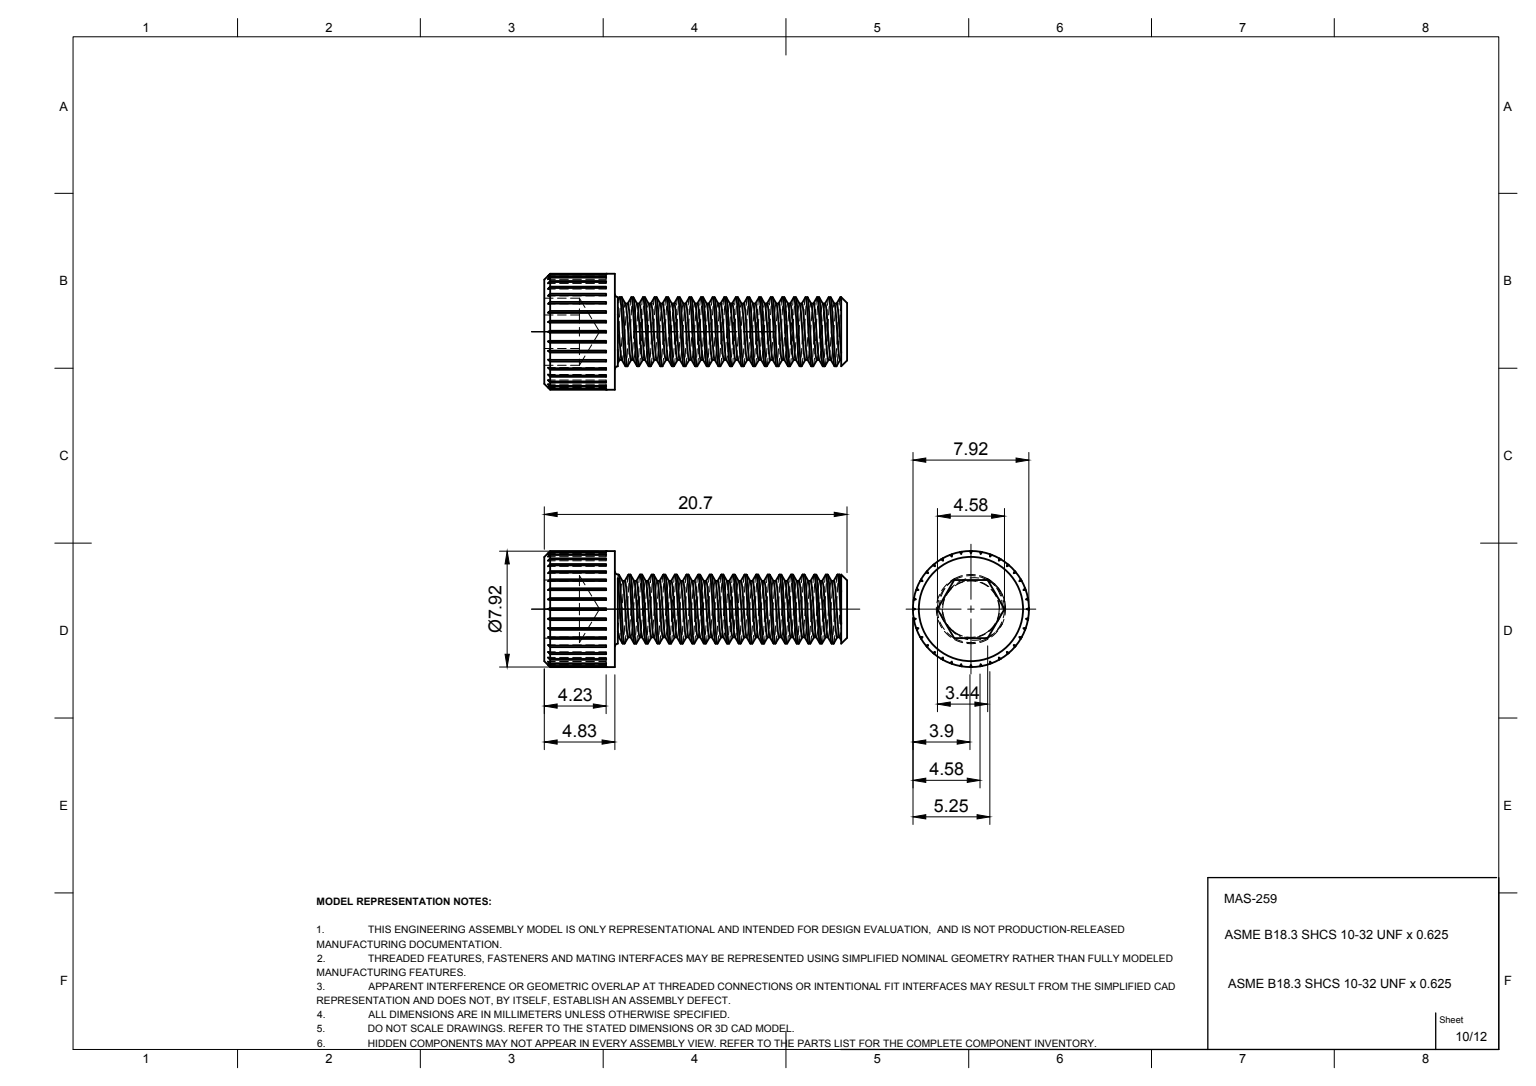
ISO-10303-21;
HEADER;
/* Generated by software containing ST-Developer
 * from STEP Tools, Inc. (www.steptools.com) 
 */

FILE_DESCRIPTION(
/* description */ (''),
/* implementation_level */ '2;1');

FILE_NAME(
/* name */ 'ASME B18.3 SHCS 10-32 UNF x 0.625.step',
/* time_stamp */ '2026-10-15T13:30:17-07:00',
/* author */ (''),
/* organization */ (''),
/* preprocessor_version */ 'ST-DEVELOPER v20.2',
/* originating_system */ 'Autodesk Translation Framework v15.15.0.0',
/* authorisation */ '');

FILE_SCHEMA (('AUTOMOTIVE_DESIGN { 1 0 10303 214 3 1 1 }'));
ENDSEC;

DATA;
#10=MECHANICAL_DESIGN_GEOMETRIC_PRESENTATION_REPRESENTATION('',(#1040),#71795);
#787=(
BOUNDED_CURVE()
B_SPLINE_CURVE(2,(#36530,#36531,#36532),.UNSPECIFIED.,.F.,.F.)
B_SPLINE_CURVE_WITH_KNOTS((3,3),(0.,0.021388782715503),.UNSPECIFIED.)
CURVE()
GEOMETRIC_REPRESENTATION_ITEM()
RATIONAL_B_SPLINE_CURVE((1.,1.00061453665269,1.00078646015663))
REPRESENTATION_ITEM('')
);
#788=(
BOUNDED_CURVE()
B_SPLINE_CURVE(2,(#36537,#36538,#36539),.UNSPECIFIED.,.F.,.F.)
B_SPLINE_CURVE_WITH_KNOTS((3,3),(0.0380048027322982,0.0593935854477557),
 .UNSPECIFIED.)
CURVE()
GEOMETRIC_REPRESENTATION_ITEM()
RATIONAL_B_SPLINE_CURVE((1.00078646015529,1.00061453665164,1.))
REPRESENTATION_ITEM('')
);
#789=(
BOUNDED_CURVE()
B_SPLINE_CURVE(2,(#36546,#36547,#36548),.UNSPECIFIED.,.F.,.F.)
B_SPLINE_CURVE_WITH_KNOTS((3,3),(0.0380048027323146,0.0593935854477557),
 .UNSPECIFIED.)
CURVE()
GEOMETRIC_REPRESENTATION_ITEM()
RATIONAL_B_SPLINE_CURVE((1.00078646015801,1.00061453665376,1.))
REPRESENTATION_ITEM('')
);
#790=(
BOUNDED_CURVE()
B_SPLINE_CURVE(2,(#36552,#36553,#36554),.UNSPECIFIED.,.F.,.F.)
B_SPLINE_CURVE_WITH_KNOTS((3,3),(0.,0.0213887827155079),.UNSPECIFIED.)
CURVE()
GEOMETRIC_REPRESENTATION_ITEM()
RATIONAL_B_SPLINE_CURVE((1.,1.00061453665303,1.00078646015707))
REPRESENTATION_ITEM('')
);
#791=(
BOUNDED_CURVE()
B_SPLINE_CURVE(2,(#36556,#36557,#36558),.UNSPECIFIED.,.F.,.F.)
B_SPLINE_CURVE_WITH_KNOTS((3,3),(0.03800480273222,0.0593935854477558),
 .UNSPECIFIED.)
CURVE()
GEOMETRIC_REPRESENTATION_ITEM()
RATIONAL_B_SPLINE_CURVE((1.00078646015217,1.0006145366492,1.))
REPRESENTATION_ITEM('')
);
#792=(
BOUNDED_CURVE()
B_SPLINE_CURVE(2,(#36562,#36563,#36564),.UNSPECIFIED.,.F.,.F.)
B_SPLINE_CURVE_WITH_KNOTS((3,3),(0.,0.0213887827155065),.UNSPECIFIED.)
CURVE()
GEOMETRIC_REPRESENTATION_ITEM()
RATIONAL_B_SPLINE_CURVE((1.,1.00061453664751,1.00078646015))
REPRESENTATION_ITEM('')
);
#793=(
BOUNDED_CURVE()
B_SPLINE_CURVE(2,(#36566,#36567,#36568),.UNSPECIFIED.,.F.,.F.)
B_SPLINE_CURVE_WITH_KNOTS((3,3),(0.0380048027322497,0.0593935854477559),
 .UNSPECIFIED.)
CURVE()
GEOMETRIC_REPRESENTATION_ITEM()
RATIONAL_B_SPLINE_CURVE((1.00078646015691,1.00061453665291,1.))
REPRESENTATION_ITEM('')
);
#794=(
BOUNDED_CURVE()
B_SPLINE_CURVE(2,(#36572,#36573,#36574),.UNSPECIFIED.,.F.,.F.)
B_SPLINE_CURVE_WITH_KNOTS((3,3),(0.,0.0213887827155146),.UNSPECIFIED.)
CURVE()
GEOMETRIC_REPRESENTATION_ITEM()
RATIONAL_B_SPLINE_CURVE((1.,1.00061453665095,1.00078646015441))
REPRESENTATION_ITEM('')
);
#795=(
BOUNDED_CURVE()
B_SPLINE_CURVE(2,(#36576,#36577,#36578),.UNSPECIFIED.,.F.,.F.)
B_SPLINE_CURVE_WITH_KNOTS((3,3),(0.0380048027321657,0.0593935854477561),
 .UNSPECIFIED.)
CURVE()
GEOMETRIC_REPRESENTATION_ITEM()
RATIONAL_B_SPLINE_CURVE((1.00078646014826,1.00061453664614,1.))
REPRESENTATION_ITEM('')
);
#796=(
BOUNDED_CURVE()
B_SPLINE_CURVE(2,(#36582,#36583,#36584),.UNSPECIFIED.,.F.,.F.)
B_SPLINE_CURVE_WITH_KNOTS((3,3),(0.,0.0213887827154277),.UNSPECIFIED.)
CURVE()
GEOMETRIC_REPRESENTATION_ITEM()
RATIONAL_B_SPLINE_CURVE((1.,1.00061453665233,1.00078646015617))
REPRESENTATION_ITEM('')
);
#797=(
BOUNDED_CURVE()
B_SPLINE_CURVE(2,(#36586,#36587,#36588),.UNSPECIFIED.,.F.,.F.)
B_SPLINE_CURVE_WITH_KNOTS((3,3),(0.0380048027322445,0.0593935854477552),
 .UNSPECIFIED.)
CURVE()
GEOMETRIC_REPRESENTATION_ITEM()
RATIONAL_B_SPLINE_CURVE((1.00078646015087,1.00061453664819,1.))
REPRESENTATION_ITEM('')
);
#798=(
BOUNDED_CURVE()
B_SPLINE_CURVE(2,(#36592,#36593,#36594),.UNSPECIFIED.,.F.,.F.)
B_SPLINE_CURVE_WITH_KNOTS((3,3),(0.,0.0213887827154996),.UNSPECIFIED.)
CURVE()
GEOMETRIC_REPRESENTATION_ITEM()
RATIONAL_B_SPLINE_CURVE((1.,1.00061453665179,1.00078646015549))
REPRESENTATION_ITEM('')
);
#799=(
BOUNDED_CURVE()
B_SPLINE_CURVE(2,(#36596,#36597,#36598),.UNSPECIFIED.,.F.,.F.)
B_SPLINE_CURVE_WITH_KNOTS((3,3),(0.0380048027322845,0.0593935854477556),
 .UNSPECIFIED.)
CURVE()
GEOMETRIC_REPRESENTATION_ITEM()
RATIONAL_B_SPLINE_CURVE((1.00078646015637,1.00061453665248,1.))
REPRESENTATION_ITEM('')
);
#800=(
BOUNDED_CURVE()
B_SPLINE_CURVE(2,(#36602,#36603,#36604),.UNSPECIFIED.,.F.,.F.)
B_SPLINE_CURVE_WITH_KNOTS((3,3),(0.,0.0213887827155547),.UNSPECIFIED.)
CURVE()
GEOMETRIC_REPRESENTATION_ITEM()
RATIONAL_B_SPLINE_CURVE((1.,1.00061453664528,1.00078646014716))
REPRESENTATION_ITEM('')
);
#801=(
BOUNDED_CURVE()
B_SPLINE_CURVE(2,(#36606,#36607,#36608),.UNSPECIFIED.,.F.,.F.)
B_SPLINE_CURVE_WITH_KNOTS((3,3),(0.0380048027322622,0.0593935854477563),
 .UNSPECIFIED.)
CURVE()
GEOMETRIC_REPRESENTATION_ITEM()
RATIONAL_B_SPLINE_CURVE((1.0007864601608,1.00061453665594,1.))
REPRESENTATION_ITEM('')
);
#802=(
BOUNDED_CURVE()
B_SPLINE_CURVE(2,(#36612,#36613,#36614),.UNSPECIFIED.,.F.,.F.)
B_SPLINE_CURVE_WITH_KNOTS((3,3),(0.,0.021388782715527),.UNSPECIFIED.)
CURVE()
GEOMETRIC_REPRESENTATION_ITEM()
RATIONAL_B_SPLINE_CURVE((1.,1.00061453664858,1.00078646015138))
REPRESENTATION_ITEM('')
);
#803=(
BOUNDED_CURVE()
B_SPLINE_CURVE(2,(#36616,#36617,#36618),.UNSPECIFIED.,.F.,.F.)
B_SPLINE_CURVE_WITH_KNOTS((3,3),(0.0380048027322087,0.0593935854477563),
 .UNSPECIFIED.)
CURVE()
GEOMETRIC_REPRESENTATION_ITEM()
RATIONAL_B_SPLINE_CURVE((1.00078646015349,1.00061453665023,1.))
REPRESENTATION_ITEM('')
);
#804=(
BOUNDED_CURVE()
B_SPLINE_CURVE(2,(#36622,#36623,#36624),.UNSPECIFIED.,.F.,.F.)
B_SPLINE_CURVE_WITH_KNOTS((3,3),(0.,0.0213887827155107),.UNSPECIFIED.)
CURVE()
GEOMETRIC_REPRESENTATION_ITEM()
RATIONAL_B_SPLINE_CURVE((1.,1.00061453665077,1.00078646015419))
REPRESENTATION_ITEM('')
);
#805=(
BOUNDED_CURVE()
B_SPLINE_CURVE(2,(#36626,#36627,#36628),.UNSPECIFIED.,.F.,.F.)
B_SPLINE_CURVE_WITH_KNOTS((3,3),(0.0380048027321878,0.0593935854477555),
 .UNSPECIFIED.)
CURVE()
GEOMETRIC_REPRESENTATION_ITEM()
RATIONAL_B_SPLINE_CURVE((1.00078646014641,1.0006145366447,1.))
REPRESENTATION_ITEM('')
);
#806=(
BOUNDED_CURVE()
B_SPLINE_CURVE(2,(#36632,#36633,#36634),.UNSPECIFIED.,.F.,.F.)
B_SPLINE_CURVE_WITH_KNOTS((3,3),(0.,0.0213887827154949),.UNSPECIFIED.)
CURVE()
GEOMETRIC_REPRESENTATION_ITEM()
RATIONAL_B_SPLINE_CURVE((1.,1.00061453665079,1.00078646015421))
REPRESENTATION_ITEM('')
);
#807=(
BOUNDED_CURVE()
B_SPLINE_CURVE(2,(#36636,#36637,#36638),.UNSPECIFIED.,.F.,.F.)
B_SPLINE_CURVE_WITH_KNOTS((3,3),(0.038004802732195,0.0593935854477556),
 .UNSPECIFIED.)
CURVE()
GEOMETRIC_REPRESENTATION_ITEM()
RATIONAL_B_SPLINE_CURVE((1.0007864601493,1.00061453664696,1.))
REPRESENTATION_ITEM('')
);
#808=(
BOUNDED_CURVE()
B_SPLINE_CURVE(2,(#36642,#36643,#36644),.UNSPECIFIED.,.F.,.F.)
B_SPLINE_CURVE_WITH_KNOTS((3,3),(0.,0.0213887827155322),.UNSPECIFIED.)
CURVE()
GEOMETRIC_REPRESENTATION_ITEM()
RATIONAL_B_SPLINE_CURVE((1.,1.00061453664703,1.00078646014939))
REPRESENTATION_ITEM('')
);
#809=(
BOUNDED_CURVE()
B_SPLINE_CURVE(2,(#36646,#36647,#36648),.UNSPECIFIED.,.F.,.F.)
B_SPLINE_CURVE_WITH_KNOTS((3,3),(0.0380048027322535,0.0593935854477551),
 .UNSPECIFIED.)
CURVE()
GEOMETRIC_REPRESENTATION_ITEM()
RATIONAL_B_SPLINE_CURVE((1.00078646015018,1.00061453664765,1.))
REPRESENTATION_ITEM('')
);
#810=(
BOUNDED_CURVE()
B_SPLINE_CURVE(2,(#36652,#36653,#36654),.UNSPECIFIED.,.F.,.F.)
B_SPLINE_CURVE_WITH_KNOTS((3,3),(0.,0.0213887827155291),.UNSPECIFIED.)
CURVE()
GEOMETRIC_REPRESENTATION_ITEM()
RATIONAL_B_SPLINE_CURVE((1.,1.00061453664596,1.00078646014803))
REPRESENTATION_ITEM('')
);
#811=(
BOUNDED_CURVE()
B_SPLINE_CURVE(2,(#36656,#36657,#36658),.UNSPECIFIED.,.F.,.F.)
B_SPLINE_CURVE_WITH_KNOTS((3,3),(0.0380048027322346,0.0593935854477561),
 .UNSPECIFIED.)
CURVE()
GEOMETRIC_REPRESENTATION_ITEM()
RATIONAL_B_SPLINE_CURVE((1.00078646015205,1.00061453664911,1.))
REPRESENTATION_ITEM('')
);
#812=(
BOUNDED_CURVE()
B_SPLINE_CURVE(2,(#36662,#36663,#36664),.UNSPECIFIED.,.F.,.F.)
B_SPLINE_CURVE_WITH_KNOTS((3,3),(0.,0.0213887827155096),.UNSPECIFIED.)
CURVE()
GEOMETRIC_REPRESENTATION_ITEM()
RATIONAL_B_SPLINE_CURVE((1.,1.00061453664827,1.00078646015098))
REPRESENTATION_ITEM('')
);
#813=(
BOUNDED_CURVE()
B_SPLINE_CURVE(2,(#36666,#36667,#36668),.UNSPECIFIED.,.F.,.F.)
B_SPLINE_CURVE_WITH_KNOTS((3,3),(0.0380048027322829,0.0593935854477556),
 .UNSPECIFIED.)
CURVE()
GEOMETRIC_REPRESENTATION_ITEM()
RATIONAL_B_SPLINE_CURVE((1.00078646015816,1.00061453665388,1.))
REPRESENTATION_ITEM('')
);
#814=(
BOUNDED_CURVE()
B_SPLINE_CURVE(2,(#36672,#36673,#36674),.UNSPECIFIED.,.F.,.F.)
B_SPLINE_CURVE_WITH_KNOTS((3,3),(0.,0.0213887827155543),.UNSPECIFIED.)
CURVE()
GEOMETRIC_REPRESENTATION_ITEM()
RATIONAL_B_SPLINE_CURVE((1.,1.00061453664662,1.00078646014886))
REPRESENTATION_ITEM('')
);
#815=(
BOUNDED_CURVE()
B_SPLINE_CURVE(2,(#36676,#36677,#36678),.UNSPECIFIED.,.F.,.F.)
B_SPLINE_CURVE_WITH_KNOTS((3,3),(0.038004802732242,0.0593935854477554),
 .UNSPECIFIED.)
CURVE()
GEOMETRIC_REPRESENTATION_ITEM()
RATIONAL_B_SPLINE_CURVE((1.00078646015479,1.00061453665125,1.))
REPRESENTATION_ITEM('')
);
#816=(
BOUNDED_CURVE()
B_SPLINE_CURVE(2,(#36682,#36683,#36684),.UNSPECIFIED.,.F.,.F.)
B_SPLINE_CURVE_WITH_KNOTS((3,3),(0.,0.0213887827155011),.UNSPECIFIED.)
CURVE()
GEOMETRIC_REPRESENTATION_ITEM()
RATIONAL_B_SPLINE_CURVE((1.,1.00061453665297,1.000786460157))
REPRESENTATION_ITEM('')
);
#817=(
BOUNDED_CURVE()
B_SPLINE_CURVE(2,(#36686,#36687,#36688),.UNSPECIFIED.,.F.,.F.)
B_SPLINE_CURVE_WITH_KNOTS((3,3),(0.0380048027323167,0.0593935854477549),
 .UNSPECIFIED.)
CURVE()
GEOMETRIC_REPRESENTATION_ITEM()
RATIONAL_B_SPLINE_CURVE((1.00078646015665,1.0006145366527,1.))
REPRESENTATION_ITEM('')
);
#818=(
BOUNDED_CURVE()
B_SPLINE_CURVE(2,(#36692,#36693,#36694),.UNSPECIFIED.,.F.,.F.)
B_SPLINE_CURVE_WITH_KNOTS((3,3),(0.,0.0213887827155084),.UNSPECIFIED.)
CURVE()
GEOMETRIC_REPRESENTATION_ITEM()
RATIONAL_B_SPLINE_CURVE((1.,1.00061453665162,1.00078646015527))
REPRESENTATION_ITEM('')
);
#819=(
BOUNDED_CURVE()
B_SPLINE_CURVE(2,(#36696,#36697,#36698),.UNSPECIFIED.,.F.,.F.)
B_SPLINE_CURVE_WITH_KNOTS((3,3),(0.0380048027322826,0.0593935854477556),
 .UNSPECIFIED.)
CURVE()
GEOMETRIC_REPRESENTATION_ITEM()
RATIONAL_B_SPLINE_CURVE((1.00078646015745,1.00061453665332,1.))
REPRESENTATION_ITEM('')
);
#820=(
BOUNDED_CURVE()
B_SPLINE_CURVE(2,(#36702,#36703,#36704),.UNSPECIFIED.,.F.,.F.)
B_SPLINE_CURVE_WITH_KNOTS((3,3),(0.,0.0213887827154213),.UNSPECIFIED.)
CURVE()
GEOMETRIC_REPRESENTATION_ITEM()
RATIONAL_B_SPLINE_CURVE((1.,1.00061453665618,1.00078646016111))
REPRESENTATION_ITEM('')
);
#821=(
BOUNDED_CURVE()
B_SPLINE_CURVE(2,(#36706,#36707,#36708),.UNSPECIFIED.,.F.,.F.)
B_SPLINE_CURVE_WITH_KNOTS((3,3),(0.0380048027322973,0.0593935854477563),
 .UNSPECIFIED.)
CURVE()
GEOMETRIC_REPRESENTATION_ITEM()
RATIONAL_B_SPLINE_CURVE((1.00078646016316,1.00061453665778,1.))
REPRESENTATION_ITEM('')
);
#822=(
BOUNDED_CURVE()
B_SPLINE_CURVE(2,(#36712,#36713,#36714),.UNSPECIFIED.,.F.,.F.)
B_SPLINE_CURVE_WITH_KNOTS((3,3),(0.,0.0213887827154844),.UNSPECIFIED.)
CURVE()
GEOMETRIC_REPRESENTATION_ITEM()
RATIONAL_B_SPLINE_CURVE((1.,1.00061453665096,1.00078646015442))
REPRESENTATION_ITEM('')
);
#823=(
BOUNDED_CURVE()
B_SPLINE_CURVE(2,(#36716,#36717,#36718),.UNSPECIFIED.,.F.,.F.)
B_SPLINE_CURVE_WITH_KNOTS((3,3),(0.0380048027322098,0.0593935854477563),
 .UNSPECIFIED.)
CURVE()
GEOMETRIC_REPRESENTATION_ITEM()
RATIONAL_B_SPLINE_CURVE((1.0007864601532,1.00061453665,1.))
REPRESENTATION_ITEM('')
);
#824=(
BOUNDED_CURVE()
B_SPLINE_CURVE(2,(#36722,#36723,#36724),.UNSPECIFIED.,.F.,.F.)
B_SPLINE_CURVE_WITH_KNOTS((3,3),(0.,0.0213887827154289),.UNSPECIFIED.)
CURVE()
GEOMETRIC_REPRESENTATION_ITEM()
RATIONAL_B_SPLINE_CURVE((1.,1.00061453665625,1.0007864601612))
REPRESENTATION_ITEM('')
);
#825=(
BOUNDED_CURVE()
B_SPLINE_CURVE(2,(#36726,#36727,#36728),.UNSPECIFIED.,.F.,.F.)
B_SPLINE_CURVE_WITH_KNOTS((3,3),(0.0380048027322686,0.0593935854477554),
 .UNSPECIFIED.)
CURVE()
GEOMETRIC_REPRESENTATION_ITEM()
RATIONAL_B_SPLINE_CURVE((1.00078646015899,1.00061453665453,1.))
REPRESENTATION_ITEM('')
);
#826=(
BOUNDED_CURVE()
B_SPLINE_CURVE(2,(#36733,#36734,#36735),.UNSPECIFIED.,.F.,.F.)
B_SPLINE_CURVE_WITH_KNOTS((3,3),(0.,0.0213887827155324),.UNSPECIFIED.)
CURVE()
GEOMETRIC_REPRESENTATION_ITEM()
RATIONAL_B_SPLINE_CURVE((1.,1.00061453664729,1.00078646014973))
REPRESENTATION_ITEM('')
);
#827=(
BOUNDED_CURVE()
B_SPLINE_CURVE(2,(#36737,#36738,#36739),.UNSPECIFIED.,.F.,.F.)
B_SPLINE_CURVE_WITH_KNOTS((3,3),(0.0380048027322402,0.0593935854477561),
 .UNSPECIFIED.)
CURVE()
GEOMETRIC_REPRESENTATION_ITEM()
RATIONAL_B_SPLINE_CURVE((1.00078646015472,1.00061453665119,1.))
REPRESENTATION_ITEM('')
);
#828=(
BOUNDED_CURVE()
B_SPLINE_CURVE(2,(#36743,#36744,#36745),.UNSPECIFIED.,.F.,.F.)
B_SPLINE_CURVE_WITH_KNOTS((3,3),(0.,0.0213887827154487),.UNSPECIFIED.)
CURVE()
GEOMETRIC_REPRESENTATION_ITEM()
RATIONAL_B_SPLINE_CURVE((1.,1.00061453665353,1.00078646015771))
REPRESENTATION_ITEM('')
);
#829=(
BOUNDED_CURVE()
B_SPLINE_CURVE(2,(#36747,#36748,#36749),.UNSPECIFIED.,.F.,.F.)
B_SPLINE_CURVE_WITH_KNOTS((3,3),(0.0380048027323105,0.0593935854477551),
 .UNSPECIFIED.)
CURVE()
GEOMETRIC_REPRESENTATION_ITEM()
RATIONAL_B_SPLINE_CURVE((1.00078646015948,1.00061453665491,1.))
REPRESENTATION_ITEM('')
);
#830=(
BOUNDED_CURVE()
B_SPLINE_CURVE(2,(#36753,#36754,#36755),.UNSPECIFIED.,.F.,.F.)
B_SPLINE_CURVE_WITH_KNOTS((3,3),(0.,0.0213887827154801),.UNSPECIFIED.)
CURVE()
GEOMETRIC_REPRESENTATION_ITEM()
RATIONAL_B_SPLINE_CURVE((1.,1.00061453665439,1.00078646015881))
REPRESENTATION_ITEM('')
);
#831=(
BOUNDED_CURVE()
B_SPLINE_CURVE(2,(#36757,#36758,#36759),.UNSPECIFIED.,.F.,.F.)
B_SPLINE_CURVE_WITH_KNOTS((3,3),(0.0380048027322703,0.0593935854477551),
 .UNSPECIFIED.)
CURVE()
GEOMETRIC_REPRESENTATION_ITEM()
RATIONAL_B_SPLINE_CURVE((1.00078646015419,1.00061453665078,1.))
REPRESENTATION_ITEM('')
);
#832=(
BOUNDED_CURVE()
B_SPLINE_CURVE(2,(#36763,#36764,#36765),.UNSPECIFIED.,.F.,.F.)
B_SPLINE_CURVE_WITH_KNOTS((3,3),(0.,0.0213887827154732),.UNSPECIFIED.)
CURVE()
GEOMETRIC_REPRESENTATION_ITEM()
RATIONAL_B_SPLINE_CURVE((1.,1.00061453665189,1.00078646015561))
REPRESENTATION_ITEM('')
);
#833=(
BOUNDED_CURVE()
B_SPLINE_CURVE(2,(#36767,#36768,#36769),.UNSPECIFIED.,.F.,.F.)
B_SPLINE_CURVE_WITH_KNOTS((3,3),(0.0380048027323814,0.0593935854477557),
 .UNSPECIFIED.)
CURVE()
GEOMETRIC_REPRESENTATION_ITEM()
RATIONAL_B_SPLINE_CURVE((1.00078646016718,1.00061453666093,1.))
REPRESENTATION_ITEM('')
);
#834=(
BOUNDED_CURVE()
B_SPLINE_CURVE(2,(#36773,#36774,#36775),.UNSPECIFIED.,.F.,.F.)
B_SPLINE_CURVE_WITH_KNOTS((3,3),(0.,0.0213887827155284),.UNSPECIFIED.)
CURVE()
GEOMETRIC_REPRESENTATION_ITEM()
RATIONAL_B_SPLINE_CURVE((1.,1.00061453664637,1.00078646014855))
REPRESENTATION_ITEM('')
);
#835=(
BOUNDED_CURVE()
B_SPLINE_CURVE(2,(#36777,#36778,#36779),.UNSPECIFIED.,.F.,.F.)
B_SPLINE_CURVE_WITH_KNOTS((3,3),(0.0380048027322513,0.0593935854477563),
 .UNSPECIFIED.)
CURVE()
GEOMETRIC_REPRESENTATION_ITEM()
RATIONAL_B_SPLINE_CURVE((1.00078646015572,1.00061453665197,1.))
REPRESENTATION_ITEM('')
);
#836=(
BOUNDED_CURVE()
B_SPLINE_CURVE(2,(#36783,#36784,#36785),.UNSPECIFIED.,.F.,.F.)
B_SPLINE_CURVE_WITH_KNOTS((3,3),(0.,0.0213887827154905),.UNSPECIFIED.)
CURVE()
GEOMETRIC_REPRESENTATION_ITEM()
RATIONAL_B_SPLINE_CURVE((1.,1.00061453665389,1.00078646015818))
REPRESENTATION_ITEM('')
);
#837=(
BOUNDED_CURVE()
B_SPLINE_CURVE(2,(#36787,#36788,#36789),.UNSPECIFIED.,.F.,.F.)
B_SPLINE_CURVE_WITH_KNOTS((3,3),(0.0380048027322515,0.0593935854477557),
 .UNSPECIFIED.)
CURVE()
GEOMETRIC_REPRESENTATION_ITEM()
RATIONAL_B_SPLINE_CURVE((1.00078646015577,1.00061453665201,1.))
REPRESENTATION_ITEM('')
);
#838=(
BOUNDED_CURVE()
B_SPLINE_CURVE(2,(#36793,#36794,#36795),.UNSPECIFIED.,.F.,.F.)
B_SPLINE_CURVE_WITH_KNOTS((3,3),(0.,0.0213887827155349),.UNSPECIFIED.)
CURVE()
GEOMETRIC_REPRESENTATION_ITEM()
RATIONAL_B_SPLINE_CURVE((1.,1.00061453664595,1.000786460148))
REPRESENTATION_ITEM('')
);
#839=(
BOUNDED_CURVE()
B_SPLINE_CURVE(2,(#36797,#36798,#36799),.UNSPECIFIED.,.F.,.F.)
B_SPLINE_CURVE_WITH_KNOTS((3,3),(0.0380048027322051,0.0593935854477563),
 .UNSPECIFIED.)
CURVE()
GEOMETRIC_REPRESENTATION_ITEM()
RATIONAL_B_SPLINE_CURVE((1.00078646015312,1.00061453664994,1.))
REPRESENTATION_ITEM('')
);
#840=(
BOUNDED_CURVE()
B_SPLINE_CURVE(2,(#36803,#36804,#36805),.UNSPECIFIED.,.F.,.F.)
B_SPLINE_CURVE_WITH_KNOTS((3,3),(0.,0.0213887827155927),.UNSPECIFIED.)
CURVE()
GEOMETRIC_REPRESENTATION_ITEM()
RATIONAL_B_SPLINE_CURVE((1.,1.00061453664415,1.0007864601457))
REPRESENTATION_ITEM('')
);
#841=(
BOUNDED_CURVE()
B_SPLINE_CURVE(2,(#36807,#36808,#36809),.UNSPECIFIED.,.F.,.F.)
B_SPLINE_CURVE_WITH_KNOTS((3,3),(0.038004802732226,0.0593935854477556),
 .UNSPECIFIED.)
CURVE()
GEOMETRIC_REPRESENTATION_ITEM()
RATIONAL_B_SPLINE_CURVE((1.0007864601527,1.00061453664962,1.))
REPRESENTATION_ITEM('')
);
#842=(
BOUNDED_CURVE()
B_SPLINE_CURVE(2,(#36813,#36814,#36815),.UNSPECIFIED.,.F.,.F.)
B_SPLINE_CURVE_WITH_KNOTS((3,3),(0.,0.0213887827155911),.UNSPECIFIED.)
CURVE()
GEOMETRIC_REPRESENTATION_ITEM()
RATIONAL_B_SPLINE_CURVE((1.,1.00061453664496,1.00078646014675))
REPRESENTATION_ITEM('')
);
#843=(
BOUNDED_CURVE()
B_SPLINE_CURVE(2,(#36817,#36818,#36819),.UNSPECIFIED.,.F.,.F.)
B_SPLINE_CURVE_WITH_KNOTS((3,3),(0.0380048027321543,0.059393585447757),
 .UNSPECIFIED.)
CURVE()
GEOMETRIC_REPRESENTATION_ITEM()
RATIONAL_B_SPLINE_CURVE((1.0007864601479,1.00061453664586,1.))
REPRESENTATION_ITEM('')
);
#844=(
BOUNDED_CURVE()
B_SPLINE_CURVE(2,(#36823,#36824,#36825),.UNSPECIFIED.,.F.,.F.)
B_SPLINE_CURVE_WITH_KNOTS((3,3),(0.,0.0213887827155128),.UNSPECIFIED.)
CURVE()
GEOMETRIC_REPRESENTATION_ITEM()
RATIONAL_B_SPLINE_CURVE((1.,1.00061453664886,1.00078646015173))
REPRESENTATION_ITEM('')
);
#845=(
BOUNDED_CURVE()
B_SPLINE_CURVE(2,(#36827,#36828,#36829),.UNSPECIFIED.,.F.,.F.)
B_SPLINE_CURVE_WITH_KNOTS((3,3),(0.0380048027322768,0.0593935854477557),
 .UNSPECIFIED.)
CURVE()
GEOMETRIC_REPRESENTATION_ITEM()
RATIONAL_B_SPLINE_CURVE((1.00078646015618,1.00061453665233,1.))
REPRESENTATION_ITEM('')
);
#846=(
BOUNDED_CURVE()
B_SPLINE_CURVE(2,(#36833,#36834,#36835),.UNSPECIFIED.,.F.,.F.)
B_SPLINE_CURVE_WITH_KNOTS((3,3),(0.,0.0213887827155095),.UNSPECIFIED.)
CURVE()
GEOMETRIC_REPRESENTATION_ITEM()
RATIONAL_B_SPLINE_CURVE((1.,1.00061453664827,1.00078646015098))
REPRESENTATION_ITEM('')
);
#847=(
BOUNDED_CURVE()
B_SPLINE_CURVE(2,(#36837,#36838,#36839),.UNSPECIFIED.,.F.,.F.)
B_SPLINE_CURVE_WITH_KNOTS((3,3),(0.0380048027321875,0.0593935854477551),
 .UNSPECIFIED.)
CURVE()
GEOMETRIC_REPRESENTATION_ITEM()
RATIONAL_B_SPLINE_CURVE((1.00078646014592,1.00061453664432,1.))
REPRESENTATION_ITEM('')
);
#848=(
BOUNDED_CURVE()
B_SPLINE_CURVE(2,(#36843,#36844,#36845),.UNSPECIFIED.,.F.,.F.)
B_SPLINE_CURVE_WITH_KNOTS((3,3),(0.,0.0213887827154677),.UNSPECIFIED.)
CURVE()
GEOMETRIC_REPRESENTATION_ITEM()
RATIONAL_B_SPLINE_CURVE((1.,1.00061453665162,1.00078646015527))
REPRESENTATION_ITEM('')
);
#849=(
BOUNDED_CURVE()
B_SPLINE_CURVE(2,(#36847,#36848,#36849),.UNSPECIFIED.,.F.,.F.)
B_SPLINE_CURVE_WITH_KNOTS((3,3),(0.0380048027322803,0.059393585447756),
 .UNSPECIFIED.)
CURVE()
GEOMETRIC_REPRESENTATION_ITEM()
RATIONAL_B_SPLINE_CURVE((1.00078646015832,1.000614536654,1.))
REPRESENTATION_ITEM('')
);
#850=(
BOUNDED_CURVE()
B_SPLINE_CURVE(2,(#36853,#36854,#36855),.UNSPECIFIED.,.F.,.F.)
B_SPLINE_CURVE_WITH_KNOTS((3,3),(0.,0.0213887827154919),.UNSPECIFIED.)
CURVE()
GEOMETRIC_REPRESENTATION_ITEM()
RATIONAL_B_SPLINE_CURVE((1.,1.00061453665363,1.00078646015784))
REPRESENTATION_ITEM('')
);
#851=(
BOUNDED_CURVE()
B_SPLINE_CURVE(2,(#36857,#36858,#36859),.UNSPECIFIED.,.F.,.F.)
B_SPLINE_CURVE_WITH_KNOTS((3,3),(0.0380048027322449,0.0593935854477551),
 .UNSPECIFIED.)
CURVE()
GEOMETRIC_REPRESENTATION_ITEM()
RATIONAL_B_SPLINE_CURVE((1.00078646015292,1.00061453664979,1.))
REPRESENTATION_ITEM('')
);
#852=(
BOUNDED_CURVE()
B_SPLINE_CURVE(2,(#36863,#36864,#36865),.UNSPECIFIED.,.F.,.F.)
B_SPLINE_CURVE_WITH_KNOTS((3,3),(0.,0.021388782715506),.UNSPECIFIED.)
CURVE()
GEOMETRIC_REPRESENTATION_ITEM()
RATIONAL_B_SPLINE_CURVE((1.,1.00061453665225,1.00078646015607))
REPRESENTATION_ITEM('')
);
#853=(
BOUNDED_CURVE()
B_SPLINE_CURVE(2,(#36867,#36868,#36869),.UNSPECIFIED.,.F.,.F.)
B_SPLINE_CURVE_WITH_KNOTS((3,3),(0.0380048027322685,0.0593935854477556),
 .UNSPECIFIED.)
CURVE()
GEOMETRIC_REPRESENTATION_ITEM()
RATIONAL_B_SPLINE_CURVE((1.00078646015217,1.0006145366492,1.))
REPRESENTATION_ITEM('')
);
#854=(
BOUNDED_CURVE()
B_SPLINE_CURVE(2,(#36873,#36874,#36875),.UNSPECIFIED.,.F.,.F.)
B_SPLINE_CURVE_WITH_KNOTS((3,3),(0.,0.0213887827154673),.UNSPECIFIED.)
CURVE()
GEOMETRIC_REPRESENTATION_ITEM()
RATIONAL_B_SPLINE_CURVE((1.,1.00061453665233,1.00078646015618))
REPRESENTATION_ITEM('')
);
#855=(
BOUNDED_CURVE()
B_SPLINE_CURVE(2,(#36877,#36878,#36879),.UNSPECIFIED.,.F.,.F.)
B_SPLINE_CURVE_WITH_KNOTS((3,3),(0.0380048027322247,0.059393585447756),
 .UNSPECIFIED.)
CURVE()
GEOMETRIC_REPRESENTATION_ITEM()
RATIONAL_B_SPLINE_CURVE((1.00078646015399,1.00061453665062,1.))
REPRESENTATION_ITEM('')
);
#856=(
BOUNDED_CURVE()
B_SPLINE_CURVE(2,(#36883,#36884,#36885),.UNSPECIFIED.,.F.,.F.)
B_SPLINE_CURVE_WITH_KNOTS((3,3),(0.,0.0213887827154374),.UNSPECIFIED.)
CURVE()
GEOMETRIC_REPRESENTATION_ITEM()
RATIONAL_B_SPLINE_CURVE((1.,1.00061453665411,1.00078646015846))
REPRESENTATION_ITEM('')
);
#857=(
BOUNDED_CURVE()
B_SPLINE_CURVE(2,(#36887,#36888,#36889),.UNSPECIFIED.,.F.,.F.)
B_SPLINE_CURVE_WITH_KNOTS((3,3),(0.0380048027322071,0.0593935854477556),
 .UNSPECIFIED.)
CURVE()
GEOMETRIC_REPRESENTATION_ITEM()
RATIONAL_B_SPLINE_CURVE((1.00078646015371,1.0006145366504,1.))
REPRESENTATION_ITEM('')
);
#858=(
BOUNDED_CURVE()
B_SPLINE_CURVE(2,(#36892,#36893,#36894),.UNSPECIFIED.,.F.,.F.)
B_SPLINE_CURVE_WITH_KNOTS((3,3),(0.,0.0213887827155641),.UNSPECIFIED.)
CURVE()
GEOMETRIC_REPRESENTATION_ITEM()
RATIONAL_B_SPLINE_CURVE((1.,1.00061453664786,1.00078646015045))
REPRESENTATION_ITEM('')
);
#1003=TOROIDAL_SURFACE('',#14146,2.56347,0.2);
#1006=B_SPLINE_SURFACE_WITH_KNOTS('',3,3,((#35331,#35332,#35333,#35334,
#35335,#35336,#35337,#35338,#35339,#35340,#35341,#35342,#35343,#35344,#35345,
#35346,#35347,#35348,#35349,#35350,#35351,#35352,#35353,#35354,#35355,#35356,
#35357,#35358,#35359,#35360,#35361,#35362,#35363,#35364,#35365,#35366,#35367,
#35368,#35369,#35370,#35371,#35372,#35373,#35374,#35375,#35376,#35377,#35378,
#35379,#35380,#35381,#35382,#35383,#35384,#35385,#35386,#35387,#35388,#35389,
#35390,#35391,#35392,#35393,#35394,#35395,#35396,#35397,#35398,#35399,#35400,
#35401,#35402,#35403,#35404,#35405,#35406,#35407,#35408,#35409,#35410,#35411,
#35412,#35413,#35414,#35415,#35416,#35417,#35418,#35419,#35420,#35421,#35422,
#35423,#35424,#35425,#35426,#35427,#35428,#35429,#35430,#35431,#35432,#35433,
#35434,#35435,#35436,#35437,#35438,#35439,#35440,#35441,#35442,#35443,#35444,
#35445,#35446,#35447,#35448,#35449,#35450,#35451,#35452,#35453,#35454,#35455,
#35456),(#35457,#35458,#35459,#35460,#35461,#35462,#35463,#35464,#35465,
#35466,#35467,#35468,#35469,#35470,#35471,#35472,#35473,#35474,#35475,#35476,
#35477,#35478,#35479,#35480,#35481,#35482,#35483,#35484,#35485,#35486,#35487,
#35488,#35489,#35490,#35491,#35492,#35493,#35494,#35495,#35496,#35497,#35498,
#35499,#35500,#35501,#35502,#35503,#35504,#35505,#35506,#35507,#35508,#35509,
#35510,#35511,#35512,#35513,#35514,#35515,#35516,#35517,#35518,#35519,#35520,
#35521,#35522,#35523,#35524,#35525,#35526,#35527,#35528,#35529,#35530,#35531,
#35532,#35533,#35534,#35535,#35536,#35537,#35538,#35539,#35540,#35541,#35542,
#35543,#35544,#35545,#35546,#35547,#35548,#35549,#35550,#35551,#35552,#35553,
#35554,#35555,#35556,#35557,#35558,#35559,#35560,#35561,#35562,#35563,#35564,
#35565,#35566,#35567,#35568,#35569,#35570,#35571,#35572,#35573,#35574,#35575,
#35576,#35577,#35578,#35579,#35580,#35581,#35582),(#35583,#35584,#35585,
#35586,#35587,#35588,#35589,#35590,#35591,#35592,#35593,#35594,#35595,#35596,
#35597,#35598,#35599,#35600,#35601,#35602,#35603,#35604,#35605,#35606,#35607,
#35608,#35609,#35610,#35611,#35612,#35613,#35614,#35615,#35616,#35617,#35618,
#35619,#35620,#35621,#35622,#35623,#35624,#35625,#35626,#35627,#35628,#35629,
#35630,#35631,#35632,#35633,#35634,#35635,#35636,#35637,#35638,#35639,#35640,
#35641,#35642,#35643,#35644,#35645,#35646,#35647,#35648,#35649,#35650,#35651,
#35652,#35653,#35654,#35655,#35656,#35657,#35658,#35659,#35660,#35661,#35662,
#35663,#35664,#35665,#35666,#35667,#35668,#35669,#35670,#35671,#35672,#35673,
#35674,#35675,#35676,#35677,#35678,#35679,#35680,#35681,#35682,#35683,#35684,
#35685,#35686,#35687,#35688,#35689,#35690,#35691,#35692,#35693,#35694,#35695,
#35696,#35697,#35698,#35699,#35700,#35701,#35702,#35703,#35704,#35705,#35706,
#35707,#35708),(#35709,#35710,#35711,#35712,#35713,#35714,#35715,#35716,
#35717,#35718,#35719,#35720,#35721,#35722,#35723,#35724,#35725,#35726,#35727,
#35728,#35729,#35730,#35731,#35732,#35733,#35734,#35735,#35736,#35737,#35738,
#35739,#35740,#35741,#35742,#35743,#35744,#35745,#35746,#35747,#35748,#35749,
#35750,#35751,#35752,#35753,#35754,#35755,#35756,#35757,#35758,#35759,#35760,
#35761,#35762,#35763,#35764,#35765,#35766,#35767,#35768,#35769,#35770,#35771,
#35772,#35773,#35774,#35775,#35776,#35777,#35778,#35779,#35780,#35781,#35782,
#35783,#35784,#35785,#35786,#35787,#35788,#35789,#35790,#35791,#35792,#35793,
#35794,#35795,#35796,#35797,#35798,#35799,#35800,#35801,#35802,#35803,#35804,
#35805,#35806,#35807,#35808,#35809,#35810,#35811,#35812,#35813,#35814,#35815,
#35816,#35817,#35818,#35819,#35820,#35821,#35822,#35823,#35824,#35825,#35826,
#35827,#35828,#35829,#35830,#35831,#35832,#35833,#35834)),.UNSPECIFIED.,
 .F.,.F.,.F.,(4,4),(4,1,1,1,1,1,1,1,1,1,1,1,1,1,1,1,1,1,1,1,1,1,1,1,1,1,
1,1,1,1,1,1,1,1,1,1,1,1,1,1,1,1,1,1,1,1,1,1,1,1,1,1,1,1,1,1,1,1,1,1,1,1,
1,1,1,1,1,1,1,1,1,1,1,1,1,1,1,1,1,1,1,1,1,1,1,1,1,1,1,1,1,1,1,1,1,1,1,1,
1,1,1,1,1,1,1,1,1,1,1,1,1,1,1,1,1,1,1,1,1,1,1,1,1,4),(-0.000406578931768313,
0.050511877590733),(8.33359626324588,9.33277702554168,10.3319577878375,
11.3311385501333,12.3303193124291,13.3295000747249,14.3286808370206,15.3278615993164,
16.3270423616122,17.326223123908,18.3254038862038,19.3245846484996,20.3237654107954,
21.3229461730912,22.322126935387,23.3213076976828,24.3204884599786,25.3196692222744,
26.3188499845702,27.318030746866,28.3172115091618,29.3163922714576,30.3155730337533,
31.3147537960491,32.3139345583449,33.3131153206407,34.3122960829365,35.3114768452323,
36.3106576075281,37.3098383698239,38.3090191321197,39.3081998944155,40.3073806567113,
41.3065614190071,42.3057421813029,43.3049229435987,44.3041037058945,45.3032844681902,
46.302465230486,47.3016459927818,48.3008267550776,49.3000075173734,50.2991882796692,
51.298369041965,52.2975498042608,53.2967305665566,54.2959113288524,55.2950920911482,
56.294272853444,57.2934536157398,58.2926343780356,59.2918151403314,60.2909959026272,
61.290176664923,62.2893574272187,63.2885381895145,64.2877189518103,65.2868997141061,
66.2860804764019,67.2852612386977,68.2844420009935,69.2836227632893,70.2828035255851,
71.2819842878809,72.2811650501767,73.2803458124725,74.2795265747683,75.2787073370641,
76.2778880993599,77.2770688616556,78.2762496239514,79.2754303862472,80.274611148543,
81.2737919108388,82.2729726731346,83.2721534354304,84.2713341977262,85.270514960022,
86.2696957223178,87.2688764846136,88.2680572469094,89.2672380092052,90.266418771501,
91.2655995337968,92.2647802960926,93.2639610583883,94.2631418206841,95.2623225829799,
96.2615033452757,97.2606841075715,98.2598648698673,99.2590456321631,100.258226394459,
101.257407156755,102.25658791905,103.255768681346,104.254949443642,105.254130205938,
106.253310968234,107.252491730529,108.251672492825,109.250853255121,110.250034017417,
111.249214779713,112.248395542008,113.247576304304,114.2467570666,115.245937828896,
116.245118591192,117.244299353487,118.243480115783,119.242660878079,120.241841640375,
121.241022402671,122.240203164966,123.239383927262,124.238564689558,125.237745451854,
126.23692621415,127.236106976445,128.235287738741,129.234468501037,130.233649263333,
131.233236604561),.UNSPECIFIED.);
#1007=B_SPLINE_SURFACE_WITH_KNOTS('',3,3,((#36002,#36003,#36004,#36005,
#36006,#36007,#36008,#36009,#36010,#36011,#36012,#36013,#36014,#36015,#36016,
#36017,#36018,#36019,#36020,#36021,#36022,#36023,#36024,#36025,#36026,#36027,
#36028,#36029,#36030,#36031,#36032,#36033,#36034,#36035,#36036,#36037,#36038,
#36039,#36040,#36041,#36042,#36043,#36044,#36045,#36046,#36047,#36048,#36049,
#36050,#36051,#36052,#36053,#36054,#36055,#36056,#36057,#36058,#36059,#36060,
#36061,#36062,#36063,#36064,#36065,#36066,#36067,#36068,#36069,#36070,#36071,
#36072,#36073,#36074,#36075,#36076,#36077,#36078,#36079,#36080,#36081,#36082,
#36083,#36084,#36085,#36086,#36087,#36088,#36089,#36090,#36091,#36092,#36093,
#36094,#36095,#36096,#36097,#36098,#36099,#36100,#36101,#36102,#36103,#36104,
#36105,#36106,#36107,#36108,#36109,#36110,#36111,#36112,#36113,#36114,#36115,
#36116,#36117,#36118,#36119,#36120,#36121,#36122,#36123,#36124,#36125,#36126,
#36127),(#36128,#36129,#36130,#36131,#36132,#36133,#36134,#36135,#36136,
#36137,#36138,#36139,#36140,#36141,#36142,#36143,#36144,#36145,#36146,#36147,
#36148,#36149,#36150,#36151,#36152,#36153,#36154,#36155,#36156,#36157,#36158,
#36159,#36160,#36161,#36162,#36163,#36164,#36165,#36166,#36167,#36168,#36169,
#36170,#36171,#36172,#36173,#36174,#36175,#36176,#36177,#36178,#36179,#36180,
#36181,#36182,#36183,#36184,#36185,#36186,#36187,#36188,#36189,#36190,#36191,
#36192,#36193,#36194,#36195,#36196,#36197,#36198,#36199,#36200,#36201,#36202,
#36203,#36204,#36205,#36206,#36207,#36208,#36209,#36210,#36211,#36212,#36213,
#36214,#36215,#36216,#36217,#36218,#36219,#36220,#36221,#36222,#36223,#36224,
#36225,#36226,#36227,#36228,#36229,#36230,#36231,#36232,#36233,#36234,#36235,
#36236,#36237,#36238,#36239,#36240,#36241,#36242,#36243,#36244,#36245,#36246,
#36247,#36248,#36249,#36250,#36251,#36252,#36253),(#36254,#36255,#36256,
#36257,#36258,#36259,#36260,#36261,#36262,#36263,#36264,#36265,#36266,#36267,
#36268,#36269,#36270,#36271,#36272,#36273,#36274,#36275,#36276,#36277,#36278,
#36279,#36280,#36281,#36282,#36283,#36284,#36285,#36286,#36287,#36288,#36289,
#36290,#36291,#36292,#36293,#36294,#36295,#36296,#36297,#36298,#36299,#36300,
#36301,#36302,#36303,#36304,#36305,#36306,#36307,#36308,#36309,#36310,#36311,
#36312,#36313,#36314,#36315,#36316,#36317,#36318,#36319,#36320,#36321,#36322,
#36323,#36324,#36325,#36326,#36327,#36328,#36329,#36330,#36331,#36332,#36333,
#36334,#36335,#36336,#36337,#36338,#36339,#36340,#36341,#36342,#36343,#36344,
#36345,#36346,#36347,#36348,#36349,#36350,#36351,#36352,#36353,#36354,#36355,
#36356,#36357,#36358,#36359,#36360,#36361,#36362,#36363,#36364,#36365,#36366,
#36367,#36368,#36369,#36370,#36371,#36372,#36373,#36374,#36375,#36376,#36377,
#36378,#36379),(#36380,#36381,#36382,#36383,#36384,#36385,#36386,#36387,
#36388,#36389,#36390,#36391,#36392,#36393,#36394,#36395,#36396,#36397,#36398,
#36399,#36400,#36401,#36402,#36403,#36404,#36405,#36406,#36407,#36408,#36409,
#36410,#36411,#36412,#36413,#36414,#36415,#36416,#36417,#36418,#36419,#36420,
#36421,#36422,#36423,#36424,#36425,#36426,#36427,#36428,#36429,#36430,#36431,
#36432,#36433,#36434,#36435,#36436,#36437,#36438,#36439,#36440,#36441,#36442,
#36443,#36444,#36445,#36446,#36447,#36448,#36449,#36450,#36451,#36452,#36453,
#36454,#36455,#36456,#36457,#36458,#36459,#36460,#36461,#36462,#36463,#36464,
#36465,#36466,#36467,#36468,#36469,#36470,#36471,#36472,#36473,#36474,#36475,
#36476,#36477,#36478,#36479,#36480,#36481,#36482,#36483,#36484,#36485,#36486,
#36487,#36488,#36489,#36490,#36491,#36492,#36493,#36494,#36495,#36496,#36497,
#36498,#36499,#36500,#36501,#36502,#36503,#36504,#36505)),.UNSPECIFIED.,
 .F.,.F.,.F.,(4,4),(4,1,1,1,1,1,1,1,1,1,1,1,1,1,1,1,1,1,1,1,1,1,1,1,1,1,
1,1,1,1,1,1,1,1,1,1,1,1,1,1,1,1,1,1,1,1,1,1,1,1,1,1,1,1,1,1,1,1,1,1,1,1,
1,1,1,1,1,1,1,1,1,1,1,1,1,1,1,1,1,1,1,1,1,1,1,1,1,1,1,1,1,1,1,1,1,1,1,1,
1,1,1,1,1,1,1,1,1,1,1,1,1,1,1,1,1,1,1,1,1,1,1,1,1,4),(-0.000343459060642306,
0.0505598735282669),(11.6721236773201,12.6717110499602,13.670891812256,
14.6700725745517,15.6692533368475,16.6684340991433,17.6676148614391,18.6667956237349,
19.6659763860307,20.6651571483265,21.6643379106223,22.6635186729181,23.6626994352139,
24.6618801975097,25.6610609598055,26.6602417221013,27.6594224843971,28.6586032466929,
29.6577840089887,30.6569647712845,31.6561455335802,32.655326295876,33.6545070581718,
34.6536878204676,35.6528685827634,36.6520493450592,37.651230107355,38.6504108696508,
39.6495916319466,40.6487723942424,41.6479531565382,42.647133918834,43.6463146811298,
44.6454954434256,45.6446762057214,46.6438569680172,47.643037730313,48.6422184926087,
49.6413992549045,50.6405800172003,51.6397607794961,52.6389415417919,53.6381223040877,
54.6373030663835,55.6364838286793,56.6356645909751,57.6348453532709,58.6340261155667,
59.6332068778625,60.6323876401583,61.6315684024541,62.6307491647499,63.6299299270457,
64.6291106893415,65.6282914516373,66.627472213933,67.6266529762288,68.6258337385246,
69.6250145008204,70.6241952631162,71.623376025412,72.6225567877078,73.6217375500036,
74.6209183122994,75.6200990745952,76.619279836891,77.6184605991868,78.6176413614826,
79.6168221237784,80.6160028860742,81.6151836483699,82.6143644106657,83.6135451729615,
84.6127259352573,85.6119066975531,86.6110874598489,87.6102682221447,88.6094489844405,
89.6086297467363,90.6078105090321,91.6069912713279,92.6061720336237,93.6053527959195,
94.6045335582153,95.6037143205111,96.6028950828069,97.6020758451027,98.6012566073985,
99.6004373696942,100.59961813199,101.598798894286,102.597979656582,103.597160418877,
104.596341181173,105.595521943469,106.594702705765,107.593883468061,108.593064230356,
109.592244992652,110.591425754948,111.590606517244,112.58978727954,113.588968041835,
114.588148804131,115.587329566427,116.586510328723,117.585691091019,118.584871853314,
119.58405261561,120.583233377906,121.582414140202,122.581594902498,123.580775664793,
124.579956427089,125.579137189385,126.578317951681,127.577498713976,128.576679476272,
129.575860238568,130.575041000864,131.57422176316,132.573402525455,133.572583287751,
134.571764050047),.UNSPECIFIED.);
#1020=SHAPE_REPRESENTATION_RELATIONSHIP('SRR','None',#72024,#1030);
#1030=ADVANCED_BREP_SHAPE_REPRESENTATION('',(#1050),#71792);
#1040=STYLED_ITEM('',(#72083),#1050);
#1050=MANIFOLD_SOLID_BREP('Body1',#13642);
#1094=CONICAL_SURFACE('',#14151,2.16347,0.785398163397448);
#1095=CONICAL_SURFACE('',#14158,3.7624,0.785398163397448);
#1096=CONICAL_SURFACE('',#14351,2.29135888084632,1.02974425867665);
#1141=B_SPLINE_CURVE_WITH_KNOTS('',3,(#19897,#19898,#19899,#19900,#19901,
#19902,#19903,#19904,#19905,#19906,#19907,#19908,#19909,#19910,#19911,#19912,
#19913,#19914,#19915,#19916,#19917,#19918,#19919,#19920,#19921,#19922,#19923,
#19924,#19925,#19926,#19927,#19928,#19929,#19930,#19931,#19932,#19933,#19934,
#19935,#19936,#19937,#19938,#19939,#19940,#19941,#19942,#19943,#19944,#19945,
#19946,#19947,#19948,#19949,#19950,#19951,#19952,#19953,#19954,#19955,#19956,
#19957,#19958,#19959,#19960,#19961,#19962,#19963,#19964,#19965,#19966,#19967,
#19968,#19969,#19970,#19971,#19972,#19973,#19974,#19975,#19976,#19977,#19978,
#19979,#19980,#19981,#19982,#19983,#19984,#19985,#19986,#19987,#19988,#19989,
#19990,#19991,#19992,#19993,#19994,#19995,#19996,#19997,#19998,#19999,#20000,
#20001,#20002,#20003,#20004,#20005,#20006,#20007,#20008,#20009,#20010,#20011,
#20012,#20013,#20014,#20015,#20016,#20017,#20018,#20019,#20020,#20021,#20022,
#20023,#20024,#20025,#20026),.UNSPECIFIED.,.F.,.F.,(4,3,3,3,3,3,3,3,3,3,
3,3,3,3,3,3,3,3,3,3,3,3,3,3,3,3,3,3,3,3,3,3,3,3,3,3,3,3,3,3,3,3,3,4),(10.3186182874638,
10.3319577878375,10.4378652798471,10.5436115957539,10.6492313119882,10.754783484694,
10.8603044745869,10.9658305963425,11.0714672342109,11.1771663451116,11.2830457101334,
11.3311385501333,11.4371331467285,11.5429710322994,11.648688489881,11.7543421829616,
11.8599683212614,11.9656030723555,12.071352874328,12.1771679068059,12.2831662388787,
12.3303193124291,12.4360258213461,12.5415702665319,12.6469878201331,12.7523377706301,
12.8576567942629,12.9629815213307,13.0684190300506,13.1739200138675,13.2796048951218,
13.3295000747249,13.4353384967336,13.5410165329372,13.6465695041155,13.7520559304393,
13.8575122821743,13.9629749846754,14.0685505048566,14.1741897271739,14.2800117420941,
14.3286808370206,14.4345182698765,14.4571413871433),.UNSPECIFIED.);
#1142=B_SPLINE_CURVE_WITH_KNOTS('',3,(#20029,#20030,#20031,#20032,#20033,
#20034,#20035,#20036,#20037,#20038,#20039,#20040,#20041,#20042,#20043,#20044,
#20045,#20046,#20047,#20048,#20049,#20050,#20051,#20052,#20053,#20054,#20055,
#20056,#20057,#20058,#20059,#20060,#20061,#20062,#20063,#20064,#20065,#20066,
#20067,#20068,#20069,#20070,#20071,#20072,#20073,#20074,#20075,#20076,#20077,
#20078,#20079,#20080,#20081,#20082,#20083,#20084,#20085,#20086,#20087,#20088,
#20089,#20090,#20091,#20092,#20093,#20094,#20095,#20096,#20097,#20098,#20099,
#20100,#20101,#20102,#20103,#20104,#20105,#20106,#20107,#20108,#20109,#20110,
#20111,#20112,#20113),.UNSPECIFIED.,.F.,.F.,(4,3,3,3,3,3,3,3,3,3,3,3,3,
3,3,3,3,3,3,3,3,3,3,3,3,3,3,3,4),(11.6725302876644,11.7807318723834,11.8921042695805,
12.0002215149502,12.1083396087937,12.2164883956815,12.3302940592512,12.4386767884211,
12.5471600419772,12.6558426310807,12.6717110499602,12.7765953511984,12.8813042105095,
12.9858701824119,13.0903589546267,13.1948083587627,13.2992561685555,13.4038114660646,
13.5084257386862,13.6132263099785,13.670891812256,13.776767494232,13.8824961979185,
13.988114518063,14.0936589161058,14.1991952494382,14.3047263271779,14.4103355213707,
14.4560074704634),.UNSPECIFIED.);
#1143=B_SPLINE_CURVE_WITH_KNOTS('',3,(#20119,#20120,#20121,#20122,#20123,
#20124,#20125,#20126,#20127,#20128,#20129,#20130,#20131,#20132,#20133,#20134,
#20135,#20136,#20137,#20138,#20139,#20140,#20141,#20142,#20143,#20144,#20145,
#20146,#20147,#20148,#20149,#20150,#20151,#20152,#20153,#20154,#20155,#20156,
#20157,#20158,#20159,#20160,#20161,#20162,#20163,#20164,#20165,#20166,#20167,
#20168,#20169,#20170,#20171,#20172,#20173,#20174,#20175,#20176,#20177,#20178,
#20179,#20180,#20181,#20182,#20183,#20184,#20185,#20186,#20187,#20188,#20189,
#20190,#20191,#20192,#20193,#20194,#20195,#20196,#20197,#20198,#20199,#20200,
#20201,#20202,#20203,#20204,#20205,#20206,#20207,#20208,#20209,#20210,#20211,
#20212,#20213,#20214,#20215,#20216,#20217,#20218,#20219,#20220,#20221,#20222,
#20223,#20224,#20225,#20226,#20227,#20228,#20229,#20230,#20231,#20232,#20233,
#20234,#20235,#20236,#20237,#20238,#20239,#20240,#20241,#20242,#20243,#20244,
#20245,#20246,#20247,#20248,#20249,#20250,#20251,#20252,#20253,#20254,#20255,
#20256,#20257,#20258,#20259,#20260,#20261,#20262,#20263,#20264,#20265,#20266,
#20267,#20268,#20269,#20270,#20271,#20272,#20273,#20274,#20275,#20276,#20277,
#20278,#20279,#20280,#20281,#20282,#20283,#20284,#20285,#20286,#20287,#20288,
#20289,#20290,#20291,#20292),.UNSPECIFIED.,.F.,.F.,(4,2,2,2,2,2,2,2,2,2,
2,2,2,2,2,2,2,2,2,2,2,2,2,2,2,2,2,2,2,2,2,2,2,2,2,2,2,2,2,2,2,2,2,2,2,2,
2,2,2,2,2,2,2,2,2,2,2,2,2,2,2,2,2,2,2,2,2,2,2,2,2,2,2,2,2,2,2,2,2,2,2,2,
2,2,2,2,4),(-0.973925068013576,-0.950916583618217,-0.905493200642175,-0.897753475521733,
-0.895184606050773,-0.893569427576055,-0.892024446877122,-0.889786345933224,
-0.883889448500355,-0.874927077808174,-0.842219678413613,-0.80692732268821,
-0.801784811841754,-0.798469610807626,-0.795803022878436,-0.792756597718315,
-0.787481654381162,-0.762329534815237,-0.729121193154261,-0.706165152782175,
-0.703027155427136,-0.701098928412001,-0.699600423889519,-0.697838800859491,
-0.694600828591246,-0.675779806694615,-0.637626900347504,-0.613177506659964,
-0.607819097580816,-0.60472347344611,-0.602061397413686,-0.598812124107507,
-0.592573771645881,-0.584649060931421,-0.566096074873262,-0.551753034556585,
-0.5150749684563,-0.510296877551879,-0.508385065260786,-0.506986508852542,
-0.505420267177212,-0.503076841056701,-0.496430331527037,-0.485859790756768,
-0.457667412673531,-0.420400942771593,-0.415279877300816,-0.411971173955281,
-0.409305076770745,-0.406254041491245,-0.400957798416744,-0.375375298975841,
-0.340102743761475,-0.31963218995123,-0.316521775388175,-0.314601626586024,
-0.31310330189229,-0.311334476348705,-0.30806554049338,-0.28842640564689,
-0.249316487113877,-0.226588624374065,-0.221307279244302,-0.218228385153227,
-0.21561712082627,-0.212448536261234,-0.209019416422941,-0.203577302512313,
-0.192881957982826,-0.14201590139986,-0.126040406731366,-0.122827049071309,
-0.121050717977937,-0.119554140856589,-0.11764657635809,-0.1136902832442,
-0.108401372273103,-0.0949827972572126,-0.0528096305379754,-0.0343385982899319,
-0.0289664209109278,-0.0255832861349313,-0.0229122525890893,-0.0204127395629368,
-0.0174678607068047,-0.010814646247928,-0.000575867290469521),
 .UNSPECIFIED.);
#1144=B_SPLINE_CURVE_WITH_KNOTS('',3,(#20293,#20294,#20295,#20296,#20297,
#20298,#20299,#20300,#20301,#20302,#20303,#20304,#20305,#20306,#20307,#20308,
#20309,#20310,#20311,#20312,#20313,#20314,#20315,#20316,#20317,#20318,#20319,
#20320,#20321,#20322,#20323,#20324,#20325,#20326,#20327,#20328,#20329,#20330,
#20331,#20332),.UNSPECIFIED.,.F.,.F.,(4,3,3,3,3,3,3,3,3,3,3,3,3,4),(14.4571413871433,
14.5659814136649,14.6715168831504,14.7769950977482,14.8824525106465,14.9879255397584,
15.0935173624096,15.1991811965176,15.3050207279912,15.3278615993164,15.4471321116664,
15.5659385083076,15.6839855814566,15.7079632675659),.UNSPECIFIED.);
#1145=B_SPLINE_CURVE_WITH_KNOTS('',3,(#20334,#20335,#20336,#20337,#20338,
#20339,#20340,#20341,#20342,#20343,#20344,#20345,#20346,#20347,#20348,#20349,
#20350,#20351,#20352,#20353,#20354,#20355,#20356,#20357,#20358,#20359,#20360,
#20361,#20362,#20363,#20364,#20365,#20366,#20367,#20368,#20369,#20370,#20371,
#20372,#20373),.UNSPECIFIED.,.F.,.F.,(4,3,3,3,3,3,3,3,3,3,3,3,3,4),(14.4560074704634,
14.5630400225075,14.6700725745517,14.776067128075,14.8819049692828,14.9876223807981,
15.0932760267801,15.1989021170178,15.3045368191538,15.410286571138,15.516101552966,
15.6220998338911,15.6692533368475,15.7079632679489),.UNSPECIFIED.);
#1146=B_SPLINE_CURVE_WITH_KNOTS('',3,(#20374,#20375,#20376,#20377,#20378,
#20379,#20380,#20381,#20382,#20383,#20384,#20385,#20386,#20387,#20388,#20389,
#20390,#20391,#20392,#20393,#20394,#20395,#20396,#20397,#20398,#20399,#20400,
#20401,#20402,#20403,#20404,#20405,#20406,#20407,#20408,#20409,#20410,#20411,
#20412,#20413,#20414,#20415,#20416,#20417,#20418,#20419,#20420,#20421,#20422,
#20423,#20424,#20425,#20426,#20427,#20428,#20429,#20430,#20431,#20432,#20433,
#20434,#20435,#20436,#20437,#20438,#20439,#20440,#20441,#20442,#20443,#20444,
#20445,#20446,#20447,#20448,#20449,#20450,#20451,#20452,#20453,#20454,#20455,
#20456,#20457,#20458,#20459,#20460,#20461,#20462,#20463,#20464,#20465,#20466,
#20467,#20468,#20469,#20470,#20471,#20472,#20473,#20474,#20475,#20476,#20477,
#20478,#20479,#20480,#20481,#20482,#20483,#20484,#20485,#20486,#20487,#20488,
#20489,#20490,#20491,#20492,#20493,#20494,#20495,#20496,#20497,#20498,#20499,
#20500,#20501,#20502,#20503,#20504,#20505,#20506,#20507,#20508,#20509,#20510,
#20511,#20512,#20513,#20514,#20515,#20516,#20517,#20518,#20519,#20520,#20521,
#20522,#20523,#20524,#20525,#20526,#20527,#20528,#20529,#20530,#20531,#20532,
#20533,#20534,#20535,#20536,#20537,#20538,#20539),.UNSPECIFIED.,.F.,.F.,
(4,2,2,2,2,2,2,2,2,2,2,2,2,2,2,2,2,2,2,2,2,2,2,2,2,2,2,2,2,2,2,2,2,2,2,
2,2,2,2,2,2,2,2,2,2,2,2,2,2,2,2,2,2,2,2,2,2,2,2,2,2,2,2,2,2,2,2,2,2,2,2,
2,2,2,2,2,2,2,2,2,2,2,4),(-2.43116705121226,-2.41825989892644,-2.36647369053139,
-2.35025992321336,-2.34562825164978,-2.34273454470215,-2.34005815576854,
-2.33658646075185,-2.32921645052342,-2.28534566527498,-2.26134546291887,
-2.25375569118682,-2.25017789072549,-2.24805388258681,-2.24618226274905,
-2.24472486204046,-2.24301186541103,-2.24007475283859,-2.22836745627527,
-2.19337697260899,-2.15973673741926,-2.15336811601201,-2.15008944227208,
-2.1474220276589,-2.14434108462187,-2.13905971325778,-2.11612030814376,
-2.07729067609646,-2.05778653059882,-2.05451766121803,-2.05274638104333,
-2.05124590055494,-2.04932184647869,-2.04620004885552,-2.02420982710104,
-1.99028567529971,-1.96496510718384,-1.95968227813066,-1.95663415458968,
-1.95396775101269,-1.950654953851,-1.94552035833235,-1.91184399138432,-1.86899400398118,
-1.86267256093303,-1.86037399166691,-1.85881744581162,-1.85741247817496,
-1.85547181027022,-1.85051634624008,-1.81953336583791,-1.78728838944621,
-1.77055887209857,-1.76586406254956,-1.76294628005505,-1.76025770014692,
-1.7567840625937,-1.74918084795132,-1.70851212927825,-1.68626113499655,
-1.67598639338314,-1.66947598569715,-1.66715266223597,-1.6655918973548,
-1.66419090788137,-1.66226812624139,-1.65742240240225,-1.6225527739334,
-1.58006393991122,-1.57380637167895,-1.5705532897928,-1.56789115924466,
-1.56479892619132,-1.55945504565141,-1.53530213154841,-1.49693977941724,
-1.47801749424984,-1.47477535942088,-1.47301270248496,-1.47151445989363,
-1.46958783402063,-1.46645427813501,-1.45799448822835),.UNSPECIFIED.);
#1147=B_SPLINE_CURVE_WITH_KNOTS('',3,(#20544,#20545,#20546,#20547,#20548,
#20549,#20550,#20551,#20552,#20553,#20554,#20555,#20556,#20557,#20558,#20559,
#20560,#20561,#20562,#20563,#20564,#20565,#20566,#20567,#20568,#20569,#20570,
#20571,#20572,#20573,#20574,#20575,#20576,#20577,#20578,#20579,#20580,#20581,
#20582,#20583,#20584,#20585,#20586,#20587,#20588,#20589,#20590,#20591,#20592,
#20593,#20594,#20595,#20596,#20597,#20598,#20599,#20600,#20601,#20602,#20603,
#20604,#20605,#20606,#20607,#20608,#20609,#20610,#20611,#20612,#20613,#20614,
#20615,#20616,#20617,#20618,#20619,#20620,#20621,#20622,#20623,#20624,#20625,
#20626,#20627,#20628,#20629,#20630,#20631,#20632,#20633,#20634,#20635,#20636,
#20637,#20638,#20639,#20640,#20641,#20642,#20643,#20644,#20645,#20646,#20647,
#20648,#20649,#20650,#20651,#20652,#20653,#20654,#20655,#20656,#20657,#20658,
#20659,#20660,#20661,#20662,#20663,#20664,#20665,#20666,#20667,#20668,#20669,
#20670,#20671,#20672,#20673,#20674,#20675,#20676,#20677,#20678,#20679,#20680,
#20681,#20682,#20683,#20684,#20685,#20686,#20687,#20688,#20689,#20690,#20691,
#20692,#20693,#20694,#20695,#20696,#20697,#20698,#20699,#20700,#20701,#20702,
#20703,#20704,#20705,#20706,#20707,#20708,#20709,#20710,#20711,#20712,#20713,
#20714,#20715,#20716,#20717,#20718,#20719,#20720,#20721,#20722,#20723,#20724,
#20725,#20726,#20727,#20728,#20729,#20730,#20731,#20732,#20733,#20734,#20735,
#20736,#20737,#20738,#20739,#20740,#20741,#20742,#20743,#20744,#20745,#20746,
#20747,#20748,#20749,#20750,#20751,#20752,#20753,#20754,#20755),
 .UNSPECIFIED.,.F.,.F.,(4,2,2,2,2,2,2,2,2,2,2,2,2,2,2,2,2,2,2,2,2,2,2,2,
2,2,2,2,2,2,2,2,2,2,2,2,2,2,2,2,2,2,2,2,2,2,2,2,2,2,2,2,2,2,2,2,2,2,2,2,
2,2,2,2,2,2,2,2,2,2,2,2,2,2,2,2,2,2,2,2,2,2,2,2,2,2,2,2,2,2,2,2,2,2,2,2,
2,2,2,2,2,2,2,2,2,4),(-2.18888770495768,-2.17440356240776,-2.15760483198674,
-2.1529013703585,-2.14998009510879,-2.14728951265677,-2.14381493702274,
-2.13621610742933,-2.09547509211733,-2.08172747531193,-2.06051870295789,
-2.05587459133256,-2.05383918232385,-2.05232911905959,-2.05063398069282,
-2.04770158677108,-2.0364564406292,-2.02570297855795,-1.99101537655758,
-1.96553909356269,-1.96024970328795,-1.95720084609208,-1.95453560810125,
-1.95122661499686,-1.94610243463115,-1.91309432495797,-1.86966794363949,
-1.86331604464308,-1.86101313797446,-1.85945555499966,-1.85805021627004,
-1.85611079474346,-1.85116696751013,-1.81977810110936,-1.78894211509328,
-1.77135846820353,-1.76658613284954,-1.76364971124354,-1.76096342398723,
-1.7575197220415,-1.7500913400709,-1.70589220198532,-1.69656608180767,-1.67987754901806,
-1.67079125353471,-1.66816622499803,-1.6665388969697,-1.66501942250558,
-1.6631765141586,-1.65847420477853,-1.61886094922967,-1.58088410189835,
-1.5745581483308,-1.57129132783081,-1.56862868744837,-1.56554790676729,
-1.56025389159061,-1.53702866601674,-1.49803501717298,-1.47872439493125,
-1.47546846403827,-1.4737031323747,-1.47220530171545,-1.47028282855015,
-1.46716349806044,-1.4452196385958,-1.41123484784928,-1.38589295777027,
-1.38060969252384,-1.37756191815101,-1.3748961844373,-1.37158469865851,
-1.36645303480537,-1.33285651672871,-1.28998301756724,-1.28366083261001,
-1.28136189386708,-1.27980499096779,-1.27839870469658,-1.27645596614525,
-1.27149344249406,-1.24188020293477,-1.21605565644257,-1.19280633788884,
-1.18751077798279,-1.18442944257999,-1.18176652851354,-1.17849963399397,
-1.17217440644923,-1.13470962514543,-1.09445035578459,-1.08980226055688,
-1.0879677578334,-1.0864501846656,-1.08481853441266,-1.08217467602329,-1.07289968352053,
-1.05567579519044,-1.01718049724718,-0.998927396005311,-0.993911819765243,
-0.990921987579742,-0.988247505054198,-0.984844934284836,-0.977833746534452,
-0.973925068013576),.UNSPECIFIED.);
#1148=B_SPLINE_CURVE_WITH_KNOTS('',3,(#20756,#20757,#20758,#20759,#20760,
#20761,#20762,#20763,#20764,#20765,#20766,#20767,#20768,#20769,#20770,#20771,
#20772,#20773,#20774,#20775,#20776,#20777,#20778,#20779,#20780,#20781,#20782,
#20783,#20784,#20785,#20786,#20787,#20788,#20789,#20790,#20791,#20792,#20793,
#20794,#20795,#20796,#20797,#20798,#20799,#20800,#20801,#20802,#20803,#20804,
#20805,#20806,#20807,#20808,#20809,#20810,#20811,#20812,#20813,#20814,#20815,
#20816,#20817,#20818,#20819,#20820,#20821,#20822,#20823,#20824,#20825,#20826,
#20827,#20828,#20829,#20830,#20831,#20832,#20833,#20834,#20835,#20836,#20837,
#20838,#20839,#20840,#20841,#20842,#20843,#20844,#20845,#20846,#20847,#20848,
#20849,#20850,#20851,#20852,#20853,#20854,#20855,#20856,#20857,#20858,#20859,
#20860,#20861,#20862,#20863,#20864,#20865,#20866,#20867,#20868,#20869,#20870,
#20871,#20872,#20873,#20874,#20875,#20876,#20877,#20878,#20879,#20880,#20881,
#20882,#20883,#20884,#20885,#20886,#20887,#20888,#20889,#20890,#20891,#20892,
#20893,#20894,#20895,#20896,#20897,#20898,#20899,#20900,#20901,#20902,#20903,
#20904,#20905,#20906,#20907,#20908,#20909,#20910,#20911,#20912,#20913,#20914,
#20915,#20916,#20917,#20918,#20919,#20920,#20921,#20922,#20923,#20924,#20925,
#20926,#20927,#20928,#20929,#20930,#20931,#20932,#20933,#20934,#20935,#20936,
#20937,#20938,#20939,#20940,#20941,#20942,#20943,#20944,#20945,#20946,#20947,
#20948,#20949,#20950,#20951,#20952,#20953,#20954,#20955,#20956,#20957,#20958,
#20959,#20960,#20961),.UNSPECIFIED.,.F.,.F.,(4,2,2,2,2,2,2,2,2,2,2,2,2,
2,2,2,2,2,2,2,2,2,2,2,2,2,2,2,2,2,2,2,2,2,2,2,2,2,2,2,2,2,2,2,2,2,2,2,2,
2,2,2,2,2,2,2,2,2,2,2,2,2,2,2,2,2,2,2,2,2,2,2,2,2,2,2,2,2,2,2,2,2,2,2,2,
2,2,2,2,2,2,2,2,2,2,2,2,2,2,2,2,2,4),(-1.45799448822835,-1.44369859826014,
-1.4103702764355,-1.38519006403529,-1.37991539342407,-1.37686979111578,
-1.37420432427642,-1.3708910545462,-1.36575257505012,-1.33176520332503,
-1.28925062247887,-1.28294848488126,-1.28065265946425,-1.27909664593552,
-1.27769028630853,-1.27574629181798,-1.27077456819685,-1.24130627610694,
-1.21615198256352,-1.19216297183634,-1.18682834779486,-1.18373868908013,
-1.18107715015986,-1.17782276776665,-1.17155637777987,-1.16358575126856,
-1.14486736881379,-1.10345826147743,-1.09115577642696,-1.08816812951347,
-1.08644352677372,-1.08509088844199,-1.08319300473201,-1.07928921225045,
-1.07409112914766,-1.06102008615378,-1.02199955019933,-0.998833693039655,
-0.993542999963677,-0.990462962085075,-0.987800262057036,-0.984532488581164,
-0.978201929049717,-0.939568411565091,-0.900633052680451,-0.895984261951173,
-0.894094773852571,-0.892563380156228,-0.890956019443983,-0.888421611277405,
-0.880200064816503,-0.865852473554847,-0.820750747330644,-0.804551168049324,
-0.799732117706123,-0.796785522238933,-0.794102054317322,-0.790620900147062,
-0.783191943218217,-0.752879198212985,-0.720642340681662,-0.704999505049405,
-0.701804168829464,-0.700032332432719,-0.698535243023055,-0.696621783418443,
-0.692637997230728,-0.68730214706372,-0.673704755880074,-0.633403907149467,
-0.612091287965335,-0.606915906687448,-0.603862129269355,-0.601197261180934,
-0.597894796916618,-0.591391778369867,-0.549596001194279,-0.514371565420689,
-0.509535194772166,-0.507613675795986,-0.506212827380192,-0.50464994023431,
-0.502321648549891,-0.495785540703312,-0.485458474152035,-0.462989283529869,
-0.422705340890909,-0.415090161046028,-0.411612385036776,-0.408921076312092,
-0.406000773055517,-0.401302808986865,-0.384570986613379,-0.352330476805928,
-0.321288902334277,-0.316331596124056,-0.314389778305016,-0.312983762683364,
-0.311426717947963,-0.309126829181139,-0.302797269005275,-0.259790057080148,
-0.242722284356607),.UNSPECIFIED.);
#1149=B_SPLINE_CURVE_WITH_KNOTS('',3,(#20967,#20968,#20969,#20970,#20971,
#20972,#20973,#20974,#20975,#20976,#20977,#20978,#20979,#20980,#20981,#20982,
#20983,#20984,#20985,#20986,#20987,#20988,#20989,#20990,#20991,#20992,#20993,
#20994,#20995,#20996,#20997,#20998,#20999,#21000,#21001,#21002,#21003,#21004,
#21005,#21006,#21007,#21008,#21009,#21010,#21011,#21012,#21013,#21014,#21015,
#21016,#21017,#21018,#21019,#21020,#21021,#21022,#21023,#21024,#21025,#21026,
#21027,#21028,#21029,#21030,#21031,#21032,#21033,#21034,#21035,#21036,#21037,
#21038,#21039,#21040,#21041,#21042,#21043,#21044,#21045,#21046,#21047,#21048,
#21049,#21050,#21051,#21052,#21053,#21054,#21055,#21056,#21057,#21058,#21059,
#21060,#21061,#21062,#21063,#21064,#21065,#21066,#21067,#21068,#21069,#21070,
#21071,#21072,#21073,#21074,#21075,#21076,#21077,#21078,#21079,#21080,#21081,
#21082,#21083,#21084,#21085,#21086,#21087,#21088,#21089,#21090,#21091,#21092,
#21093,#21094,#21095,#21096,#21097,#21098,#21099,#21100,#21101,#21102,#21103,
#21104,#21105,#21106,#21107,#21108,#21109,#21110,#21111,#21112,#21113,#21114,
#21115,#21116,#21117,#21118,#21119,#21120,#21121,#21122,#21123,#21124,#21125,
#21126,#21127,#21128,#21129,#21130,#21131,#21132,#21133,#21134,#21135,#21136,
#21137,#21138,#21139,#21140),.UNSPECIFIED.,.F.,.F.,(4,2,2,2,2,2,2,2,2,2,
2,2,2,2,2,2,2,2,2,2,2,2,2,2,2,2,2,2,2,2,2,2,2,2,2,2,2,2,2,2,2,2,2,2,2,2,
2,2,2,2,2,2,2,2,2,2,2,2,2,2,2,2,2,2,2,2,2,2,2,2,2,2,2,2,2,2,2,2,2,2,2,2,
2,2,2,2,4),(-0.97373548788866,-0.973604728194627,-0.971304204815467,-0.964972036506884,
-0.921921862329116,-0.888535807356521,-0.883406613516542,-0.880095551096803,
-0.877429421992487,-0.874380391823306,-0.869092894546673,-0.843684647440481,
-0.809416338882272,-0.787776625017307,-0.784651797334878,-0.782727512220894,
-0.78122928828612,-0.779464671914078,-0.776213097806986,-0.757031339542577,
-0.718189338689354,-0.707008573991512,-0.69317330880848,-0.688618202861663,
-0.68572859672968,-0.683025537646131,-0.679412424831105,-0.671254008276013,
-0.660051178133697,-0.627218225834422,-0.59696077961473,-0.592014492293333,
-0.590074366644002,-0.588668617756306,-0.587110685802799,-0.58480745382514,
-0.578455726437245,-0.535045578816015,-0.502037618027926,-0.49691265809777,
-0.493602900567647,-0.490936898281507,-0.48788700403431,-0.482595408226687,
-0.457102972014939,-0.422382293104705,-0.411609293767327,-0.400364188362582,
-0.39743114527212,-0.395735550918995,-0.394225006123276,-0.392188881164949,
-0.387542776652187,-0.366323765661868,-0.352429809005365,-0.311874991196785,
-0.304269038113326,-0.300792541335656,-0.298101005782164,-0.295179231159805,
-0.290476160073781,-0.273693586696225,-0.241274892374953,-0.210465338169429,
-0.205519084545317,-0.203578958087331,-0.202173203462676,-0.200646575954329,
-0.198418594633079,-0.195828334265892,-0.191064542594281,-0.142545504539599,
-0.115283373729028,-0.109800370965303,-0.106676548222583,-0.104281696601305,
-0.101175562291424,-0.0956222642232126,-0.0632739055048681,-0.0223188693324635,
-0.0134075072082791,-0.0107024827845414,-0.00905719579829945,-0.0076267449158626,
-0.00611663410577336,-0.00356811798796674,-0.000573380549723848),
 .UNSPECIFIED.);
#1150=B_SPLINE_CURVE_WITH_KNOTS('',3,(#21141,#21142,#21143,#21144,#21145,
#21146,#21147,#21148,#21149,#21150,#21151,#21152,#21153,#21154,#21155,#21156,
#21157,#21158,#21159,#21160,#21161,#21162,#21163,#21164,#21165,#21166,#21167,
#21168,#21169,#21170,#21171,#21172,#21173,#21174,#21175,#21176,#21177,#21178,
#21179,#21180,#21181,#21182),.UNSPECIFIED.,.F.,.F.,(4,2,2,2,2,2,2,2,2,2,
2,2,2,2,2,2,2,2,2,2,4),(-2.4308877319842,-2.40572329914951,-2.38654123381901,
-2.3572219218908,-2.34858689679086,-2.34489311136623,-2.34217776507696,
-2.33931915586052,-2.33490404708301,-2.32218461137482,-2.26758946851478,
-2.25664267001732,-2.25202917463806,-2.24949613063449,-2.24735265802882,
-2.24583264341316,-2.24442746066131,-2.24248841672118,-2.23754619127848,
-2.20688713278786,-2.18888770495768),.UNSPECIFIED.);
#1151=B_SPLINE_CURVE_WITH_KNOTS('',3,(#21184,#21185,#21186,#21187,#21188,
#21189,#21190,#21191,#21192,#21193,#21194,#21195,#21196,#21197,#21198,#21199,
#21200,#21201,#21202,#21203,#21204,#21205,#21206,#21207,#21208,#21209,#21210,
#21211,#21212,#21213,#21214,#21215,#21216,#21217,#21218,#21219,#21220,#21221,
#21222,#21223,#21224,#21225,#21226,#21227,#21228,#21229,#21230,#21231,#21232,
#21233,#21234,#21235,#21236,#21237,#21238,#21239,#21240,#21241,#21242,#21243,
#21244,#21245),.UNSPECIFIED.,.F.,.F.,(4,2,2,2,2,2,2,2,2,2,2,2,2,2,2,2,2,
2,2,2,2,2,2,2,2,2,2,2,2,2,4),(-0.242722284356607,-0.226318259385084,-0.22120460494511,
-0.217898602287688,-0.215233340481677,-0.215182011302106,-0.215143779362832,
-0.215083835499035,-0.215027516824497,-0.211975580060041,-0.208709367535101,
-0.203661761444521,-0.194061184282351,-0.168978162152365,-0.128935362626007,
-0.123295441388878,-0.121032386526694,-0.119498167859693,-0.117894973057576,
-0.115379671990079,-0.107330219378015,-0.0934241922212276,-0.0512612172895995,
-0.0327255814975402,-0.0272962239111053,-0.0241847876084111,-0.0217759015420467,
-0.0192546829051084,-0.0161911752762037,-0.00990648707394315,-0.00057360079793139),
 .UNSPECIFIED.);
#1152=B_SPLINE_CURVE_WITH_KNOTS('',3,(#21246,#21247,#21248,#21249,#21250,
#21251,#21252,#21253,#21254,#21255,#21256,#21257,#21258,#21259,#21260,#21261,
#21262,#21263,#21264,#21265,#21266,#21267,#21268,#21269,#21270,#21271,#21272,
#21273,#21274,#21275,#21276,#21277,#21278,#21279,#21280,#21281,#21282,#21283,
#21284,#21285,#21286,#21287,#21288,#21289,#21290,#21291,#21292,#21293,#21294,
#21295,#21296,#21297,#21298,#21299,#21300,#21301,#21302,#21303,#21304,#21305,
#21306,#21307,#21308,#21309,#21310,#21311,#21312,#21313,#21314,#21315,#21316,
#21317,#21318,#21319,#21320,#21321,#21322,#21323,#21324,#21325,#21326,#21327,
#21328,#21329,#21330,#21331,#21332,#21333,#21334,#21335,#21336,#21337,#21338,
#21339,#21340,#21341,#21342,#21343,#21344,#21345,#21346,#21347,#21348,#21349,
#21350,#21351,#21352,#21353,#21354,#21355,#21356,#21357,#21358,#21359,#21360,
#21361,#21362,#21363,#21364,#21365,#21366,#21367,#21368,#21369,#21370,#21371,
#21372,#21373,#21374,#21375,#21376,#21377,#21378,#21379,#21380,#21381,#21382,
#21383,#21384,#21385,#21386,#21387,#21388,#21389,#21390,#21391,#21392,#21393,
#21394,#21395,#21396,#21397,#21398,#21399,#21400,#21401,#21402,#21403,#21404,
#21405,#21406,#21407,#21408,#21409,#21410,#21411,#21412,#21413,#21414,#21415,
#21416,#21417,#21418,#21419,#21420,#21421,#21422,#21423),.UNSPECIFIED.,
 .F.,.F.,(4,2,2,2,2,2,2,2,2,2,2,2,2,2,2,2,2,2,2,2,2,2,2,2,2,2,2,2,2,2,2,
2,2,2,2,2,2,2,2,2,2,2,2,2,2,2,2,2,2,2,2,2,2,2,2,2,2,2,2,2,2,2,2,2,2,2,2,
2,2,2,2,2,2,2,2,2,2,2,2,2,2,2,2,2,2,2,2,2,4),(-2.43072114342198,-2.38276134734879,
-2.36879770025489,-2.36072718495424,-2.35821004161092,-2.35660680600177,
-2.35507351307365,-2.35317550959972,-2.34847524724012,-2.31077926545563,
-2.28801107601814,-2.27515887765741,-2.2689788211344,-2.26524959406597,
-2.26187752410252,-2.26181526849542,-2.26178716691591,-2.2617563388158,
-2.26172245002302,-2.26168511195143,-2.26164386986024,-2.25908620410354,
-2.25610229025896,-2.25111016739191,-2.23315677617736,-2.18976770432065,
-2.17566124075281,-2.16753467588931,-2.16501116048251,-2.16340645597938,
-2.16187399488937,-2.15997937094444,-2.15529911200416,-2.11708003630143,
-2.08982473700654,-2.07973586822317,-2.07220657030665,-2.06870726012314,
-2.06602180216787,-2.06308493925768,-2.05830887488936,-2.04249631680944,
-2.00169566616791,-1.97596383251657,-1.97253734310369,-1.97073623965491,
-1.96924137849381,-1.9673646643111,-1.96439723563123,-1.94775450060935,
-1.90890171522837,-1.88288479493016,-1.87756958646194,-1.87451533452724,
-1.87185095261923,-1.86855025571772,-1.86345285229067,-1.83277661150112,
-1.78478913746452,-1.78000728641993,-1.77794786395009,-1.7764343884367,
-1.77475134709595,-1.77187389523294,-1.76125209015473,-1.72539049655759,
-1.6913224699871,-1.68501461540306,-1.68175167537826,-1.67908952215944,
-1.6760063166571,-1.67070072643705,-1.64726180099989,-1.60837527431319,
-1.58916777450283,-1.58591577596048,-1.58415139795992,-1.58265366920229,
-1.5807304568846,-1.57760826524219,-1.555500156363,-1.52163916867148,-1.49632195760372,
-1.49104018898702,-1.4879929511025,-1.48532750636872,-1.48201615788284,
-1.4768843119462,-1.45771362438087),.UNSPECIFIED.);
#1153=B_SPLINE_CURVE_WITH_KNOTS('',3,(#21428,#21429,#21430,#21431,#21432,
#21433,#21434,#21435,#21436,#21437,#21438,#21439,#21440,#21441,#21442,#21443,
#21444,#21445,#21446,#21447,#21448,#21449,#21450,#21451,#21452,#21453,#21454,
#21455,#21456,#21457,#21458,#21459,#21460,#21461,#21462,#21463,#21464,#21465,
#21466,#21467,#21468,#21469,#21470,#21471,#21472,#21473,#21474,#21475,#21476,
#21477,#21478,#21479,#21480,#21481,#21482,#21483,#21484,#21485,#21486,#21487,
#21488,#21489,#21490,#21491,#21492,#21493,#21494,#21495,#21496,#21497,#21498,
#21499,#21500,#21501,#21502,#21503,#21504,#21505,#21506,#21507,#21508,#21509,
#21510,#21511,#21512,#21513,#21514,#21515,#21516,#21517,#21518,#21519,#21520,
#21521,#21522,#21523,#21524,#21525,#21526,#21527,#21528,#21529,#21530,#21531,
#21532,#21533,#21534,#21535,#21536,#21537,#21538,#21539,#21540,#21541,#21542,
#21543,#21544,#21545,#21546,#21547,#21548,#21549,#21550,#21551,#21552,#21553,
#21554,#21555,#21556,#21557,#21558,#21559,#21560,#21561,#21562,#21563,#21564,
#21565,#21566,#21567,#21568,#21569,#21570,#21571,#21572,#21573,#21574,#21575,
#21576,#21577,#21578,#21579,#21580,#21581,#21582,#21583,#21584,#21585,#21586,
#21587,#21588,#21589,#21590,#21591,#21592,#21593,#21594,#21595,#21596,#21597,
#21598,#21599,#21600,#21601,#21602,#21603,#21604,#21605,#21606,#21607,#21608,
#21609,#21610,#21611,#21612,#21613,#21614,#21615,#21616,#21617,#21618,#21619,
#21620,#21621,#21622,#21623,#21624,#21625,#21626,#21627,#21628,#21629,#21630,
#21631,#21632,#21633,#21634,#21635,#21636,#21637,#21638,#21639),
 .UNSPECIFIED.,.F.,.F.,(4,2,2,2,2,2,2,2,2,2,2,2,2,2,2,2,2,2,2,2,2,2,2,2,
2,2,2,2,2,2,2,2,2,2,2,2,2,2,2,2,2,2,2,2,2,2,2,2,2,2,2,2,2,2,2,2,2,2,2,2,
2,2,2,2,2,2,2,2,2,2,2,2,2,2,2,2,2,2,2,2,2,2,2,2,2,2,2,2,2,2,2,2,2,2,2,2,
2,2,2,2,2,2,2,2,2,4),(-2.18887902963404,-2.18779188971815,-2.14458953969837,
-2.13824969393521,-2.13594842248798,-2.13439114163079,-2.13298544183683,
-2.13104471703317,-2.12609350142366,-2.09669228265521,-2.06440082352862,
-2.0463670771056,-2.04155693725538,-2.03861220791026,-2.03592809262195,
-2.03250060481311,-2.02516071506774,-1.9798097606552,-1.97156333430698,
-1.94711875847882,-1.94371736288988,-1.94192125821609,-1.94042577121953,
-1.93854220906575,-1.93555284436288,-1.9183831448492,-1.90436129199647,
-1.88057157478502,-1.85570341255035,-1.84946564663623,-1.84621659021721,
-1.84355463634892,-1.84045908688399,-1.83510062419631,-1.81067803282439,
-1.7724906343299,-1.75365097440494,-1.7504122192542,-1.74865045401465,-1.74715209650678,
-1.74522436266864,-1.74208761634755,-1.7191674717933,-1.67918445458263,
-1.66010267785497,-1.65520884403076,-1.65224565862551,-1.64956578452849,
-1.64611563298955,-1.63885393747365,-1.59262975537905,-1.57043742882706,
-1.56317742478124,-1.55813637820146,-1.55603272210668,-1.55451209701436,
-1.55284854193223,-1.55006047043855,-1.54041060039024,-1.49782899287477,
-1.47053882238745,-1.46347976150915,-1.46006810383705,-1.45739272614607,
-1.45440836201934,-1.44941748281705,-1.43164248648742,-1.38269062400031,
-1.37209248498086,-1.36543427394653,-1.36308930374289,-1.3615227641838,
-1.36012441989612,-1.35821359358642,-1.35344143863045,-1.31685842951866,
-1.28852631141926,-1.27298714008495,-1.26840126191458,-1.26550502906752,
-1.26280466704692,-1.25927044523936,-1.25164384538175,-1.21558541551855,
-1.17621304810398,-1.17148743978843,-1.16964060539473,-1.16811992585334,
-1.16649383191799,-1.16387548828637,-1.15485953794626,-1.13837303329464,
-1.12568279567418,-1.08484665284819,-1.07725059933467,-1.07377588084827,
-1.07108459708419,-1.06816197155948,-1.06345503779931,-1.04662967522134,
-1.01405979828696,-0.98346852379255,-0.978510534681342,-0.976568391694447,
-0.975162117925436,-0.97373548788866),.UNSPECIFIED.);
#1154=B_SPLINE_CURVE_WITH_KNOTS('',3,(#21640,#21641,#21642,#21643,#21644,
#21645,#21646,#21647,#21648,#21649,#21650,#21651,#21652,#21653,#21654,#21655,
#21656,#21657,#21658,#21659,#21660,#21661,#21662,#21663,#21664,#21665,#21666,
#21667,#21668,#21669,#21670,#21671,#21672,#21673,#21674,#21675,#21676,#21677,
#21678,#21679,#21680,#21681,#21682,#21683,#21684,#21685,#21686,#21687,#21688,
#21689,#21690,#21691,#21692,#21693,#21694,#21695,#21696,#21697,#21698,#21699,
#21700,#21701,#21702,#21703,#21704,#21705,#21706,#21707,#21708,#21709,#21710,
#21711,#21712,#21713,#21714,#21715,#21716,#21717,#21718,#21719,#21720,#21721,
#21722,#21723,#21724,#21725,#21726,#21727,#21728,#21729,#21730,#21731,#21732,
#21733,#21734,#21735,#21736,#21737,#21738,#21739,#21740,#21741,#21742,#21743,
#21744,#21745,#21746,#21747,#21748,#21749,#21750,#21751,#21752,#21753,#21754,
#21755,#21756,#21757,#21758,#21759,#21760,#21761,#21762,#21763,#21764,#21765,
#21766,#21767,#21768,#21769,#21770,#21771,#21772,#21773,#21774,#21775,#21776,
#21777,#21778,#21779,#21780,#21781,#21782,#21783,#21784,#21785,#21786,#21787,
#21788,#21789,#21790,#21791,#21792,#21793,#21794,#21795,#21796,#21797,#21798,
#21799,#21800,#21801,#21802,#21803,#21804,#21805,#21806,#21807,#21808,#21809,
#21810,#21811,#21812,#21813,#21814,#21815,#21816,#21817,#21818,#21819,#21820,
#21821,#21822,#21823,#21824,#21825,#21826,#21827,#21828,#21829,#21830,#21831,
#21832,#21833,#21834,#21835,#21836,#21837,#21838,#21839,#21840,#21841,#21842,
#21843),.UNSPECIFIED.,.F.,.F.,(4,2,2,2,2,2,2,2,2,2,2,2,2,2,2,2,2,2,2,2,
2,2,2,2,2,2,2,2,2,2,2,2,2,2,2,2,2,2,2,2,2,2,2,2,2,2,2,2,2,2,2,2,2,2,2,2,
2,2,2,2,2,2,2,2,2,2,2,2,2,2,2,2,2,2,2,2,2,2,2,2,2,2,2,2,2,2,2,2,2,2,2,2,
2,2,2,2,2,2,2,2,2,4),(-1.45771362438087,-1.44042256863282,-1.41399613211339,
-1.39586250675788,-1.39265172242565,-1.39089612954797,-1.38939737789245,
-1.38746187054114,-1.38429831392562,-1.35951211632451,-1.35277051501603,
-1.32818523683517,-1.30307746458597,-1.29780601040883,-1.2947609234272,
-1.29209511672579,-1.28878039382736,-1.2836376629233,-1.24835200954516,
-1.21559674475117,-1.20240893850855,-1.19935924627799,-1.19762033398754,
-1.19626970511579,-1.19439158724814,-1.19058812509207,-1.16040482887616,
-1.11287268119788,-1.10574900670334,-1.10232533647546,-1.09964898027898,
-1.09667222563652,-1.0917148101817,-1.07177465942165,-1.02472905344581,
-1.00933686210975,-1.00615464267641,-1.00438570022016,-1.00288824948975,
-1.00097072482877,-0.996966241393652,-0.991594654335988,-0.97785942373292,
-0.936875085724848,-0.916349886461119,-0.911226143515123,-0.908184034343339,
-0.905543163612789,-0.902236222277869,-0.895711341102798,-0.887319638126186,
-0.867067484876713,-0.842139587236554,-0.816595305298695,-0.813424871707151,
-0.81148728411627,-0.809988284158567,-0.808233972044277,-0.805029465425721,
-0.787049734118612,-0.760781535610508,-0.723975493133445,-0.718874583209737,
-0.715572499401652,-0.71290759203684,-0.709853388922403,-0.704539966444257,
-0.678580991744954,-0.640357146823222,-0.623018272463115,-0.620021929988422,
-0.618136314402451,-0.616640801704105,-0.614846618791814,-0.61145419257761,
-0.587408093184771,-0.57413411884912,-0.533845271999984,-0.526230477237613,
-0.522752830216865,-0.520061602518235,-0.517141368687712,-0.512443476116218,
-0.495711471755008,-0.463469771819595,-0.43243120601779,-0.427473836368519,
-0.425532040276686,-0.424126057893796,-0.422569062606413,-0.420269284231241,
-0.413940270099266,-0.370941323991666,-0.337493047809635,-0.332363644730183,
-0.329052902822178,-0.326387339871642,-0.323339304539173,-0.31805446218761,
-0.292685391250116,-0.258662021533076,-0.242408550118657),.UNSPECIFIED.);
#1155=B_SPLINE_CURVE_WITH_KNOTS('',3,(#21849,#21850,#21851,#21852,#21853,
#21854,#21855,#21856,#21857,#21858,#21859,#21860,#21861,#21862,#21863,#21864,
#21865,#21866,#21867,#21868,#21869,#21870,#21871,#21872,#21873,#21874,#21875,
#21876,#21877,#21878,#21879,#21880,#21881,#21882,#21883,#21884,#21885,#21886,
#21887,#21888,#21889,#21890,#21891,#21892,#21893,#21894,#21895,#21896,#21897,
#21898,#21899,#21900,#21901,#21902,#21903,#21904,#21905,#21906,#21907,#21908,
#21909,#21910,#21911,#21912,#21913,#21914,#21915,#21916,#21917,#21918,#21919,
#21920,#21921,#21922,#21923,#21924,#21925,#21926,#21927,#21928,#21929,#21930,
#21931,#21932,#21933,#21934,#21935,#21936,#21937,#21938,#21939,#21940,#21941,
#21942,#21943,#21944,#21945,#21946,#21947,#21948,#21949,#21950,#21951,#21952,
#21953,#21954,#21955,#21956,#21957,#21958,#21959,#21960,#21961,#21962,#21963,
#21964,#21965,#21966,#21967,#21968,#21969,#21970,#21971,#21972,#21973,#21974,
#21975,#21976,#21977,#21978,#21979,#21980,#21981,#21982,#21983,#21984,#21985,
#21986,#21987,#21988,#21989,#21990,#21991,#21992,#21993,#21994,#21995,#21996,
#21997,#21998,#21999,#22000,#22001,#22002,#22003,#22004,#22005,#22006,#22007,
#22008,#22009,#22010,#22011,#22012,#22013,#22014,#22015,#22016,#22017,#22018,
#22019,#22020,#22021,#22022,#22023,#22024,#22025,#22026,#22027,#22028,#22029,
#22030,#22031,#22032,#22033,#22034,#22035,#22036,#22037,#22038),
 .UNSPECIFIED.,.F.,.F.,(4,2,2,2,2,2,2,2,2,2,2,2,2,2,2,2,2,2,2,2,2,2,2,2,
2,2,2,2,2,2,2,2,2,2,2,2,2,2,2,2,2,2,2,2,2,2,2,2,2,2,2,2,2,2,2,2,2,2,2,2,
2,2,2,2,2,2,2,2,2,2,2,2,2,2,2,2,2,2,2,2,2,2,2,2,2,2,2,2,2,2,2,2,2,2,4),
(-0.973910253760765,-0.970007335956458,-0.964667944357671,-0.961576352313021,
-0.958913621710933,-0.955658361597496,-0.949392046898408,-0.91112105632681,
-0.871659387208275,-0.866939882565676,-0.865093908203904,-0.863573345849303,
-0.861946636119496,-0.859325930210996,-0.850287972304353,-0.833740452778761,
-0.82193107628202,-0.780241949326078,-0.772678529725419,-0.769209537951511,
-0.766518907252409,-0.763593202294974,-0.758872884172139,-0.741900740212514,
-0.708807985344714,-0.67889608448649,-0.673943935020186,-0.672002696917308,
-0.670596576677982,-0.669038754928178,-0.666736571655642,-0.660393359338801,
-0.617147114423141,-0.583959659125359,-0.578832377611862,-0.575521746446493,
-0.572855445137152,-0.569805650796398,-0.564515367204381,-0.539057550574652,
-0.504539140678535,-0.493805736823831,-0.482311645400885,-0.479357328303278,
-0.477656965076492,-0.476147471472981,-0.474119931413592,-0.469523055971169,
-0.448768158291233,-0.412539521157562,-0.390043428086862,-0.38478985217901,
-0.38171762119792,-0.379053360498759,-0.375773064954076,-0.369383835400975,
-0.326330713663641,-0.29224060814059,-0.287357532236295,-0.285427782319721,
-0.28402453072648,-0.282463307492475,-0.280144862564058,-0.273684522411905,
-0.263524488281457,-0.234864010360416,-0.197416756382406,-0.191838908032126,
-0.188669621715466,-0.186071841971015,-0.185953164450266,-0.185842802818211,
-0.185739176926683,-0.18564104505233,-0.185547409424046,-0.18545745196806,
-0.185370489254994,-0.185285940113418,-0.185203301766309,-0.185122131959548,
-0.185042035091654,-0.181629860913606,-0.17770542800625,-0.148797542523752,
-0.113508106682466,-0.0963909586767748,-0.0934027590896143,-0.0915192262306326,
-0.0900232638601776,-0.0882259807922269,-0.0848207291040813,-0.0602277111366393,
-0.00936464206830907,-0.00384968017010287,-0.00057394889050387),
 .UNSPECIFIED.);
#1156=B_SPLINE_CURVE_WITH_KNOTS('',3,(#22039,#22040,#22041,#22042,#22043,
#22044,#22045,#22046,#22047,#22048,#22049,#22050,#22051,#22052,#22053,#22054,
#22055,#22056,#22057,#22058,#22059,#22060,#22061,#22062,#22063,#22064,#22065,
#22066,#22067,#22068,#22069,#22070,#22071,#22072,#22073,#22074,#22075,#22076,
#22077,#22078,#22079,#22080,#22081,#22082,#22083,#22084,#22085,#22086),
 .UNSPECIFIED.,.F.,.F.,(4,2,2,2,2,2,2,2,2,2,2,2,2,2,2,2,2,2,2,2,2,2,2,4),
(-2.43085648084854,-2.42887934336279,-2.42647850822906,-2.42393550147241,
-2.42107988776888,-2.41684207527017,-2.40480128623111,-2.35859764609427,
-2.33571224737799,-2.33089544752737,-2.32882995986386,-2.32731553120602,
-2.32563524922959,-2.32277050655347,-2.31228859045544,-2.27633802420747,
-2.25267587834801,-2.2387796649061,-2.23548276615809,-2.23240114174611,
-2.22979458349587,-2.22662945598436,-2.22106611756832,-2.18887902963404),
 .UNSPECIFIED.);
#1157=B_SPLINE_CURVE_WITH_KNOTS('',3,(#22088,#22089,#22090,#22091,#22092,
#22093,#22094,#22095,#22096,#22097,#22098,#22099,#22100,#22101,#22102,#22103,
#22104,#22105,#22106,#22107,#22108,#22109,#22110,#22111,#22112,#22113,#22114,
#22115,#22116,#22117,#22118,#22119,#22120,#22121,#22122,#22123,#22124,#22125,
#22126,#22127,#22128,#22129,#22130,#22131,#22132,#22133,#22134,#22135,#22136,
#22137,#22138,#22139),.UNSPECIFIED.,.F.,.F.,(4,2,2,2,2,2,2,2,2,2,2,2,2,
2,2,2,2,2,2,2,2,2,2,2,2,4),(-0.242408550118657,-0.236717564735722,-0.233597745241758,
-0.231675167927113,-0.230177381040449,-0.228412269050664,-0.225272045602489,
-0.221258788898725,-0.212327099012181,-0.179844890610788,-0.144261837331527,
-0.139122017576931,-0.135808131122734,-0.133142346452952,-0.130096575382254,
-0.124822129015066,-0.101721457752813,-0.0693196227094799,-0.0435634375784882,
-0.0403919137704319,-0.0384540101339557,-0.0369549914634115,-0.0352009208108212,
-0.0333298928224582,-0.0303889327839463,-0.000573497123783065),
 .UNSPECIFIED.);
#1158=B_SPLINE_CURVE_WITH_KNOTS('',3,(#22140,#22141,#22142,#22143,#22144,
#22145,#22146,#22147,#22148,#22149,#22150,#22151,#22152,#22153,#22154,#22155,
#22156,#22157,#22158,#22159,#22160,#22161,#22162,#22163,#22164,#22165,#22166,
#22167,#22168,#22169,#22170,#22171,#22172,#22173,#22174,#22175,#22176,#22177,
#22178,#22179,#22180,#22181,#22182,#22183,#22184,#22185,#22186,#22187,#22188,
#22189,#22190,#22191,#22192,#22193,#22194,#22195,#22196,#22197,#22198,#22199,
#22200,#22201,#22202,#22203,#22204,#22205,#22206,#22207,#22208,#22209,#22210,
#22211,#22212,#22213,#22214,#22215,#22216,#22217,#22218,#22219,#22220,#22221,
#22222,#22223,#22224,#22225,#22226,#22227,#22228,#22229,#22230,#22231,#22232,
#22233,#22234,#22235,#22236,#22237,#22238,#22239,#22240,#22241,#22242,#22243,
#22244,#22245,#22246,#22247,#22248,#22249,#22250,#22251,#22252,#22253,#22254,
#22255,#22256,#22257,#22258,#22259,#22260,#22261,#22262,#22263,#22264,#22265,
#22266,#22267,#22268,#22269,#22270,#22271,#22272,#22273,#22274,#22275,#22276,
#22277,#22278,#22279,#22280,#22281,#22282,#22283,#22284,#22285,#22286,#22287,
#22288,#22289,#22290,#22291,#22292,#22293,#22294,#22295,#22296,#22297,#22298,
#22299,#22300,#22301,#22302,#22303,#22304,#22305,#22306,#22307),
 .UNSPECIFIED.,.F.,.F.,(4,2,2,2,2,2,2,2,2,2,2,2,2,2,2,2,2,2,2,2,2,2,2,2,
2,2,2,2,2,2,2,2,2,2,2,2,2,2,2,2,2,2,2,2,2,2,2,2,2,2,2,2,2,2,2,2,2,2,2,2,
2,2,2,2,2,2,2,2,2,2,2,2,2,2,2,2,2,2,2,2,2,2,2,4),(-2.43118060654611,-2.39196463195278,
-2.3809253323704,-2.37561453331713,-2.37256143721174,-2.36989725642257,
-2.36659576347962,-2.36149512428364,-2.32465356621113,-2.29362904853487,
-2.28451810846221,-2.27862253645854,-2.27642174469659,-2.2748560104628,
-2.2734582909036,-2.27154822780952,-2.26677753380414,-2.2302723028536,-2.20189143935604,
-2.19156205004826,-2.18389507731415,-2.18037068504966,-2.17768191026985,
-2.17475706331223,-2.17003557193757,-2.15471966165479,-2.14713155745807,
-2.1064341139553,-2.08729506461695,-2.08404597051078,-2.08228237933332,
-2.08078483115809,-2.07886122321812,-2.07573717832556,-2.05416041397805,
-2.01987877406766,-1.99447550416318,-1.98919010730847,-1.98614238427989,
-1.98347746232974,-1.98016799574784,-1.9750414445666,-1.9417843913852,-1.89858104190176,
-1.89224129540744,-1.88994027453577,-1.88838323447976,-1.88697782964416,
-1.88503763803769,-1.88008844053518,-1.8501980744753,-1.81712877061964,
-1.8001653238274,-1.79544731112538,-1.79252301168753,-1.78983366583339,
-1.78636633137133,-1.77880668002459,-1.73703102362976,-1.72529624345423,
-1.70873127944794,-1.69968890412828,-1.69706851448798,-1.6954423769428,
-1.69392266450157,-1.69207810075664,-1.6873641910727,-1.64788570824375,
-1.60977856535439,-1.60345220448604,-1.60018561015662,-1.59752338242236,
-1.59444334597592,-1.58915130795254,-1.56595436450651,-1.52693288556181,
-1.50760561576952,-1.50434940332452,-1.50258418239375,-1.50108662753164,
-1.49916478288441,-1.49604701680975,-1.47434180177083,-1.45794268266291),
 .UNSPECIFIED.);
#1159=B_SPLINE_CURVE_WITH_KNOTS('',3,(#22312,#22313,#22314,#22315,#22316,
#22317,#22318,#22319,#22320,#22321,#22322,#22323,#22324,#22325,#22326,#22327,
#22328,#22329,#22330,#22331,#22332,#22333,#22334,#22335,#22336,#22337,#22338,
#22339,#22340,#22341,#22342,#22343,#22344,#22345,#22346,#22347,#22348,#22349,
#22350,#22351,#22352,#22353,#22354,#22355,#22356,#22357,#22358,#22359,#22360,
#22361,#22362,#22363,#22364,#22365,#22366,#22367,#22368,#22369,#22370,#22371,
#22372,#22373,#22374,#22375,#22376,#22377,#22378,#22379,#22380,#22381,#22382,
#22383,#22384,#22385,#22386,#22387,#22388,#22389,#22390,#22391,#22392,#22393,
#22394,#22395,#22396,#22397,#22398,#22399,#22400,#22401,#22402,#22403,#22404,
#22405,#22406,#22407,#22408,#22409,#22410,#22411,#22412,#22413,#22414,#22415,
#22416,#22417,#22418,#22419,#22420,#22421,#22422,#22423,#22424,#22425,#22426,
#22427,#22428,#22429,#22430,#22431,#22432,#22433,#22434,#22435,#22436,#22437,
#22438,#22439,#22440,#22441,#22442,#22443,#22444,#22445,#22446,#22447,#22448,
#22449,#22450,#22451,#22452,#22453,#22454,#22455,#22456,#22457,#22458,#22459,
#22460,#22461,#22462,#22463,#22464,#22465,#22466,#22467,#22468,#22469,#22470,
#22471,#22472,#22473,#22474,#22475,#22476,#22477,#22478,#22479,#22480,#22481,
#22482,#22483,#22484,#22485,#22486,#22487,#22488,#22489,#22490,#22491,#22492,
#22493,#22494,#22495,#22496,#22497,#22498,#22499,#22500,#22501,#22502,#22503,
#22504,#22505,#22506,#22507,#22508,#22509,#22510,#22511,#22512,#22513,#22514,
#22515,#22516,#22517),.UNSPECIFIED.,.F.,.F.,(4,2,2,2,2,2,2,2,2,2,2,2,2,
2,2,2,2,2,2,2,2,2,2,2,2,2,2,2,2,2,2,2,2,2,2,2,2,2,2,2,2,2,2,2,2,2,2,2,2,
2,2,2,2,2,2,2,2,2,2,2,2,2,2,2,2,2,2,2,2,2,2,2,2,2,2,2,2,2,2,2,2,2,2,2,2,
2,2,2,2,2,2,2,2,2,2,2,2,2,2,2,2,2,4),(-2.18915184178403,-2.15490999477389,
-2.12934284439123,-2.12404765414707,-2.12099690624184,-2.11833086968842,
-2.11502199532586,-2.10990013838036,-2.07245149451288,-2.04381121124193,
-2.03361443564529,-2.0271380977853,-2.02481763265576,-2.02325613646213,
-2.02185347927595,-2.0199256280696,-2.01505300186312,-1.98075382772371,
-1.95086985910927,-1.9402303164555,-1.93238640388379,-1.92882890385024,
-1.92613420710193,-1.92322163857381,-1.91856116240269,-1.90382209648975,
-1.86207770094449,-1.83823982733854,-1.8333281168825,-1.83124601000624,
-1.82972864175353,-1.82805520105691,-1.82522306717366,-1.81510238335029,
-1.77887203181308,-1.74477528697373,-1.73834683113047,-1.73505875360406,
-1.73239414653274,-1.72932813196587,-1.72410141056089,-1.70204385928499,
-1.66235668161618,-1.64888273188695,-1.64357872247701,-1.63961342816253,
-1.63770320160982,-1.6363487401082,-1.6346312495718,-1.63167656027281,-1.61981590200441,
-1.61021933546096,-1.57859516134911,-1.5594777374016,-1.55139465839931,
-1.54505788097344,-1.54178826282123,-1.53912471138593,-1.53604440800509,
-1.53075501662727,-1.50763454073341,-1.46857267785558,-1.44919311550179,
-1.44593392733638,-1.44416757799018,-1.44266935110309,-1.44074696870063,
-1.43762893070031,-1.41582932483268,-1.38170779025377,-1.35633135472746,
-1.35104517410425,-1.34799620257989,-1.34532970765976,-1.34201764868971,
-1.33688581603828,-1.30026302319391,-1.27371520508049,-1.25583597384861,
-1.25263466486787,-1.2508806650077,-1.24938100123402,-1.24744132589427,
-1.24426505959426,-1.21611646879554,-1.16847562782958,-1.15992461066259,
-1.15651728394349,-1.15400981362371,-1.15128505896313,-1.14754291434882,
-1.13862344030486,-1.11156221845835,-1.08570731636402,-1.06302336013755,
-1.05988994033273,-1.057963036089,-1.05646451961364,-1.05470160784962,-1.05145835426928,
-1.03250609183763,-0.994058097561331,-0.973910253760765),.UNSPECIFIED.);
#1160=B_SPLINE_CURVE_WITH_KNOTS('',3,(#22518,#22519,#22520,#22521,#22522,
#22523,#22524,#22525,#22526,#22527,#22528,#22529,#22530,#22531,#22532,#22533,
#22534,#22535,#22536,#22537,#22538,#22539,#22540,#22541,#22542,#22543,#22544,
#22545,#22546,#22547,#22548,#22549,#22550,#22551,#22552,#22553,#22554,#22555,
#22556,#22557,#22558,#22559,#22560,#22561,#22562,#22563,#22564,#22565,#22566,
#22567,#22568,#22569,#22570,#22571,#22572,#22573,#22574,#22575,#22576,#22577,
#22578,#22579,#22580,#22581,#22582,#22583,#22584,#22585,#22586,#22587,#22588,
#22589,#22590,#22591,#22592,#22593,#22594,#22595,#22596,#22597,#22598,#22599,
#22600,#22601,#22602,#22603,#22604,#22605,#22606,#22607,#22608,#22609,#22610,
#22611,#22612,#22613,#22614,#22615,#22616,#22617,#22618,#22619,#22620,#22621,
#22622,#22623,#22624,#22625,#22626,#22627,#22628,#22629,#22630,#22631,#22632,
#22633,#22634,#22635,#22636,#22637,#22638,#22639,#22640,#22641,#22642,#22643,
#22644,#22645,#22646,#22647,#22648,#22649,#22650,#22651,#22652,#22653,#22654,
#22655,#22656,#22657,#22658,#22659,#22660,#22661,#22662,#22663,#22664,#22665,
#22666,#22667,#22668,#22669,#22670,#22671,#22672,#22673,#22674,#22675,#22676,
#22677,#22678,#22679,#22680,#22681,#22682,#22683,#22684,#22685,#22686,#22687,
#22688,#22689,#22690,#22691,#22692,#22693,#22694,#22695,#22696,#22697,#22698,
#22699,#22700,#22701,#22702,#22703,#22704,#22705,#22706,#22707,#22708,#22709,
#22710,#22711,#22712,#22713,#22714,#22715,#22716,#22717,#22718,#22719,#22720,
#22721,#22722,#22723,#22724,#22725,#22726,#22727,#22728,#22729),
 .UNSPECIFIED.,.F.,.F.,(4,2,2,2,2,2,2,2,2,2,2,2,2,2,2,2,2,2,2,2,2,2,2,2,
2,2,2,2,2,2,2,2,2,2,2,2,2,2,2,2,2,2,2,2,2,2,2,2,2,2,2,2,2,2,2,2,2,2,2,2,
2,2,2,2,2,2,2,2,2,2,2,2,2,2,2,2,2,2,2,2,2,2,2,2,2,2,2,2,2,2,2,2,2,2,2,2,
2,2,2,2,2,2,2,2,2,4),(-1.45794268266291,-1.44741604209633,-1.41523403763836,
-1.4096870430057,-1.40658285703536,-1.40418878487334,-1.4010649788763,-1.39557942906996,
-1.368235977078,-1.31973183901951,-1.31498320576016,-1.31134506237608,-1.30950018017305,
-1.30815247162596,-1.30638760804386,-1.3032233109807,-1.28815722245847,
-1.24084097654734,-1.22086306844774,-1.21590312159041,-1.21292585344607,
-1.21024966652087,-1.20682708690974,-1.19970896741868,-1.17194602596127,
-1.14588706875495,-1.1215090502018,-1.11835002744888,-1.11641589782808,
-1.11491729963146,-1.11316080137868,-1.10994568863615,-1.0916990789769,
-1.06538139823776,-1.02898729524518,-1.02385073471877,-1.02053797097581,
-1.01787245770853,-1.01482630823605,-1.00954943799119,-0.984333624491158,
-0.95089539424183,-0.928229785922014,-0.925097503499517,-0.923171307247067,
-0.921673356854007,-0.919911167851877,-0.916669426887916,-0.897734553467061,
-0.859316396819779,-0.849172847576924,-0.833933291937676,-0.829219660349825,
-0.826296177641502,-0.823606316291107,-0.820077087298475,-0.812385741515092,
-0.802012983536029,-0.773429723432609,-0.769801592665367,-0.73737707533017,
-0.732451521680624,-0.73051521712097,-0.729110727930674,-0.727552401013611,
-0.72524557892704,-0.718864847481034,-0.674901249235493,-0.642473041565614,
-0.63735448937604,-0.63404722312669,-0.631382174919448,-0.628332232641843,
-0.623037649948009,-0.597461823843092,-0.562234841188767,-0.541711838760622,
-0.538600249233992,-0.536680221536827,-0.535182762950412,-0.533416087002461,
-0.530153227023742,-0.510637425658817,-0.471499603816394,-0.448624523026994,
-0.443350625960008,-0.440274604786087,-0.437611926626121,-0.434339794927307,
-0.427986655175696,-0.419875367136937,-0.400651783053862,-0.365369896465283,
-0.34825509704715,-0.345268039864167,-0.343385344048045,-0.341890137594176,
-0.340093911674002,-0.336691105833041,-0.312151847820454,-0.274447010008433,
-0.254991237744784,-0.249878314528817,-0.246867795098266,-0.244464745431678,
-0.242785158976033),.UNSPECIFIED.);
#1161=B_SPLINE_CURVE_WITH_KNOTS('',3,(#22735,#22736,#22737,#22738,#22739,
#22740,#22741,#22742,#22743,#22744,#22745,#22746,#22747,#22748,#22749,#22750,
#22751,#22752,#22753,#22754,#22755,#22756,#22757,#22758,#22759,#22760,#22761,
#22762,#22763,#22764,#22765,#22766,#22767,#22768,#22769,#22770,#22771,#22772,
#22773,#22774,#22775,#22776,#22777,#22778,#22779,#22780,#22781,#22782,#22783,
#22784,#22785,#22786,#22787,#22788,#22789,#22790,#22791,#22792,#22793,#22794,
#22795,#22796,#22797,#22798,#22799,#22800,#22801,#22802,#22803,#22804,#22805,
#22806,#22807,#22808,#22809,#22810,#22811,#22812,#22813,#22814,#22815,#22816,
#22817,#22818,#22819,#22820,#22821,#22822,#22823,#22824,#22825,#22826,#22827,
#22828,#22829,#22830,#22831,#22832,#22833,#22834,#22835,#22836,#22837,#22838,
#22839,#22840,#22841,#22842,#22843,#22844,#22845,#22846,#22847,#22848,#22849,
#22850,#22851,#22852,#22853,#22854,#22855,#22856,#22857,#22858,#22859,#22860,
#22861,#22862,#22863,#22864,#22865,#22866,#22867,#22868,#22869,#22870,#22871,
#22872,#22873,#22874,#22875,#22876,#22877,#22878,#22879,#22880,#22881,#22882,
#22883,#22884,#22885,#22886,#22887,#22888,#22889,#22890,#22891,#22892,#22893,
#22894,#22895,#22896,#22897,#22898,#22899,#22900,#22901,#22902),
 .UNSPECIFIED.,.F.,.F.,(4,2,2,2,2,2,2,2,2,2,2,2,2,2,2,2,2,2,2,2,2,2,2,2,
2,2,2,2,2,2,2,2,2,2,2,2,2,2,2,2,2,2,2,2,2,2,2,2,2,2,2,2,2,2,2,2,2,2,2,2,
2,2,2,2,2,2,2,2,2,2,2,2,2,2,2,2,2,2,2,2,2,2,2,4),(-0.973989629254837,-0.95370340523295,
-0.949006287027863,-0.947108390963949,-0.945574726407962,-0.943970481800047,
-0.941450662212924,-0.933361580641841,-0.919354220863292,-0.876879867039386,
-0.858036318789459,-0.852975820902075,-0.849976343347942,-0.847571115569945,
-0.84431636718101,-0.838050651751994,-0.830081547811707,-0.811369770786281,
-0.770038718874264,-0.757673886359593,-0.754681189889249,-0.752955156507968,
-0.751602403878788,-0.74970556619611,-0.745807973286562,-0.74062067838746,
-0.727590901734445,-0.688640449053001,-0.665367696956002,-0.660070769465804,
-0.656989085533034,-0.654326136787533,-0.651059537064942,-0.644735961771175,
-0.607644871700186,-0.566942885259483,-0.562339545667482,-0.560332770647229,
-0.558821431547906,-0.557129108857349,-0.554210772635803,-0.541587226277578,
-0.512481966633443,-0.475900708408141,-0.468210944966627,-0.464719486296983,
-0.462025838666575,-0.459111181434841,-0.454440292483736,-0.43800874162127,
-0.384560180050917,-0.371264718516689,-0.368207345636911,-0.366466373572813,
-0.364979287713289,-0.363028789375391,-0.358853087871692,-0.330670806325827,
-0.281389189774354,-0.274471941641788,-0.271087335097601,-0.268414552712803,
-0.26541362182941,-0.260347862576554,-0.23884078735134,-0.211095868981101,
-0.181048084277188,-0.176095616844316,-0.174154413701037,-0.172748376948766,
-0.17122194460444,-0.169094856309564,-0.166569417164278,-0.1619767698802,
-0.151105029433998,-0.0978381037468989,-0.0839777173712444,-0.0794197387270606,
-0.0765296024105952,-0.073826943794206,-0.0702157250734403,-0.062067537268756,
-0.050882973528803,-0.000574376623881859),.UNSPECIFIED.);
#1162=B_SPLINE_CURVE_WITH_KNOTS('',3,(#22903,#22904,#22905,#22906,#22907,
#22908,#22909,#22910,#22911,#22912,#22913,#22914,#22915,#22916,#22917,#22918,
#22919,#22920,#22921,#22922,#22923,#22924,#22925,#22926,#22927,#22928,#22929,
#22930,#22931,#22932,#22933,#22934,#22935,#22936,#22937,#22938,#22939,#22940,
#22941,#22942,#22943,#22944,#22945,#22946,#22947,#22948,#22949,#22950,#22951,
#22952,#22953,#22954,#22955,#22956,#22957,#22958,#22959,#22960,#22961,#22962,
#22963,#22964,#22965,#22966,#22967,#22968,#22969,#22970,#22971,#22972,#22973,
#22974,#22975,#22976,#22977,#22978,#22979,#22980,#22981,#22982,#22983,#22984,
#22985,#22986,#22987,#22988,#22989,#22990,#22991,#22992,#22993,#22994,#22995,
#22996,#22997,#22998,#22999,#23000,#23001,#23002,#23003,#23004,#23005,#23006,
#23007,#23008,#23009,#23010,#23011,#23012,#23013,#23014,#23015,#23016,#23017,
#23018,#23019,#23020,#23021,#23022,#23023,#23024,#23025,#23026,#23027,#23028,
#23029,#23030,#23031,#23032),.UNSPECIFIED.,.F.,.F.,(4,2,2,2,2,2,2,2,2,2,
2,2,2,2,2,2,2,2,2,2,2,2,2,2,2,2,2,2,2,2,2,2,2,2,2,2,2,2,2,2,2,2,2,2,2,2,
2,2,2,2,2,2,2,2,2,2,2,2,2,2,2,2,2,2,4),(-2.43101907711719,-2.4201435497811,
-2.41446115353093,-2.41244095905634,-2.4109370374652,-2.409500923963,-2.40784459936654,
-2.40508954469771,-2.39574741320926,-2.38292146361354,-2.34823399544202,
-2.32258381158638,-2.31728473374966,-2.31423321738437,-2.31156737387828,
-2.30825986190856,-2.30314227594429,-2.26685454718313,-2.240844590539,-2.22820931205344,
-2.22312722866662,-2.21932249573791,-2.21745208274786,-2.21744545958929,
-2.21743877481767,-2.21743202798643,-2.21742521798897,-2.21741834407562,
-2.21741140573566,-2.2174044021135,-2.21739733223398,-2.21739019518902,
-2.21738299025269,-2.21737571665299,-2.21736837358268,-2.2173609600107,
-2.21735347508426,-2.21734591824579,-2.21733828827653,-2.21733058430711,
-2.21732280549441,-2.21731495081584,-2.21730701928989,-2.21729900993269,
-2.21729092185761,-2.21728275405164,-2.21727450538882,-2.21726617507049,
-2.21725776191911,-2.21724926482013,-2.21724068268989,-2.21723201446122,
-2.21722325925826,-2.21721441571959,-2.21720548263654,-2.21719645901663,
-2.21718734360108,-2.21717813541115,-2.21716883304915,-2.21715943530605,
-2.21566153841624,-2.21374197653291,-2.21063311736965,-2.1896358019075,
-2.18915184178403),.UNSPECIFIED.);
#1163=B_SPLINE_CURVE_WITH_KNOTS('',3,(#23034,#23035,#23036,#23037,#23038,
#23039,#23040,#23041,#23042,#23043,#23044,#23045,#23046,#23047,#23048,#23049,
#23050,#23051,#23052,#23053,#23054,#23055,#23056,#23057,#23058,#23059,#23060,
#23061,#23062,#23063,#23064,#23065,#23066,#23067,#23068,#23069,#23070,#23071,
#23072,#23073,#23074,#23075,#23076,#23077),.UNSPECIFIED.,.F.,.F.,(4,2,2,
2,2,2,2,2,2,2,2,2,2,2,2,2,2,2,2,2,2,4),(-0.242785158976033,-0.241227316072973,
-0.235044448781371,-0.227208788780809,-0.208968798338147,-0.164855613220994,
-0.154238467454242,-0.151361302165026,-0.149678282332967,-0.148164701370528,
-0.146105001164423,-0.141515626576424,-0.117068669363286,-0.092648514982216,
-0.0627097051517281,-0.0576267011093042,-0.0543300841093095,-0.0516656013047632,
-0.0486075016806466,-0.0454116381819875,-0.0405346762332557,-0.000573798641427919),
 .UNSPECIFIED.);
#1164=B_SPLINE_CURVE_WITH_KNOTS('',3,(#23078,#23079,#23080,#23081,#23082,
#23083,#23084,#23085,#23086,#23087,#23088,#23089,#23090,#23091,#23092,#23093,
#23094,#23095,#23096,#23097,#23098,#23099,#23100,#23101,#23102,#23103,#23104,
#23105,#23106,#23107,#23108,#23109,#23110,#23111,#23112,#23113,#23114,#23115,
#23116,#23117,#23118,#23119,#23120,#23121,#23122,#23123,#23124,#23125,#23126,
#23127,#23128,#23129,#23130,#23131,#23132,#23133,#23134,#23135,#23136,#23137,
#23138,#23139,#23140,#23141,#23142,#23143,#23144,#23145,#23146,#23147,#23148,
#23149,#23150,#23151,#23152,#23153,#23154,#23155,#23156,#23157,#23158,#23159,
#23160,#23161,#23162,#23163,#23164,#23165,#23166,#23167,#23168,#23169,#23170,
#23171,#23172,#23173,#23174,#23175,#23176,#23177,#23178,#23179,#23180,#23181,
#23182,#23183,#23184,#23185,#23186,#23187,#23188,#23189,#23190,#23191,#23192,
#23193,#23194,#23195,#23196,#23197,#23198,#23199,#23200,#23201,#23202,#23203,
#23204,#23205,#23206,#23207,#23208,#23209,#23210,#23211,#23212,#23213,#23214,
#23215,#23216,#23217,#23218,#23219,#23220,#23221,#23222,#23223,#23224,#23225,
#23226,#23227,#23228),.UNSPECIFIED.,.F.,.F.,(4,3,3,3,3,3,3,3,3,3,3,3,3,
3,3,3,3,3,3,3,3,3,3,3,3,3,3,3,3,3,3,3,3,3,3,3,3,3,3,3,3,3,3,3,3,3,3,3,3,
3,4),(53.4070751110264,53.5488498236995,53.6381223040877,53.7439426673302,
53.8496026361662,53.9551376190527,54.0606061171701,54.1660446288859,54.2714896077376,
54.3770477039605,54.4826696481002,54.5884747927751,54.6373030663835,54.743123429626,
54.8487833984619,54.9543183813483,55.0597868794657,55.1652253911815,55.2706703700334,
55.3762284662562,55.481850410396,55.5876555550709,55.6364838286793,55.7423041919218,
55.8479641607577,55.9534991436442,56.0589676417616,56.1644061534774,56.2698511323292,
56.3754092285521,56.4810311726919,56.5868363173668,56.6356645909751,56.7414849542176,
56.8471449230535,56.95267990594,57.0581484040574,57.1635869157733,57.2690318946251,
57.374589990848,57.4802119349878,57.5860170796627,57.6348453532709,57.7406331779413,
57.8462753337061,57.9518085486852,58.0572694189163,58.1627286964347,58.2681840438519,
58.3737305088498,58.438333049783),.UNSPECIFIED.);
#1165=B_SPLINE_CURVE_WITH_KNOTS('',3,(#23233,#23234,#23235,#23236,#23237,
#23238,#23239,#23240,#23241,#23242,#23243,#23244,#23245,#23246,#23247,#23248,
#23249,#23250,#23251,#23252,#23253,#23254,#23255,#23256,#23257,#23258,#23259,
#23260,#23261,#23262,#23263,#23264,#23265,#23266,#23267,#23268,#23269,#23270,
#23271,#23272,#23273,#23274,#23275,#23276,#23277,#23278,#23279,#23280,#23281,
#23282,#23283,#23284,#23285,#23286,#23287,#23288,#23289,#23290,#23291,#23292,
#23293,#23294,#23295,#23296,#23297,#23298,#23299,#23300,#23301,#23302,#23303,
#23304,#23305,#23306,#23307,#23308,#23309,#23310,#23311,#23312,#23313,#23314,
#23315,#23316,#23317,#23318,#23319,#23320,#23321,#23322,#23323,#23324,#23325,
#23326,#23327,#23328,#23329,#23330,#23331,#23332,#23333,#23334,#23335,#23336,
#23337,#23338,#23339,#23340,#23341,#23342,#23343,#23344,#23345,#23346,#23347,
#23348,#23349,#23350,#23351,#23352,#23353,#23354,#23355,#23356,#23357,#23358,
#23359,#23360,#23361,#23362,#23363,#23364,#23365,#23366,#23367,#23368,#23369,
#23370,#23371,#23372,#23373,#23374,#23375,#23376,#23377,#23378,#23379,#23380,
#23381,#23382,#23383,#23384,#23385,#23386,#23387,#23388,#23389,#23390,#23391,
#23392,#23393,#23394,#23395,#23396,#23397,#23398,#23399,#23400,#23401,#23402,
#23403,#23404,#23405,#23406,#23407,#23408,#23409,#23410,#23411,#23412,#23413,
#23414,#23415,#23416,#23417,#23418,#23419,#23420,#23421,#23422,#23423,#23424,
#23425,#23426,#23427,#23428,#23429,#23430,#23431,#23432,#23433,#23434,#23435,
#23436,#23437,#23438),.UNSPECIFIED.,.F.,.F.,(4,2,2,2,2,2,2,2,2,2,2,2,2,
2,2,2,2,2,2,2,2,2,2,2,2,2,2,2,2,2,2,2,2,2,2,2,2,2,2,2,2,2,2,2,2,2,2,2,2,
2,2,2,2,2,2,2,2,2,2,2,2,2,2,2,2,2,2,2,2,2,2,2,2,2,2,2,2,2,2,2,2,2,2,2,2,
2,2,2,2,2,2,2,2,2,2,2,2,2,2,2,2,2,4),(-2.189001750981,-2.14225794250904,
-2.11149306444298,-2.10767380722915,-2.10579262300464,-2.10444175848357,
-2.10270521951084,-2.09966569351592,-2.08662571360936,-2.08131111737203,
-2.07758280351107,-2.04317976059327,-2.01775494815292,-2.01246798904254,
-2.00941961035485,-2.00675424740815,-2.00344439262422,-1.99831751517754,
-1.96506045065472,-1.92186946920969,-1.91553026636808,-1.91322909264721,
-1.9116718380376,-1.9102661305893,-1.90832535526835,-1.90337380772395,-1.8725717084742,
-1.84020013229762,-1.82343242970201,-1.81873147053482,-1.81581056814682,
-1.8131195384669,-1.80964327519445,-1.80203615956091,-1.76150922799894,
-1.73919681621692,-1.72890645338217,-1.72238784261669,-1.72006195559318,
-1.71849959533238,-1.71709832776201,-1.71517512064348,-1.71032859246593,
-1.67550056100348,-1.63295953315827,-1.62672164201925,-1.62347278327525,
-1.62081112223071,-1.61771606136226,-1.6123588178702,-1.58798198472502,
-1.54976824761276,-1.53091804545937,-1.52767917739744,-1.5259175089066,
-1.52441933182097,-1.52249195669889,-1.51935603948711,-1.49646617107584,
-1.46899890230181,-1.4411879861954,-1.43406339052084,-1.43063938873421,
-1.4279628061315,-1.42498582254446,-1.42002804972072,-1.40262899828603,
-1.36290024948229,-1.34584224522774,-1.33662599841886,-1.33398803534395,
-1.33235780167674,-1.33083974129108,-1.32900280833424,-1.32433863369126,
-1.28428918802367,-1.27846229687321,-1.25063430291216,-1.24170277689903,
-1.23795922699513,-1.23523472839415,-1.2323911005675,-1.22804851800325,
-1.21589747069481,-1.19601363549382,-1.15347748098336,-1.14371425460895,
-1.1409151249908,-1.13924915491815,-1.13772948436155,-1.13563157467613,
-1.13062475074033,-1.1234308251802,-1.10157858815624,-1.05486202190455,
-1.04765304364835,-1.0442129006471,-1.04153428988957,-1.03856586990926,
-1.03364785696611,-1.01424781010532,-0.991532890587958,-0.973989629254837),
 .UNSPECIFIED.);
#1166=B_SPLINE_CURVE_WITH_KNOTS('',3,(#23440,#23441,#23442,#23443,#23444,
#23445,#23446,#23447,#23448,#23449,#23450,#23451,#23452,#23453,#23454,#23455,
#23456,#23457,#23458,#23459,#23460,#23461,#23462,#23463,#23464,#23465,#23466,
#23467,#23468,#23469,#23470,#23471,#23472,#23473,#23474,#23475,#23476,#23477,
#23478,#23479),.UNSPECIFIED.,.F.,.F.,(4,3,3,3,3,3,3,3,3,3,3,3,3,4),(58.438333049783,
58.5441224300846,58.6340261155667,58.7398464788092,58.8455064476451,58.9510414305316,
59.0565099286489,59.1619484403647,59.2673934192164,59.3729515154392,59.478573459579,
59.5843786042538,59.6332068778625,59.6902604182061),.UNSPECIFIED.);
#1167=B_SPLINE_CURVE_WITH_KNOTS('',3,(#23480,#23481,#23482,#23483,#23484,
#23485,#23486,#23487,#23488),.UNSPECIFIED.,.F.,.F.,(4,1,1,1,1,1,4),(59.6902673029908,
60.6323876401583,61.6315684024541,62.6307491647499,63.6299299270457,64.6291106893415,
64.7226639182745),.UNSPECIFIED.);
#1168=B_SPLINE_CURVE_WITH_KNOTS('',3,(#23494,#23495,#23496,#23497,#23498,
#23499,#23500,#23501,#23502),.UNSPECIFIED.,.F.,.F.,(4,1,1,1,1,1,4),(65.9734520027693,
66.2860804764019,67.2852612386977,68.2844420009935,69.2836227632893,70.2828035255851,
71.0044067958708),.UNSPECIFIED.);
#1169=B_SPLINE_CURVE_WITH_KNOTS('',3,(#23503,#23504,#23505,#23506,#23507,
#23508,#23509,#23510,#23511,#23512,#23513,#23514,#23515,#23516,#23517,#23518,
#23519,#23520,#23521,#23522,#23523,#23524,#23525,#23526,#23527,#23528,#23529,
#23530,#23531,#23532,#23533,#23534,#23535,#23536,#23537,#23538,#23539,#23540,
#23541,#23542,#23543,#23544,#23545,#23546,#23547,#23548,#23549,#23550,#23551,
#23552,#23553,#23554,#23555,#23556,#23557,#23558,#23559,#23560,#23561,#23562,
#23563,#23564,#23565,#23566,#23567,#23568,#23569,#23570,#23571,#23572,#23573,
#23574,#23575,#23576,#23577,#23578,#23579,#23580,#23581,#23582,#23583,#23584,
#23585,#23586,#23587,#23588,#23589,#23590,#23591,#23592,#23593,#23594,#23595,
#23596,#23597,#23598,#23599,#23600,#23601,#23602,#23603,#23604,#23605,#23606,
#23607,#23608,#23609,#23610),.UNSPECIFIED.,.F.,.F.,(4,2,2,2,2,2,2,2,2,2,
2,2,2,2,2,2,2,2,2,2,2,2,2,2,2,2,2,2,2,2,2,2,2,2,2,2,2,2,2,2,2,2,2,2,2,2,
2,2,2,2,2,2,2,4),(-2.43103019217924,-2.41217091518336,-2.40266616406287,
-2.39929537754217,-2.39668852902964,-2.39400774005481,-2.39105235808666,
-2.3861918764179,-2.3695930752094,-2.35000957128429,-2.30999805620414,-2.3048060717791,
-2.30090625589495,-2.29900927956527,-2.2976568206229,-2.29593167669591,
-2.29294169404183,-2.28060525376839,-2.27405386106923,-2.2428478186499,
-2.22185086546765,-2.21326197753705,-2.20666897445879,-2.2034488225326,
-2.20343115831572,-2.20341246364597,-2.20339267491428,-2.20337172420637,
-2.20334953900008,-2.20332604187673,-2.20330114998533,-2.20327477463628,
-2.20324682097543,-2.20321718749107,-2.20318576532779,-2.20315243785984,
-2.20311707992428,-2.20307955727866,-2.20303972585846,-2.20299743086428,
-2.2029525060551,-2.20290477272776,-2.20285403884808,-2.20280009795184,
-2.20274272813671,-2.20268169089799,-2.20263697406887,-2.20257699048357,
-2.20249652378171,-2.202388585695,-2.19971090533018,-2.19627453084266,-2.18908317483088,
-2.189001750981),.UNSPECIFIED.);
#1170=B_SPLINE_CURVE_WITH_KNOTS('',3,(#23612,#23613,#23614,#23615,#23616),
 .UNSPECIFIED.,.F.,.F.,(4,1,4),(64.7226639182745,65.6282914516373,65.9734383180058),
 .UNSPECIFIED.);
#1171=B_SPLINE_CURVE_WITH_KNOTS('',3,(#23617,#23618,#23619,#23620,#23621,
#23622,#23623,#23624,#23625,#23626,#23627,#23628,#23629,#23630,#23631,#23632,
#23633,#23634,#23635,#23636,#23637,#23638,#23639,#23640,#23641,#23642,#23643,
#23644,#23645,#23646,#23647,#23648,#23649,#23650,#23651,#23652,#23653,#23654,
#23655,#23656,#23657,#23658,#23659,#23660,#23661,#23662,#23663,#23664,#23665,
#23666,#23667,#23668,#23669,#23670,#23671,#23672,#23673,#23674,#23675,#23676,
#23677,#23678,#23679,#23680,#23681,#23682,#23683,#23684,#23685,#23686,#23687,
#23688,#23689,#23690,#23691,#23692,#23693,#23694,#23695,#23696,#23697,#23698,
#23699,#23700,#23701,#23702,#23703,#23704,#23705,#23706,#23707,#23708,#23709,
#23710,#23711,#23712,#23713,#23714,#23715,#23716,#23717,#23718,#23719,#23720,
#23721,#23722,#23723,#23724,#23725,#23726,#23727,#23728,#23729,#23730,#23731,
#23732,#23733,#23734,#23735,#23736,#23737,#23738,#23739,#23740,#23741,#23742,
#23743,#23744,#23745,#23746,#23747,#23748,#23749,#23750,#23751,#23752,#23753,
#23754,#23755,#23756,#23757,#23758,#23759,#23760,#23761,#23762,#23763,#23764,
#23765,#23766,#23767,#23768,#23769,#23770,#23771,#23772,#23773,#23774,#23775,
#23776,#23777,#23778,#23779,#23780,#23781,#23782,#23783,#23784,#23785,#23786,
#23787,#23788,#23789,#23790,#23791,#23792),.UNSPECIFIED.,.F.,.F.,(4,2,2,
2,2,2,2,2,2,2,2,2,2,2,2,2,2,2,2,2,2,2,2,2,2,2,2,2,2,2,2,2,2,2,2,2,2,2,2,
2,2,2,2,2,2,2,2,2,2,2,2,2,2,2,2,2,2,2,2,2,2,2,2,2,2,2,2,2,2,2,2,2,2,2,2,
2,2,2,2,2,2,2,2,2,2,2,2,4),(-2.43122156991905,-2.41740188853736,-2.4093327733779,
-2.40590964227835,-2.4032856118482,-2.40072669449692,-2.39783687629169,
-2.39327630227369,-2.37938394661034,-2.35744382917557,-2.31469050536173,
-2.30837579829069,-2.30607838843393,-2.30452217671395,-2.30311624872971,
-2.30117371357907,-2.29621020343292,-2.26662662311645,-2.24085266165562,
-2.2252094959536,-2.21813981860739,-2.21405477499885,-2.21042245807682,
-2.20774918356246,-2.20524828129091,-2.20121608808074,-2.19118114876341,
-2.14506180475598,-2.1409661220333,-2.11722528897416,-2.11384007303311,
-2.11204760675826,-2.11055229022504,-2.10866537196592,-2.10566413752689,
-2.08818712863389,-2.07437502791,-2.04036593179245,-2.02314655945143,-2.01840598438993,
-2.01547675198109,-2.01278887666726,-2.00933181003124,-2.00182875647805,
-1.95885090316993,-1.94832763199638,-1.92402418771038,-1.92062621899117,
-1.91883102801624,-1.9173357913925,-1.91545194236067,-1.91246104236256,
-1.89524555958718,-1.88160975532147,-1.84724874496579,-1.82993540816725,
-1.82518651326017,-1.82225538142978,-1.81956790872277,-1.81611434207564,
-1.80863100464044,-1.76528520350111,-1.73176870790186,-1.72775452305202,
-1.72583522224988,-1.72433776182905,-1.7225704142123,-1.71939490784715,
-1.70412150133219,-1.65262819098408,-1.64188440756512,-1.63398231757764,
-1.63041523817908,-1.62771998166277,-1.62481325919949,-1.6201762290837,
-1.60563418704462,-1.55868324364107,-1.5441942441099,-1.53863120870868,
-1.53451720653437,-1.53257881871942,-1.53109340826038,-1.5293454572945,
-1.52625567310631,-1.51247154949388,-1.47891218751976,-1.45794880066605),
 .UNSPECIFIED.);
#1172=B_SPLINE_CURVE_WITH_KNOTS('',3,(#23798,#23799,#23800,#23801,#23802,
#23803,#23804,#23805,#23806,#23807,#23808,#23809,#23810,#23811,#23812,#23813,
#23814,#23815,#23816,#23817,#23818,#23819,#23820,#23821,#23822,#23823,#23824,
#23825,#23826,#23827,#23828,#23829,#23830,#23831,#23832,#23833,#23834,#23835,
#23836,#23837,#23838,#23839,#23840,#23841,#23842,#23843,#23844,#23845,#23846,
#23847,#23848,#23849,#23850,#23851,#23852,#23853,#23854,#23855,#23856,#23857,
#23858,#23859,#23860,#23861,#23862,#23863,#23864,#23865,#23866,#23867,#23868,
#23869,#23870,#23871,#23872,#23873,#23874,#23875,#23876,#23877,#23878,#23879,
#23880,#23881,#23882,#23883,#23884,#23885,#23886,#23887,#23888,#23889,#23890,
#23891,#23892,#23893,#23894,#23895,#23896,#23897,#23898,#23899,#23900,#23901,
#23902,#23903,#23904,#23905,#23906,#23907,#23908,#23909,#23910,#23911,#23912,
#23913,#23914,#23915,#23916,#23917,#23918,#23919,#23920,#23921,#23922,#23923,
#23924,#23925,#23926,#23927,#23928,#23929,#23930,#23931,#23932,#23933,#23934,
#23935,#23936,#23937,#23938,#23939,#23940,#23941,#23942,#23943,#23944,#23945,
#23946,#23947,#23948,#23949,#23950,#23951,#23952,#23953,#23954),
 .UNSPECIFIED.,.F.,.F.,(4,3,3,3,3,3,3,3,3,3,3,3,3,3,3,3,3,3,3,3,3,3,3,3,
3,3,3,3,3,3,3,3,3,3,3,3,3,3,3,3,3,3,3,3,3,3,3,3,3,3,3,3,4),(72.2566310325652,
72.2811650501767,72.3869854134193,72.4926453822552,72.5981803651418,72.7036488632592,
72.809087374975,72.9145323538269,73.0200904500499,73.1257123941897,73.2315175388647,
73.2803458124725,73.386166175715,73.4918261445509,73.5973611274374,73.7028296255547,
73.8082681372705,73.9137131161223,74.0192712123451,74.1248931564849,74.2306983011597,
74.2795265747683,74.3853469380109,74.4910069068467,74.5965418897333,74.7020103878507,
74.8074488995665,74.9128938784183,75.0184519746412,75.124073918781,75.2298790634559,
75.2787073370641,75.3845277003066,75.4901876691425,75.595722652029,75.7011911501463,
75.8066296618621,75.9120746407139,76.0176327369367,76.1232546810765,76.2290598257514,
76.2778880993599,76.3837084626024,76.4893684314383,76.5949034143247,76.7003719124421,
76.8058104241579,76.9112554030097,77.0168134992326,77.1224354433723,77.2282405880472,
77.2770688616556,77.2885547891013),.UNSPECIFIED.);
#1173=B_SPLINE_CURVE_WITH_KNOTS('',3,(#23955,#23956,#23957,#23958,#23959),
 .UNSPECIFIED.,.F.,.F.,(4,1,4),(71.0044067958708,71.2819842878809,72.256627539715),
 .UNSPECIFIED.);
#1174=B_SPLINE_CURVE_WITH_KNOTS('',3,(#23960,#23961,#23962,#23963,#23964,
#23965,#23966,#23967,#23968,#23969,#23970,#23971,#23972,#23973,#23974,#23975,
#23976,#23977,#23978,#23979,#23980,#23981,#23982,#23983,#23984,#23985,#23986,
#23987,#23988,#23989,#23990,#23991,#23992,#23993,#23994,#23995,#23996,#23997,
#23998,#23999,#24000,#24001,#24002,#24003,#24004,#24005,#24006,#24007,#24008,
#24009,#24010,#24011,#24012,#24013,#24014,#24015,#24016,#24017,#24018,#24019,
#24020,#24021,#24022,#24023,#24024,#24025,#24026,#24027,#24028,#24029,#24030,
#24031,#24032,#24033,#24034,#24035,#24036,#24037,#24038,#24039,#24040,#24041,
#24042,#24043,#24044,#24045,#24046,#24047,#24048,#24049,#24050,#24051,#24052,
#24053,#24054,#24055,#24056,#24057,#24058,#24059,#24060,#24061,#24062,#24063,
#24064,#24065,#24066,#24067,#24068,#24069,#24070,#24071,#24072,#24073,#24074,
#24075,#24076,#24077,#24078,#24079,#24080,#24081,#24082,#24083,#24084,#24085,
#24086,#24087,#24088,#24089,#24090,#24091,#24092,#24093,#24094,#24095,#24096,
#24097,#24098,#24099,#24100,#24101,#24102,#24103,#24104,#24105,#24106,#24107,
#24108,#24109,#24110,#24111,#24112,#24113,#24114,#24115,#24116,#24117,#24118,
#24119,#24120,#24121,#24122,#24123,#24124,#24125,#24126,#24127,#24128,#24129,
#24130,#24131,#24132,#24133,#24134,#24135,#24136,#24137,#24138,#24139,#24140,
#24141,#24142,#24143,#24144,#24145,#24146,#24147,#24148,#24149,#24150,#24151,
#24152,#24153,#24154,#24155,#24156,#24157,#24158,#24159,#24160,#24161,#24162,
#24163,#24164,#24165,#24166,#24167,#24168,#24169,#24170,#24171,#24172,#24173,
#24174,#24175,#24176,#24177,#24178,#24179,#24180,#24181),.UNSPECIFIED.,
 .F.,.F.,(4,2,2,2,2,2,2,2,2,2,2,2,2,2,2,2,2,2,2,2,2,2,2,2,2,2,2,2,2,2,2,
2,2,2,2,2,2,2,2,2,2,2,2,2,2,2,2,2,2,2,2,2,2,2,2,2,2,2,2,2,2,2,2,2,2,2,2,
2,2,2,2,2,2,2,2,2,2,2,2,2,2,2,2,2,2,2,2,2,2,2,2,2,2,2,2,2,2,2,2,2,2,2,2,
2,2,2,2,2,2,2,4),(-1.45794880066605,-1.44624583571765,-1.43988442584939,
-1.43661057713039,-1.43394773679398,-1.43087290480914,-1.42560445174949,
-1.40283074358948,-1.36365295036055,-1.35037177699628,-1.3451186259298,
-1.34118311006444,-1.33927907839669,-1.33792574755609,-1.33620524424236,
-1.33323582115914,-1.32117645524588,-1.31414670900283,-1.28263613648096,
-1.25432591061907,-1.24713909071555,-1.24370345531477,-1.24102573820999,
-1.23805564787756,-1.23312863735979,-1.21583347700753,-1.18497150596766,
-1.15355369204604,-1.14860798580015,-1.14666826839542,-1.1452628842504,
-1.14370546287263,-1.14140320700633,-1.13505565425296,-1.09171147953475,
-1.05863054385238,-1.05350572852608,-1.05019650976018,-1.04753124311002,
-1.04448253104394,-1.03919389959753,-1.01374196838361,-0.979244378436831,
-0.968515689473857,-0.956998261618626,-0.954042680044054,-0.952342440646011,
-0.950833670468636,-0.948807974718877,-0.944218910033777,-0.923529693423371,
-0.887367842065201,-0.864747161548468,-0.859487633063125,-0.856414765503111,
-0.853751675864774,-0.850475033727133,-0.844100159448475,-0.835953623514413,
-0.816602813065972,-0.781181109754996,-0.77816482347728,-0.76410347150806,
-0.760998252123578,-0.759246768097607,-0.757747476756573,-0.755806015301985,
-0.751676037795849,-0.746085610191573,-0.731488182406631,-0.682244381522221,
-0.669687503721353,-0.665292923386707,-0.662438501485609,-0.659720558330306,
-0.656012876785706,-0.647296464341834,-0.618761573177164,-0.586297399801915,
-0.570972098293276,-0.567793724762032,-0.566025764400172,-0.564528403530472,
-0.562610041717839,-0.55860056303628,-0.553220146140338,-0.539449872453238,
-0.498283151384905,-0.477975133994351,-0.47280529456626,-0.469782366597916,
-0.46738088870423,-0.464160365097725,-0.458059881052783,-0.418238394251748,
-0.38016866975499,-0.375480296488304,-0.37358407013704,-0.372051004934755,
-0.370446495475348,-0.367924749888287,-0.359816415676196,-0.345759603294467,
-0.302983491661031,-0.284454747495694,-0.279418354307256,-0.276424414403936,
-0.274018760713709,-0.270757045763547,-0.264455664153103,-0.242747535804741),
 .UNSPECIFIED.);
#1175=B_SPLINE_CURVE_WITH_KNOTS('',3,(#24187,#24188,#24189,#24190,#24191,
#24192,#24193,#24194,#24195,#24196,#24197,#24198,#24199,#24200,#24201,#24202,
#24203,#24204,#24205,#24206,#24207,#24208,#24209,#24210,#24211,#24212,#24213,
#24214,#24215,#24216,#24217,#24218,#24219,#24220,#24221,#24222,#24223,#24224,
#24225,#24226,#24227,#24228,#24229,#24230,#24231,#24232,#24233,#24234,#24235,
#24236,#24237,#24238,#24239,#24240,#24241,#24242,#24243,#24244,#24245,#24246,
#24247,#24248,#24249,#24250,#24251,#24252,#24253,#24254,#24255,#24256,#24257,
#24258,#24259,#24260,#24261,#24262,#24263,#24264,#24265,#24266,#24267,#24268,
#24269,#24270,#24271,#24272,#24273,#24274,#24275,#24276,#24277,#24278,#24279,
#24280,#24281,#24282,#24283,#24284,#24285,#24286,#24287,#24288,#24289,#24290,
#24291,#24292,#24293,#24294,#24295,#24296,#24297,#24298,#24299,#24300,#24301,
#24302,#24303,#24304,#24305,#24306,#24307,#24308,#24309,#24310,#24311,#24312,
#24313,#24314,#24315,#24316,#24317,#24318,#24319,#24320,#24321,#24322,#24323,
#24324,#24325,#24326,#24327,#24328,#24329,#24330,#24331,#24332,#24333,#24334,
#24335,#24336,#24337,#24338,#24339,#24340,#24341,#24342,#24343,#24344,#24345,
#24346,#24347,#24348,#24349,#24350,#24351,#24352,#24353,#24354,#24355,#24356,
#24357,#24358,#24359,#24360),.UNSPECIFIED.,.F.,.F.,(4,2,2,2,2,2,2,2,2,2,
2,2,2,2,2,2,2,2,2,2,2,2,2,2,2,2,2,2,2,2,2,2,2,2,2,2,2,2,2,2,2,2,2,2,2,2,
2,2,2,2,2,2,2,2,2,2,2,2,2,2,2,2,2,2,2,2,2,2,2,2,2,2,2,2,2,2,2,2,2,2,2,2,
2,2,2,2,4),(-0.973882930196809,-0.944219937250399,-0.921904536119179,-0.918777710195008,
-0.91685282360926,-0.915354543274545,-0.913590344154815,-0.91034076376922,
-0.891213882423294,-0.852451212595539,-0.844176821288675,-0.827850967344199,
-0.823016528795024,-0.820066095282667,-0.81738273765496,-0.813906840357539,
-0.806508943917871,-0.776464141743833,-0.76839603253496,-0.730722904709127,
-0.726018052964024,-0.724118672175214,-0.722584467970821,-0.72098046981968,
-0.718462445648489,-0.71039140922058,-0.696431000629615,-0.654238625258667,
-0.635090389733211,-0.629998336572393,-0.626991719434676,-0.624587153286583,
-0.621341639154425,-0.615122516984872,-0.60722902830931,-0.588787258900323,
-0.562682126076683,-0.535520250092716,-0.532346444750821,-0.530407652113421,
-0.5289082615078,-0.527154085472223,-0.52395125884013,-0.50602312727782,
-0.479496203386512,-0.442948143474137,-0.437823682432759,-0.434514084214073,
-0.431848104869673,-0.42879812173562,-0.423506074937283,-0.398004075686,
-0.363228067327037,-0.352443867188458,-0.341265491734738,-0.338338188761974,
-0.33664385964487,-0.33513298368972,-0.333094430513295,-0.32843449508106,
-0.307084319225128,-0.276704102858013,-0.249475516282498,-0.243993774060742,
-0.240870156261451,-0.238234585146884,-0.235028725449389,-0.229158204643075,
-0.221721078250796,-0.204858344090895,-0.164049181648068,-0.148561766286696,
-0.145373992918243,-0.143603540342072,-0.142105807475087,-0.14018915712708,
-0.136376403077181,-0.105253522109437,-0.0818081601489447,-0.056113797427619,
-0.050699364712091,-0.0475907848367115,-0.0449544151876206,-0.0417309778911177,
-0.038301942588913,-0.0328593950830175,-0.000573591561804652),
 .UNSPECIFIED.);
#1176=B_SPLINE_CURVE_WITH_KNOTS('',3,(#24361,#24362,#24363,#24364,#24365,
#24366,#24367,#24368,#24369,#24370,#24371,#24372,#24373,#24374,#24375,#24376,
#24377,#24378,#24379,#24380,#24381,#24382,#24383,#24384,#24385,#24386,#24387,
#24388,#24389,#24390,#24391,#24392,#24393,#24394,#24395,#24396,#24397),
 .UNSPECIFIED.,.F.,.F.,(4,3,3,3,3,3,3,3,3,3,3,3,4),(77.2885547891013,77.3943557879778,
77.5045925174745,77.6101150423719,77.7155766333603,77.8210137795483,77.9264629309739,
78.0320286129095,78.1376631195039,78.2434760803445,78.2762496239514,78.4105186845177,
78.5398163394612),.UNSPECIFIED.);
#1177=B_SPLINE_CURVE_WITH_KNOTS('',3,(#24399,#24400,#24401,#24402,#24403,
#24404,#24405,#24406,#24407,#24408,#24409,#24410,#24411,#24412,#24413,#24414,
#24415,#24416,#24417,#24418,#24419,#24420,#24421,#24422,#24423,#24424,#24425,
#24426,#24427,#24428,#24429,#24430,#24431,#24432,#24433,#24434,#24435,#24436),
 .UNSPECIFIED.,.F.,.F.,(4,2,2,2,2,2,2,2,2,2,2,2,2,2,2,2,2,2,4),(-0.242747535804741,
-0.223836868626812,-0.186992156459622,-0.18223779622474,-0.180330219392406,
-0.178932872265027,-0.177397228214326,-0.175215061136868,-0.172619024178979,
-0.167839411107292,-0.119303502477546,-0.0920807826407651,-0.0866003096148791,
-0.0834775358710877,-0.0808427586427267,-0.0776379762208395,-0.0716139334229604,
-0.0340705181892316,-0.000574328313784234),.UNSPECIFIED.);
#1178=B_SPLINE_CURVE_WITH_KNOTS('',3,(#24437,#24438,#24439,#24440,#24441,
#24442,#24443,#24444,#24445,#24446,#24447,#24448,#24449,#24450,#24451,#24452,
#24453,#24454,#24455,#24456,#24457,#24458,#24459,#24460,#24461,#24462,#24463,
#24464,#24465,#24466,#24467,#24468,#24469,#24470,#24471,#24472,#24473,#24474,
#24475,#24476,#24477,#24478,#24479,#24480,#24481,#24482,#24483,#24484,#24485,
#24486,#24487,#24488,#24489,#24490,#24491,#24492,#24493,#24494,#24495,#24496,
#24497,#24498,#24499,#24500,#24501,#24502,#24503,#24504,#24505,#24506,#24507,
#24508,#24509,#24510,#24511,#24512,#24513,#24514,#24515,#24516,#24517,#24518,
#24519,#24520,#24521,#24522,#24523,#24524,#24525,#24526,#24527,#24528,#24529,
#24530,#24531,#24532,#24533,#24534,#24535,#24536,#24537,#24538,#24539,#24540,
#24541,#24542,#24543,#24544,#24545,#24546,#24547,#24548,#24549,#24550,#24551,
#24552,#24553,#24554,#24555,#24556,#24557,#24558,#24559,#24560,#24561,#24562,
#24563,#24564,#24565,#24566,#24567,#24568,#24569,#24570,#24571,#24572,#24573,
#24574,#24575,#24576,#24577,#24578,#24579,#24580,#24581,#24582,#24583,#24584,
#24585,#24586,#24587,#24588,#24589,#24590,#24591,#24592,#24593,#24594,#24595,
#24596,#24597,#24598,#24599,#24600,#24601,#24602,#24603,#24604,#24605,#24606),
 .UNSPECIFIED.,.F.,.F.,(4,2,2,2,2,2,2,2,2,2,2,2,2,2,2,2,2,2,2,2,2,2,2,2,
2,2,2,2,2,2,2,2,2,2,2,2,2,2,2,2,2,2,2,2,2,2,2,2,2,2,2,2,2,2,2,2,2,2,2,2,
2,2,2,2,2,2,2,2,2,2,2,2,2,2,2,2,2,2,2,2,2,2,2,2,4),(-2.43107777278142,-2.4216364324254,
-2.41932244202859,-2.41770638159793,-2.41630998116545,-2.41479108515786,
-2.41294963960475,-2.40825520827373,-2.39630263645416,-2.36157565826851,
-2.32934693264584,-2.32379892703653,-2.32069466021498,-2.31830074764382,
-2.31517746502707,-2.30969365184746,-2.28238376064854,-2.23386733437854,
-2.22910969561732,-2.22652207082348,-2.22429890510821,-2.22277261991302,
-2.22136752681913,-2.21942880521082,-2.21448858493093,-2.18328521629785,
-2.15118763940105,-2.13449740174692,-2.12980367821092,-2.12688453840775,
-2.12419331191462,-2.12071424852467,-2.11309053295057,-2.07304840388646,
-2.05038849796661,-2.0400160823175,-2.03346018588833,-2.03112937133336,
-2.02956609366946,-2.02816588101134,-2.02624651462117,-2.02142215583497,
-1.9859760447991,-1.94399983033855,-1.93776351499308,-1.93451516597527,
-1.93185378161207,-1.92875889438622,-1.92340161419112,-1.89913200765131,
-1.8608297152583,-1.84194398007218,-1.83870393329097,-1.83694211661892,
-1.83544413256886,-1.83351745958127,-1.83038358874895,-1.80760884713865,
-1.77428789038115,-1.74910774785104,-1.74383285866949,-1.74078712610847,
-1.73812154444079,-1.73480813158663,-1.72966942538366,-1.6956762828095,
-1.65316954903024,-1.64686762612116,-1.64457168082692,-1.64301551906721,
-1.64160889423659,-1.63966444876635,-1.63469108009369,-1.60523632508808,
-1.57299071051188,-1.56105717805104,-1.55249767501423,-1.54881615395698,
-1.54610247230968,-1.5435818490515,-1.54012025179612,-1.53123501631135,
-1.48392839280664,-1.46447905982084,-1.45793772452377),.UNSPECIFIED.);
#1179=B_SPLINE_CURVE_WITH_KNOTS('',3,(#24611,#24612,#24613,#24614,#24615,
#24616,#24617,#24618,#24619,#24620,#24621,#24622,#24623,#24624,#24625,#24626,
#24627,#24628,#24629,#24630,#24631,#24632,#24633,#24634,#24635,#24636,#24637,
#24638,#24639,#24640,#24641,#24642,#24643,#24644,#24645,#24646,#24647,#24648,
#24649,#24650,#24651,#24652,#24653,#24654,#24655,#24656,#24657,#24658,#24659,
#24660,#24661,#24662,#24663,#24664,#24665,#24666,#24667,#24668,#24669,#24670,
#24671,#24672,#24673,#24674,#24675,#24676,#24677,#24678,#24679,#24680,#24681,
#24682,#24683,#24684,#24685,#24686,#24687,#24688,#24689,#24690,#24691,#24692,
#24693,#24694,#24695,#24696,#24697,#24698,#24699,#24700,#24701,#24702,#24703,
#24704,#24705,#24706,#24707,#24708,#24709,#24710,#24711,#24712,#24713,#24714,
#24715,#24716,#24717,#24718,#24719,#24720,#24721,#24722,#24723,#24724,#24725,
#24726,#24727,#24728,#24729,#24730,#24731,#24732,#24733,#24734,#24735,#24736,
#24737,#24738,#24739,#24740,#24741,#24742,#24743,#24744,#24745,#24746,#24747,
#24748,#24749,#24750,#24751,#24752,#24753,#24754,#24755,#24756,#24757,#24758,
#24759,#24760,#24761,#24762,#24763,#24764,#24765,#24766,#24767,#24768,#24769,
#24770,#24771,#24772,#24773,#24774,#24775,#24776,#24777,#24778,#24779,#24780,
#24781,#24782,#24783,#24784,#24785,#24786,#24787,#24788,#24789,#24790,#24791,
#24792,#24793,#24794,#24795,#24796,#24797,#24798,#24799,#24800,#24801,#24802,
#24803,#24804,#24805,#24806,#24807,#24808,#24809,#24810,#24811,#24812,#24813,
#24814,#24815,#24816,#24817,#24818,#24819,#24820,#24821,#24822,#24823,#24824),
 .UNSPECIFIED.,.F.,.F.,(4,2,2,2,2,2,2,2,2,2,2,2,2,2,2,2,2,2,2,2,2,2,2,2,
2,2,2,2,2,2,2,2,2,2,2,2,2,2,2,2,2,2,2,2,2,2,2,2,2,2,2,2,2,2,2,2,2,2,2,2,
2,2,2,2,2,2,2,2,2,2,2,2,2,2,2,2,2,2,2,2,2,2,2,2,2,2,2,2,2,2,2,2,2,2,2,2,
2,2,2,2,2,2,2,2,2,2,4),(-2.18919381409884,-2.18542769624879,-2.1777550237912,
-2.17422858908373,-2.17153847469439,-2.16861237384775,-2.16388928441978,
-2.14857128267781,-2.10261070908038,-2.08809248688705,-2.08252165729276,
-2.07840294323425,-2.07646327995554,-2.07497731303468,-2.0732291679483,
-2.07014005085251,-2.05637759821995,-2.00342625063843,-1.98705445192856,
-1.98238917352435,-1.97947574326804,-1.976781691186,-1.97328752886651,-1.96586912773494,
-1.92308683471171,-1.89858077769942,-1.89089199082272,-1.88562898840809,
-1.88348891756278,-1.88196214043551,-1.88051843314864,-1.87800479452204,
-1.8706858724857,-1.82469417385007,-1.79784198361439,-1.79083888670194,
-1.78743792333612,-1.78476366425887,-1.78177299964344,-1.77675342853374,
-1.75845083450918,-1.71544045981571,-1.70134356018655,-1.69321996452482,
-1.690696145298,-1.68909095117362,-1.6875577429757,-1.68566187193951,-1.68097691931811,
-1.64285247617887,-1.6203412173297,-1.60103565878672,-1.59612451272635,
-1.5931573941776,-1.59047814195304,-1.58703463879686,-1.57980908547012,
-1.53320777337025,-1.51124999396228,-1.50403509618806,-1.49901756117681,
-1.49691771975033,-1.49539761352437,-1.49373219991273,-1.49093611821525,
-1.48120699232189,-1.43867198146836,-1.41141562442926,-1.40436056946333,
-1.40094950720844,-1.39827400401815,-1.39528888692692,-1.39029528082016,
-1.37249159492932,-1.32356413018792,-1.31296712999778,-1.30630927328946,
-1.30396422927291,-1.30239758477807,-1.30099910392051,-1.2990880372357,
-1.29431500741867,-1.25773782524663,-1.21592120741526,-1.21077910597509,
-1.20746409577167,-1.2047976176147,-1.2017512723742,-1.19647635650801,-1.1713220702832,
-1.13810540300183,-1.1151603057416,-1.11202252287472,-1.11009437201323,
-1.10859582331981,-1.10683397245524,-1.10359544058248,-1.08476539751549,
-1.04659329765605,-1.02217500090176,-1.01681715453497,-1.01372148048733,
-1.01105913531796,-1.00780924510266,-1.00156877734155,-0.977939243506538,
-0.973882930196809),.UNSPECIFIED.);
#1180=B_SPLINE_CURVE_WITH_KNOTS('',3,(#24825,#24826,#24827,#24828,#24829,
#24830,#24831,#24832,#24833,#24834,#24835,#24836,#24837,#24838,#24839,#24840,
#24841,#24842,#24843,#24844,#24845,#24846,#24847,#24848,#24849,#24850,#24851,
#24852,#24853,#24854,#24855,#24856,#24857,#24858,#24859,#24860,#24861,#24862,
#24863,#24864,#24865,#24866,#24867,#24868,#24869,#24870,#24871,#24872,#24873,
#24874,#24875,#24876,#24877,#24878,#24879,#24880,#24881,#24882,#24883,#24884,
#24885,#24886,#24887,#24888,#24889,#24890,#24891,#24892,#24893,#24894,#24895,
#24896,#24897,#24898,#24899,#24900,#24901,#24902,#24903,#24904,#24905,#24906,
#24907,#24908,#24909,#24910,#24911,#24912,#24913,#24914,#24915,#24916,#24917,
#24918,#24919,#24920,#24921,#24922,#24923,#24924,#24925,#24926,#24927,#24928,
#24929,#24930,#24931,#24932,#24933,#24934,#24935,#24936,#24937,#24938,#24939,
#24940,#24941,#24942,#24943,#24944,#24945,#24946,#24947,#24948,#24949,#24950,
#24951,#24952,#24953,#24954,#24955,#24956,#24957,#24958,#24959,#24960,#24961,
#24962,#24963,#24964,#24965,#24966,#24967,#24968,#24969,#24970,#24971,#24972,
#24973,#24974,#24975,#24976,#24977,#24978,#24979,#24980,#24981,#24982,#24983,
#24984,#24985,#24986,#24987,#24988,#24989,#24990,#24991,#24992,#24993,#24994,
#24995,#24996,#24997,#24998,#24999,#25000,#25001,#25002,#25003,#25004,#25005,
#25006,#25007,#25008,#25009,#25010,#25011,#25012,#25013,#25014,#25015,#25016,
#25017,#25018,#25019,#25020,#25021,#25022,#25023,#25024,#25025,#25026,#25027,
#25028,#25029,#25030,#25031,#25032,#25033,#25034,#25035,#25036,#25037,#25038,
#25039,#25040,#25041,#25042),.UNSPECIFIED.,.F.,.F.,(4,2,2,2,2,2,2,2,2,2,
2,2,2,2,2,2,2,2,2,2,2,2,2,2,2,2,2,2,2,2,2,2,2,2,2,2,2,2,2,2,2,2,2,2,2,2,
2,2,2,2,2,2,2,2,2,2,2,2,2,2,2,2,2,2,2,2,2,2,2,2,2,2,2,2,2,2,2,2,2,2,2,2,
2,2,2,2,2,2,2,2,2,2,2,2,2,2,2,2,2,2,2,2,2,2,2,2,2,2,4),(-1.45793772452377,
-1.45777260193418,-1.45302510647799,-1.45097148119764,-1.44945870609026,
-1.44777250859995,-1.44488130714998,-1.43410949080527,-1.42326776027908,
-1.38816492231145,-1.36261109191867,-1.35731728178986,-1.35426725838252,
-1.35160182549809,-1.34829367472127,-1.34317292084646,-1.31064906147403,
-1.26672852869036,-1.2603490701703,-1.25804216883641,-1.25648364598898,
-1.25507886058817,-1.25314201465082,-1.24821429570316,-1.21607450283724,
-1.17290643617366,-1.16541401843643,-1.16195846157678,-1.15927034153411,
-1.15633941416287,-1.15159290171079,-1.13431420204943,-1.10008974803179,
-1.08603721795572,-1.0689892503762,-1.06600454508107,-1.06412240731802,
-1.06262700769033,-1.0608297859991,-1.05742302373645,-1.03271633723126,
-1.03018026579809,-0.985573901999544,-0.974000860973215,-0.969739201323046,
-0.967195311141253,-0.964495470080255,-0.960900192787971,-0.952840943924294,
-0.941815908503195,-0.909944670525386,-0.878387172933484,-0.87344512441187,
-0.871505950686854,-0.8701006318668,-0.868542888226062,-0.866239485521736,
-0.85988450826816,-0.816409187166543,-0.783459588513825,-0.778335694898967,
-0.775026615041645,-0.77236116509105,-0.769311920914844,-0.764021535459174,
-0.738540521405353,-0.70389236572519,-0.693133871966376,-0.681793968046884,
-0.678853204095014,-0.677156130011352,-0.675646392456661,-0.673614280273694,
-0.668989536000823,-0.647968709999461,-0.637911410746544,-0.592909663164301,
-0.585541557029416,-0.582108903140882,-0.579424125852703,-0.576482132769866,
-0.571684385101919,-0.553801624567775,-0.52201272084882,-0.491855394997577,
-0.48690870579373,-0.484968752166898,-0.483563251706732,-0.482005767265275,
-0.47970352997016,-0.473356738445829,-0.430031118061,-0.396925879821879,
-0.391800519269523,-0.388491027004843,-0.385825590895464,-0.382776740491327,
-0.37748801206359,-0.352039160988258,-0.317564269844856,-0.306839703351112,
-0.295291557202058,-0.29233325901375,-0.290632359355875,-0.289123635477083,
-0.287098856002939,-0.282515369392134,-0.261879296234975,-0.242598015109206),
 .UNSPECIFIED.);
#1181=B_SPLINE_CURVE_WITH_KNOTS('',3,(#25048,#25049,#25050,#25051,#25052,
#25053,#25054,#25055,#25056,#25057,#25058,#25059,#25060,#25061,#25062,#25063,
#25064,#25065,#25066,#25067,#25068,#25069,#25070,#25071,#25072,#25073,#25074,
#25075,#25076,#25077,#25078,#25079,#25080,#25081,#25082,#25083,#25084,#25085,
#25086,#25087,#25088,#25089,#25090,#25091,#25092,#25093,#25094,#25095,#25096,
#25097,#25098,#25099,#25100,#25101,#25102,#25103,#25104,#25105,#25106,#25107,
#25108,#25109,#25110,#25111,#25112,#25113,#25114,#25115,#25116,#25117,#25118,
#25119,#25120,#25121,#25122,#25123,#25124,#25125,#25126,#25127,#25128,#25129,
#25130,#25131,#25132,#25133,#25134,#25135,#25136,#25137,#25138,#25139,#25140,
#25141,#25142,#25143,#25144,#25145,#25146,#25147,#25148,#25149,#25150,#25151,
#25152,#25153,#25154,#25155,#25156,#25157,#25158,#25159,#25160,#25161,#25162,
#25163,#25164,#25165,#25166,#25167,#25168,#25169,#25170,#25171,#25172,#25173,
#25174,#25175,#25176,#25177,#25178,#25179,#25180,#25181,#25182,#25183,#25184,
#25185,#25186,#25187,#25188,#25189,#25190,#25191,#25192,#25193,#25194,#25195,
#25196,#25197,#25198,#25199,#25200,#25201,#25202,#25203,#25204,#25205,#25206,
#25207,#25208,#25209,#25210,#25211,#25212,#25213,#25214,#25215,#25216,#25217,
#25218,#25219,#25220,#25221,#25222,#25223),.UNSPECIFIED.,.F.,.F.,(4,2,2,
2,2,2,2,2,2,2,2,2,2,2,2,2,2,2,2,2,2,2,2,2,2,2,2,2,2,2,2,2,2,2,2,2,2,2,2,
2,2,2,2,2,2,2,2,2,2,2,2,2,2,2,2,2,2,2,2,2,2,2,2,2,2,2,2,2,2,2,2,2,2,2,2,
2,2,2,2,2,2,2,2,2,2,2,2,4),(-0.973675603579949,-0.971516545702564,-0.930207628100764,
-0.910055662766931,-0.904894525557746,-0.901872638858196,-0.899469778060034,
-0.896244545073618,-0.890125455208344,-0.882393248108257,-0.864518822685786,
-0.822516491085122,-0.809555093950112,-0.806519786723747,-0.80478373302264,
-0.803432056024337,-0.801548231090491,-0.797718261896276,-0.766595679976655,
-0.720227631034037,-0.712980580123312,-0.709532686935743,-0.70685253418381,
-0.703886974766604,-0.698984401662838,-0.679800807313866,-0.639366388857412,
-0.616934035005804,-0.613804741691513,-0.611878969585161,-0.610380414445586,
-0.608616378284783,-0.605368329087662,-0.58629352483316,-0.547613866466647,
-0.523885721762268,-0.518563001989904,-0.515475006691077,-0.512811776446246,
-0.509551367970992,-0.50326068605035,-0.495251781037841,-0.476400612464549,
-0.453745058672016,-0.443404562924578,-0.423606817613433,-0.420522643710844,
-0.418610360662707,-0.417112853054904,-0.415338884977469,-0.412043920266098,
-0.391611772752849,-0.350030570565927,-0.330191463439554,-0.325051095962264,
-0.322033793843072,-0.31963044514499,-0.316399220770562,-0.310250665249883,
-0.302471048839356,-0.284430818090247,-0.261065134729581,-0.232835747709177,
-0.227898432150552,-0.225959748821636,-0.224554301354016,-0.222995809771584,
-0.22077740087351,-0.214805222085212,-0.205623932127911,-0.171239789863074,
-0.137946773011612,-0.13281829323107,-0.129507294688439,-0.126840960263971,
-0.123791414958773,-0.118502302402707,-0.093068436308353,-0.075759600010088,
-0.0561909817124832,-0.0370787145087763,-0.0340184316652335,-0.032113354409625,
-0.0306164029671963,-0.0291941361075527,-0.0274304870625983,-0.0247525085311,
-0.00057331623553469),.UNSPECIFIED.);
#1182=B_SPLINE_CURVE_WITH_KNOTS('',3,(#25224,#25225,#25226,#25227,#25228,
#25229,#25230,#25231,#25232,#25233,#25234,#25235,#25236,#25237,#25238,#25239,
#25240,#25241,#25242,#25243,#25244,#25245,#25246,#25247,#25248,#25249,#25250,
#25251,#25252,#25253,#25254,#25255,#25256,#25257,#25258,#25259,#25260,#25261,
#25262,#25263),.UNSPECIFIED.,.F.,.F.,(4,2,2,2,2,2,2,2,2,2,2,2,2,2,2,2,2,
2,2,4),(-2.43135763693152,-2.39010762561609,-2.3736094853284,-2.3689324498023,
-2.36601639977979,-2.36332310713148,-2.35983442650161,-2.35216055904289,
-2.31704743805613,-2.28764413026702,-2.27844799834302,-2.27249722781729,
-2.2702960836424,-2.26872965301005,-2.26733120275681,-2.26541997702744,
-2.26064552361995,-2.2241812751241,-2.19576577617892,-2.18919381409884),
 .UNSPECIFIED.);
#1183=B_SPLINE_CURVE_WITH_KNOTS('',3,(#25265,#25266,#25267,#25268,#25269,
#25270,#25271,#25272,#25273,#25274,#25275,#25276,#25277,#25278,#25279,#25280,
#25281,#25282,#25283,#25284,#25285,#25286,#25287,#25288,#25289,#25290,#25291,
#25292,#25293,#25294,#25295,#25296,#25297,#25298,#25299,#25300,#25301,#25302,
#25303,#25304,#25305,#25306,#25307,#25308),.UNSPECIFIED.,.F.,.F.,(4,2,2,
2,2,2,2,2,2,2,2,2,2,2,2,2,2,2,2,2,2,4),(-0.242598015109206,-0.227163281818878,
-0.203228039698266,-0.197905029555936,-0.194857094765726,-0.192436765906469,
-0.189919151777873,-0.18506649448357,-0.166510004901814,-0.12697888806249,
-0.102972664901064,-0.0998183661447284,-0.0978855205166566,-0.0963868748126413,
-0.0946291020277296,-0.0914086123451188,-0.0730339436113313,-0.0468214669586457,
-0.0105994822371148,-0.0049216022030536,-0.00224184904898379,-0.000573763776605669),
 .UNSPECIFIED.);
#1184=B_SPLINE_CURVE_WITH_KNOTS('',3,(#25309,#25310,#25311,#25312,#25313,
#25314,#25315,#25316,#25317,#25318,#25319,#25320,#25321,#25322,#25323,#25324,
#25325,#25326,#25327,#25328,#25329,#25330,#25331,#25332,#25333,#25334,#25335,
#25336,#25337,#25338,#25339,#25340,#25341,#25342,#25343,#25344,#25345,#25346,
#25347,#25348,#25349,#25350,#25351,#25352,#25353,#25354,#25355,#25356,#25357,
#25358,#25359,#25360,#25361,#25362,#25363,#25364,#25365,#25366,#25367,#25368,
#25369,#25370,#25371,#25372,#25373,#25374,#25375,#25376,#25377,#25378,#25379,
#25380,#25381,#25382,#25383,#25384,#25385,#25386,#25387,#25388,#25389,#25390,
#25391,#25392,#25393,#25394,#25395,#25396,#25397,#25398,#25399,#25400,#25401,
#25402,#25403,#25404,#25405,#25406,#25407,#25408,#25409,#25410,#25411,#25412,
#25413,#25414,#25415,#25416,#25417,#25418,#25419,#25420,#25421,#25422,#25423,
#25424,#25425,#25426,#25427,#25428,#25429,#25430,#25431,#25432,#25433,#25434,
#25435,#25436,#25437,#25438,#25439,#25440,#25441,#25442,#25443,#25444,#25445,
#25446,#25447,#25448,#25449,#25450,#25451,#25452,#25453,#25454,#25455,#25456,
#25457,#25458,#25459,#25460,#25461,#25462,#25463,#25464,#25465,#25466,#25467,
#25468,#25469,#25470,#25471,#25472,#25473,#25474,#25475,#25476,#25477,#25478,
#25479,#25480),.UNSPECIFIED.,.F.,.F.,(4,2,2,2,2,2,2,2,2,2,2,2,2,2,2,2,2,
2,2,2,2,2,2,2,2,2,2,2,2,2,2,2,2,2,2,2,2,2,2,2,2,2,2,2,2,2,2,2,2,2,2,2,2,
2,2,2,2,2,2,2,2,2,2,2,2,2,2,2,2,2,2,2,2,2,2,2,2,2,2,2,2,2,2,2,2,4),(-2.43064787994583,
-2.4289190210585,-2.42590811732101,-2.42030236014,-2.38685906955935,-2.34389011788488,
-2.33756419720643,-2.33526545999383,-2.33370916013169,-2.33230379034719,
-2.33036283993118,-2.32540758614958,-2.29569892686985,-2.26251447774013,
-2.24552119086148,-2.24080133843114,-2.23829282289489,-2.23584217532018,
-2.23273719918661,-2.22715894983949,-2.19068040242632,-2.16422719106788,
-2.14615275733102,-2.14294522181671,-2.14119069149659,-2.13969239880238,
-2.13775690350697,-2.13459222877797,-2.10959332943499,-2.10307293607284,
-2.07848455943645,-2.05340159386969,-2.04813276729518,-2.04508890314991,
-2.04242399270497,-2.03911015689396,-2.03396836240495,-1.9988459325157,
-1.96627775410301,-1.95711350629871,-1.95112099402074,-1.94886973898967,
-1.94732291346048,-1.94590794469718,-1.9439301998852,-1.93984041333757,
-1.89855366435952,-1.86609895593524,-1.85705972856345,-1.85329963442785,
-1.85057314229474,-1.84807189670572,-1.8446850018454,-1.83624862938741,
-1.78259217885247,-1.76191112988104,-1.75732366100261,-1.75529851846876,
-1.75379011226426,-1.7520902015077,-1.74913505322763,-1.73761679237468,
-1.72690675488464,-1.69243946737807,-1.66700178032922,-1.66171495221982,
-1.65866704501352,-1.65600233945449,-1.65269363251008,-1.64756920491083,
-1.61448414016948,-1.57112173838723,-1.56477359990295,-1.56247150322932,
-1.56091431370218,-1.55950922833424,-1.55757005656073,-1.55262638160502,
-1.52231856401055,-1.4906834685268,-1.47887261063741,-1.47038015652668,
-1.46671046107402,-1.46399919321191,-1.46113238353101,-1.45771014066774),
 .UNSPECIFIED.);
#1185=B_SPLINE_CURVE_WITH_KNOTS('',3,(#25485,#25486,#25487,#25488,#25489,
#25490,#25491,#25492,#25493,#25494,#25495,#25496,#25497,#25498,#25499,#25500,
#25501,#25502,#25503,#25504,#25505,#25506,#25507,#25508,#25509,#25510,#25511,
#25512,#25513,#25514,#25515,#25516,#25517,#25518,#25519,#25520,#25521,#25522,
#25523,#25524,#25525,#25526,#25527,#25528,#25529,#25530,#25531,#25532,#25533,
#25534,#25535,#25536,#25537,#25538,#25539,#25540,#25541,#25542,#25543,#25544,
#25545,#25546,#25547,#25548,#25549,#25550,#25551,#25552,#25553,#25554,#25555,
#25556,#25557,#25558,#25559,#25560,#25561,#25562,#25563,#25564,#25565,#25566,
#25567,#25568,#25569,#25570,#25571,#25572,#25573,#25574,#25575,#25576,#25577,
#25578,#25579,#25580,#25581,#25582,#25583,#25584,#25585,#25586,#25587,#25588,
#25589,#25590,#25591,#25592,#25593,#25594,#25595,#25596,#25597,#25598,#25599,
#25600,#25601,#25602,#25603,#25604,#25605,#25606,#25607,#25608,#25609,#25610,
#25611,#25612,#25613,#25614,#25615,#25616,#25617,#25618,#25619,#25620,#25621,
#25622,#25623,#25624,#25625,#25626,#25627,#25628,#25629,#25630,#25631,#25632,
#25633,#25634,#25635,#25636,#25637,#25638,#25639,#25640,#25641,#25642,#25643,
#25644,#25645,#25646,#25647,#25648,#25649,#25650,#25651,#25652,#25653,#25654,
#25655,#25656,#25657,#25658,#25659,#25660,#25661,#25662,#25663,#25664,#25665,
#25666,#25667,#25668,#25669,#25670,#25671,#25672,#25673,#25674,#25675,#25676,
#25677,#25678,#25679,#25680,#25681,#25682,#25683,#25684,#25685,#25686,#25687,
#25688,#25689,#25690,#25691,#25692,#25693,#25694,#25695,#25696,#25697,#25698,
#25699,#25700,#25701,#25702,#25703,#25704,#25705,#25706),.UNSPECIFIED.,
 .F.,.F.,(4,2,2,2,2,2,2,2,2,2,2,2,2,2,2,2,2,2,2,2,2,2,2,2,2,2,2,2,2,2,2,
2,2,2,2,2,2,2,2,2,2,2,2,2,2,2,2,2,2,2,2,2,2,2,2,2,2,2,2,2,2,2,2,2,2,2,2,
2,2,2,2,2,2,2,2,2,2,2,2,2,2,2,2,2,2,2,2,2,2,2,2,2,2,2,2,2,2,2,2,2,2,2,2,
2,2,2,2,2,2,2,4),(-2.18893440373178,-2.18602305786878,-2.16487091400591,
-2.16023231457417,-2.15819763181326,-2.1566874213041,-2.15499135353963,
-2.15205568663814,-2.14077685919479,-2.13002647373089,-2.09535795113231,
-2.06988112048211,-2.064590891489,-2.06154147031496,-2.05887569195832,-2.05556596644588,
-2.05044053335471,-2.01740304575757,-1.97398955760533,-1.96763755204927,
-1.9653343451133,-1.9637764821387,-1.96237082841933,-1.96043089521855,-1.95548537618928,
-1.92535396810428,-1.89358592516691,-1.88174720020594,-1.87323888998993,
-1.86956560541463,-1.86685287536765,-1.86432949074828,-1.86085835727804,
-1.85191396969911,-1.79887899223932,-1.77827687901786,-1.7736967184568,
-1.77167218648568,-1.7701631495298,-1.76846127573765,-1.76549991484857,
-1.75392099002902,-1.74321722797438,-1.70879026024711,-1.68335451852561,
-1.67806565603243,-1.67501622121556,-1.67234995917235,-1.66903901954368,
-1.66391052276692,-1.6306526074751,-1.5874370888434,-1.58109519990408,-1.57879317217166,
-1.57723537522772,-1.57582920619691,-1.57388782924634,-1.5689349279576,
-1.53808269105599,-1.5057295628002,-1.48896453399656,-1.48426273646838,
-1.4813410096129,-1.47864901713721,-1.47517122472504,-1.46755958068519,
-1.42707670052492,-1.40471700609384,-1.39441375747966,-1.38788865915149,
-1.38556140289252,-1.38399839314225,-1.38259675313312,-1.38067329990869,
-1.37582753832456,-1.3409293869156,-1.31144764697642,-1.30088876153053,
-1.29309029771994,-1.28954076003256,-1.28684701406824,-1.28393055504674,
-1.27925305117643,-1.26435976829608,-1.25438270843973,-1.21556411502999,
-1.20696664149327,-1.19582403134391,-1.1928994913769,-1.19120559517347,
-1.18969427530323,-1.18765399453005,-1.18298537480698,-1.16155642862552,
-1.14618853845349,-1.10741217210891,-1.0997575243565,-1.09627189659431,
-1.09357863695319,-1.09066031336706,-1.08597455117074,-1.06938876259283,
-1.03766007233324,-1.02329890733008,-1.00343974320704,-1.00035324565996,
-0.998440232838664,-0.99694262591694,-0.995169098041974,-0.991876390883277,
-0.973675603579949),.UNSPECIFIED.);
#1186=B_SPLINE_CURVE_WITH_KNOTS('',3,(#25707,#25708,#25709,#25710,#25711,
#25712,#25713,#25714,#25715,#25716,#25717,#25718,#25719,#25720,#25721,#25722,
#25723,#25724,#25725,#25726,#25727,#25728,#25729,#25730,#25731,#25732,#25733,
#25734,#25735,#25736,#25737,#25738,#25739,#25740,#25741,#25742,#25743,#25744,
#25745,#25746,#25747,#25748,#25749,#25750,#25751,#25752,#25753,#25754,#25755,
#25756,#25757,#25758,#25759,#25760,#25761,#25762,#25763,#25764,#25765,#25766,
#25767,#25768,#25769,#25770,#25771,#25772,#25773,#25774,#25775,#25776,#25777,
#25778,#25779,#25780,#25781,#25782,#25783,#25784,#25785,#25786,#25787,#25788,
#25789,#25790,#25791,#25792,#25793,#25794,#25795,#25796,#25797,#25798,#25799,
#25800,#25801,#25802,#25803,#25804,#25805,#25806,#25807,#25808,#25809,#25810,
#25811,#25812,#25813,#25814,#25815,#25816,#25817,#25818,#25819,#25820,#25821,
#25822,#25823,#25824,#25825,#25826,#25827,#25828,#25829,#25830,#25831,#25832,
#25833,#25834,#25835,#25836,#25837,#25838,#25839,#25840,#25841,#25842,#25843,
#25844,#25845,#25846,#25847,#25848,#25849,#25850,#25851,#25852,#25853,#25854,
#25855,#25856,#25857,#25858,#25859,#25860,#25861,#25862,#25863,#25864,#25865,
#25866,#25867,#25868,#25869,#25870,#25871,#25872,#25873,#25874,#25875,#25876,
#25877,#25878,#25879,#25880,#25881,#25882,#25883,#25884,#25885,#25886,#25887,
#25888,#25889,#25890,#25891,#25892,#25893,#25894,#25895,#25896,#25897,#25898,
#25899,#25900,#25901,#25902,#25903,#25904,#25905,#25906,#25907,#25908),
 .UNSPECIFIED.,.F.,.F.,(4,2,2,2,2,2,2,2,2,2,2,2,2,2,2,2,2,2,2,2,2,2,2,2,
2,2,2,2,2,2,2,2,2,2,2,2,2,2,2,2,2,2,2,2,2,2,2,2,2,2,2,2,2,2,2,2,2,2,2,2,
2,2,2,2,2,2,2,2,2,2,2,2,2,2,2,2,2,2,2,2,2,2,2,2,2,2,2,2,2,2,2,2,2,2,2,2,
2,2,2,2,4),(-1.45771014066774,-1.45667896209667,-1.4436589147369,-1.3949449356228,
-1.38036652437068,-1.37478123034979,-1.37065459855406,-1.36871390249068,
-1.36721483707466,-1.36546317299772,-1.36235665252896,-1.34826800834459,
-1.29563748950007,-1.27930531203896,-1.2746449174408,-1.27173332242007,
-1.26904015774483,-1.26554601325508,-1.25812343967897,-1.21546100192093,
-1.18283601992191,-1.17791177013262,-1.17597580612725,-1.1745715048641,
-1.17301331536511,-1.17070657569251,-1.16432529795637,-1.12034299655681,
-1.08794315292719,-1.08282539651323,-1.07951856671759,-1.07685381988491,
-1.07380416748319,-1.06850994601822,-1.04293230290773,-1.00767946574459,
-0.987191059266374,-0.984081164631363,-0.982161751905746,-0.980664489394589,
-0.978897711057709,-0.975633811286164,-0.956080509205561,-0.916934485389681,
-0.894111378017313,-0.888840883348332,-0.885765842745586,-0.883103411165743,
-0.879830815892662,-0.873474297335921,-0.830878874654645,-0.796266644605056,
-0.791407783296881,-0.789482695654562,-0.788081124010819,-0.786519723641954,
-0.784197549563012,-0.777704262364909,-0.767470357860424,-0.74538974999726,
-0.70455457474415,-0.696960129142908,-0.693486529616642,-0.690796286215908,
-0.687874974636894,-0.683170592283469,-0.666360274833386,-0.633837989435531,
-0.603209809923447,-0.598237640064125,-0.596293539579796,-0.594887128982579,
-0.593331145199573,-0.591035377371374,-0.584733268469614,-0.542208660200637,
-0.508282019138443,-0.503145329396524,-0.499832687773274,-0.497167405390114,
-0.49412166431872,-0.488845872908267,-0.463644235162826,-0.430252348335858,
-0.407534388992947,-0.404401451037019,-0.402475151664517,-0.400977316991683,
-0.399215493912936,-0.395975005937027,-0.377067344638283,-0.338707948943681,
-0.314576396216332,-0.309214885121022,-0.306119167061324,-0.303458019368198,
-0.300211151864504,-0.293981470332704,-0.286070135113773,-0.267562130815639,
-0.242523000470694),.UNSPECIFIED.);
#1187=B_SPLINE_CURVE_WITH_KNOTS('',3,(#25914,#25915,#25916,#25917,#25918,
#25919,#25920,#25921,#25922,#25923,#25924,#25925,#25926,#25927,#25928,#25929,
#25930,#25931,#25932,#25933,#25934,#25935,#25936,#25937,#25938,#25939,#25940,
#25941,#25942,#25943,#25944,#25945,#25946,#25947,#25948,#25949,#25950,#25951,
#25952,#25953,#25954,#25955,#25956,#25957,#25958,#25959,#25960,#25961,#25962,
#25963,#25964,#25965,#25966,#25967,#25968,#25969,#25970,#25971,#25972,#25973,
#25974,#25975,#25976,#25977,#25978,#25979,#25980,#25981,#25982,#25983,#25984,
#25985,#25986,#25987,#25988,#25989,#25990,#25991,#25992,#25993,#25994,#25995,
#25996,#25997,#25998,#25999,#26000,#26001,#26002,#26003,#26004,#26005,#26006,
#26007,#26008,#26009,#26010,#26011,#26012,#26013,#26014,#26015,#26016,#26017,
#26018,#26019,#26020,#26021,#26022,#26023,#26024,#26025,#26026,#26027,#26028,
#26029,#26030,#26031,#26032,#26033,#26034,#26035,#26036,#26037,#26038,#26039,
#26040,#26041,#26042,#26043,#26044,#26045,#26046,#26047,#26048,#26049,#26050,
#26051,#26052,#26053,#26054,#26055,#26056,#26057,#26058,#26059,#26060,#26061,
#26062,#26063,#26064,#26065,#26066,#26067,#26068,#26069,#26070,#26071,#26072,
#26073,#26074,#26075,#26076,#26077,#26078,#26079,#26080,#26081,#26082,#26083,
#26084,#26085,#26086,#26087),.UNSPECIFIED.,.F.,.F.,(4,2,2,2,2,2,2,2,2,2,
2,2,2,2,2,2,2,2,2,2,2,2,2,2,2,2,2,2,2,2,2,2,2,2,2,2,2,2,2,2,2,2,2,2,2,2,
2,2,2,2,2,2,2,2,2,2,2,2,2,2,2,2,2,2,2,2,2,2,2,2,2,2,2,2,2,2,2,2,2,2,2,2,
2,2,2,2,4),(-0.973953791624347,-0.967465283548968,-0.93257382470948,-0.894350184248222,
-0.889667267830394,-0.887771673941779,-0.886238480733053,-0.884633020449155,
-0.882108315310275,-0.873977447167938,-0.859864109875752,-0.816722088528658,
-0.798592648572637,-0.793583341054268,-0.790594766678859,-0.787919862796101,
-0.784514637423928,-0.777490251075113,-0.750471891894025,-0.706204541135851,
-0.697629614907016,-0.69495920454513,-0.693321547969722,-0.691789277177381,
-0.689618848966036,-0.684165984301634,-0.676104448185037,-0.649427519433313,
-0.609666667085141,-0.602035471931189,-0.598554287537814,-0.595861918601123,
-0.592942027209865,-0.58824815409868,-0.571569594685118,-0.539517057923146,
-0.508214878954685,-0.503267252809573,-0.501326820288319,-0.49992092930726,
-0.498362936215472,-0.496059777511753,-0.489709292117109,-0.446327241972436,
-0.413284282842176,-0.408158636613833,-0.40484854774077,-0.402182350935323,
-0.399132313220868,-0.393840672264474,-0.368353088603507,-0.333667606726196,
-0.32290141055539,-0.311610242154255,-0.308673126592816,-0.306976564446801,
-0.305466139022737,-0.303431506604102,-0.298794354924746,-0.277661467989196,
-0.267257679463108,-0.222792088207318,-0.215387494571896,-0.211947562297166,
-0.209338104763373,-0.209118628772211,-0.206205006617162,-0.203140246674459,
-0.19858310458366,-0.19029767399017,-0.170441064598559,-0.127939719980367,
-0.118095997031503,-0.11528904690412,-0.113621126960683,-0.112101720114293,
-0.110007019702433,-0.105020942601532,-0.0804123930246865,-0.0394781845988557,
-0.0248226972464058,-0.020173041506687,-0.0172627057060512,-0.0146929297418167,
-0.0120771358670828,-0.00710051591487547,-0.000573354566209522),
 .UNSPECIFIED.);
#1188=B_SPLINE_CURVE_WITH_KNOTS('',3,(#26088,#26089,#26090,#26091,#26092,
#26093,#26094,#26095,#26096,#26097,#26098,#26099,#26100,#26101,#26102,#26103,
#26104,#26105,#26106,#26107,#26108,#26109,#26110,#26111,#26112,#26113,#26114,
#26115,#26116,#26117,#26118,#26119,#26120,#26121,#26122,#26123,#26124,#26125,
#26126,#26127,#26128,#26129),.UNSPECIFIED.,.F.,.F.,(4,2,2,2,2,2,2,2,2,2,
2,2,2,2,2,2,2,2,2,2,4),(-2.43089244675199,-2.40677745000843,-2.35827798625117,
-2.35352462500566,-2.35146986841046,-2.34995680866057,-2.34827086484605,
-2.34538127194777,-2.33462896991367,-2.32694146459418,-2.28202576276737,
-2.26906222322403,-2.26284470438802,-2.25909990257145,-2.25575924492405,
-2.25317421810439,-2.25062377863152,-2.24632839655743,-2.23451447360949,
-2.19012167723457,-2.18893440373178),.UNSPECIFIED.);
#1189=B_SPLINE_CURVE_WITH_KNOTS('',3,(#26131,#26132,#26133,#26134,#26135,
#26136,#26137,#26138,#26139,#26140,#26141,#26142,#26143,#26144,#26145,#26146,
#26147,#26148,#26149,#26150,#26151,#26152,#26153,#26154,#26155,#26156,#26157,
#26158,#26159,#26160,#26161,#26162,#26163,#26164,#26165,#26166,#26167,#26168,
#26169,#26170,#26171,#26172,#26173,#26174,#26175,#26176,#26177,#26178,#26179,
#26180,#26181,#26182,#26183,#26184),.UNSPECIFIED.,.F.,.F.,(4,2,2,2,2,2,
2,2,2,2,2,2,2,2,2,2,2,2,2,2,2,2,2,2,2,2,4),(-0.242523000470694,-0.225437215451584,
-0.213483329943007,-0.21052208750719,-0.208803534643909,-0.207328355820071,
-0.205402718327066,-0.203242716653735,-0.199587124904956,-0.191779697504846,
-0.166594550645333,-0.124805976705311,-0.117249000866896,-0.113782134205105,
-0.111092826629847,-0.108168244987422,-0.103449063901853,-0.0864739067951593,
-0.0342141991625467,-0.0222927842798497,-0.0184345143076221,-0.0165127155936031,
-0.0151118482286253,-0.0137081037350018,-0.0121594087514008,-0.0100183340058566,
-0.000573215276035292),.UNSPECIFIED.);
#1190=B_SPLINE_CURVE_WITH_KNOTS('',3,(#26185,#26186,#26187,#26188,#26189,
#26190,#26191,#26192,#26193,#26194,#26195,#26196,#26197,#26198,#26199,#26200,
#26201,#26202,#26203,#26204,#26205,#26206,#26207,#26208,#26209,#26210,#26211,
#26212,#26213,#26214,#26215,#26216,#26217,#26218,#26219,#26220,#26221,#26222,
#26223,#26224,#26225,#26226,#26227,#26228,#26229,#26230,#26231,#26232,#26233,
#26234,#26235,#26236,#26237,#26238,#26239,#26240,#26241,#26242,#26243,#26244,
#26245,#26246,#26247,#26248,#26249,#26250,#26251,#26252,#26253,#26254,#26255,
#26256,#26257,#26258,#26259,#26260,#26261,#26262,#26263,#26264,#26265,#26266,
#26267,#26268,#26269,#26270,#26271,#26272,#26273,#26274,#26275,#26276,#26277,
#26278,#26279,#26280,#26281,#26282,#26283,#26284,#26285,#26286,#26287,#26288,
#26289,#26290,#26291,#26292,#26293,#26294,#26295,#26296,#26297,#26298,#26299,
#26300,#26301,#26302,#26303,#26304,#26305,#26306,#26307,#26308,#26309,#26310,
#26311,#26312,#26313,#26314,#26315,#26316,#26317,#26318,#26319,#26320,#26321,
#26322,#26323,#26324,#26325,#26326,#26327,#26328,#26329,#26330,#26331,#26332,
#26333,#26334,#26335,#26336,#26337,#26338,#26339,#26340,#26341,#26342,#26343,
#26344,#26345,#26346,#26347,#26348,#26349,#26350),.UNSPECIFIED.,.F.,.F.,
(4,2,2,2,2,2,2,2,2,2,2,2,2,2,2,2,2,2,2,2,2,2,2,2,2,2,2,2,2,2,2,2,2,2,2,
2,2,2,2,2,2,2,2,2,2,2,2,2,2,2,2,2,2,2,2,2,2,2,2,2,2,2,2,2,2,2,2,2,2,2,2,
2,2,2,2,2,2,2,2,2,2,2,4),(-2.43140146279566,-2.38370979736051,-2.35858650028034,
-2.35331485990005,-2.35027001609835,-2.34760462941594,-2.3442906989176,
-2.33914971997813,-2.30371362431687,-2.27108906035359,-2.26213777882005,
-2.25811879143242,-2.25581520230946,-2.2538368257165,-2.2523519783445,-2.25070353057344,
-2.24798224076958,-2.2389479479071,-2.20195248740586,-2.17119534139135,
-2.1621984943043,-2.15844482225991,-2.1557190505994,-2.15321574617055,-2.14982190611309,
-2.14134635258128,-2.08772673698565,-2.06704764588328,-2.06245990744073,
-2.06043447086318,-2.05892577366725,-2.05722545440735,-2.05426941865898,
-2.04274542382737,-2.03203374958153,-1.99756225872869,-1.97211992349234,
-1.96683204606896,-1.96378352461148,-1.96111827654726,-1.95780888885823,
-1.95268339319331,-1.91958902034189,-1.87622025808154,-1.86987096202069,
-1.86756841575638,-1.86601091336605,-1.86460553882285,-1.86266595920262,
-1.85772120050715,-1.82743146116468,-1.79464970466104,-1.77776521256565,
-1.77305379162657,-1.77013066613508,-1.76744045664711,-1.76396928754582,
-1.75639006957688,-1.71506016713977,-1.68950523112516,-1.68163302011892,
-1.67627664297594,-1.67412185138993,-1.67259272297262,-1.6709500866416,
-1.66825578780362,-1.65946702755077,-1.62221375103456,-1.58735157548973,
-1.58103957103891,-1.57777563667933,-1.57511323924908,-1.57203038677833,
-1.56672698860878,-1.54333370761027,-1.5044156167401,-1.48518439795463,
-1.48193133968392,-1.48016665390761,-1.47866882862526,-1.47674570447627,
-1.47362406522875,-1.45805210159456),.UNSPECIFIED.);
#1191=B_SPLINE_CURVE_WITH_KNOTS('',3,(#26355,#26356,#26357,#26358,#26359,
#26360,#26361,#26362,#26363,#26364,#26365,#26366,#26367,#26368,#26369,#26370,
#26371,#26372,#26373,#26374,#26375,#26376,#26377,#26378,#26379,#26380,#26381,
#26382,#26383,#26384,#26385,#26386,#26387,#26388,#26389,#26390,#26391,#26392,
#26393,#26394,#26395,#26396,#26397,#26398,#26399,#26400,#26401,#26402,#26403,
#26404,#26405,#26406,#26407,#26408,#26409,#26410,#26411,#26412,#26413,#26414,
#26415,#26416,#26417,#26418,#26419,#26420,#26421,#26422,#26423,#26424,#26425,
#26426,#26427,#26428,#26429,#26430,#26431,#26432,#26433,#26434,#26435,#26436,
#26437,#26438,#26439,#26440,#26441,#26442,#26443,#26444,#26445,#26446,#26447,
#26448,#26449,#26450,#26451,#26452,#26453,#26454,#26455,#26456,#26457,#26458,
#26459,#26460,#26461,#26462,#26463,#26464,#26465,#26466,#26467,#26468,#26469,
#26470,#26471,#26472,#26473,#26474,#26475,#26476,#26477,#26478,#26479,#26480,
#26481,#26482,#26483,#26484,#26485,#26486,#26487,#26488,#26489,#26490,#26491,
#26492,#26493,#26494,#26495,#26496,#26497,#26498,#26499,#26500,#26501,#26502,
#26503,#26504,#26505,#26506,#26507,#26508,#26509,#26510,#26511,#26512,#26513,
#26514,#26515,#26516,#26517,#26518,#26519,#26520,#26521,#26522,#26523,#26524,
#26525,#26526,#26527,#26528,#26529,#26530,#26531,#26532,#26533,#26534,#26535,
#26536,#26537,#26538,#26539,#26540,#26541,#26542,#26543,#26544,#26545,#26546,
#26547,#26548,#26549,#26550,#26551,#26552,#26553,#26554,#26555,#26556,#26557,
#26558,#26559,#26560,#26561,#26562,#26563,#26564,#26565,#26566,#26567,#26568,
#26569,#26570),.UNSPECIFIED.,.F.,.F.,(4,2,2,2,2,2,2,2,2,2,2,2,2,2,2,2,2,
2,2,2,2,2,2,2,2,2,2,2,2,2,2,2,2,2,2,2,2,2,2,2,2,2,2,2,2,2,2,2,2,2,2,2,2,
2,2,2,2,2,2,2,2,2,2,2,2,2,2,2,2,2,2,2,2,2,2,2,2,2,2,2,2,2,2,2,2,2,2,2,2,
2,2,2,2,2,2,2,2,2,2,2,2,2,2,2,2,2,2,4),(-2.18908437233165,-2.18018897530132,
-2.16147584202253,-2.1535059286629,-2.14723917490848,-2.14398413157484,
-2.14157877424435,-2.13857926260685,-2.13351900829028,-2.11468332877233,
-2.07646810778413,-2.05169001029865,-2.04828132401378,-2.04648358683509,
-2.04498802921325,-2.04310600217505,-2.04012204858244,-2.02309177048872,
-1.98461402729307,-1.95863660825575,-1.95332209409581,-1.95026735957319,
-1.94760202824388,-1.94429945837683,-1.93919779280146,-1.90236137329814,
-1.87607577873784,-1.85811309456896,-1.85490881003816,-1.85315437472235,
-1.8516550916492,-1.84971688455819,-1.8465449384384,-1.82061848294505,-1.79609686870761,
-1.76840600251381,-1.76129593804436,-1.75787438079302,-1.75519771874331,
-1.75221859884262,-1.74725240130115,-1.7297647183804,-1.68599126390407,
-1.67178639394292,-1.66362059419485,-1.66109199454717,-1.6594856939297,
-1.65795309219008,-1.6560597201182,-1.65138956113164,-1.61289579102747,
-1.57393927536086,-1.56758160551049,-1.56430792359671,-1.56164434582861,
-1.55856767741368,-1.55329360686779,-1.5304384447075,-1.49128283574657,
-1.4717223947889,-1.46845698503998,-1.46668940168618,-1.46519144171741,
-1.46327109001382,-1.46015959070346,-1.43965840171215,-1.40444384221564,
-1.3788735253873,-1.37357817129341,-1.37052738355103,-1.36786134426156,
-1.36455250817576,-1.35943079075152,-1.32201509685289,-1.29311230136627,
-1.28305869310448,-1.27664802728967,-1.27433658392991,-1.27277694721012,
-1.27137266659989,-1.26943840522657,-1.26452736074527,-1.23136005854359,
-1.21611666486218,-1.18625101294632,-1.18116878531827,-1.17787190342583,
-1.1752066923533,-1.17214717987868,-1.16681158537516,-1.1403977464359,-1.11656711192485,
-1.1025136908001,-1.08534256231142,-1.08235254472572,-1.08046861774952,
-1.07897285931959,-1.07717644124281,-1.07377450652148,-1.04931653877236,
-1.04148220225156,-0.995695977725987,-0.989120603118532,-0.985762090778382,
-0.983266831226487,-0.980532244715124,-0.976733915400356,-0.973953791624347),
 .UNSPECIFIED.);
#1192=B_SPLINE_CURVE_WITH_KNOTS('',3,(#26571,#26572,#26573,#26574,#26575,
#26576,#26577,#26578,#26579,#26580,#26581,#26582,#26583,#26584,#26585,#26586,
#26587,#26588,#26589,#26590,#26591,#26592,#26593,#26594,#26595,#26596,#26597,
#26598,#26599,#26600,#26601,#26602,#26603,#26604,#26605,#26606,#26607,#26608,
#26609,#26610,#26611,#26612,#26613,#26614,#26615,#26616,#26617,#26618,#26619,
#26620,#26621,#26622,#26623,#26624,#26625,#26626,#26627,#26628,#26629,#26630,
#26631,#26632,#26633,#26634,#26635,#26636,#26637,#26638,#26639,#26640,#26641,
#26642,#26643,#26644,#26645,#26646,#26647,#26648,#26649,#26650,#26651,#26652,
#26653,#26654,#26655,#26656,#26657,#26658,#26659,#26660,#26661,#26662,#26663,
#26664,#26665,#26666,#26667,#26668,#26669,#26670,#26671,#26672,#26673,#26674,
#26675,#26676,#26677,#26678,#26679,#26680,#26681,#26682,#26683,#26684,#26685,
#26686,#26687,#26688,#26689,#26690,#26691,#26692,#26693,#26694,#26695,#26696,
#26697,#26698,#26699,#26700,#26701,#26702,#26703,#26704,#26705,#26706,#26707,
#26708,#26709,#26710,#26711,#26712,#26713,#26714,#26715,#26716,#26717,#26718,
#26719,#26720,#26721,#26722,#26723,#26724,#26725,#26726,#26727,#26728,#26729,
#26730,#26731,#26732,#26733,#26734,#26735,#26736,#26737,#26738,#26739,#26740,
#26741,#26742,#26743,#26744,#26745,#26746,#26747,#26748,#26749,#26750,#26751,
#26752,#26753,#26754,#26755,#26756,#26757,#26758,#26759,#26760,#26761,#26762,
#26763,#26764,#26765,#26766,#26767,#26768,#26769,#26770,#26771,#26772,#26773,
#26774,#26775,#26776,#26777,#26778,#26779,#26780,#26781,#26782),
 .UNSPECIFIED.,.F.,.F.,(4,2,2,2,2,2,2,2,2,2,2,2,2,2,2,2,2,2,2,2,2,2,2,2,
2,2,2,2,2,2,2,2,2,2,2,2,2,2,2,2,2,2,2,2,2,2,2,2,2,2,2,2,2,2,2,2,2,2,2,2,
2,2,2,2,2,2,2,2,2,2,2,2,2,2,2,2,2,2,2,2,2,2,2,2,2,2,2,2,2,2,2,2,2,2,2,2,
2,2,2,2,2,2,2,2,2,4),(-1.45805210159456,-1.45155832824827,-1.41765818253014,
-1.39233078637762,-1.38704820423083,-1.38400064475323,-1.38133500580256,
-1.37802352940773,-1.37289170412753,-1.33930255891899,-1.29639934286917,
-1.2900751176326,-1.28777593157304,-1.28621901397535,-1.28481283948997,
-1.28287046280774,-1.27790994558091,-1.24824005346882,-1.21613472700597,
-1.19848888329236,-1.19350923827962,-1.19052739993062,-1.18785166355357,
-1.18443594985395,-1.17735535784278,-1.14989380355426,-1.13973334595397,
-1.10100471792365,-1.09634369476463,-1.09445204800143,-1.09292005251862,
-1.09131341960513,-1.08878266943041,-1.08059533491553,-1.06633662164289,
-1.02209861898637,-1.00505955494107,-1.00015690592514,-0.997191891165642,
-0.994512615658126,-0.991066404841612,-0.983825110958358,-0.95507452038955,
-0.923972351031826,-0.917250699546878,-0.904971523359243,-0.901985201712351,
-0.900260689400688,-0.8989077994464,-0.897009080966061,-0.893101552106182,
-0.887897196921466,-0.874803028849946,-0.835751626717067,-0.812637959816677,
-0.807349899771707,-0.804270337130832,-0.80160741738904,-0.798338576229525,
-0.792003391534514,-0.783921681803954,-0.764806748120944,-0.729639509155669,
-0.712247545169637,-0.709248964360094,-0.707362622897675,-0.705867002370958,
-0.704073250379847,-0.700683148148376,-0.676746967370331,-0.662588265387774,
-0.623102640789911,-0.615464304194692,-0.611982296638298,-0.609290300048909,
-0.606371828086698,-0.601682506472688,-0.585046985829955,-0.553142881480964,
-0.521627852765654,-0.516684149974468,-0.514744636695253,-0.513339186199238,
-0.511781433824716,-0.509478251580026,-0.503125366750244,-0.459692398241449,
-0.426694449356944,-0.421569845191526,-0.41826046255989,-0.415594869710006,
-0.412545572364426,-0.40725537892338,-0.38178235461823,-0.347183712815403,
-0.336434810682388,-0.325032544647356,-0.322086412055251,-0.320388107912964,
-0.318878592942747,-0.316848563458607,-0.312235938004416,-0.291329855913279,
-0.287488014356654,-0.244499584275477,-0.242711045913264),.UNSPECIFIED.);
#1193=B_SPLINE_CURVE_WITH_KNOTS('',3,(#26788,#26789,#26790,#26791,#26792,
#26793,#26794,#26795,#26796,#26797,#26798,#26799,#26800,#26801,#26802,#26803,
#26804,#26805,#26806,#26807,#26808,#26809,#26810,#26811,#26812,#26813,#26814,
#26815,#26816,#26817,#26818,#26819,#26820,#26821,#26822,#26823,#26824,#26825,
#26826,#26827,#26828,#26829,#26830,#26831,#26832,#26833,#26834,#26835,#26836,
#26837,#26838,#26839,#26840,#26841,#26842,#26843,#26844,#26845,#26846,#26847,
#26848,#26849,#26850,#26851,#26852,#26853,#26854,#26855,#26856,#26857,#26858,
#26859,#26860,#26861,#26862,#26863,#26864,#26865,#26866,#26867,#26868,#26869,
#26870,#26871,#26872,#26873,#26874,#26875,#26876,#26877,#26878,#26879,#26880,
#26881,#26882,#26883,#26884,#26885,#26886,#26887,#26888,#26889,#26890,#26891,
#26892,#26893,#26894,#26895,#26896,#26897,#26898,#26899,#26900,#26901,#26902,
#26903,#26904,#26905,#26906,#26907,#26908,#26909,#26910,#26911,#26912,#26913,
#26914,#26915,#26916,#26917,#26918,#26919,#26920,#26921,#26922,#26923,#26924,
#26925,#26926,#26927,#26928,#26929,#26930,#26931,#26932,#26933,#26934,#26935,
#26936,#26937,#26938,#26939,#26940,#26941,#26942,#26943,#26944,#26945,#26946,
#26947,#26948,#26949,#26950,#26951,#26952,#26953,#26954,#26955,#26956,#26957,
#26958,#26959,#26960,#26961,#26962,#26963,#26964,#26965),.UNSPECIFIED.,
 .F.,.F.,(4,2,2,2,2,2,2,2,2,2,2,2,2,2,2,2,2,2,2,2,2,2,2,2,2,2,2,2,2,2,2,
2,2,2,2,2,2,2,2,2,2,2,2,2,2,2,2,2,2,2,2,2,2,2,2,2,2,2,2,2,2,2,2,2,2,2,2,
2,2,2,2,2,2,2,2,2,2,2,2,2,2,2,2,2,2,2,2,2,4),(-0.973680670967328,-0.973307112572624,
-0.970220541363192,-0.968473310280311,-0.966987818653059,-0.965048391252937,
-0.960928624075663,-0.95535589718811,-0.940828043205159,-0.893006977768661,
-0.879263898633052,-0.874720999707776,-0.871834782675239,-0.869131868753156,
-0.865514359003847,-0.857325865642324,-0.846067488257675,-0.812917873193628,
-0.783111919959633,-0.778158141897692,-0.77621714532033,-0.774811531052763,
-0.773254517483143,-0.770954214231317,-0.76462061636457,-0.721522501514497,
-0.688210222796253,-0.683083250219667,-0.679773334948916,-0.677107942420935,
-0.674059548236232,-0.668772614842662,-0.643352814329744,-0.608991222007037,
-0.594277944636392,-0.586000149579008,-0.583365199668248,-0.5817357104235,
-0.580199965929129,-0.578008413965618,-0.572416758313034,-0.564076622368752,
-0.535656242335143,-0.498199762596961,-0.490532534490196,-0.487045628025484,
-0.484353187475155,-0.481437547404829,-0.476760049399391,-0.460248456596532,
-0.406066518825857,-0.393522706038287,-0.390517210355603,-0.388788323940043,
-0.387436142727619,-0.385543740037546,-0.381668302843481,-0.376518843685185,
-0.363631187904509,-0.324961652495334,-0.301243430819132,-0.295922541049584,
-0.292835567998951,-0.290173196477519,-0.286913810897248,-0.280625014431996,
-0.243988883928487,-0.202645276554972,-0.198234021075032,-0.196223672501802,
-0.194763546437064,-0.193364279321359,-0.191718970663122,-0.186607333298091,
-0.179212623817119,-0.156310733632371,-0.111229925958632,-0.103869968369257,
-0.100438647868069,-0.0977538578003124,-0.0948107634063591,-0.0900087154509661,
-0.0720766169546895,-0.0143120872675185,-0.0061825986812647,-0.00361975116399399,
-0.00201508611533718,-0.00101558929569232,-0.0005762572455496),
 .UNSPECIFIED.);
#1194=B_SPLINE_CURVE_WITH_KNOTS('',3,(#26966,#26967,#26968,#26969,#26970,
#26971,#26972,#26973,#26974,#26975,#26976,#26977,#26978,#26979,#26980,#26981,
#26982,#26983,#26984,#26985,#26986,#26987,#26988,#26989,#26990,#26991,#26992,
#26993,#26994,#26995,#26996,#26997,#26998,#26999,#27000,#27001,#27002,#27003,
#27004,#27005,#27006,#27007),.UNSPECIFIED.,.F.,.F.,(4,2,2,2,2,2,2,2,2,2,
2,2,2,2,2,2,2,2,2,2,4),(-2.43110192767283,-2.43046386845514,-2.4286601279836,
-2.42395621479106,-2.38392888016529,-2.34632532223177,-2.34029961040404,
-2.33709440964267,-2.3344595056279,-2.3313368283343,-2.32585712279234,-2.29865413240242,
-2.25008607935706,-2.24301003239931,-2.24061086161376,-2.23921421723126,
-2.23770922238876,-2.23560160568965,-2.23067339359046,-2.20291808918862,
-2.18908437233165),.UNSPECIFIED.);
#1195=B_SPLINE_CURVE_WITH_KNOTS('',3,(#27009,#27010,#27011,#27012,#27013,
#27014,#27015,#27016,#27017,#27018,#27019,#27020,#27021,#27022,#27023,#27024,
#27025,#27026,#27027,#27028,#27029,#27030,#27031,#27032,#27033,#27034,#27035,
#27036,#27037,#27038,#27039,#27040,#27041,#27042,#27043,#27044,#27045,#27046,
#27047,#27048,#27049,#27050,#27051,#27052,#27053,#27054,#27055,#27056,#27057,
#27058,#27059,#27060,#27061,#27062,#27063,#27064),.UNSPECIFIED.,.F.,.F.,
(4,2,2,2,2,2,2,2,2,2,2,2,2,2,2,2,2,2,2,2,2,2,2,2,2,2,2,4),(-0.242711045913264,
-0.231176709974483,-0.226684594073206,-0.22380892673107,-0.221154531929772,
-0.217633423655963,-0.213704703696832,-0.207029271880388,-0.192651858150418,
-0.164304706903861,-0.157250992792754,-0.132746176728411,-0.12958524641712,
-0.127650438261172,-0.126151631030437,-0.124395257839107,-0.121181296267978,
-0.102970487894109,-0.0656064654841873,-0.047230945741886,-0.0370128089892073,
-0.0329512545508428,-0.0304445845184497,-0.0279065401753038,-0.0252520144840107,
-0.0217418394651842,-0.0138411091822967,-0.000573273520096065),
 .UNSPECIFIED.);
#1196=B_SPLINE_CURVE_WITH_KNOTS('',3,(#27065,#27066,#27067,#27068,#27069,
#27070,#27071,#27072,#27073,#27074,#27075,#27076,#27077,#27078,#27079,#27080,
#27081,#27082,#27083,#27084,#27085,#27086,#27087,#27088,#27089,#27090,#27091,
#27092,#27093,#27094,#27095,#27096,#27097,#27098,#27099,#27100,#27101,#27102,
#27103,#27104,#27105,#27106,#27107,#27108,#27109,#27110,#27111,#27112,#27113,
#27114,#27115,#27116,#27117,#27118,#27119,#27120,#27121,#27122,#27123,#27124,
#27125,#27126,#27127,#27128,#27129,#27130,#27131,#27132,#27133,#27134,#27135,
#27136,#27137,#27138,#27139,#27140,#27141,#27142,#27143,#27144,#27145,#27146,
#27147,#27148,#27149,#27150,#27151,#27152,#27153,#27154,#27155,#27156,#27157,
#27158,#27159,#27160,#27161,#27162,#27163,#27164,#27165,#27166,#27167,#27168,
#27169,#27170,#27171,#27172,#27173,#27174,#27175,#27176,#27177,#27178,#27179,
#27180,#27181,#27182,#27183,#27184,#27185,#27186,#27187,#27188,#27189,#27190,
#27191,#27192,#27193,#27194,#27195,#27196,#27197,#27198,#27199,#27200,#27201,
#27202,#27203,#27204,#27205,#27206,#27207,#27208,#27209,#27210,#27211,#27212,
#27213,#27214,#27215,#27216,#27217,#27218,#27219,#27220,#27221,#27222,#27223,
#27224,#27225,#27226,#27227,#27228,#27229,#27230,#27231,#27232,#27233,#27234,
#27235,#27236,#27237,#27238,#27239,#27240,#27241,#27242,#27243,#27244,#27245,
#27246,#27247,#27248),.UNSPECIFIED.,.F.,.F.,(4,2,2,2,2,2,2,2,2,2,2,2,2,
2,2,2,2,2,2,2,2,2,2,2,2,2,2,2,2,2,2,2,2,2,2,2,2,2,2,2,2,2,2,2,2,2,2,2,2,
2,2,2,2,2,2,2,2,2,2,2,2,2,2,2,2,2,2,2,2,2,2,2,2,2,2,2,2,2,2,2,2,2,2,2,2,
2,2,2,2,2,2,4),(-2.43059120140729,-2.40176411519585,-2.37924065705335,-2.37191823912807,
-2.36684510743679,-2.36473671149885,-2.36321586566685,-2.3615555629141,
-2.35877998558255,-2.34924819275323,-2.31258978755237,-2.28864380702338,
-2.27931354962663,-2.2722873728991,-2.26891256605437,-2.26885041105801,
-2.26882259043734,-2.26879192438638,-2.26875805672232,-2.26872057308606,
-2.26867898886497,-2.268632733327,-2.26600523940527,-2.26298236445286,-2.25781076479936,
-2.23771651997203,-2.19527932024513,-2.1759384101753,-2.17268207697178,
-2.17091698551516,-2.16941966203352,-2.1674982700754,-2.16438153606426,
-2.1425609685007,-2.10847038795447,-2.08310668312617,-2.07782340813856,
-2.07477622294913,-2.0721113674349,-2.06880145790918,-2.06367320676321,
-2.03025474691899,-1.98720856692464,-1.98087757698263,-1.97857783629604,
-1.97702110400056,-1.97561553824432,-1.97367456521103,-1.96872052565076,
-1.9377000258246,-1.90548737825386,-1.88876505130444,-1.88406877644971,
-1.88114929104664,-1.87845857759594,-1.87498134652716,-1.86736649729363,
-1.82707107844286,-1.80459233392749,-1.7942629259308,-1.7877267676132,-1.78539878519538,
-1.7838362138004,-1.78243569868484,-1.78051474842912,-1.7756803150939,-1.74047688857932,
-1.71121863782505,-1.70070704339347,-1.69293626210463,-1.68939286501308,
-1.68670119331296,-1.68378448128163,-1.67910109205838,-1.66413884314958,
-1.65424683554806,-1.61543674897209,-1.59628315833094,-1.5930333385922,
-1.59126951169962,-1.58977187376964,-1.58784828772541,-1.58472452416869,
-1.56320591087893,-1.52887149709664,-1.50345648675929,-1.49817025296574,
-1.49512223096155,-1.49245715624619,-1.48914764185125,-1.48402129172557,
-1.45774156469356),.UNSPECIFIED.);
#1197=B_SPLINE_CURVE_WITH_KNOTS('',3,(#27253,#27254,#27255,#27256,#27257,
#27258,#27259,#27260,#27261,#27262,#27263,#27264,#27265,#27266,#27267,#27268,
#27269,#27270,#27271,#27272,#27273,#27274,#27275,#27276,#27277,#27278,#27279,
#27280,#27281,#27282,#27283,#27284,#27285,#27286,#27287,#27288,#27289,#27290,
#27291,#27292,#27293,#27294,#27295,#27296,#27297,#27298,#27299,#27300,#27301,
#27302,#27303,#27304,#27305,#27306,#27307,#27308,#27309,#27310,#27311,#27312,
#27313,#27314,#27315,#27316,#27317,#27318,#27319,#27320,#27321,#27322,#27323,
#27324,#27325,#27326,#27327,#27328,#27329,#27330,#27331,#27332,#27333,#27334,
#27335,#27336,#27337,#27338,#27339,#27340,#27341,#27342,#27343,#27344,#27345,
#27346,#27347,#27348,#27349,#27350,#27351,#27352,#27353,#27354,#27355,#27356,
#27357,#27358,#27359,#27360,#27361,#27362,#27363,#27364,#27365,#27366,#27367,
#27368,#27369,#27370,#27371,#27372,#27373,#27374,#27375,#27376,#27377,#27378,
#27379,#27380,#27381,#27382,#27383,#27384,#27385,#27386,#27387,#27388,#27389,
#27390,#27391,#27392,#27393,#27394,#27395,#27396,#27397,#27398,#27399,#27400,
#27401,#27402,#27403,#27404,#27405,#27406,#27407,#27408,#27409,#27410,#27411,
#27412,#27413,#27414,#27415,#27416,#27417,#27418,#27419,#27420,#27421,#27422,
#27423,#27424,#27425,#27426,#27427,#27428,#27429,#27430,#27431,#27432,#27433,
#27434,#27435,#27436,#27437,#27438,#27439,#27440,#27441,#27442,#27443,#27444,
#27445,#27446,#27447,#27448,#27449,#27450,#27451,#27452,#27453,#27454,#27455,
#27456),.UNSPECIFIED.,.F.,.F.,(4,2,2,2,2,2,2,2,2,2,2,2,2,2,2,2,2,2,2,2,
2,2,2,2,2,2,2,2,2,2,2,2,2,2,2,2,2,2,2,2,2,2,2,2,2,2,2,2,2,2,2,2,2,2,2,2,
2,2,2,2,2,2,2,2,2,2,2,2,2,2,2,2,2,2,2,2,2,2,2,2,2,2,2,2,2,2,2,2,2,2,2,2,
2,2,2,2,2,2,2,2,2,4),(-2.18849108915717,-2.15266013468229,-2.13281934407809,
-2.12953807643128,-2.12776459071803,-2.1262696251205,-2.12436212834478,
-2.12127664626578,-2.10117972039313,-2.06558767109897,-2.04160339281333,
-2.03538884025472,-2.03215696032724,-2.02976736911702,-2.02678602079028,
-2.0217536328847,-2.00304045513004,-1.95472191134549,-1.94416894088238,
-1.93753929223462,-1.93520875496794,-1.93365257342325,-1.93225578835142,
-1.93034928785462,-1.92559383454869,-1.8886671237466,-1.84844494068774,
-1.84195091334751,-1.83864673129327,-1.83600188812104,-1.83294821141922,
-1.82778782534966,-1.80675962260305,-1.76643055187204,-1.74633971953345,
-1.74305035011965,-1.7412745648043,-1.73977427310048,-1.73785560607621,
-1.73475232613582,-1.71448898236866,-1.67909908352295,-1.65352095508538,
-1.64822512625401,-1.64517395417711,-1.64250749105697,-1.63919799698376,
-1.63407499966821,-1.59659594405102,-1.5679143463654,-1.55774813459632,
-1.55128604804088,-1.54896793492492,-1.54740728361188,-1.54600572536922,
-1.5440787692502,-1.53920555437016,-1.50500423318681,-1.48755700157245,
-1.46953798830174,-1.46176657325522,-1.45562407869187,-1.45239637310504,
-1.44999580223646,-1.44698224204046,-1.44184898309285,-1.42206268676701,
-1.38039460898463,-1.35994186780902,-1.35664890488591,-1.35487669537028,
-1.35338027033035,-1.35146931769891,-1.34838859788563,-1.32866247366433,
-1.29274268820445,-1.26707154246869,-1.2617714319881,-1.25871962402025,
-1.25605368973657,-1.25274626062083,-1.2476291187028,-1.21544667268272,
-1.19159390250438,-1.16714204705005,-1.16398156093356,-1.16204651928411,
-1.16054735685897,-1.15879040479579,-1.1555739960999,-1.13730219780434,
-1.111015762905,-1.0746174170429,-1.06949637276067,-1.06618819079095,-1.06352283731794,
-1.06047300664893,-1.05517977129378,-1.02963633647775,-0.994598971063149,
-0.987054886639988,-0.973680670967328),.UNSPECIFIED.);
#1198=B_SPLINE_CURVE_WITH_KNOTS('',3,(#27457,#27458,#27459,#27460,#27461,
#27462,#27463,#27464,#27465,#27466,#27467,#27468,#27469,#27470,#27471,#27472,
#27473,#27474,#27475,#27476,#27477,#27478,#27479,#27480,#27481,#27482,#27483,
#27484,#27485,#27486,#27487,#27488,#27489,#27490,#27491,#27492,#27493,#27494,
#27495,#27496,#27497,#27498,#27499,#27500,#27501,#27502,#27503,#27504,#27505,
#27506,#27507,#27508,#27509,#27510,#27511,#27512,#27513,#27514,#27515,#27516,
#27517,#27518,#27519,#27520,#27521,#27522,#27523,#27524,#27525,#27526,#27527,
#27528,#27529,#27530,#27531,#27532,#27533,#27534,#27535,#27536,#27537,#27538,
#27539,#27540,#27541,#27542,#27543,#27544,#27545,#27546,#27547,#27548,#27549,
#27550,#27551,#27552,#27553,#27554,#27555,#27556,#27557,#27558,#27559,#27560,
#27561,#27562,#27563,#27564,#27565,#27566,#27567,#27568,#27569,#27570,#27571,
#27572,#27573,#27574,#27575,#27576,#27577,#27578,#27579,#27580,#27581,#27582,
#27583,#27584,#27585,#27586,#27587,#27588,#27589,#27590,#27591,#27592,#27593,
#27594,#27595,#27596,#27597,#27598,#27599,#27600,#27601,#27602,#27603,#27604,
#27605,#27606,#27607,#27608,#27609,#27610,#27611,#27612,#27613,#27614,#27615,
#27616,#27617,#27618,#27619,#27620,#27621,#27622,#27623,#27624,#27625,#27626,
#27627,#27628,#27629,#27630,#27631,#27632,#27633,#27634,#27635,#27636,#27637,
#27638,#27639,#27640,#27641,#27642,#27643,#27644,#27645,#27646,#27647,#27648,
#27649,#27650,#27651,#27652,#27653,#27654,#27655,#27656,#27657,#27658,#27659,
#27660,#27661,#27662,#27663,#27664,#27665,#27666),.UNSPECIFIED.,.F.,.F.,
(4,2,2,2,2,2,2,2,2,2,2,2,2,2,2,2,2,2,2,2,2,2,2,2,2,2,2,2,2,2,2,2,2,2,2,
2,2,2,2,2,2,2,2,2,2,2,2,2,2,2,2,2,2,2,2,2,2,2,2,2,2,2,2,2,2,2,2,2,2,2,2,
2,2,2,2,2,2,2,2,2,2,2,2,2,2,2,2,2,2,2,2,2,2,2,2,2,2,2,2,2,2,2,2,2,4),(-1.45774156469356,
-1.44739981159367,-1.42086196857323,-1.40297846348158,-1.39977814107482,
-1.39802489162989,-1.3965260130748,-1.39458758625038,-1.39141385330027,
-1.36359096878459,-1.35983368817261,-1.33512240877691,-1.31019738194206,
-1.30493554098366,-1.30189269784308,-1.29922689825234,-1.29590962827869,
-1.29075799384052,-1.25434783568208,-1.22794769439444,-1.21569342014878,
-1.2084541263403,-1.20595162122452,-1.2045103706597,-1.20298269617185,-1.20083591818395,
-1.19552938897309,-1.18775587556551,-1.16276588515745,-1.12070722810191,
-1.11391086713143,-1.11049812197198,-1.10798992813832,-1.10526752472965,
-1.10153432047915,-1.09266411867427,-1.04164484768245,-1.01700046353567,
-1.01383803011727,-1.01190282475087,-1.01040411329617,-1.00864838145331,
-1.00543660980835,-0.98727117919836,-0.960889904626584,-0.924453566308083,
-0.919322527633418,-0.916011508584598,-0.913346231091153,-0.910299081276575,
-0.905017225778567,-0.879699325078244,-0.845854186821235,-0.823684998781276,
-0.820561437869342,-0.818637867130274,-0.817140134727259,-0.815376050876469,
-0.812125556132187,-0.792956890817172,-0.754118616731859,-0.743488300243655,
-0.729182413309358,-0.724572265490336,-0.721671134195013,-0.718973363557861,
-0.715391464363775,-0.707407736370249,-0.696517620997121,-0.643187740116664,
-0.629767640441604,-0.626702273475596,-0.624959562333876,-0.62347255218525,
-0.621524341348986,-0.61736225612228,-0.611716185186961,-0.596898061999179,
-0.546733502324264,-0.535158172327656,-0.530895471465228,-0.528350851481221,
-0.525650144588506,-0.522053536958216,-0.513990430579724,-0.50295954172223,
-0.47106306676251,-0.439533622379584,-0.434589937295616,-0.432650548447213,
-0.43124514422834,-0.429688700694187,-0.427387590571668,-0.421040792031044,
-0.377695071781274,-0.344568260414681,-0.339444298874924,-0.3361364709531,
-0.333472915158102,-0.330426840172926,-0.325144641405455,-0.299778962680421,
-0.26546578814229,-0.243803969752984,-0.242412075418231),.UNSPECIFIED.);
#1199=B_SPLINE_CURVE_WITH_KNOTS('',3,(#27670,#27671,#27672,#27673,#27674,
#27675,#27676,#27677,#27678,#27679,#27680,#27681,#27682,#27683,#27684,#27685,
#27686,#27687,#27688,#27689,#27690,#27691,#27692,#27693,#27694,#27695,#27696,
#27697,#27698,#27699,#27700,#27701,#27702,#27703,#27704,#27705,#27706,#27707,
#27708,#27709,#27710,#27711,#27712,#27713,#27714,#27715,#27716,#27717,#27718,
#27719,#27720,#27721,#27722,#27723,#27724,#27725,#27726,#27727,#27728,#27729,
#27730,#27731,#27732,#27733,#27734,#27735,#27736),.UNSPECIFIED.,.F.,.F.,
(4,3,3,3,3,3,3,3,3,3,3,3,3,3,3,3,3,3,3,3,3,3,4),(-4.03543298028448,-3.99672304918318,
-3.89595759133389,-3.79533840330999,-3.69483804394509,-3.59440285562119,
-3.49400173130791,-3.39360360625489,-3.29310883660255,-3.19256758969348,
-3.09184776189799,-2.99754228688738,-2.89689019062382,-2.79638182227688,
-2.69598798286087,-2.59565665698743,-2.49535661742761,-2.39505667661869,
-2.29465488736954,-2.1942039278363,-2.09356879289011,-1.99836152459159,
-1.98502202421796),.UNSPECIFIED.);
#1200=B_SPLINE_CURVE_WITH_KNOTS('',3,(#27740,#27741,#27742,#27743,#27744),
 .UNSPECIFIED.,.F.,.F.,(4,1,4),(0.,0.99918076229579,1.09118169752329),
 .UNSPECIFIED.);
#1201=B_SPLINE_CURVE_WITH_KNOTS('',3,(#27746,#27747,#27748,#27749,#27750,
#27751,#27752,#27753,#27754,#27755,#27756,#27757,#27758,#27759,#27760,#27761,
#27762,#27763,#27764,#27765,#27766,#27767,#27768,#27769,#27770,#27771,#27772,
#27773,#27774,#27775,#27776,#27777,#27778,#27779,#27780,#27781,#27782,#27783,
#27784,#27785,#27786,#27787,#27788,#27789,#27790,#27791,#27792,#27793,#27794,
#27795,#27796,#27797,#27798,#27799,#27800,#27801,#27802,#27803,#27804,#27805,
#27806,#27807,#27808,#27809,#27810,#27811,#27812,#27813,#27814,#27815,#27816,
#27817,#27818,#27819,#27820,#27821,#27822,#27823,#27824,#27825,#27826,#27827,
#27828,#27829,#27830,#27831,#27832,#27833,#27834,#27835,#27836,#27837,#27838,
#27839,#27840,#27841,#27842,#27843,#27844,#27845,#27846,#27847,#27848,#27849,
#27850,#27851,#27852,#27853,#27854,#27855,#27856,#27857,#27858,#27859,#27860,
#27861,#27862,#27863,#27864,#27865,#27866,#27867,#27868,#27869,#27870,#27871,
#27872,#27873,#27874,#27875,#27876,#27877,#27878,#27879,#27880,#27881,#27882,
#27883,#27884,#27885,#27886,#27887,#27888,#27889,#27890,#27891,#27892,#27893,
#27894,#27895,#27896,#27897,#27898,#27899,#27900,#27901,#27902,#27903,#27904,
#27905,#27906,#27907,#27908,#27909,#27910,#27911,#27912,#27913,#27914,#27915,
#27916,#27917,#27918,#27919,#27920,#27921,#27922,#27923,#27924,#27925,#27926,
#27927,#27928,#27929,#27930,#27931,#27932,#27933,#27934,#27935,#27936,#27937,
#27938),.UNSPECIFIED.,.F.,.F.,(4,3,3,3,3,3,3,3,3,3,3,3,3,3,3,3,3,3,3,3,
3,3,3,3,3,3,3,3,3,3,3,3,3,3,3,3,3,3,3,3,3,3,3,3,3,3,3,3,3,3,3,3,3,3,3,3,
3,3,3,3,3,3,3,3,4),(1.09118169752329,1.1896959556779,1.29077915179211,1.38904433454204,
1.48725511535204,1.58544488685155,1.68867404628656,1.78698419332035,1.88536024163621,
1.98389249908034,1.99836152459159,2.09902676471727,2.19954548948454,2.29994544373208,
2.40028030446876,2.50058130287116,2.60087962797148,2.70127576315601,2.801718856171,
2.90234245763168,2.99754228688738,3.09829032006072,3.1988958757297,3.29938836910179,
3.39981920029758,3.50021947039764,3.60062024155676,3.7011231397562,3.80167552218592,
3.9024114541881,3.99672304918318,4.09719725455871,4.19752413466765,4.29773195500147,
4.39787459266619,4.49798354981372,4.59809028643905,4.6982969173245,4.798551330636,
4.89898993011201,4.99590381147897,5.09650340045884,5.19695718532926,5.29729360980329,
5.39756583082475,5.49780517353264,5.5980429218164,5.69838063612143,5.79876638986576,
5.89933520417227,5.99508457377477,6.09568510891062,6.196140215738,6.29647852714504,
6.39675297823251,6.49699489176417,6.59723554958376,6.69757669172742,6.79796616153923,
6.8985391436799,6.99426533607056,7.10763214834903,7.22058123652918,7.33282228707307,
7.37436700447423),.UNSPECIFIED.);
#1202=B_SPLINE_CURVE_WITH_KNOTS('',3,(#27940,#27941,#27942,#27943,#27944,
#27945,#27946,#27947,#27948,#27949,#27950,#27951,#27952,#27953,#27954,#27955,
#27956,#27957,#27958,#27959,#27960,#27961,#27962,#27963,#27964,#27965,#27966,
#27967,#27968,#27969,#27970,#27971,#27972,#27973,#27974,#27975,#27976,#27977,
#27978,#27979,#27980,#27981,#27982,#27983,#27984,#27985,#27986,#27987,#27988,
#27989,#27990,#27991,#27992,#27993,#27994,#27995,#27996,#27997,#27998,#27999,
#28000,#28001,#28002,#28003,#28004,#28005,#28006,#28007,#28008,#28009,#28010,
#28011,#28012,#28013,#28014,#28015,#28016,#28017,#28018,#28019,#28020,#28021,
#28022,#28023,#28024,#28025,#28026,#28027,#28028,#28029,#28030,#28031,#28032,
#28033,#28034,#28035,#28036,#28037,#28038,#28039,#28040,#28041,#28042,#28043,
#28044,#28045,#28046,#28047,#28048,#28049,#28050,#28051,#28052,#28053,#28054,
#28055,#28056,#28057,#28058,#28059,#28060,#28061,#28062,#28063,#28064,#28065,
#28066,#28067,#28068,#28069,#28070,#28071,#28072,#28073,#28074,#28075,#28076,
#28077,#28078,#28079,#28080,#28081,#28082,#28083,#28084,#28085,#28086,#28087,
#28088,#28089,#28090,#28091,#28092,#28093,#28094,#28095,#28096,#28097,#28098,
#28099,#28100,#28101,#28102,#28103,#28104,#28105,#28106,#28107,#28108,#28109,
#28110,#28111,#28112,#28113,#28114,#28115,#28116,#28117,#28118,#28119,#28120,
#28121,#28122,#28123,#28124,#28125,#28126,#28127,#28128,#28129),
 .UNSPECIFIED.,.F.,.F.,(4,3,3,3,3,3,3,3,3,3,3,3,3,3,3,3,3,3,3,3,3,3,3,3,
3,3,3,3,3,3,3,3,3,3,3,3,3,3,3,3,3,3,3,3,3,3,3,3,3,3,3,3,3,3,3,3,3,3,3,3,
3,3,3,4),(7.37436700470286,7.47544920574276,7.5765487283242,7.68077307083474,
7.78206527225033,7.88775568530835,7.99344609836636,8.09403166845495,8.19447144366285,
8.29479394118139,8.39505229193151,8.49527784072248,8.59550189117569,8.69582615791945,
8.79619857851924,8.89675441596759,8.99262686066215,9.09321116618092,9.19364970284286,
9.29397100745409,9.39422819361974,9.49445260784943,9.59467555549259,9.69499877779154,
9.7953701840505,9.89592507111648,9.99180762295794,10.0923882266938,10.1928229895668,
10.2931404293427,10.393393696979,10.4936141443668,10.5938330821875,10.6941522547303,
10.7945195828049,10.8950703914646,10.9909883852537,11.0915713241027,11.1920084546912,
11.2923283001836,11.392583995592,11.4928068894489,11.5930282890972,11.6933499304325,
11.793719735156,11.8942730043996,11.9901691475495,12.0907517522298,12.191188549124,
12.2915080632764,12.3917634289269,12.4919859950748,12.5922070695311,12.6925283919897,
12.7928978807551,12.893450842842,12.9893499098453,13.0898277925669,13.190163629574,
13.2903890484297,13.390540824841,13.4906480029083,13.590772326802,13.6575523118825),
 .UNSPECIFIED.);
#1203=B_SPLINE_CURVE_WITH_KNOTS('',3,(#28131,#28132,#28133,#28134,#28135,
#28136,#28137,#28138,#28139,#28140,#28141,#28142,#28143,#28144,#28145,#28146,
#28147,#28148,#28149,#28150,#28151,#28152,#28153,#28154,#28155,#28156,#28157,
#28158,#28159,#28160,#28161,#28162,#28163,#28164,#28165,#28166,#28167,#28168,
#28169,#28170,#28171,#28172,#28173,#28174,#28175,#28176,#28177,#28178,#28179,
#28180,#28181,#28182,#28183,#28184,#28185,#28186,#28187,#28188,#28189,#28190,
#28191,#28192,#28193,#28194,#28195,#28196,#28197,#28198,#28199,#28200,#28201,
#28202,#28203,#28204,#28205,#28206,#28207,#28208,#28209,#28210,#28211,#28212,
#28213,#28214,#28215,#28216,#28217,#28218,#28219,#28220,#28221,#28222,#28223,
#28224,#28225,#28226,#28227,#28228,#28229,#28230,#28231,#28232,#28233,#28234,
#28235,#28236,#28237,#28238,#28239,#28240,#28241,#28242,#28243,#28244,#28245,
#28246,#28247,#28248,#28249,#28250,#28251,#28252,#28253,#28254,#28255,#28256,
#28257,#28258,#28259,#28260,#28261,#28262,#28263,#28264,#28265,#28266,#28267,
#28268,#28269,#28270,#28271,#28272,#28273,#28274,#28275,#28276,#28277,#28278,
#28279,#28280,#28281,#28282,#28283,#28284,#28285,#28286,#28287,#28288,#28289,
#28290,#28291,#28292,#28293,#28294,#28295,#28296,#28297,#28298,#28299,#28300,
#28301,#28302,#28303,#28304,#28305,#28306,#28307,#28308,#28309,#28310,#28311,
#28312,#28313,#28314,#28315,#28316,#28317,#28318,#28319,#28320),
 .UNSPECIFIED.,.F.,.F.,(4,3,3,3,3,3,3,3,3,3,3,3,3,3,3,3,3,3,3,3,3,3,3,3,
3,3,3,3,3,3,3,3,3,3,3,3,3,3,3,3,3,3,3,3,3,3,3,3,3,3,3,3,3,3,3,3,3,3,3,3,
3,3,3,4),(13.6575523120968,13.774561329179,13.8928200570759,13.9885306721411,
14.089113174966,14.1895498660058,14.2898692687403,14.3901245196356,14.4903469678447,
14.590567921329,14.6908891188475,14.791258480304,14.8918113125242,14.9877114344369,
15.0882938735373,15.1887305005501,15.289049839111,15.3893050257722,15.4895274097768,
15.5897482991763,15.6900694332554,15.7904387315201,15.89099150173,15.9868921967327,
16.0874745927285,16.1879111756588,16.2882304688656,16.3884856094189,16.4887079466247,
16.5889287885971,16.6892498745856,16.7896191243191,16.8901718458187,16.9860729590285,
17.0866553946192,17.1870920177533,17.2874113518932,17.3876665338053,17.4878889127384,
17.5881097967499,17.6884309249752,17.7888002171228,17.8893529808349,17.9852537213243,
18.0858361462718,18.186272758679,18.2865920820166,18.3868472530856,18.4870696211499,
18.5872904942819,18.687611611688,18.7879808930314,18.8885336460944,18.9844344836201,
19.0843400792264,19.1841005133511,19.2837456873425,19.383328985701,19.4828826102244,
19.5824387231545,19.6820933266986,19.7818013921032,19.8816760023566,19.9407376187629),
 .UNSPECIFIED.);
#1204=B_SPLINE_CURVE_WITH_KNOTS('',3,(#28322,#28323,#28324,#28325,#28326,
#28327,#28328,#28329,#28330,#28331,#28332,#28333,#28334,#28335,#28336,#28337,
#28338,#28339,#28340,#28341,#28342,#28343,#28344,#28345,#28346,#28347,#28348,
#28349,#28350,#28351,#28352,#28353,#28354,#28355,#28356,#28357,#28358,#28359,
#28360,#28361,#28362,#28363,#28364,#28365,#28366,#28367,#28368,#28369,#28370,
#28371,#28372,#28373,#28374,#28375,#28376,#28377,#28378,#28379,#28380,#28381,
#28382,#28383,#28384,#28385,#28386,#28387,#28388,#28389,#28390,#28391,#28392,
#28393,#28394,#28395,#28396,#28397,#28398,#28399,#28400,#28401,#28402,#28403,
#28404,#28405,#28406,#28407,#28408,#28409,#28410,#28411,#28412,#28413,#28414,
#28415,#28416,#28417,#28418,#28419,#28420,#28421,#28422,#28423,#28424,#28425,
#28426,#28427,#28428,#28429,#28430,#28431,#28432,#28433,#28434,#28435,#28436,
#28437,#28438,#28439,#28440,#28441,#28442,#28443,#28444,#28445,#28446,#28447,
#28448,#28449,#28450,#28451,#28452,#28453,#28454,#28455,#28456,#28457,#28458,
#28459,#28460,#28461,#28462,#28463,#28464,#28465,#28466,#28467,#28468,#28469,
#28470,#28471,#28472,#28473,#28474,#28475,#28476,#28477,#28478,#28479,#28480,
#28481,#28482,#28483,#28484,#28485,#28486,#28487,#28488,#28489,#28490,#28491,
#28492,#28493,#28494,#28495,#28496,#28497,#28498,#28499,#28500,#28501,#28502,
#28503,#28504,#28505,#28506,#28507,#28508,#28509,#28510,#28511),
 .UNSPECIFIED.,.F.,.F.,(4,3,3,3,3,3,3,3,3,3,3,3,3,3,3,3,3,3,3,3,3,3,3,3,
3,3,3,3,3,3,3,3,3,3,3,3,3,3,3,3,3,3,3,3,3,3,3,3,3,3,3,3,3,3,3,3,3,3,3,3,
3,3,3,4),(19.9407376190621,19.9836152459159,20.0841976716306,20.1846342847766,
20.2849536088068,20.3852087805397,20.4854311492384,20.585652022974,20.6859731409308,
20.7863424227969,20.8868951763282,20.9827960082117,21.0833784322771,21.1838150437577,
21.2841343661058,21.3843895361473,21.4846119031475,21.5848327751802,21.6851538914387,
21.7855231716063,21.886075923459,21.9819767705075,22.0825591942063,22.1829958053088,
22.2833151272632,22.3835702969016,22.4837926634901,22.5840135351027,22.6843346509311,
22.7847039306623,22.8852566820731,22.9811575328033,23.0817399571192,23.1821765688491,
23.2824958914437,23.3827510617297,23.4829734289723,23.5831943012447,23.6835154177372,
23.783884698136,23.8844374502123,23.9803382950991,24.0809207191718,24.1813573306558,
24.2816766530015,24.381931823037,24.4821541900276,24.5823750620472,24.682696178287,
24.7830654584328,24.8836182102586,24.9795190573948,25.0801014814436,25.1805380929028,
25.2808574152219,25.3811125852299,25.4813349521921,25.5815558241822,25.6818769403915,
25.7822462205059,25.8827989722996,25.9786998196906,26.1100759682844,26.2239229259801),
 .UNSPECIFIED.);
#1205=B_SPLINE_CURVE_WITH_KNOTS('',3,(#28513,#28514,#28515,#28516,#28517,
#28518,#28519,#28520,#28521,#28522,#28523,#28524,#28525,#28526,#28527,#28528,
#28529,#28530,#28531,#28532,#28533,#28534,#28535,#28536,#28537,#28538,#28539,
#28540,#28541,#28542,#28543,#28544,#28545,#28546,#28547,#28548,#28549,#28550,
#28551,#28552,#28553,#28554,#28555,#28556,#28557,#28558,#28559,#28560,#28561,
#28562,#28563,#28564,#28565,#28566,#28567,#28568,#28569,#28570,#28571,#28572,
#28573,#28574,#28575,#28576,#28577,#28578,#28579,#28580,#28581,#28582,#28583,
#28584,#28585,#28586,#28587,#28588,#28589,#28590,#28591,#28592,#28593,#28594,
#28595,#28596,#28597,#28598,#28599,#28600,#28601,#28602,#28603,#28604,#28605,
#28606,#28607,#28608,#28609,#28610,#28611,#28612,#28613,#28614,#28615,#28616,
#28617,#28618,#28619,#28620,#28621,#28622,#28623,#28624,#28625,#28626,#28627,
#28628,#28629,#28630,#28631,#28632,#28633,#28634,#28635,#28636,#28637,#28638,
#28639,#28640,#28641,#28642,#28643,#28644,#28645,#28646,#28647,#28648,#28649,
#28650,#28651,#28652,#28653,#28654,#28655,#28656,#28657,#28658,#28659,#28660,
#28661,#28662,#28663,#28664,#28665,#28666,#28667,#28668,#28669,#28670,#28671,
#28672,#28673,#28674,#28675,#28676,#28677,#28678,#28679,#28680,#28681,#28682,
#28683,#28684,#28685,#28686,#28687,#28688,#28689,#28690,#28691,#28692,#28693,
#28694,#28695,#28696,#28697,#28698,#28699,#28700,#28701,#28702),
 .UNSPECIFIED.,.F.,.F.,(4,3,3,3,3,3,3,3,3,3,3,3,3,3,3,3,3,3,3,3,3,3,3,3,
3,3,3,3,3,3,3,3,3,3,3,3,3,3,3,3,3,3,3,3,3,3,3,3,3,3,3,3,3,3,3,3,3,3,3,3,
3,3,3,4),(26.2239229262416,26.3230559083015,26.4221251848231,26.5211634966858,
26.6202035420719,26.7193428737506,26.8185358680633,26.9178980737154,26.9778805819864,
27.0784630060752,27.1788996175751,27.2792189399362,27.3794741099869,27.4796964769925,
27.5799173490265,27.6802384652802,27.7806077454396,27.8811604972783,27.9770613442822,
28.077643768371,28.1780803798707,28.2783997022315,28.3786548722818,28.4788772392868,
28.5790981113202,28.6794192275731,28.7797885077316,28.8803412595694,28.976242106578,
29.0768245306755,29.1772611421844,29.2775804645544,29.3778356346138,29.4780580016284,
29.5782788736713,29.6785999899338,29.778969270102,29.8795220219494,29.9754228688738,
30.0760052929666,30.1764419044703,30.2767612268354,30.3770163968898,30.4772387638994,
30.5774596359376,30.6777807521952,30.7781500323582,30.8787027842006,30.9746036311696,
31.0751860552629,31.1756226667668,31.2759419891322,31.3761971591871,31.4764195261968,
31.5766403982353,31.676961514493,31.7773307946564,31.8778835464991,31.9737843934654,
32.0780783946679,32.1853358543562,32.2892156838711,32.3981619586461,32.5071082334212),
 .UNSPECIFIED.);
#1206=B_SPLINE_CURVE_WITH_KNOTS('',3,(#28704,#28705,#28706,#28707,#28708,
#28709,#28710,#28711,#28712,#28713,#28714,#28715,#28716,#28717,#28718,#28719,
#28720,#28721,#28722,#28723,#28724,#28725,#28726,#28727,#28728,#28729,#28730,
#28731,#28732,#28733,#28734,#28735,#28736,#28737,#28738,#28739,#28740,#28741,
#28742,#28743,#28744,#28745,#28746,#28747,#28748,#28749,#28750,#28751,#28752,
#28753,#28754,#28755,#28756,#28757,#28758,#28759,#28760,#28761,#28762,#28763,
#28764,#28765,#28766,#28767,#28768,#28769,#28770,#28771,#28772,#28773,#28774,
#28775,#28776,#28777,#28778,#28779,#28780,#28781,#28782,#28783,#28784,#28785,
#28786,#28787,#28788,#28789,#28790,#28791,#28792,#28793,#28794,#28795,#28796,
#28797,#28798,#28799,#28800,#28801,#28802,#28803,#28804,#28805,#28806,#28807,
#28808,#28809,#28810,#28811,#28812,#28813,#28814,#28815,#28816,#28817,#28818,
#28819,#28820,#28821,#28822,#28823,#28824,#28825,#28826,#28827,#28828,#28829,
#28830,#28831,#28832,#28833,#28834,#28835,#28836,#28837,#28838,#28839,#28840,
#28841,#28842,#28843,#28844,#28845,#28846,#28847,#28848,#28849,#28850,#28851,
#28852,#28853,#28854,#28855,#28856,#28857,#28858,#28859,#28860,#28861,#28862,
#28863,#28864,#28865,#28866,#28867,#28868,#28869,#28870,#28871,#28872,#28873,
#28874,#28875,#28876,#28877,#28878,#28879,#28880,#28881,#28882,#28883,#28884,
#28885,#28886,#28887,#28888,#28889,#28890,#28891,#28892,#28893,#28894,#28895,
#28896),.UNSPECIFIED.,.F.,.F.,(4,3,3,3,3,3,3,3,3,3,3,3,3,3,3,3,3,3,3,3,
3,3,3,3,3,3,3,3,3,3,3,3,3,3,3,3,3,3,3,3,3,3,3,3,3,3,3,3,3,3,3,3,3,3,3,3,
3,3,3,3,3,3,3,3,4),(32.5071082337745,32.6136854124345,32.7206393044122,
32.8277947974754,32.935264742081,32.9729651557612,33.0735475798547,33.1739841913593,
33.274303513725,33.3745586837803,33.4747810507904,33.575001922829,33.6753230390872,
33.775692319251,33.8762450710941,33.972145918057,34.0727283421507,34.1731649536554,
34.2734842760213,34.3737394460767,34.473961813087,34.5741826851257,34.6745038013841,
34.7748730815481,34.8754258333912,34.9713266803528,35.0719091044466,35.1723457159514,
35.2726650383175,35.372920208373,35.4731425753834,35.5733634474223,35.6736845636808,
35.7740538438449,35.8746065956882,35.9705074426486,36.0710898667423,36.1715264782471,
36.271845800613,36.3721009706685,36.4723233376788,36.5725442097176,36.672865325976,
36.77323460614,36.8737873579833,36.9696882049444,37.0702706290381,37.1707072405429,
37.2710265629088,37.3712817329643,37.4715040999747,37.5717249720135,37.6720460882719,
37.772415368436,37.8729681202792,37.9688689672402,38.0715470388752,38.1704609817843,
38.2692818278376,38.3680426710374,38.4667765229307,38.5655590052605,38.6643713321975,
38.7632960917447,38.7902935403205),.UNSPECIFIED.);
#1207=B_SPLINE_CURVE_WITH_KNOTS('',3,(#28898,#28899,#28900,#28901,#28902,
#28903,#28904,#28905,#28906,#28907,#28908,#28909,#28910,#28911,#28912,#28913,
#28914,#28915,#28916,#28917,#28918,#28919,#28920,#28921,#28922,#28923,#28924,
#28925,#28926,#28927,#28928,#28929,#28930,#28931,#28932,#28933,#28934,#28935,
#28936,#28937,#28938,#28939,#28940,#28941,#28942,#28943,#28944,#28945,#28946,
#28947,#28948,#28949,#28950,#28951,#28952,#28953,#28954,#28955,#28956,#28957,
#28958,#28959,#28960,#28961,#28962,#28963,#28964,#28965,#28966,#28967,#28968,
#28969,#28970,#28971,#28972,#28973,#28974,#28975,#28976,#28977,#28978,#28979,
#28980,#28981,#28982,#28983,#28984,#28985,#28986,#28987,#28988,#28989,#28990,
#28991,#28992,#28993,#28994,#28995,#28996,#28997,#28998,#28999,#29000,#29001,
#29002,#29003,#29004,#29005,#29006,#29007,#29008,#29009,#29010,#29011,#29012,
#29013,#29014,#29015,#29016,#29017,#29018,#29019,#29020,#29021,#29022,#29023,
#29024,#29025,#29026,#29027,#29028,#29029,#29030,#29031,#29032,#29033,#29034,
#29035,#29036,#29037,#29038,#29039,#29040,#29041,#29042,#29043,#29044,#29045,
#29046,#29047,#29048,#29049,#29050,#29051,#29052,#29053,#29054,#29055,#29056,
#29057,#29058,#29059,#29060,#29061,#29062,#29063,#29064,#29065,#29066,#29067,
#29068,#29069,#29070,#29071,#29072,#29073,#29074,#29075,#29076,#29077,#29078,
#29079,#29080,#29081,#29082,#29083,#29084,#29085,#29086,#29087),
 .UNSPECIFIED.,.F.,.F.,(4,3,3,3,3,3,3,3,3,3,3,3,3,3,3,3,3,3,3,3,3,3,3,3,
3,3,3,3,3,3,3,3,3,3,3,3,3,3,3,3,3,3,3,3,3,3,3,3,3,3,3,3,3,3,3,3,3,3,3,3,
3,3,3,4),(38.7902935406008,38.9439982042354,38.968049729536,39.0686321536296,
39.1690687651342,39.2693880875,39.3696432575553,39.4698656245654,39.5700864966042,
39.6704076128624,39.7707768930262,39.8713296448693,39.9672304918318,40.0678129159255,
40.1682495274303,40.2685688497962,40.3688240198517,40.469046386862,40.5692672589008,
40.6695883751592,40.7699576553232,40.8705104071664,40.9664112541276,41.0669936782214,
41.1674302897262,41.2677496120922,41.3680047821478,41.4682271491582,41.5684480211971,
41.6687691374555,41.7691384176196,41.8696911694629,41.9655920164233,42.0661744405169,
42.1666110520216,42.2669303743875,42.3671855444429,42.4674079114532,42.567628783492,
42.6679498997503,42.7683191799143,42.8688719317574,42.9647727787191,43.0653552028129,
43.1657918143178,43.2661111366838,43.3663663067393,43.4665886737497,43.5668095457887,
43.6671306620471,43.7674999422112,43.8680526940545,43.9639535410149,44.0645359651086,
44.1649725766133,44.2652918989792,44.3655470690347,44.465769436045,44.5659903080837,
44.6663114243421,44.7666807045061,44.8672334563492,44.9631343033107,45.0734788477804),
 .UNSPECIFIED.);
#1208=B_SPLINE_CURVE_WITH_KNOTS('',3,(#29089,#29090,#29091,#29092,#29093,
#29094,#29095,#29096,#29097,#29098,#29099,#29100,#29101,#29102,#29103,#29104,
#29105,#29106,#29107,#29108,#29109,#29110,#29111,#29112,#29113,#29114,#29115,
#29116,#29117,#29118,#29119,#29120,#29121,#29122,#29123,#29124,#29125,#29126,
#29127,#29128,#29129,#29130,#29131,#29132,#29133,#29134,#29135,#29136,#29137,
#29138,#29139,#29140,#29141,#29142,#29143,#29144,#29145,#29146,#29147,#29148,
#29149,#29150,#29151,#29152,#29153,#29154,#29155,#29156,#29157,#29158,#29159,
#29160,#29161,#29162,#29163,#29164,#29165,#29166,#29167,#29168,#29169,#29170,
#29171,#29172,#29173,#29174,#29175,#29176,#29177,#29178,#29179,#29180,#29181,
#29182,#29183,#29184,#29185,#29186,#29187,#29188,#29189,#29190,#29191,#29192,
#29193,#29194,#29195,#29196,#29197,#29198,#29199,#29200,#29201,#29202,#29203,
#29204,#29205,#29206,#29207,#29208,#29209,#29210,#29211,#29212,#29213,#29214,
#29215,#29216,#29217,#29218,#29219,#29220,#29221,#29222,#29223,#29224,#29225,
#29226,#29227,#29228,#29229,#29230,#29231,#29232,#29233,#29234,#29235,#29236,
#29237,#29238,#29239,#29240,#29241,#29242,#29243,#29244,#29245,#29246,#29247,
#29248,#29249,#29250,#29251,#29252,#29253,#29254,#29255,#29256,#29257,#29258,
#29259,#29260,#29261,#29262,#29263,#29264,#29265,#29266,#29267,#29268,#29269,
#29270,#29271,#29272,#29273,#29274,#29275,#29276,#29277,#29278),
 .UNSPECIFIED.,.F.,.F.,(4,3,3,3,3,3,3,3,3,3,3,3,3,3,3,3,3,3,3,3,3,3,3,3,
3,3,3,3,3,3,3,3,3,3,3,3,3,3,3,3,3,3,3,3,3,3,3,3,3,3,3,3,3,3,3,3,3,3,3,3,
3,3,3,4),(45.0734788480091,45.1726643676828,45.2717096259563,45.3706772508578,
45.4696001387515,45.5685111265611,45.6675114574198,45.7665534619267,45.8657746186064,
45.9623150656065,46.0628974897002,46.1633341012049,46.2636534235708,46.3639085936263,
46.4641309606367,46.5643518326753,46.6646729489337,46.7650422290977,46.8655949809409,
46.9614958279023,47.062078251996,47.1625148635009,47.2628341858669,47.3630893559225,
47.4633117229327,47.5635325949716,47.6638537112301,47.764222991394,47.8647757432373,
47.9606765901981,48.0612590142918,48.1616956257966,48.2620149481625,48.3622701182179,
48.4624924852283,48.562713357267,48.6630344735255,48.7634037536895,48.8639565055327,
48.9598573524939,49.0604397765875,49.1608763880926,49.2611957104586,49.3614508805141,
49.4616732475243,49.5618941195634,49.6622152358218,49.7625845159858,49.863137267829,
49.9590381147897,50.0596205388833,50.1600571503878,50.2603764727537,50.3606316428091,
50.4608540098193,50.5610748818582,50.6613959981166,50.7617652782805,50.8623180301237,
50.9582188770855,51.070080858906,51.181585042824,51.2924809446677,51.3566641547469),
 .UNSPECIFIED.);
#1209=B_SPLINE_CURVE_WITH_KNOTS('',3,(#29280,#29281,#29282,#29283,#29284,
#29285,#29286,#29287,#29288,#29289,#29290,#29291,#29292,#29293,#29294,#29295,
#29296,#29297,#29298,#29299,#29300,#29301,#29302,#29303,#29304,#29305,#29306,
#29307,#29308,#29309,#29310,#29311,#29312,#29313,#29314,#29315,#29316,#29317,
#29318,#29319,#29320,#29321,#29322,#29323,#29324,#29325,#29326,#29327,#29328,
#29329,#29330,#29331,#29332,#29333,#29334,#29335,#29336,#29337,#29338,#29339,
#29340,#29341,#29342,#29343,#29344,#29345,#29346,#29347,#29348,#29349,#29350,
#29351,#29352,#29353,#29354,#29355,#29356,#29357,#29358,#29359,#29360,#29361,
#29362,#29363,#29364,#29365,#29366,#29367,#29368,#29369,#29370,#29371,#29372,
#29373,#29374,#29375,#29376,#29377,#29378,#29379,#29380,#29381,#29382,#29383,
#29384,#29385,#29386,#29387,#29388,#29389,#29390,#29391,#29392,#29393,#29394,
#29395,#29396,#29397,#29398,#29399,#29400,#29401,#29402,#29403,#29404,#29405,
#29406,#29407,#29408,#29409,#29410,#29411,#29412,#29413,#29414,#29415,#29416,
#29417,#29418,#29419,#29420,#29421,#29422,#29423,#29424,#29425,#29426,#29427,
#29428,#29429,#29430,#29431,#29432,#29433,#29434,#29435,#29436,#29437,#29438,
#29439,#29440,#29441,#29442,#29443,#29444,#29445,#29446,#29447,#29448,#29449,
#29450,#29451,#29452,#29453,#29454,#29455,#29456,#29457,#29458,#29459,#29460,
#29461,#29462,#29463,#29464,#29465,#29466,#29467,#29468,#29469),
 .UNSPECIFIED.,.F.,.F.,(4,3,3,3,3,3,3,3,3,3,3,3,3,3,3,3,3,3,3,3,3,3,3,3,
3,3,3,3,3,3,3,3,3,3,3,3,3,3,3,3,3,3,3,3,3,3,3,3,3,3,3,3,3,3,3,3,3,3,3,3,
3,3,3,4),(51.35666415496,51.4582046051034,51.5597783328067,51.6614969549953,
51.7632886368995,51.8652929421708,51.9573996393813,52.057982063475,52.1584186749796,
52.2587379973455,52.3589931674009,52.4592155344113,52.5594364064501,52.6597575227085,
52.7601268028724,52.8606795547156,52.9565804016771,53.0571628257708,53.1575994372756,
53.2579187596415,53.358173929697,53.4583962967073,53.5586171687462,53.6589382850046,
53.7593075651686,53.8598603170118,53.9557611639729,54.0563435880666,54.1567801995714,
54.2570995219374,54.3573546919928,54.4575770590032,54.5577979310419,54.6581190473004,
54.7584883274645,54.8590410793077,54.9549419262687,55.0555243503623,55.1559609618672,
55.2562802842331,55.3565354542886,55.456757821299,55.556978693338,55.6572998095964,
55.7576690897604,55.8582218416037,55.9541226885645,56.0547051126583,56.1551417241628,
56.2554610465287,56.3557162165841,56.4559385835944,56.556159455633,56.6564805718914,
56.7568498520554,56.8574026038986,56.9533034508602,57.053466577448,57.1534907762757,
57.2534080991903,57.3532611161024,57.4530730259249,57.5529179342892,57.6398494621396),
 .UNSPECIFIED.);
#1210=B_SPLINE_CURVE_WITH_KNOTS('',3,(#29471,#29472,#29473,#29474,#29475,
#29476,#29477,#29478,#29479,#29480,#29481,#29482,#29483,#29484,#29485,#29486,
#29487,#29488,#29489,#29490,#29491,#29492,#29493,#29494,#29495,#29496,#29497,
#29498,#29499,#29500,#29501,#29502,#29503,#29504,#29505,#29506,#29507,#29508,
#29509,#29510,#29511,#29512,#29513,#29514,#29515,#29516,#29517,#29518,#29519,
#29520,#29521,#29522,#29523,#29524,#29525,#29526,#29527,#29528,#29529,#29530,
#29531,#29532,#29533,#29534,#29535,#29536,#29537,#29538,#29539,#29540,#29541,
#29542,#29543,#29544,#29545,#29546,#29547,#29548,#29549,#29550,#29551,#29552,
#29553,#29554,#29555,#29556,#29557,#29558,#29559,#29560,#29561,#29562,#29563,
#29564,#29565,#29566,#29567,#29568,#29569,#29570,#29571,#29572,#29573,#29574,
#29575,#29576,#29577,#29578,#29579,#29580,#29581,#29582,#29583,#29584,#29585,
#29586,#29587,#29588,#29589,#29590,#29591,#29592,#29593,#29594,#29595,#29596,
#29597,#29598,#29599,#29600,#29601,#29602,#29603,#29604,#29605,#29606,#29607,
#29608,#29609,#29610,#29611,#29612,#29613,#29614,#29615,#29616,#29617,#29618,
#29619,#29620,#29621,#29622,#29623,#29624,#29625,#29626,#29627,#29628,#29629,
#29630,#29631,#29632,#29633,#29634,#29635,#29636,#29637,#29638,#29639,#29640,
#29641,#29642,#29643,#29644,#29645,#29646,#29647,#29648,#29649,#29650,#29651,
#29652,#29653,#29654,#29655,#29656,#29657,#29658,#29659,#29660),
 .UNSPECIFIED.,.F.,.F.,(4,3,3,3,3,3,3,3,3,3,3,3,3,3,3,3,3,3,3,3,3,3,3,3,
3,3,3,3,3,3,3,3,3,3,3,3,3,3,3,3,3,3,3,3,3,3,3,3,3,3,3,3,3,3,3,3,3,3,3,3,
3,3,3,4),(57.6398494625214,57.7589701131946,57.8795801756191,57.9524842131561,
58.0530666372499,58.1535032487546,58.2538225711206,58.354077741176,58.4543001081864,
58.5545209802252,58.6548420964837,58.7552113766477,58.855764128491,58.9516649754518,
59.0522473995455,59.1526840110503,59.2530033334162,59.3532585034717,59.4534808704821,
59.553701742521,59.6540228587794,59.7543921389434,59.8549448907867,59.9508457377476,
60.0514281618413,60.1518647733461,60.252184095712,60.3524392657675,60.4526616327778,
60.5528825048166,60.653203621075,60.753572901239,60.8541256530822,60.9500265000434,
61.0506089241371,61.1510455356419,61.2513648580079,61.3516200280634,61.4518423950738,
61.5520632671126,61.652384383371,61.752753663535,61.8533064153783,61.9492072623392,
62.0497896864329,62.1502262979376,62.2505456203036,62.3508007903591,62.4510231573694,
62.5512440294082,62.6515651456666,62.7519344258307,62.8524871776739,62.948388024635,
63.0485570779958,63.1485806798993,63.2484883191134,63.3483332353989,63.4481473208821,
63.5479624276795,63.6478773952426,63.7478438550818,63.8479848096707,63.9230347689432),
 .UNSPECIFIED.);
#1211=B_SPLINE_CURVE_WITH_KNOTS('',3,(#29662,#29663,#29664,#29665,#29666,
#29667,#29668,#29669,#29670,#29671,#29672,#29673,#29674,#29675,#29676,#29677,
#29678,#29679,#29680,#29681,#29682,#29683,#29684,#29685,#29686,#29687,#29688,
#29689,#29690,#29691,#29692,#29693,#29694,#29695,#29696,#29697,#29698,#29699,
#29700,#29701,#29702,#29703,#29704,#29705,#29706,#29707,#29708,#29709,#29710,
#29711,#29712,#29713,#29714,#29715,#29716,#29717,#29718,#29719,#29720,#29721,
#29722,#29723,#29724,#29725,#29726,#29727,#29728,#29729,#29730,#29731,#29732,
#29733,#29734,#29735,#29736,#29737,#29738,#29739,#29740,#29741,#29742,#29743,
#29744,#29745,#29746,#29747,#29748,#29749,#29750,#29751,#29752,#29753,#29754,
#29755,#29756,#29757,#29758,#29759,#29760,#29761,#29762,#29763,#29764,#29765,
#29766,#29767,#29768,#29769,#29770,#29771,#29772,#29773,#29774,#29775,#29776,
#29777,#29778,#29779,#29780,#29781,#29782,#29783,#29784,#29785,#29786,#29787,
#29788,#29789,#29790,#29791,#29792,#29793,#29794,#29795,#29796,#29797,#29798,
#29799,#29800,#29801,#29802,#29803,#29804,#29805,#29806,#29807,#29808,#29809,
#29810,#29811,#29812,#29813,#29814,#29815,#29816,#29817,#29818,#29819,#29820,
#29821,#29822,#29823,#29824,#29825,#29826,#29827,#29828,#29829,#29830,#29831,
#29832,#29833,#29834,#29835,#29836,#29837,#29838,#29839,#29840,#29841,#29842,
#29843,#29844,#29845,#29846,#29847,#29848,#29849,#29850,#29851),
 .UNSPECIFIED.,.F.,.F.,(4,3,3,3,3,3,3,3,3,3,3,3,3,3,3,3,3,3,3,3,3,3,3,3,
3,3,3,3,3,3,3,3,3,3,3,3,3,3,3,3,3,3,3,3,3,3,3,3,3,3,3,3,3,3,3,3,3,3,3,3,
3,3,3,4),(63.9230347693192,63.9475687869308,64.0481512110245,64.1485878225294,
64.2489071448954,64.3491623149509,64.4493846819612,64.5496055540001,64.6499266702586,
64.7502959504226,64.8508487022659,64.9467495492266,65.0473319733203,65.1477685848251,
65.248087907191,65.3483430772466,65.448565444257,65.5487863162958,65.6491074325543,
65.7494767127183,65.8500294645616,65.9459303115224,66.0465127356161,66.1469493471208,
66.2472686694868,66.3475238395422,66.4477462065526,66.5479670785914,66.6482881948498,
66.7486574750138,66.849210226857,66.9451110738182,67.0456934979119,67.1461301094167,
67.2464494317826,67.3467046018381,67.4469269688484,67.5471478408872,67.6474689571456,
67.7478382373096,67.8483909891528,67.944291836114,68.0448742602077,68.1453108717125,
68.2456301940785,68.345885364134,68.4461077311443,68.5463286031831,68.6466497194415,
68.7470189996055,68.8475717514488,68.9434725984098,69.0440550225035,69.1444916340084,
69.2448109563743,69.3450661264298,69.4452884934402,69.5455093654791,69.6458304817376,
69.7461997619017,69.8467525137449,69.9426533607056,70.0744367184332,70.2062200761607),
 .UNSPECIFIED.);
#1212=B_SPLINE_CURVE_WITH_KNOTS('',3,(#29853,#29854,#29855,#29856,#29857,
#29858,#29859,#29860,#29861,#29862,#29863,#29864,#29865,#29866,#29867,#29868,
#29869,#29870,#29871,#29872,#29873,#29874,#29875,#29876,#29877,#29878,#29879,
#29880,#29881,#29882,#29883,#29884,#29885,#29886,#29887,#29888,#29889,#29890,
#29891,#29892,#29893,#29894,#29895,#29896,#29897,#29898,#29899,#29900,#29901,
#29902,#29903,#29904,#29905,#29906,#29907,#29908,#29909,#29910,#29911,#29912,
#29913,#29914,#29915,#29916,#29917,#29918,#29919,#29920,#29921,#29922,#29923,
#29924,#29925,#29926,#29927,#29928,#29929,#29930,#29931,#29932,#29933,#29934,
#29935,#29936,#29937,#29938,#29939,#29940,#29941,#29942,#29943,#29944,#29945,
#29946,#29947,#29948,#29949,#29950,#29951,#29952,#29953,#29954,#29955,#29956,
#29957,#29958,#29959,#29960,#29961,#29962,#29963,#29964,#29965,#29966,#29967,
#29968,#29969,#29970,#29971,#29972,#29973,#29974,#29975,#29976,#29977,#29978,
#29979,#29980,#29981,#29982,#29983,#29984,#29985,#29986,#29987,#29988,#29989,
#29990,#29991,#29992,#29993,#29994,#29995,#29996,#29997,#29998,#29999,#30000,
#30001,#30002,#30003,#30004,#30005,#30006,#30007,#30008,#30009,#30010,#30011,
#30012,#30013,#30014,#30015,#30016,#30017,#30018,#30019,#30020,#30021,#30022,
#30023,#30024,#30025,#30026,#30027,#30028,#30029,#30030,#30031,#30032,#30033,
#30034,#30035,#30036,#30037,#30038,#30039,#30040,#30041,#30042,#30043,#30044,
#30045),.UNSPECIFIED.,.F.,.F.,(4,3,3,3,3,3,3,3,3,3,3,3,3,3,3,3,3,3,3,3,
3,3,3,3,3,3,3,3,3,3,3,3,3,3,3,3,3,3,3,3,3,3,3,3,3,3,3,3,3,3,3,3,3,3,3,3,
3,3,3,3,3,3,3,3,4),(70.2062200764988,70.305495551724,70.4047158033365,70.503913389098,
70.6031208337801,70.7024336389929,70.8018070712722,70.9013453472432,70.9418341230014,
71.0424165470951,71.1428531586,71.243172480966,71.3434276510215,71.4436500180318,
71.5438708900706,71.644192006329,71.744561286493,71.8451140383363,71.9410148852972,
72.0415973093909,72.1420339208956,72.2423532432615,72.3426084133169,72.4428307803273,
72.5430516523662,72.6433727686245,72.7437420487885,72.8442948006317,72.9401956475929,
73.0407780716866,73.1412146831914,73.2415340055574,73.3417891756129,73.4420115426231,
73.5422324146621,73.6425535309205,73.7429228110844,73.8434755629275,73.9393764098887,
74.0399588339824,74.1403954454876,74.2407147678536,74.340969937909,74.4411923049193,
74.5414131769583,74.6417342932166,74.7421035733806,74.8426563252239,74.9385571721845,
75.0391395962781,75.139576207783,75.239895530149,75.3401507002046,75.440373067215,
75.5405939392537,75.6409150555122,75.7412843356761,75.8418370875194,75.9377379344803,
76.0413335477396,76.1447484660192,76.247965445848,76.3510651505503,76.4540511721591,
76.4894053836784),.UNSPECIFIED.);
#1213=B_SPLINE_CURVE_WITH_KNOTS('',3,(#30047,#30048,#30049,#30050,#30051,
#30052,#30053,#30054,#30055,#30056,#30057,#30058,#30059,#30060,#30061,#30062,
#30063,#30064,#30065,#30066,#30067,#30068,#30069,#30070,#30071,#30072,#30073,
#30074,#30075,#30076,#30077,#30078,#30079,#30080,#30081,#30082,#30083,#30084,
#30085,#30086,#30087,#30088,#30089,#30090,#30091,#30092,#30093,#30094,#30095,
#30096,#30097,#30098,#30099,#30100,#30101,#30102,#30103,#30104,#30105,#30106,
#30107,#30108,#30109,#30110,#30111,#30112,#30113,#30114,#30115,#30116,#30117,
#30118,#30119,#30120,#30121,#30122,#30123,#30124,#30125,#30126,#30127,#30128,
#30129,#30130,#30131,#30132,#30133,#30134,#30135,#30136,#30137,#30138,#30139,
#30140,#30141,#30142,#30143,#30144,#30145,#30146,#30147,#30148,#30149,#30150,
#30151,#30152,#30153,#30154,#30155,#30156,#30157,#30158,#30159,#30160,#30161,
#30162,#30163,#30164,#30165,#30166,#30167,#30168,#30169,#30170,#30171,#30172,
#30173,#30174,#30175,#30176,#30177,#30178,#30179,#30180,#30181,#30182,#30183,
#30184,#30185,#30186,#30187,#30188,#30189,#30190,#30191,#30192,#30193,#30194,
#30195,#30196,#30197,#30198,#30199,#30200,#30201,#30202,#30203,#30204,#30205,
#30206,#30207,#30208,#30209,#30210,#30211,#30212,#30213,#30214,#30215,#30216,
#30217,#30218,#30219,#30220,#30221,#30222,#30223,#30224,#30225,#30226,#30227,
#30228,#30229,#30230,#30231,#30232,#30233,#30234,#30235,#30236),
 .UNSPECIFIED.,.F.,.F.,(4,3,3,3,3,3,3,3,3,3,3,3,3,3,3,3,3,3,3,3,3,3,3,3,
3,3,3,3,3,3,3,3,3,3,3,3,3,3,3,3,3,3,3,3,3,3,3,3,3,3,3,3,3,3,3,3,3,3,3,3,
3,3,3,4),(76.4894053839406,76.6012837121495,76.7092937118267,76.8231062043014,
76.9369186967761,77.0375011208698,77.1379377323746,77.2382570547405,77.338512224796,
77.4387345918064,77.5389554638453,77.6392765801037,77.7396458602678,77.840198612111,
77.9360994590719,78.0366818831656,78.1371184946705,78.2374378170365,78.337692987092,
78.4379153541024,78.5381362261413,78.6384573423997,78.7388266225638,78.8393793744071,
78.9352802213677,79.0358626454614,79.1362992569661,79.2366185793321,79.3368737493875,
79.4370961163978,79.5373169884366,79.637638104695,79.7380073848589,79.8385601367021,
79.9344609836635,80.0350434077572,80.135480019262,80.235799341628,80.3360545116835,
80.4362768786938,80.5364977507326,80.636818866991,80.737188147155,80.8377408989983,
80.9336417459593,81.0342241700531,81.1346607815578,81.2349801039237,81.3352352739792,
81.4354576409896,81.5356785130284,81.6359996292869,81.7363689094508,81.8369216612941,
81.9328225082551,82.0319079799504,82.130826023152,82.229650296528,82.3284138954426,
82.427149832368,82.5259386101351,82.6247563736218,82.723698889131,82.7725906905032),
 .UNSPECIFIED.);
#1214=B_SPLINE_CURVE_WITH_KNOTS('',3,(#30238,#30239,#30240,#30241,#30242,
#30243,#30244,#30245,#30246,#30247,#30248,#30249,#30250,#30251,#30252,#30253,
#30254,#30255,#30256,#30257,#30258,#30259,#30260,#30261,#30262,#30263,#30264,
#30265,#30266,#30267,#30268,#30269,#30270,#30271,#30272,#30273,#30274,#30275,
#30276,#30277,#30278,#30279,#30280,#30281,#30282,#30283,#30284,#30285,#30286,
#30287,#30288,#30289,#30290,#30291,#30292,#30293,#30294,#30295,#30296,#30297,
#30298,#30299,#30300,#30301,#30302,#30303,#30304,#30305,#30306,#30307,#30308,
#30309,#30310,#30311,#30312,#30313,#30314,#30315,#30316,#30317,#30318,#30319,
#30320,#30321,#30322,#30323,#30324,#30325,#30326,#30327,#30328,#30329,#30330,
#30331,#30332,#30333,#30334,#30335,#30336,#30337,#30338,#30339,#30340,#30341,
#30342,#30343,#30344,#30345,#30346,#30347,#30348,#30349,#30350,#30351,#30352,
#30353,#30354,#30355,#30356,#30357,#30358,#30359,#30360,#30361,#30362,#30363,
#30364,#30365,#30366,#30367,#30368,#30369,#30370,#30371,#30372,#30373,#30374,
#30375,#30376,#30377,#30378,#30379,#30380,#30381,#30382,#30383,#30384,#30385,
#30386,#30387,#30388,#30389,#30390,#30391,#30392,#30393,#30394,#30395,#30396,
#30397,#30398,#30399,#30400,#30401,#30402,#30403,#30404,#30405,#30406,#30407,
#30408,#30409,#30410,#30411,#30412,#30413,#30414,#30415,#30416,#30417,#30418,
#30419,#30420,#30421,#30422,#30423,#30424),.UNSPECIFIED.,.F.,.F.,(4,3,3,
3,3,3,3,3,3,3,3,3,3,3,3,3,3,3,3,3,3,3,3,3,3,3,3,3,3,3,3,3,3,3,3,3,3,3,3,
3,3,3,3,3,3,3,3,3,3,3,3,3,3,3,3,3,3,3,3,3,3,3,4),(82.772590690858,82.9320032705509,
83.0325856946445,83.1330223061491,83.2333416285149,83.3335967985702,83.4338191655803,
83.5340400376191,83.6343611538773,83.7347304340412,83.8352831858843,83.9311840328467,
84.0317664569405,84.1322030684453,84.2325223908113,84.3327775608669,84.4329999278774,
84.5332207999163,84.6335419161747,84.7339111963388,84.8344639481822,84.9303647951425,
85.0309472192362,85.131383830741,85.231703153107,85.3319583231625,85.4321806901728,
85.5324015622116,85.63272267847,85.733091958634,85.8336447104773,85.9295455574383,
86.0301279815319,86.1305645930366,86.2308839154025,86.3311390854579,86.4313614524681,
86.5315823245069,86.6319034407652,86.7322727209291,86.8328254727723,86.9287263197341,
87.0293087438279,87.1297453553328,87.2300646776988,87.3303198477544,87.4305422147649,
87.5307630868038,87.6310842030623,87.7314534832264,87.8320062350697,87.9279070820299,
88.0284895061235,88.1289261176283,88.2292454399941,88.3295006100496,88.4297229770599,
88.5299438490986,88.6302649653569,88.7306342455209,88.8311869973641,88.9270878443257,
89.0557759980376),.UNSPECIFIED.);
#1215=B_SPLINE_CURVE_WITH_KNOTS('',3,(#30426,#30427,#30428,#30429,#30430,
#30431,#30432,#30433,#30434,#30435,#30436,#30437,#30438,#30439,#30440,#30441,
#30442,#30443,#30444,#30445,#30446,#30447,#30448,#30449,#30450,#30451,#30452,
#30453,#30454,#30455,#30456,#30457,#30458,#30459,#30460,#30461,#30462,#30463,
#30464,#30465,#30466,#30467,#30468,#30469,#30470,#30471,#30472,#30473,#30474,
#30475,#30476,#30477,#30478,#30479,#30480,#30481,#30482,#30483,#30484,#30485,
#30486,#30487,#30488,#30489,#30490,#30491,#30492,#30493,#30494,#30495,#30496,
#30497,#30498,#30499,#30500,#30501,#30502,#30503,#30504,#30505,#30506,#30507,
#30508,#30509,#30510,#30511,#30512,#30513,#30514,#30515,#30516,#30517,#30518,
#30519,#30520,#30521,#30522,#30523,#30524,#30525,#30526,#30527,#30528,#30529,
#30530,#30531,#30532,#30533,#30534,#30535,#30536,#30537,#30538,#30539,#30540,
#30541,#30542,#30543,#30544,#30545,#30546,#30547,#30548,#30549,#30550,#30551,
#30552,#30553,#30554,#30555,#30556,#30557,#30558,#30559,#30560,#30561,#30562,
#30563,#30564,#30565,#30566,#30567,#30568,#30569,#30570,#30571,#30572,#30573,
#30574,#30575,#30576,#30577,#30578,#30579,#30580,#30581,#30582,#30583,#30584,
#30585,#30586,#30587,#30588,#30589,#30590,#30591,#30592,#30593,#30594,#30595,
#30596,#30597,#30598,#30599,#30600,#30601,#30602,#30603,#30604,#30605,#30606,
#30607,#30608,#30609,#30610,#30611,#30612,#30613,#30614,#30615),
 .UNSPECIFIED.,.F.,.F.,(4,3,3,3,3,3,3,3,3,3,3,3,3,3,3,3,3,3,3,3,3,3,3,3,
3,3,3,3,3,3,3,3,3,3,3,3,3,3,3,3,3,3,3,3,3,3,3,3,3,3,3,3,3,3,3,3,3,3,3,3,
3,3,3,4),(89.0557759982561,89.1548478356137,89.2537870669335,89.3526536190256,
89.4514804608427,89.550300507013,89.6492130022719,89.7481719107378,89.8473039942485,
89.9262686066214,90.0268510307156,90.1272876422209,90.2276069645874,90.3278621346434,
90.4280845016543,90.5283053736936,90.6286264899526,90.7289957701171,90.8295485219609,
90.9254493689172,91.0260317930103,91.1264684045144,91.2267877268798,91.3270428969347,
91.4272652639444,91.5274861359828,91.6278072522406,91.728176532404,91.8287292842468,
91.924630131213,92.0252125553059,92.1256491668097,92.2259684891748,92.3262236592295,
92.426446026239,92.5266668982769,92.6269880145345,92.7273572946976,92.82791004654,
92.9238108935088,93.0243933176066,93.1248299291159,93.2251492514859,93.3254044215455,
93.42562678856,93.525847660603,93.6261687768654,93.7265380570335,93.8270908088807,
93.9229916558046,94.0235740798929,94.1240106913923,94.2243300137529,94.324585183803,
94.4248075508081,94.5250284228413,94.6253495390945,94.7257188192534,94.8262715710917,
94.9221724181004,95.0326493234279,95.1428149119553,95.2524554430212,95.3389613048398),
 .UNSPECIFIED.);
#1216=B_SPLINE_CURVE_WITH_KNOTS('',3,(#30617,#30618,#30619,#30620,#30621,
#30622,#30623,#30624,#30625,#30626,#30627,#30628,#30629,#30630,#30631,#30632,
#30633,#30634,#30635,#30636,#30637,#30638,#30639,#30640,#30641,#30642,#30643,
#30644,#30645,#30646,#30647,#30648,#30649,#30650,#30651,#30652,#30653,#30654,
#30655,#30656,#30657,#30658,#30659,#30660,#30661,#30662,#30663,#30664,#30665,
#30666,#30667,#30668,#30669,#30670,#30671,#30672,#30673,#30674,#30675,#30676,
#30677,#30678,#30679,#30680,#30681,#30682,#30683,#30684,#30685,#30686,#30687,
#30688,#30689,#30690,#30691,#30692,#30693,#30694,#30695,#30696,#30697,#30698,
#30699,#30700,#30701,#30702,#30703,#30704,#30705,#30706,#30707,#30708,#30709,
#30710,#30711,#30712,#30713,#30714,#30715,#30716,#30717,#30718,#30719,#30720,
#30721,#30722,#30723,#30724,#30725,#30726,#30727,#30728,#30729,#30730,#30731,
#30732,#30733,#30734,#30735,#30736,#30737,#30738,#30739,#30740,#30741,#30742,
#30743,#30744,#30745,#30746,#30747,#30748,#30749,#30750,#30751,#30752,#30753,
#30754,#30755,#30756,#30757,#30758,#30759,#30760,#30761,#30762,#30763,#30764,
#30765,#30766,#30767,#30768,#30769,#30770,#30771,#30772,#30773,#30774,#30775,
#30776,#30777,#30778,#30779,#30780,#30781,#30782,#30783,#30784,#30785,#30786,
#30787,#30788,#30789,#30790,#30791,#30792,#30793,#30794,#30795,#30796,#30797,
#30798,#30799,#30800,#30801,#30802,#30803,#30804,#30805,#30806),
 .UNSPECIFIED.,.F.,.F.,(4,3,3,3,3,3,3,3,3,3,3,3,3,3,3,3,3,3,3,3,3,3,3,3,
3,3,3,3,3,3,3,3,3,3,3,3,3,3,3,3,3,3,3,3,3,3,3,3,3,3,3,3,3,3,3,3,3,3,3,3,
3,3,3,4),(95.3389613052171,95.4409974933841,95.5430847052396,95.6453339618529,
95.7476693299862,95.8502180918647,95.9213531803962,96.0219356045212,96.1223722160572,
96.2226915384546,96.3229467085413,96.4231690755829,96.5233899476529,96.6237110639422,
96.7240803441367,96.8246330960099,96.920533942692,97.0211163667362,97.1215529781915,
97.2218723005085,97.3221274705153,97.4223498374773,97.5225707094681,97.6228918256795,
97.723261105797,97.823813857595,97.9197147049878,98.0202971290644,98.1207337405514,
98.2210530628988,98.3213082329353,98.4215305999262,98.521751471945,98.6220725881831,
98.7224418683265,98.8229946201489,98.9188954672836,99.0194778916097,99.1199145033476,
99.2202338259468,99.3204889962355,99.4207113634785,99.5209322357496,99.6212533522374,
99.7216226326296,99.8221753846965,99.9180762295794,100.018658653241,100.119095264314,
100.219414586251,100.31966975588,100.419892122466,100.520112994084,100.62043410993,
100.720803389684,100.821356141129,100.917256991875,101.017146774421,101.116900249328,
101.216549802348,101.31794900486,101.417504245207,101.519825428802,101.622146612397),
 .UNSPECIFIED.);
#1217=B_SPLINE_CURVE_WITH_KNOTS('',3,(#30808,#30809,#30810,#30811,#30812,
#30813,#30814,#30815,#30816,#30817,#30818,#30819,#30820,#30821,#30822,#30823,
#30824,#30825,#30826,#30827,#30828,#30829,#30830,#30831,#30832,#30833,#30834,
#30835,#30836,#30837,#30838,#30839,#30840,#30841,#30842,#30843,#30844,#30845,
#30846,#30847,#30848,#30849,#30850,#30851,#30852,#30853,#30854,#30855,#30856,
#30857,#30858,#30859,#30860,#30861,#30862,#30863,#30864,#30865,#30866,#30867,
#30868,#30869,#30870,#30871,#30872,#30873,#30874,#30875,#30876,#30877,#30878,
#30879,#30880,#30881,#30882,#30883,#30884,#30885,#30886,#30887,#30888,#30889,
#30890,#30891,#30892,#30893,#30894,#30895,#30896,#30897,#30898,#30899,#30900,
#30901,#30902,#30903,#30904,#30905,#30906,#30907,#30908,#30909,#30910,#30911,
#30912,#30913,#30914,#30915,#30916,#30917,#30918,#30919,#30920,#30921,#30922,
#30923,#30924,#30925,#30926,#30927,#30928,#30929,#30930,#30931,#30932,#30933,
#30934,#30935,#30936,#30937,#30938,#30939,#30940,#30941,#30942,#30943,#30944,
#30945,#30946,#30947,#30948,#30949,#30950,#30951,#30952,#30953,#30954,#30955,
#30956,#30957,#30958,#30959,#30960,#30961,#30962,#30963,#30964,#30965,#30966,
#30967,#30968,#30969,#30970,#30971,#30972,#30973,#30974,#30975,#30976,#30977,
#30978,#30979,#30980,#30981,#30982,#30983,#30984,#30985,#30986,#30987,#30988,
#30989,#30990,#30991,#30992,#30993,#30994,#30995,#30996,#30997),
 .UNSPECIFIED.,.F.,.F.,(4,3,3,3,3,3,3,3,3,3,3,3,3,3,3,3,3,3,3,3,3,3,3,3,
3,3,3,3,3,3,3,3,3,3,3,3,3,3,3,3,3,3,3,3,3,3,3,3,3,3,3,3,3,3,3,3,3,3,3,3,
3,3,3,4),(101.622146612713,101.743648563498,101.866952969244,101.916437754171,
102.017020179948,102.117456793143,102.217776117202,102.318031288951,102.418253657653,
102.51847453138,102.618795649309,102.719164931136,102.819717684611,102.915618516467,
103.016200936897,103.11663754474,103.216956863466,103.317212029896,103.417434393299,
103.517655261755,103.617976374493,103.718345651164,103.818898399605,103.914799278763,
104.015381704087,104.115818316789,104.216137640298,104.316392811462,104.416615179546,
104.516836052622,104.617157169854,104.717526450959,104.818079203675,104.913980041058,
105.01456247698,105.114999100375,105.215318434665,105.315573616661,105.415795995612,
105.516016879574,105.616338007647,105.716707299584,105.817260062992,105.913160803354,
106.013743197147,106.114179778353,106.214499070561,106.314754210557,106.414976547646,
106.515197389943,106.615518476947,106.715887728074,106.816440451595,106.91234156565,
107.012812979089,107.113138663605,107.213347435279,107.313492448411,107.413605205227,
107.51371716713,107.61392945356,107.714190827401,107.81463362687,107.905331919362),
 .UNSPECIFIED.);
#1218=B_SPLINE_CURVE_WITH_KNOTS('',3,(#30999,#31000,#31001,#31002,#31003,
#31004,#31005,#31006,#31007,#31008,#31009,#31010,#31011,#31012,#31013,#31014,
#31015,#31016,#31017,#31018,#31019,#31020,#31021,#31022,#31023,#31024,#31025,
#31026,#31027,#31028,#31029,#31030,#31031,#31032,#31033,#31034,#31035,#31036,
#31037,#31038,#31039,#31040,#31041,#31042,#31043,#31044,#31045,#31046,#31047,
#31048,#31049,#31050,#31051,#31052,#31053,#31054,#31055,#31056,#31057,#31058,
#31059,#31060,#31061,#31062,#31063,#31064,#31065,#31066,#31067,#31068,#31069,
#31070,#31071,#31072,#31073,#31074,#31075,#31076,#31077,#31078,#31079,#31080,
#31081,#31082,#31083,#31084,#31085,#31086,#31087,#31088,#31089,#31090,#31091,
#31092,#31093,#31094,#31095,#31096,#31097,#31098,#31099,#31100,#31101,#31102,
#31103,#31104,#31105,#31106,#31107,#31108,#31109,#31110,#31111,#31112,#31113,
#31114,#31115,#31116,#31117,#31118,#31119,#31120,#31121,#31122,#31123,#31124,
#31125,#31126,#31127,#31128,#31129,#31130,#31131,#31132,#31133,#31134,#31135,
#31136,#31137,#31138,#31139,#31140,#31141,#31142,#31143,#31144,#31145,#31146,
#31147,#31148,#31149,#31150,#31151,#31152,#31153,#31154,#31155,#31156,#31157,
#31158,#31159,#31160,#31161,#31162,#31163,#31164,#31165,#31166,#31167,#31168,
#31169,#31170,#31171,#31172,#31173,#31174,#31175,#31176,#31177,#31178,#31179,
#31180,#31181,#31182,#31183,#31184,#31185,#31186,#31187,#31188,#31189,#31190,
#31191),.UNSPECIFIED.,.F.,.F.,(4,3,3,3,3,3,3,3,3,3,3,3,3,3,3,3,3,3,3,3,
3,3,3,3,3,3,3,3,3,3,3,3,3,3,3,3,3,3,3,3,3,3,3,3,3,3,3,3,3,3,3,3,3,3,3,3,
3,3,3,3,3,3,3,3,4),(107.905331919576,107.911522327946,108.012104832105,
108.11254152419,108.212860927529,108.313116178762,108.413338627042,108.51355958033,
108.613880777234,108.714250137846,108.814802968842,108.910703090242,109.011285269332,
109.111721635678,109.212040713789,109.312295640242,109.412517764625,109.51273839534,
109.613059274002,109.713428318213,109.813980839695,109.909883852537,110.010466487225,
110.110903307623,110.211222835385,110.311478208629,110.411700776365,110.511921846407,
110.612243155036,110.712612624817,110.813165559368,110.909064614833,111.009647553955,
111.110084684757,111.210404530373,111.310660225851,111.410883119722,111.51110451933,
111.61142616054,111.711795965091,111.812349234085,111.908245377129,112.008825861756,
112.109260531332,112.209577917086,112.309831154579,112.410051595662,112.510270551,
112.610589778432,112.710957181861,112.811508099817,112.907426139425,113.008010700115,
113.10844943665,113.20877085699,113.309028107726,113.409252535454,113.509475445561,
113.609798550258,113.71016979507,113.810724447976,113.906606901721,114.032061637831,
114.155474775546,114.188517226495),.UNSPECIFIED.);
#1219=B_SPLINE_CURVE_WITH_KNOTS('',3,(#31193,#31194,#31195,#31196,#31197,
#31198,#31199,#31200,#31201,#31202,#31203,#31204,#31205,#31206,#31207,#31208,
#31209,#31210,#31211,#31212,#31213,#31214,#31215,#31216,#31217,#31218,#31219,
#31220,#31221,#31222,#31223,#31224,#31225,#31226,#31227,#31228,#31229,#31230,
#31231,#31232,#31233,#31234,#31235,#31236,#31237,#31238,#31239,#31240,#31241,
#31242,#31243,#31244,#31245,#31246,#31247,#31248,#31249,#31250,#31251,#31252,
#31253,#31254,#31255,#31256,#31257,#31258,#31259,#31260,#31261,#31262,#31263,
#31264,#31265,#31266,#31267,#31268,#31269,#31270,#31271,#31272,#31273,#31274,
#31275,#31276,#31277,#31278,#31279,#31280,#31281,#31282,#31283,#31284,#31285,
#31286,#31287,#31288,#31289,#31290,#31291,#31292,#31293,#31294,#31295,#31296,
#31297,#31298,#31299,#31300,#31301,#31302,#31303,#31304,#31305,#31306,#31307,
#31308,#31309,#31310,#31311,#31312,#31313,#31314,#31315,#31316,#31317,#31318,
#31319,#31320,#31321,#31322,#31323,#31324,#31325,#31326,#31327,#31328,#31329,
#31330,#31331,#31332,#31333,#31334,#31335,#31336,#31337,#31338,#31339,#31340,
#31341,#31342,#31343,#31344,#31345,#31346,#31347,#31348,#31349,#31350,#31351,
#31352,#31353,#31354,#31355,#31356,#31357,#31358,#31359,#31360,#31361,#31362,
#31363,#31364,#31365,#31366,#31367,#31368,#31369,#31370,#31371,#31372,#31373,
#31374,#31375,#31376,#31377,#31378,#31379,#31380,#31381,#31382,#31383,#31384,
#31385),.UNSPECIFIED.,.F.,.F.,(4,3,3,3,3,3,3,3,3,3,3,3,3,3,3,3,3,3,3,3,
3,3,3,3,3,3,3,3,3,3,3,3,3,3,3,3,3,3,3,3,3,3,3,3,3,3,3,3,3,3,3,3,3,3,3,3,
3,3,3,3,3,3,3,3,4),(114.188517226756,114.287978532167,114.387393774356,
114.486795269358,114.586215309855,114.685747211439,114.785347086434,114.885107888347,
114.905787664016,115.006355055542,115.106776605851,115.207080893984,115.307321052522,
115.407528450849,115.507734417188,115.60804083083,115.708395494866,115.808933951395,
115.904968426312,116.005571080338,116.10602784679,116.20636711905,116.306642106101,
116.406884131427,116.507124477183,116.607464642396,116.707852771135,116.80842380852,
116.904149188608,117.004747547077,117.105200368142,117.205536234604,117.305808144354,
117.406047422113,117.506285351591,117.606623633199,117.70701016571,117.807580109372,
117.903329950904,118.003798493702,118.104120937105,118.204326186812,118.30446738779,
118.404576040251,118.504683603356,118.604892837216,118.705150825343,118.805594615079,
118.902510713199,119.003276219575,119.103895455646,119.204395862128,119.304831096984,
119.405232267188,119.505630437432,119.606125250882,119.706666540895,119.807386410131,
119.901691475495,120.004328434329,120.106799487655,120.209100979967,120.311302855602,
120.413424519418,120.471702533936),.UNSPECIFIED.);
#1220=B_SPLINE_CURVE_WITH_KNOTS('',3,(#31387,#31388,#31389,#31390,#31391,
#31392,#31393,#31394,#31395,#31396,#31397,#31398,#31399,#31400,#31401,#31402),
 .UNSPECIFIED.,.F.,.F.,(4,3,3,3,3,4),(120.471702534265,120.581378567869,
120.691378633643,120.801880018795,120.900872237791,120.914211738165),
 .UNSPECIFIED.);
#1221=B_SPLINE_CURVE_WITH_KNOTS('',3,(#31408,#31409,#31410,#31411,#31412,
#31413,#31414,#31415,#31416),.UNSPECIFIED.,.F.,.F.,(4,1,1,1,1,1,4),(-122.899233762383,
-121.900053000087,-120.900872237791,-119.901691475495,-118.9025107132,-117.903329950904,
-117.132769022939),.UNSPECIFIED.);
#1222=B_SPLINE_CURVE_WITH_KNOTS('',3,(#31418,#31419,#31420,#31421,#31422,
#31423,#31424,#31425,#31426,#31427,#31428,#31429,#31430,#31431,#31432,#31433,
#31434,#31435,#31436,#31437,#31438,#31439,#31440,#31441,#31442,#31443,#31444,
#31445,#31446,#31447,#31448,#31449,#31450,#31451,#31452,#31453,#31454,#31455,
#31456,#31457,#31458,#31459,#31460,#31461,#31462,#31463,#31464,#31465,#31466,
#31467,#31468,#31469,#31470,#31471,#31472,#31473,#31474,#31475,#31476,#31477,
#31478,#31479,#31480,#31481,#31482,#31483,#31484,#31485,#31486,#31487,#31488,
#31489,#31490,#31491,#31492,#31493,#31494,#31495,#31496,#31497,#31498,#31499,
#31500,#31501,#31502,#31503,#31504,#31505,#31506,#31507,#31508,#31509,#31510,
#31511,#31512,#31513,#31514,#31515,#31516,#31517,#31518,#31519,#31520,#31521,
#31522,#31523,#31524,#31525,#31526,#31527,#31528,#31529,#31530,#31531,#31532,
#31533,#31534,#31535,#31536,#31537,#31538,#31539,#31540,#31541,#31542,#31543,
#31544,#31545,#31546,#31547,#31548,#31549,#31550,#31551,#31552,#31553,#31554,
#31555,#31556,#31557,#31558,#31559,#31560,#31561,#31562,#31563,#31564,#31565,
#31566,#31567,#31568,#31569,#31570,#31571,#31572,#31573,#31574,#31575,#31576,
#31577,#31578,#31579,#31580,#31581,#31582,#31583,#31584,#31585,#31586,#31587,
#31588,#31589,#31590,#31591,#31592,#31593,#31594,#31595,#31596,#31597,#31598,
#31599,#31600,#31601,#31602,#31603,#31604,#31605,#31606,#31607),
 .UNSPECIFIED.,.F.,.F.,(4,3,3,3,3,3,3,3,3,3,3,3,3,3,3,3,3,3,3,3,3,3,3,3,
3,3,3,3,3,3,3,3,3,3,3,3,3,3,3,3,3,3,3,3,3,3,3,3,3,3,3,3,3,3,3,3,3,3,3,3,
3,3,3,4),(-117.132768509517,-116.99762221968,-116.904149188608,-116.803548664545,
-116.70309356908,-116.602755269422,-116.502480830314,-116.402238928977,
-116.30199828355,-116.20165715403,-116.101267696988,-116.000694727717,-115.904968426312,
-115.804400176277,-115.703977948936,-115.603673260019,-115.50343286865,
-115.403225405187,-115.303019541313,-115.20271349326,-115.102359338845,
-115.001821631126,-114.905787664016,-114.805202101569,-114.704762334078,
-114.604439844353,-114.504181501441,-114.40395596052,-114.303731917959,
-114.203407659086,-114.103035246359,-114.002479416692,-113.906606901721,
-113.806022597919,-113.705584063024,-113.605262760248,-113.505005575957,
-113.404781163642,-113.304558217948,-113.204234997641,-113.103863593401,
-113.003308708377,-112.907426139425,-112.806845532387,-112.70641076616,
-112.606093322967,-112.505840051877,-112.405619601004,-112.305400659671,
-112.205081483597,-112.104714151975,-112.004163339784,-111.908245377129,
-111.807662439649,-111.707225310445,-111.606905466351,-111.50664977235,
-111.406426879908,-111.306205481679,-111.20588384176,-111.105514038454,
-111.004960770612,-110.909064614833,-110.849583202338),.UNSPECIFIED.);
#1223=B_SPLINE_CURVE_WITH_KNOTS('',3,(#31609,#31610,#31611,#31612,#31613,
#31614,#31615,#31616,#31617,#31618,#31619,#31620,#31621,#31622,#31623,#31624,
#31625,#31626,#31627,#31628,#31629,#31630,#31631,#31632,#31633,#31634,#31635,
#31636,#31637,#31638,#31639,#31640,#31641,#31642,#31643,#31644,#31645,#31646,
#31647,#31648,#31649,#31650,#31651,#31652,#31653,#31654,#31655,#31656,#31657,
#31658,#31659,#31660,#31661,#31662,#31663,#31664,#31665,#31666,#31667,#31668,
#31669,#31670,#31671,#31672,#31673,#31674,#31675,#31676,#31677,#31678,#31679,
#31680,#31681,#31682,#31683,#31684,#31685,#31686,#31687,#31688,#31689,#31690,
#31691,#31692,#31693,#31694,#31695,#31696,#31697,#31698,#31699,#31700,#31701,
#31702,#31703,#31704,#31705,#31706,#31707,#31708,#31709,#31710,#31711,#31712,
#31713,#31714,#31715,#31716,#31717,#31718,#31719,#31720,#31721,#31722,#31723,
#31724,#31725,#31726,#31727,#31728,#31729,#31730,#31731,#31732,#31733,#31734,
#31735,#31736,#31737,#31738,#31739,#31740,#31741,#31742,#31743,#31744,#31745,
#31746,#31747,#31748,#31749,#31750,#31751,#31752,#31753,#31754,#31755,#31756,
#31757,#31758,#31759,#31760,#31761,#31762,#31763,#31764,#31765,#31766,#31767,
#31768,#31769,#31770,#31771,#31772,#31773,#31774,#31775,#31776,#31777,#31778,
#31779,#31780,#31781,#31782,#31783,#31784,#31785,#31786,#31787,#31788,#31789,
#31790,#31791,#31792,#31793,#31794,#31795,#31796,#31797,#31798),
 .UNSPECIFIED.,.F.,.F.,(4,3,3,3,3,3,3,3,3,3,3,3,3,3,3,3,3,3,3,3,3,3,3,3,
3,3,3,3,3,3,3,3,3,3,3,3,3,3,3,3,3,3,3,3,3,3,3,3,3,3,3,3,3,3,3,3,3,3,3,3,
3,3,3,4),(-110.849583201969,-110.749906777761,-110.65036988621,-110.550939824221,
-110.451566049954,-110.352216145972,-110.252857728841,-110.153395285142,
-110.053873649823,-109.954186934386,-109.909883852537,-109.80930165653,
-109.708865276814,-109.608546190731,-109.50829125959,-109.408069133795,
-109.307848504946,-109.207527633292,-109.107158598905,-109.006606091923,
-108.910703090242,-108.810120587652,-108.709683896851,-108.609364494357,
-108.509109243704,-108.408886795739,-108.308665842499,-108.208344645225,
-108.107975284014,-108.007422452036,-107.911522327946,-107.81093988886,
-107.710503261861,-107.610183923317,-107.509928736672,-107.409706352685,
-107.309485463304,-107.209164329244,-107.108795031,-107.008242260811,-106.91234156565,
-106.811759169579,-106.711322586572,-106.611003293288,-106.510748152655,
-106.41052581537,-106.310304973317,-106.209983887248,-106.109614637433,
-106.009061915852,-105.913160803354,-105.812578367802,-105.712141744707,
-105.611822410606,-105.511567228734,-105.411344849841,-105.31112396587,
-105.210802837685,-105.110433545577,-105.009880781905,-104.913980041058,
-104.797419643664,-104.681890702285,-104.566397895385),.UNSPECIFIED.);
#1224=B_SPLINE_CURVE_WITH_KNOTS('',3,(#31800,#31801,#31802,#31803,#31804,
#31805,#31806,#31807,#31808,#31809,#31810,#31811,#31812,#31813,#31814,#31815,
#31816,#31817,#31818,#31819,#31820,#31821,#31822,#31823,#31824,#31825,#31826,
#31827,#31828,#31829,#31830,#31831,#31832,#31833,#31834,#31835,#31836,#31837,
#31838,#31839,#31840,#31841,#31842,#31843,#31844,#31845,#31846,#31847,#31848,
#31849,#31850,#31851,#31852,#31853,#31854,#31855,#31856,#31857,#31858,#31859,
#31860,#31861,#31862,#31863,#31864,#31865,#31866,#31867,#31868,#31869,#31870,
#31871,#31872,#31873,#31874,#31875,#31876,#31877,#31878,#31879,#31880,#31881,
#31882,#31883,#31884,#31885,#31886,#31887,#31888,#31889,#31890,#31891,#31892,
#31893,#31894,#31895,#31896,#31897,#31898,#31899,#31900,#31901,#31902,#31903,
#31904,#31905,#31906,#31907,#31908,#31909,#31910,#31911,#31912,#31913,#31914,
#31915,#31916,#31917,#31918,#31919,#31920,#31921,#31922,#31923,#31924,#31925,
#31926,#31927,#31928,#31929,#31930,#31931,#31932,#31933,#31934,#31935,#31936,
#31937,#31938,#31939,#31940,#31941,#31942,#31943,#31944,#31945,#31946,#31947,
#31948,#31949,#31950,#31951,#31952,#31953,#31954,#31955,#31956,#31957,#31958,
#31959,#31960,#31961,#31962,#31963,#31964,#31965,#31966,#31967,#31968,#31969,
#31970,#31971,#31972,#31973,#31974,#31975,#31976,#31977,#31978,#31979,#31980,
#31981,#31982,#31983,#31984,#31985,#31986,#31987,#31988,#31989,#31990,#31991,
#31992),.UNSPECIFIED.,.F.,.F.,(4,3,3,3,3,3,3,3,3,3,3,3,3,3,3,3,3,3,3,3,
3,3,3,3,3,3,3,3,3,3,3,3,3,3,3,3,3,3,3,3,3,3,3,3,3,3,3,3,3,3,3,3,3,3,3,3,
3,3,3,3,3,3,3,3,4),(-104.566397895158,-104.465980669188,-104.365570501461,
-104.265136550864,-104.164578820184,-104.063951390142,-103.9631441112,-103.914799278763,
-103.814216858034,-103.713780249953,-103.613460931085,-103.513205764572,
-103.412983401142,-103.312762532717,-103.212441420101,-103.112072143601,
-103.011519395415,-102.915618516467,-102.815036090758,-102.714599477618,
-102.614280153594,-102.514024981867,-102.413802613174,-102.313581739445,
-102.213260621494,-102.112891339635,-102.01233858611,-101.916437754171,
-101.815855330105,-101.715418718623,-101.615099396275,-101.514844226233,
-101.414621859232,-101.314400987198,-101.214079870939,-101.113710590771,
-101.013157838918,-100.917256991875,-100.816674568175,-100.716237957071,
-100.615918635115,-100.515663465475,-100.415441098886,-100.315220227272,
-100.214899111442,-100.114529831709,-100.013977080297,-99.9180762295794,
-99.8174938052647,-99.7170571935358,-99.6167378709423,-99.5164827006572,
-99.4162603334156,-99.316039461144,-99.2157183446526,-99.1153490642547,
-99.0147963121794,-98.9188954672836,-98.8177509139559,-98.7167554082157,
-98.6158783757221,-98.5150934552823,-98.414361403763,-98.3136395349575,
-98.2832125879784),.UNSPECIFIED.);
#1225=B_SPLINE_CURVE_WITH_KNOTS('',3,(#31994,#31995,#31996,#31997,#31998,
#31999,#32000,#32001,#32002,#32003,#32004,#32005,#32006,#32007,#32008,#32009,
#32010,#32011,#32012,#32013,#32014,#32015,#32016,#32017,#32018,#32019,#32020,
#32021,#32022,#32023,#32024,#32025,#32026,#32027,#32028,#32029,#32030,#32031,
#32032,#32033,#32034,#32035,#32036,#32037,#32038,#32039,#32040,#32041,#32042,
#32043,#32044,#32045,#32046,#32047,#32048,#32049,#32050,#32051,#32052,#32053,
#32054,#32055,#32056,#32057,#32058,#32059,#32060,#32061,#32062,#32063,#32064,
#32065,#32066,#32067,#32068,#32069,#32070,#32071,#32072,#32073,#32074,#32075,
#32076,#32077,#32078,#32079,#32080,#32081,#32082,#32083,#32084,#32085,#32086,
#32087,#32088,#32089,#32090,#32091,#32092,#32093,#32094,#32095,#32096,#32097,
#32098,#32099,#32100,#32101,#32102,#32103,#32104,#32105,#32106,#32107,#32108,
#32109,#32110,#32111,#32112,#32113,#32114,#32115,#32116,#32117,#32118,#32119,
#32120,#32121,#32122,#32123,#32124,#32125,#32126,#32127,#32128,#32129,#32130,
#32131,#32132,#32133,#32134,#32135,#32136,#32137,#32138,#32139,#32140,#32141,
#32142,#32143,#32144,#32145,#32146,#32147,#32148,#32149,#32150,#32151,#32152,
#32153,#32154,#32155,#32156,#32157,#32158,#32159,#32160,#32161,#32162,#32163,
#32164,#32165,#32166,#32167,#32168,#32169,#32170,#32171,#32172,#32173,#32174,
#32175,#32176,#32177,#32178,#32179,#32180,#32181,#32182,#32183,#32184,#32185,
#32186),.UNSPECIFIED.,.F.,.F.,(4,3,3,3,3,3,3,3,3,3,3,3,3,3,3,3,3,3,3,3,
3,3,3,3,3,3,3,3,3,3,3,3,3,3,3,3,3,3,3,3,3,3,3,3,3,3,3,3,3,3,3,3,3,3,3,3,
3,3,3,3,3,3,3,3,4),(-98.2832125877455,-98.1694097971249,-98.0550264144753,
-97.9399742888503,-97.9197147049878,-97.8191322809388,-97.7186956694796,
-97.6183763471603,-97.5181211771522,-97.4178988101899,-97.3176779381995,
-97.2173568219901,-97.1169875418754,-97.0164347900815,-96.920533942692,
-96.8199515185687,-96.719514907034,-96.6191955846376,-96.5189404145513,
-96.4187180475099,-96.3184971754399,-96.2181760591502,-96.1178067789548,
-96.0172540270803,-95.9213531803962,-95.8207707563073,-95.7203341448072,
-95.620014822446,-95.5197596523953,-95.4195372853897,-95.3193164133555,
-95.2189952971017,-95.1186260169423,-95.0180732651035,-94.9221724181004,
-94.8215899940116,-94.7211533825118,-94.620834060151,-94.5205788901007,
-94.4203565230957,-94.3201356510622,-94.2198145348092,-94.1194452546507,
-94.0188925028129,-93.9229916558047,-93.8224092317071,-93.7219726201984,
-93.6216532978285,-93.5213981277689,-93.4211757607546,-93.3209548887116,
-93.2206337724491,-93.1202644922809,-93.0197117404336,-92.9238108935089,
-92.8242800268147,-92.7212484335895,-92.6219796999193,-92.5227705795473,
-92.4235884764662,-92.3244008328193,-92.2251181263679,-92.1257782787119,
-92.0262884834329,-92.0000272810126),.UNSPECIFIED.);
#1226=B_SPLINE_CURVE_WITH_KNOTS('',3,(#32188,#32189,#32190,#32191,#32192,
#32193,#32194,#32195,#32196,#32197,#32198,#32199,#32200,#32201,#32202,#32203,
#32204,#32205,#32206,#32207,#32208,#32209,#32210,#32211,#32212,#32213,#32214,
#32215,#32216,#32217,#32218,#32219,#32220,#32221,#32222,#32223,#32224,#32225,
#32226,#32227,#32228,#32229,#32230,#32231,#32232,#32233,#32234,#32235,#32236,
#32237,#32238,#32239,#32240,#32241,#32242,#32243,#32244,#32245,#32246,#32247,
#32248,#32249,#32250,#32251,#32252,#32253,#32254,#32255,#32256,#32257,#32258,
#32259,#32260,#32261,#32262,#32263,#32264,#32265,#32266,#32267,#32268,#32269,
#32270,#32271,#32272,#32273,#32274,#32275,#32276,#32277,#32278,#32279,#32280,
#32281,#32282,#32283,#32284,#32285,#32286,#32287,#32288,#32289,#32290,#32291,
#32292,#32293,#32294,#32295,#32296,#32297,#32298,#32299,#32300,#32301,#32302,
#32303,#32304,#32305,#32306,#32307,#32308,#32309,#32310,#32311,#32312,#32313,
#32314,#32315,#32316,#32317,#32318,#32319,#32320,#32321,#32322,#32323,#32324,
#32325,#32326,#32327,#32328,#32329,#32330,#32331,#32332,#32333,#32334,#32335,
#32336,#32337,#32338,#32339,#32340,#32341,#32342,#32343,#32344,#32345,#32346,
#32347,#32348,#32349,#32350,#32351,#32352,#32353,#32354,#32355,#32356,#32357,
#32358,#32359,#32360,#32361,#32362,#32363,#32364,#32365,#32366,#32367,#32368,
#32369,#32370,#32371,#32372,#32373,#32374,#32375,#32376,#32377),
 .UNSPECIFIED.,.F.,.F.,(4,3,3,3,3,3,3,3,3,3,3,3,3,3,3,3,3,3,3,3,3,3,3,3,
3,3,3,3,3,3,3,3,3,3,3,3,3,3,3,3,3,3,3,3,3,3,3,3,3,3,3,3,3,3,3,3,3,3,3,3,
3,3,3,4),(-92.0000272807988,-91.9246301312131,-91.82404770712,-91.7236110956159,
-91.6232917732506,-91.5230366031958,-91.4228142361862,-91.3225933641481,
-91.2222722478904,-91.1219029677271,-91.0213502158846,-90.9254493689173,
-90.824866944823,-90.7244303333177,-90.6241110109511,-90.523855840895,-90.4236334738841,
-90.3234126018446,-90.2230914855856,-90.122722205421,-90.0221694535771,
-89.9262686066215,-89.825686182528,-89.7252495710234,-89.6249302486576,
-89.5246750786023,-89.4244527115922,-89.3242318395535,-89.2239107232953,
-89.1235414431315,-89.0229886912884,-88.9270878443257,-88.826505420232,
-88.7260688087273,-88.6257494863614,-88.5254943163059,-88.4252719492956,
-88.3250510772568,-88.2247299609984,-88.1243606808344,-88.0238079289912,
-87.9279070820299,-87.8273246579361,-87.7268880464313,-87.6265687240653,
-87.5263135540097,-87.4260911869993,-87.3258703149604,-87.2255491987019,
-87.1251799185378,-87.0246271666945,-86.9287263197341,-86.8281438956404,
-86.7277072841356,-86.6273879617697,-86.5271327917142,-86.426910424704,
-86.3266895526652,-86.2263684364068,-86.1259991562429,-86.0254464043996,
-85.9295455574383,-85.7895984276924,-85.7168419736192),.UNSPECIFIED.);
#1227=B_SPLINE_CURVE_WITH_KNOTS('',3,(#32379,#32380,#32381,#32382,#32383,
#32384,#32385,#32386,#32387,#32388,#32389,#32390,#32391,#32392,#32393,#32394,
#32395,#32396,#32397,#32398,#32399,#32400,#32401,#32402,#32403,#32404,#32405,
#32406,#32407,#32408,#32409,#32410,#32411,#32412,#32413,#32414,#32415,#32416,
#32417,#32418,#32419,#32420,#32421,#32422,#32423,#32424,#32425,#32426,#32427,
#32428,#32429,#32430,#32431,#32432,#32433,#32434,#32435,#32436,#32437,#32438,
#32439,#32440,#32441,#32442,#32443,#32444,#32445,#32446,#32447,#32448,#32449,
#32450,#32451,#32452,#32453,#32454,#32455,#32456,#32457,#32458,#32459,#32460,
#32461,#32462,#32463,#32464,#32465,#32466,#32467,#32468,#32469,#32470,#32471,
#32472,#32473,#32474,#32475,#32476,#32477,#32478,#32479,#32480,#32481,#32482,
#32483,#32484,#32485,#32486,#32487,#32488,#32489,#32490,#32491,#32492,#32493,
#32494,#32495,#32496,#32497,#32498,#32499,#32500,#32501,#32502,#32503,#32504,
#32505,#32506,#32507,#32508,#32509,#32510,#32511,#32512,#32513,#32514,#32515,
#32516,#32517,#32518,#32519,#32520,#32521,#32522,#32523,#32524,#32525,#32526,
#32527,#32528,#32529,#32530,#32531,#32532,#32533,#32534,#32535,#32536,#32537,
#32538,#32539,#32540,#32541,#32542,#32543,#32544,#32545,#32546,#32547,#32548,
#32549,#32550,#32551,#32552,#32553,#32554,#32555,#32556,#32557,#32558,#32559,
#32560,#32561,#32562,#32563,#32564,#32565,#32566,#32567,#32568),
 .UNSPECIFIED.,.F.,.F.,(4,3,3,3,3,3,3,3,3,3,3,3,3,3,3,3,3,3,3,3,3,3,3,3,
3,3,3,3,3,3,3,3,3,3,3,3,3,3,3,3,3,3,3,3,3,3,3,3,3,3,3,3,3,3,3,3,3,3,3,3,
3,3,3,4),(-85.7168419733983,-85.6178735192426,-85.5189824534746,-85.4201358121954,
-85.3213006913025,-85.2223761543513,-85.1234094807557,-85.0242647323262,
-84.9303647951425,-84.8297823710488,-84.7293457595441,-84.6290264371782,
-84.5287712671227,-84.4285489001124,-84.3283280280738,-84.2280069118154,
-84.1276376316514,-84.0270848798082,-83.9311840328467,-83.8306016087529,
-83.7301649972482,-83.6298456748821,-83.5295905048266,-83.4293681378162,
-83.3291472657775,-83.228826149519,-83.1284568693549,-83.0279041175116,
-82.9320032705509,-82.8314208464572,-82.7309842349524,-82.6306649125865,
-82.5304097425309,-82.4301873755207,-82.3299665034819,-82.2296453872236,
-82.1292761070595,-82.0287233552163,-81.9328225082551,-81.8322400841614,
-81.7318034726565,-81.6314841502906,-81.5312289802351,-81.4310066132246,
-81.3307857411861,-81.2304646249277,-81.1300953447638,-81.0295425929205,
-80.9336417459593,-80.8330593218657,-80.7326227103606,-80.6323033879947,
-80.5320482179393,-80.4318258509289,-80.3316049788899,-80.2312838626314,
-80.1309145824676,-80.0303618306243,-79.9344609836635,-79.8287563918983,
-79.7233516333537,-79.6181260623224,-79.5131294138356,-79.4336566664396),
 .UNSPECIFIED.);
#1228=B_SPLINE_CURVE_WITH_KNOTS('',3,(#32570,#32571,#32572,#32573,#32574,
#32575,#32576,#32577,#32578,#32579,#32580,#32581,#32582,#32583,#32584,#32585,
#32586,#32587,#32588,#32589,#32590,#32591,#32592,#32593,#32594,#32595,#32596,
#32597,#32598,#32599,#32600,#32601,#32602,#32603,#32604,#32605,#32606,#32607,
#32608,#32609,#32610,#32611,#32612,#32613,#32614,#32615,#32616,#32617,#32618,
#32619,#32620,#32621,#32622,#32623,#32624,#32625,#32626,#32627,#32628,#32629,
#32630,#32631,#32632,#32633,#32634,#32635,#32636,#32637,#32638,#32639,#32640,
#32641,#32642,#32643,#32644,#32645,#32646,#32647,#32648,#32649,#32650,#32651,
#32652,#32653,#32654,#32655,#32656,#32657,#32658,#32659,#32660,#32661,#32662,
#32663,#32664,#32665,#32666,#32667,#32668,#32669,#32670,#32671,#32672,#32673,
#32674,#32675,#32676,#32677,#32678,#32679,#32680,#32681,#32682,#32683,#32684,
#32685,#32686,#32687,#32688,#32689,#32690,#32691,#32692,#32693,#32694,#32695,
#32696,#32697,#32698,#32699,#32700,#32701,#32702,#32703,#32704,#32705,#32706,
#32707,#32708,#32709,#32710,#32711,#32712,#32713,#32714,#32715,#32716,#32717,
#32718,#32719,#32720,#32721,#32722,#32723,#32724,#32725,#32726,#32727,#32728,
#32729,#32730,#32731,#32732,#32733,#32734,#32735,#32736,#32737,#32738,#32739,
#32740,#32741,#32742,#32743,#32744,#32745,#32746,#32747,#32748,#32749,#32750,
#32751,#32752,#32753,#32754,#32755,#32756,#32757,#32758,#32759),
 .UNSPECIFIED.,.F.,.F.,(4,3,3,3,3,3,3,3,3,3,3,3,3,3,3,3,3,3,3,3,3,3,3,3,
3,3,3,3,3,3,3,3,3,3,3,3,3,3,3,3,3,3,3,3,3,3,3,3,3,3,3,3,3,3,3,3,3,3,3,3,
3,3,3,4),(-79.4336566660391,-79.32862297329,-79.223297972688,-79.1178224512306,
-79.0120566743491,-78.9352802213677,-78.834697797274,-78.7342611857693,
-78.6339418634034,-78.5336866933479,-78.4334643263377,-78.3332434542988,
-78.2329223380405,-78.1325530578765,-78.0320003060333,-77.936099459072,
-77.8355170349783,-77.7350804234736,-77.6347611011076,-77.5345059310521,
-77.4342835640418,-77.334062692003,-77.2337415757446,-77.1333722955806,
-77.0328195437373,-76.9369186967762,-76.8363362726825,-76.7358996611777,
-76.6355803388117,-76.5353251687562,-76.4351028017458,-76.334881929707,
-76.2345608134485,-76.1341915332845,-76.0336387814412,-75.9377379344804,
-75.8371555103867,-75.7367188988819,-75.636399576516,-75.5361444064605,
-75.4359220394502,-75.3357011674114,-75.235380051153,-75.1350107709891,
-75.0344580191458,-74.9385571721846,-74.8379747480909,-74.737538136586,
-74.6372188142201,-74.5369636441646,-74.4367412771542,-74.3365204051153,
-74.2361992888569,-74.1358300086929,-74.0352772568497,-73.9393764098888,
-73.8402435573838,-73.7412396430733,-73.6423315119675,-73.5434861373362,
-73.4446309224566,-73.3457775064429,-73.246816995228,-73.1504713595064),
 .UNSPECIFIED.);
#1229=B_SPLINE_CURVE_WITH_KNOTS('',3,(#32761,#32762,#32763,#32764,#32765,
#32766,#32767,#32768,#32769,#32770,#32771,#32772,#32773,#32774,#32775,#32776,
#32777,#32778,#32779,#32780,#32781,#32782,#32783,#32784,#32785,#32786,#32787,
#32788,#32789,#32790,#32791,#32792,#32793,#32794,#32795,#32796,#32797,#32798,
#32799,#32800,#32801,#32802,#32803,#32804,#32805,#32806,#32807,#32808,#32809,
#32810,#32811,#32812,#32813,#32814,#32815,#32816,#32817,#32818,#32819,#32820,
#32821,#32822,#32823,#32824,#32825,#32826,#32827,#32828,#32829,#32830,#32831,
#32832,#32833,#32834,#32835,#32836,#32837,#32838,#32839,#32840,#32841,#32842,
#32843,#32844,#32845,#32846,#32847,#32848,#32849,#32850,#32851,#32852,#32853,
#32854,#32855,#32856,#32857,#32858,#32859,#32860,#32861,#32862,#32863,#32864,
#32865,#32866,#32867,#32868,#32869,#32870,#32871,#32872,#32873,#32874,#32875,
#32876,#32877,#32878,#32879,#32880,#32881,#32882,#32883,#32884,#32885,#32886,
#32887,#32888,#32889,#32890,#32891,#32892,#32893,#32894,#32895,#32896,#32897,
#32898,#32899,#32900,#32901,#32902,#32903,#32904,#32905,#32906,#32907,#32908,
#32909,#32910,#32911,#32912,#32913,#32914,#32915,#32916,#32917,#32918,#32919,
#32920,#32921,#32922,#32923,#32924,#32925,#32926,#32927,#32928,#32929,#32930,
#32931,#32932,#32933,#32934,#32935,#32936,#32937,#32938,#32939,#32940,#32941,
#32942,#32943,#32944,#32945,#32946,#32947,#32948,#32949,#32950),
 .UNSPECIFIED.,.F.,.F.,(4,3,3,3,3,3,3,3,3,3,3,3,3,3,3,3,3,3,3,3,3,3,3,3,
3,3,3,3,3,3,3,3,3,3,3,3,3,3,3,3,3,3,3,3,3,3,3,3,3,3,3,3,3,3,3,3,3,3,3,3,
3,3,3,4),(-73.15047135926,-73.0097533718863,-72.940195647593,-72.8396132234992,
-72.7391766119943,-72.6388572896282,-72.5386021195726,-72.4383797525622,
-72.3381588805232,-72.2378377642647,-72.1374684841005,-72.0369157322571,
-71.9410148852972,-71.8404324612035,-71.7399958496988,-71.6396765273329,
-71.5394213572774,-71.4391989902671,-71.3389781182283,-71.2386570019699,
-71.138287721806,-71.0377349699627,-70.9418341230014,-70.8412516989077,
-70.7408150874029,-70.6404957650369,-70.5402405949815,-70.4400182279711,
-70.3397973559323,-70.2394762396739,-70.1391069595099,-70.0385542076666,
-69.9426533607056,-69.8420709366119,-69.7416343251071,-69.6413150027412,
-69.5410598326856,-69.4408374656753,-69.3406165936365,-69.2402954773781,
-69.1399261972141,-69.0393734453708,-68.9434725984098,-68.8428901743161,
-68.7424535628113,-68.6421342404454,-68.5418790703899,-68.4416567033796,
-68.3414358313408,-68.2411147150824,-68.1407454349183,-68.0401926830751,
-67.944291836114,-67.8437094120203,-67.7432728005156,-67.6429534781497,
-67.5426983080942,-67.4424759410838,-67.3422550690451,-67.2419339527867,
-67.1415646726227,-67.0410119207795,-66.9451110738182,-66.8672860520804),
 .UNSPECIFIED.);
#1230=B_SPLINE_CURVE_WITH_KNOTS('',3,(#32952,#32953,#32954,#32955,#32956,
#32957,#32958,#32959,#32960,#32961,#32962,#32963,#32964,#32965,#32966,#32967,
#32968,#32969,#32970,#32971,#32972,#32973,#32974,#32975,#32976,#32977,#32978,
#32979,#32980,#32981,#32982,#32983,#32984,#32985,#32986,#32987,#32988,#32989,
#32990,#32991,#32992,#32993,#32994,#32995,#32996,#32997,#32998,#32999,#33000,
#33001,#33002,#33003,#33004,#33005,#33006,#33007,#33008,#33009,#33010,#33011,
#33012,#33013,#33014,#33015,#33016,#33017,#33018,#33019,#33020,#33021,#33022,
#33023,#33024,#33025,#33026,#33027,#33028,#33029,#33030,#33031,#33032,#33033,
#33034,#33035,#33036,#33037,#33038,#33039,#33040,#33041,#33042,#33043,#33044,
#33045,#33046,#33047,#33048,#33049,#33050,#33051,#33052,#33053,#33054,#33055,
#33056,#33057,#33058,#33059,#33060,#33061,#33062,#33063,#33064,#33065,#33066,
#33067,#33068,#33069,#33070,#33071,#33072,#33073,#33074,#33075,#33076,#33077,
#33078,#33079,#33080,#33081,#33082,#33083,#33084,#33085,#33086,#33087,#33088,
#33089,#33090,#33091,#33092,#33093,#33094,#33095,#33096,#33097,#33098,#33099,
#33100,#33101,#33102,#33103,#33104,#33105,#33106,#33107,#33108,#33109,#33110,
#33111,#33112,#33113,#33114,#33115,#33116,#33117,#33118,#33119,#33120,#33121,
#33122,#33123,#33124,#33125,#33126,#33127,#33128,#33129,#33130,#33131,#33132,
#33133,#33134,#33135,#33136,#33137,#33138,#33139,#33140,#33141,#33142,#33143,
#33144),.UNSPECIFIED.,.F.,.F.,(4,3,3,3,3,3,3,3,3,3,3,3,3,3,3,3,3,3,3,3,
3,3,3,3,3,3,3,3,3,3,3,3,3,3,3,3,3,3,3,3,3,3,3,3,3,3,3,3,3,3,3,3,3,3,3,3,
3,3,3,3,3,3,3,3,4),(-66.8672860518669,-66.7678166672169,-66.6650808727551,
-66.5658511493962,-66.4666728636925,-66.3675134088591,-66.2683402071068,
-66.1690603763527,-66.0697162817546,-65.9702133876511,-65.9459303115224,
-65.8453478874287,-65.7449112759237,-65.6445919535578,-65.5443367835023,
-65.4441144164919,-65.3438935444529,-65.2435724281946,-65.1432031480306,
-65.0426503961873,-64.9467495492266,-64.8461671251329,-64.7457305136282,
-64.6454111912623,-64.5451560212068,-64.4449336541966,-64.3447127821579,
-64.2443916658995,-64.1440223857354,-64.0434696338922,-63.9475687869308,
-63.8469863628371,-63.7465497513326,-63.6462304289666,-63.5459752589111,
-63.4457528919008,-63.3455320198621,-63.2452109036037,-63.1448416234397,
-63.0442888715964,-62.948388024635,-62.8478056005413,-62.7473689890367,
-62.6470496666707,-62.5467944966153,-62.4465721296051,-62.3463512575662,
-62.2460301413079,-62.1456608611438,-62.0451081093007,-61.9492072623393,
-61.8486248382457,-61.7481882267407,-61.6478689043748,-61.5476137343193,
-61.4473913673091,-61.34717049527,-61.2468493790115,-61.1464800988477,-61.0459273470045,
-60.9500265000435,-60.8353267768354,-60.7211028297473,-60.607680245254,
-60.5841007451335),.UNSPECIFIED.);
#1231=B_SPLINE_CURVE_WITH_KNOTS('',3,(#33146,#33147,#33148,#33149,#33150,
#33151,#33152,#33153,#33154,#33155,#33156,#33157,#33158,#33159,#33160,#33161,
#33162,#33163,#33164,#33165,#33166,#33167,#33168,#33169,#33170,#33171,#33172,
#33173,#33174,#33175,#33176,#33177,#33178,#33179,#33180,#33181,#33182,#33183,
#33184,#33185,#33186,#33187,#33188,#33189,#33190,#33191,#33192,#33193,#33194,
#33195,#33196,#33197,#33198,#33199,#33200,#33201,#33202,#33203,#33204,#33205,
#33206,#33207,#33208,#33209,#33210,#33211,#33212,#33213,#33214,#33215,#33216,
#33217,#33218,#33219,#33220,#33221,#33222,#33223,#33224,#33225,#33226,#33227,
#33228,#33229,#33230,#33231,#33232,#33233,#33234,#33235,#33236,#33237,#33238,
#33239,#33240,#33241,#33242,#33243,#33244,#33245,#33246,#33247,#33248,#33249,
#33250,#33251,#33252,#33253,#33254,#33255,#33256,#33257,#33258,#33259,#33260,
#33261,#33262,#33263,#33264,#33265,#33266,#33267,#33268,#33269,#33270,#33271,
#33272,#33273,#33274,#33275,#33276,#33277,#33278,#33279,#33280,#33281,#33282,
#33283,#33284,#33285,#33286,#33287,#33288,#33289,#33290,#33291,#33292,#33293,
#33294,#33295,#33296,#33297,#33298,#33299,#33300,#33301,#33302,#33303,#33304,
#33305,#33306,#33307,#33308,#33309,#33310,#33311,#33312,#33313,#33314,#33315,
#33316,#33317,#33318,#33319,#33320,#33321,#33322,#33323,#33324,#33325,#33326,
#33327,#33328,#33329,#33330,#33331,#33332,#33333,#33334,#33335,#33336,#33337,
#33338),.UNSPECIFIED.,.F.,.F.,(4,3,3,3,3,3,3,3,3,3,3,3,3,3,3,3,3,3,3,3,
3,3,3,3,3,3,3,3,3,3,3,3,3,3,3,3,3,3,3,3,3,3,3,3,3,3,3,3,3,3,3,3,3,3,3,3,
3,3,3,3,3,3,3,3,4),(-60.5841007449008,-60.4833190396952,-60.3825311205423,
-60.2817068382764,-60.1807479736463,-60.0797095309897,-59.978493193977,
-59.9508457377477,-59.850263313654,-59.749826702149,-59.649507379783,-59.5492522097275,
-59.4490298427171,-59.3488089706783,-59.2484878544198,-59.1481185742557,
-59.0475658224124,-58.9516649754519,-58.8510825513582,-58.7506459398535,
-58.6503266174876,-58.5500714474321,-58.4498490804218,-58.3496282083831,
-58.2493070921247,-58.1489378119608,-58.0483850601176,-57.9524842131561,
-57.8519017890623,-57.7514651775573,-57.6511458551914,-57.5508906851359,
-57.4506683181256,-57.3504474460868,-57.2501263298283,-57.1497570496644,
-57.0492042978211,-56.9533034508603,-56.8527210267666,-56.7522844152619,
-56.651965092896,-56.5517099228405,-56.4514875558302,-56.3512666837915,
-56.2509455675331,-56.1505762873691,-56.0500235355259,-55.9541226885645,
-55.8535402644708,-55.7531036529662,-55.6527843306003,-55.5525291605447,
-55.4523067935341,-55.3520859214954,-55.251764805237,-55.1513955250728,
-55.0508427732296,-54.9549419262687,-54.8541907418917,-54.7535843979548,
-54.6530916721567,-54.5526803013764,-54.4523167667248,-54.3519481085295,
-54.3009154377212),.UNSPECIFIED.);
#1232=B_SPLINE_CURVE_WITH_KNOTS('',3,(#33340,#33341,#33342,#33343,#33344,
#33345,#33346,#33347,#33348,#33349,#33350,#33351,#33352,#33353,#33354,#33355,
#33356,#33357,#33358,#33359,#33360,#33361,#33362,#33363,#33364,#33365,#33366,
#33367,#33368,#33369,#33370,#33371,#33372,#33373,#33374,#33375,#33376,#33377,
#33378,#33379,#33380,#33381,#33382,#33383,#33384,#33385,#33386,#33387,#33388,
#33389,#33390,#33391,#33392,#33393,#33394,#33395,#33396,#33397,#33398,#33399,
#33400,#33401,#33402,#33403,#33404,#33405,#33406,#33407,#33408,#33409,#33410,
#33411,#33412,#33413,#33414,#33415,#33416,#33417,#33418,#33419,#33420,#33421,
#33422,#33423,#33424,#33425,#33426,#33427,#33428,#33429,#33430,#33431,#33432,
#33433,#33434,#33435,#33436,#33437,#33438,#33439,#33440,#33441,#33442,#33443,
#33444,#33445,#33446,#33447,#33448,#33449,#33450,#33451,#33452,#33453,#33454,
#33455,#33456,#33457,#33458,#33459,#33460,#33461,#33462,#33463,#33464,#33465,
#33466,#33467,#33468,#33469,#33470,#33471,#33472,#33473,#33474,#33475,#33476,
#33477,#33478,#33479,#33480,#33481,#33482,#33483,#33484,#33485,#33486,#33487,
#33488,#33489,#33490,#33491,#33492,#33493,#33494,#33495,#33496,#33497,#33498,
#33499,#33500,#33501,#33502,#33503,#33504,#33505,#33506,#33507,#33508,#33509,
#33510,#33511,#33512,#33513,#33514,#33515,#33516,#33517,#33518,#33519,#33520,
#33521,#33522,#33523,#33524,#33525,#33526,#33527,#33528,#33529),
 .UNSPECIFIED.,.F.,.F.,(4,3,3,3,3,3,3,3,3,3,3,3,3,3,3,3,3,3,3,3,3,3,3,3,
3,3,3,3,3,3,3,3,3,3,3,3,3,3,3,3,3,3,3,3,3,3,3,3,3,3,3,3,3,3,3,3,3,3,3,3,
3,3,3,4),(-54.3009154374959,-54.185380291694,-54.0687436090842,-53.9557611639729,
-53.855178739879,-53.754742128374,-53.654422806008,-53.5541676359524,-53.4539452689419,
-53.353724396903,-53.2534032806445,-53.1530340004804,-53.052481248637,-52.9565804016771,
-52.8559979775834,-52.7555613660786,-52.6552420437127,-52.5549868736572,
-52.454764506647,-52.3545436346082,-52.2542225183498,-52.1538532381859,
-52.0533004863427,-51.9573996393813,-51.8568172152876,-51.7563806037828,
-51.6560612814169,-51.5558061113614,-51.455583744351,-51.3553628723122,
-51.2550417560538,-51.1546724758898,-51.0541197240466,-50.9582188770855,
-50.8576364529918,-50.757199841487,-50.656880519121,-50.5566253490656,-50.4564029820552,
-50.3561821100164,-50.255860993758,-50.155491713594,-50.0549389617507,-49.9590381147897,
-49.858455690696,-49.7580190791912,-49.6576997568252,-49.5574445867697,
-49.4572222197594,-49.3570013477206,-49.2566802314622,-49.1563109512982,
-49.0557581994549,-48.9598573524939,-48.8601294116964,-48.7605464198726,
-48.6610783124346,-48.5616715488526,-48.4622937332782,-48.3629125092727,
-48.2634343733349,-48.1639015109284,-48.064208747103,-48.0177301309082),
 .UNSPECIFIED.);
#1233=B_SPLINE_CURVE_WITH_KNOTS('',3,(#33531,#33532,#33533,#33534,#33535,
#33536,#33537,#33538,#33539,#33540,#33541,#33542,#33543,#33544,#33545,#33546,
#33547,#33548,#33549,#33550,#33551,#33552,#33553,#33554,#33555,#33556,#33557,
#33558,#33559,#33560,#33561,#33562,#33563,#33564,#33565,#33566,#33567,#33568,
#33569,#33570,#33571,#33572,#33573,#33574,#33575,#33576,#33577,#33578,#33579,
#33580,#33581,#33582,#33583,#33584,#33585,#33586,#33587,#33588,#33589,#33590,
#33591,#33592,#33593,#33594,#33595,#33596,#33597,#33598,#33599,#33600,#33601,
#33602,#33603,#33604,#33605,#33606,#33607,#33608,#33609,#33610,#33611,#33612,
#33613,#33614,#33615,#33616,#33617,#33618,#33619,#33620,#33621,#33622,#33623,
#33624,#33625,#33626,#33627,#33628,#33629,#33630,#33631,#33632,#33633,#33634,
#33635,#33636,#33637,#33638,#33639,#33640,#33641,#33642,#33643,#33644,#33645,
#33646,#33647,#33648,#33649,#33650,#33651,#33652,#33653,#33654,#33655,#33656,
#33657,#33658,#33659,#33660,#33661,#33662,#33663,#33664,#33665,#33666,#33667,
#33668,#33669,#33670,#33671,#33672,#33673,#33674,#33675,#33676,#33677,#33678,
#33679,#33680,#33681,#33682,#33683,#33684,#33685,#33686,#33687,#33688,#33689,
#33690,#33691,#33692,#33693,#33694,#33695,#33696,#33697,#33698,#33699,#33700,
#33701,#33702,#33703,#33704,#33705,#33706,#33707,#33708,#33709,#33710,#33711,
#33712,#33713,#33714,#33715,#33716,#33717,#33718,#33719,#33720),
 .UNSPECIFIED.,.F.,.F.,(4,3,3,3,3,3,3,3,3,3,3,3,3,3,3,3,3,3,3,3,3,3,3,3,
3,3,3,3,3,3,3,3,3,3,3,3,3,3,3,3,3,3,3,3,3,3,3,3,3,3,3,3,3,3,3,3,3,3,3,3,
3,3,3,4),(-48.0177301305417,-47.9606765901981,-47.8600941661048,-47.7596575546004,
-47.6593382322349,-47.5590830621798,-47.45886069517,-47.3586398231315,-47.2583187068736,
-47.1579494267101,-47.0573966748673,-46.9614958279023,-46.8609134038085,
-46.7604767923035,-46.6601574699374,-46.5599022998818,-46.4596799328713,
-46.3594590608323,-46.2591379445738,-46.1587686644096,-46.0582159125662,
-45.9623150656065,-45.8617326415128,-45.761296030008,-45.660976707642,-45.5607215375865,
-45.4604991705762,-45.3602782985374,-45.2599571822789,-45.1595879021149,
-45.0590351502717,-44.9631343033107,-44.862551879217,-44.7621152677123,
-44.6617959453463,-44.5615407752909,-44.4613184082806,-44.3610975362418,
-44.2607764199834,-44.1604071398194,-44.0598543879762,-43.9639535410149,
-43.8633711169212,-43.7629345054164,-43.6626151830505,-43.562360012995,
-43.4621376459846,-43.3619167739458,-43.2615956576874,-43.1612263775234,
-43.0606736256801,-42.9647727787192,-42.8641903546255,-42.7637537431207,
-42.6634344207548,-42.5631792506994,-42.4629568836891,-42.3627360116502,
-42.2624148953918,-42.1620456152278,-42.0614928633846,-41.9655920164234,
-41.830834925829,-41.734544823362),.UNSPECIFIED.);
#1234=B_SPLINE_CURVE_WITH_KNOTS('',3,(#33722,#33723,#33724,#33725,#33726,
#33727,#33728,#33729,#33730,#33731,#33732,#33733,#33734,#33735,#33736,#33737,
#33738,#33739,#33740,#33741,#33742,#33743,#33744,#33745,#33746,#33747,#33748,
#33749,#33750,#33751,#33752,#33753,#33754,#33755,#33756,#33757,#33758,#33759,
#33760,#33761,#33762,#33763,#33764,#33765,#33766,#33767,#33768,#33769,#33770,
#33771,#33772,#33773,#33774,#33775,#33776,#33777,#33778,#33779,#33780,#33781,
#33782,#33783,#33784,#33785,#33786,#33787,#33788,#33789,#33790,#33791,#33792,
#33793,#33794,#33795,#33796,#33797,#33798,#33799,#33800,#33801,#33802,#33803,
#33804,#33805,#33806,#33807,#33808,#33809,#33810,#33811,#33812,#33813,#33814,
#33815,#33816,#33817,#33818,#33819,#33820,#33821,#33822,#33823,#33824,#33825,
#33826,#33827,#33828,#33829,#33830,#33831,#33832,#33833,#33834,#33835,#33836,
#33837,#33838,#33839,#33840,#33841,#33842,#33843,#33844,#33845,#33846,#33847,
#33848,#33849,#33850,#33851,#33852,#33853,#33854,#33855,#33856,#33857,#33858,
#33859,#33860,#33861,#33862,#33863,#33864,#33865,#33866,#33867,#33868,#33869,
#33870,#33871,#33872,#33873,#33874,#33875,#33876,#33877,#33878,#33879,#33880,
#33881,#33882,#33883,#33884,#33885,#33886,#33887,#33888,#33889,#33890,#33891,
#33892,#33893,#33894,#33895,#33896,#33897,#33898,#33899,#33900,#33901,#33902,
#33903,#33904,#33905,#33906,#33907,#33908,#33909,#33910,#33911),
 .UNSPECIFIED.,.F.,.F.,(4,3,3,3,3,3,3,3,3,3,3,3,3,3,3,3,3,3,3,3,3,3,3,3,
3,3,3,3,3,3,3,3,3,3,3,3,3,3,3,3,3,3,3,3,3,3,3,3,3,3,3,3,3,3,3,3,3,3,3,3,
3,3,3,4),(-41.7345448230988,-41.6354972405392,-41.536519530477,-41.4375788402514,
-41.3386423674142,-41.2396110473611,-41.1405312145927,-41.0412784805418,
-40.9664112541276,-40.8658288300339,-40.7653922185292,-40.6650728961633,
-40.5648177261078,-40.4645953590974,-40.3643744870585,-40.2640533708001,
-40.1636840906361,-40.0631313387928,-39.9672304918318,-39.8666480677381,
-39.7662114562332,-39.6658921338672,-39.5656369638116,-39.4654145968013,
-39.3651937247626,-39.2648726085041,-39.1645033283401,-39.0639505764968,
-38.968049729536,-38.8674673054423,-38.7670306939372,-38.6667113715712,
-38.5664562015157,-38.4662338345054,-38.3660129624668,-38.2656918462084,
-38.1653225660444,-38.0647698142011,-37.9688689672402,-37.8682865431464,
-37.7678499316415,-37.6675306092756,-37.56727543922,-37.4670530722098,-37.3668322001707,
-37.2665110839123,-37.1661418037483,-37.0655890519051,-36.9696882049444,
-36.8691057808506,-36.7686691693456,-36.6683498469797,-36.5680946769243,
-36.4678723099141,-36.3676514378752,-36.2673303216168,-36.1669610414528,
-36.0664082896095,-35.9705074426486,-35.8656270199032,-35.7610219707335,
-35.6565790613792,-35.5523314356879,-35.4513595161825),.UNSPECIFIED.);
#1235=B_SPLINE_CURVE_WITH_KNOTS('',3,(#33913,#33914,#33915,#33916,#33917,
#33918,#33919,#33920,#33921,#33922,#33923,#33924,#33925,#33926,#33927,#33928,
#33929,#33930,#33931,#33932,#33933,#33934,#33935,#33936,#33937,#33938,#33939,
#33940,#33941,#33942,#33943,#33944,#33945,#33946,#33947,#33948,#33949,#33950,
#33951,#33952,#33953,#33954,#33955,#33956,#33957,#33958,#33959,#33960,#33961,
#33962,#33963,#33964,#33965,#33966,#33967,#33968,#33969,#33970,#33971,#33972,
#33973,#33974,#33975,#33976,#33977,#33978,#33979,#33980,#33981,#33982,#33983,
#33984,#33985,#33986,#33987,#33988,#33989,#33990,#33991,#33992,#33993,#33994,
#33995,#33996,#33997,#33998,#33999,#34000,#34001,#34002,#34003,#34004,#34005,
#34006,#34007,#34008,#34009,#34010,#34011,#34012,#34013,#34014,#34015,#34016,
#34017,#34018,#34019,#34020,#34021,#34022,#34023,#34024,#34025,#34026,#34027,
#34028,#34029,#34030,#34031,#34032,#34033,#34034,#34035,#34036,#34037,#34038,
#34039,#34040,#34041,#34042,#34043,#34044,#34045,#34046,#34047,#34048,#34049,
#34050,#34051,#34052,#34053,#34054,#34055,#34056,#34057,#34058,#34059,#34060,
#34061,#34062,#34063,#34064,#34065,#34066,#34067,#34068,#34069,#34070,#34071,
#34072,#34073,#34074,#34075,#34076,#34077,#34078,#34079,#34080,#34081,#34082,
#34083,#34084,#34085,#34086,#34087,#34088,#34089,#34090,#34091,#34092,#34093,
#34094,#34095,#34096,#34097,#34098,#34099,#34100,#34101,#34102,#34103,#34104,
#34105),.UNSPECIFIED.,.F.,.F.,(4,3,3,3,3,3,3,3,3,3,3,3,3,3,3,3,3,3,3,3,
3,3,3,3,3,3,3,3,3,3,3,3,3,3,3,3,3,3,3,3,3,3,3,3,3,3,3,3,3,3,3,3,3,3,3,3,
3,3,3,3,3,3,3,3,4),(-35.4513595157648,-35.345485624045,-35.2392752592576,
-35.1328871370317,-35.0261959781545,-34.9713266803528,-34.8707442562593,
-34.7703076447547,-34.6699883223889,-34.5697331523335,-34.4695107853233,
-34.3692899132845,-34.2689687970262,-34.1685995168624,-34.0680467650193,
-33.972145918057,-33.8715634939634,-33.7711268824587,-33.6708075600929,
-33.5705523900376,-33.4703300230273,-33.3701091509886,-33.2697880347303,
-33.1694187545665,-33.0688660027233,-32.9729651557612,-32.8723827316669,
-32.7719461201616,-32.6716267977951,-32.5713716277391,-32.4711492607282,
-32.3709283886889,-32.2706072724299,-32.1702379922654,-32.0696852404216,
-31.9737843934654,-31.8732019693723,-31.7727653578681,-31.6724460355027,
-31.5721908654478,-31.471968498438,-31.3717476263997,-31.2714265101418,
-31.1710572299784,-31.0705044781357,-30.9746036311696,-30.8740212070767,
-30.7735845955729,-30.6732652732078,-30.5730101031532,-30.4727877361437,
-30.3725668641058,-30.2722457478483,-30.1718764676851,-30.0713237158428,
-29.9754228688738,-29.8745167864168,-29.7755770001772,-29.6767314645433,
-29.577947102431,-29.4755038791276,-29.3767031531877,-29.2778723689772,
-29.1789381542911,-29.1681742092176),.UNSPECIFIED.);
#1236=B_SPLINE_CURVE_WITH_KNOTS('',3,(#34107,#34108,#34109,#34110,#34111,
#34112,#34113,#34114,#34115,#34116,#34117,#34118,#34119,#34120,#34121,#34122,
#34123,#34124,#34125,#34126,#34127,#34128,#34129,#34130,#34131,#34132,#34133,
#34134,#34135,#34136,#34137,#34138,#34139,#34140,#34141,#34142,#34143,#34144,
#34145,#34146,#34147,#34148,#34149,#34150,#34151,#34152,#34153,#34154,#34155,
#34156,#34157,#34158,#34159,#34160,#34161,#34162,#34163,#34164,#34165,#34166,
#34167,#34168,#34169,#34170,#34171,#34172,#34173,#34174,#34175,#34176,#34177,
#34178,#34179,#34180,#34181,#34182,#34183,#34184,#34185,#34186,#34187,#34188,
#34189,#34190,#34191,#34192,#34193,#34194,#34195,#34196,#34197,#34198,#34199,
#34200,#34201,#34202,#34203,#34204,#34205,#34206,#34207,#34208,#34209,#34210,
#34211,#34212,#34213,#34214,#34215,#34216,#34217,#34218,#34219,#34220,#34221,
#34222,#34223,#34224,#34225,#34226,#34227,#34228,#34229,#34230,#34231,#34232,
#34233,#34234,#34235,#34236,#34237,#34238,#34239,#34240,#34241,#34242,#34243,
#34244,#34245,#34246,#34247,#34248,#34249,#34250,#34251,#34252,#34253,#34254,
#34255,#34256,#34257,#34258,#34259,#34260,#34261,#34262,#34263,#34264,#34265,
#34266,#34267,#34268,#34269,#34270,#34271,#34272,#34273,#34274,#34275,#34276,
#34277,#34278,#34279,#34280,#34281,#34282,#34283,#34284,#34285,#34286,#34287,
#34288,#34289,#34290,#34291,#34292,#34293,#34294,#34295,#34296),
 .UNSPECIFIED.,.F.,.F.,(4,3,3,3,3,3,3,3,3,3,3,3,3,3,3,3,3,3,3,3,3,3,3,3,
3,3,3,3,3,3,3,3,3,3,3,3,3,3,3,3,3,3,3,3,3,3,3,3,3,3,3,3,3,3,3,3,3,3,3,3,
3,3,3,4),(-29.1681742090029,-29.0208248230063,-28.976242106578,-28.8756596824898,
-28.7752230709906,-28.6749037486302,-28.5746485785802,-28.4744262115752,
-28.3742053395417,-28.2738842232886,-28.1735149431298,-28.0729621912916,
-27.9770613442822,-27.876478920193,-27.7760423086927,-27.6757229863314,
-27.5754678162805,-27.4752454492749,-27.3750245772408,-27.2747034609872,
-27.174334180828,-27.0737814289895,-26.9778805819864,-26.8772981578615,
-26.7768615463255,-26.6765422239283,-26.5762870538417,-26.4760646868002,
-26.3758438147304,-26.2755226984413,-26.1751534182469,-26.0746006663738,
-25.9786998196906,-25.8781173956462,-25.7776807841907,-25.6773614618735,
-25.5771062918666,-25.4768839249044,-25.3766630529134,-25.2763419367019,
-25.1759726565842,-25.0754199047861,-24.9795190573949,-24.8789366333182,
-24.778500021831,-24.6781806994834,-24.5779255294467,-24.4777031624557,
-24.3774822904366,-24.2771611741983,-24.1767918940548,-24.0762391422323,
-23.9803382950991,-23.8797558707739,-23.7793192590369,-23.6789999364387,
-23.578744766151,-23.4785223989088,-23.3783015266388,-23.277980410152,-23.1776111297607,
-23.0770583776947,-22.9811575328033,-22.8849889018233),.UNSPECIFIED.);
#1237=B_SPLINE_CURVE_WITH_KNOTS('',3,(#34298,#34299,#34300,#34301,#34302,
#34303,#34304,#34305,#34306,#34307,#34308,#34309,#34310,#34311,#34312,#34313,
#34314,#34315,#34316,#34317,#34318,#34319,#34320,#34321,#34322,#34323,#34324,
#34325,#34326,#34327,#34328,#34329,#34330,#34331,#34332,#34333,#34334,#34335,
#34336,#34337,#34338,#34339,#34340,#34341,#34342,#34343,#34344,#34345,#34346,
#34347,#34348,#34349,#34350,#34351,#34352,#34353,#34354,#34355,#34356,#34357,
#34358,#34359,#34360,#34361,#34362,#34363,#34364,#34365,#34366,#34367,#34368,
#34369,#34370,#34371,#34372,#34373,#34374,#34375,#34376,#34377,#34378,#34379,
#34380,#34381,#34382,#34383,#34384,#34385,#34386,#34387,#34388,#34389,#34390,
#34391,#34392,#34393,#34394,#34395,#34396,#34397,#34398,#34399,#34400,#34401,
#34402,#34403,#34404,#34405,#34406,#34407,#34408,#34409,#34410,#34411,#34412,
#34413,#34414,#34415,#34416,#34417,#34418,#34419,#34420,#34421,#34422,#34423,
#34424,#34425,#34426,#34427,#34428,#34429,#34430,#34431,#34432,#34433,#34434,
#34435,#34436,#34437,#34438,#34439,#34440,#34441,#34442,#34443,#34444,#34445,
#34446,#34447,#34448,#34449,#34450,#34451,#34452,#34453,#34454,#34455,#34456,
#34457,#34458,#34459,#34460,#34461,#34462,#34463,#34464,#34465,#34466,#34467,
#34468,#34469,#34470,#34471,#34472,#34473,#34474,#34475,#34476,#34477,#34478,
#34479,#34480,#34481,#34482,#34483,#34484,#34485,#34486,#34487),
 .UNSPECIFIED.,.F.,.F.,(4,3,3,3,3,3,3,3,3,3,3,3,3,3,3,3,3,3,3,3,3,3,3,3,
3,3,3,3,3,3,3,3,3,3,3,3,3,3,3,3,3,3,3,3,3,3,3,3,3,3,3,3,3,3,3,3,3,3,3,3,
3,3,3,4),(-22.8849889015957,-22.785692606535,-22.6852281270316,-22.5861595338316,
-22.4871388318715,-22.3881332689759,-22.2865941443588,-22.1874612031866,
-22.0847189868471,-21.9819767705075,-21.8813943464021,-21.7809577348901,
-21.6806384125236,-21.5803832424715,-21.4801608754687,-21.3799400034411,
-21.2796188872001,-21.1792496070569,-21.0786968552397,-20.9827960082117,
-20.8822135824413,-20.7817769692529,-20.6814576452008,-20.5812024734585,
-20.4809801047627,-20.3807592310424,-20.2804381131202,-20.1800688312996,
-20.0795160778312,-19.9836152459159,-19.883032825475,-19.7825962176206,
-19.6822768988838,-19.5820217324432,-19.4817993690288,-19.3815785005619,
-19.2812573878133,-19.1808881111309,-19.0803353626801,-18.9844344836201,
-18.8838520582959,-18.7834154455939,-18.6830961220852,-18.5828409509208,
-18.4826185828361,-18.3823977097594,-18.2820765925266,-18.1817073114211,
-18.0811545587033,-17.9852537213243,-17.8846712854417,-17.7842346620878,
-17.6839153278377,-17.5836601458819,-17.4834377669715,-17.3832168830492,
-17.2828957550165,-17.1825264631186,-17.0819736997497,-16.9860729590285,
-16.8730392479783,-16.7604081100515,-16.6484609984442,-16.6018035948693),
 .UNSPECIFIED.);
#1238=B_SPLINE_CURVE_WITH_KNOTS('',3,(#34489,#34490,#34491,#34492,#34493,
#34494,#34495,#34496,#34497,#34498,#34499,#34500,#34501,#34502,#34503,#34504,
#34505,#34506,#34507,#34508,#34509,#34510,#34511,#34512,#34513,#34514,#34515,
#34516,#34517,#34518,#34519,#34520,#34521,#34522,#34523,#34524,#34525,#34526,
#34527,#34528,#34529,#34530,#34531,#34532,#34533,#34534,#34535,#34536,#34537,
#34538,#34539,#34540,#34541,#34542,#34543,#34544,#34545,#34546,#34547,#34548,
#34549,#34550,#34551,#34552,#34553,#34554,#34555,#34556,#34557,#34558,#34559,
#34560,#34561,#34562,#34563,#34564,#34565,#34566,#34567,#34568,#34569,#34570,
#34571,#34572,#34573,#34574,#34575,#34576,#34577,#34578,#34579,#34580,#34581,
#34582,#34583,#34584,#34585,#34586,#34587,#34588,#34589,#34590,#34591,#34592,
#34593,#34594,#34595,#34596,#34597,#34598,#34599,#34600,#34601,#34602,#34603,
#34604,#34605,#34606,#34607,#34608,#34609,#34610,#34611,#34612,#34613,#34614,
#34615,#34616,#34617,#34618,#34619,#34620,#34621,#34622,#34623,#34624,#34625,
#34626,#34627,#34628,#34629,#34630,#34631,#34632,#34633,#34634,#34635,#34636,
#34637,#34638,#34639,#34640,#34641,#34642,#34643,#34644,#34645,#34646,#34647,
#34648,#34649,#34650,#34651,#34652,#34653,#34654,#34655,#34656,#34657,#34658,
#34659,#34660,#34661,#34662,#34663,#34664,#34665,#34666,#34667,#34668,#34669,
#34670,#34671,#34672,#34673,#34674,#34675,#34676,#34677,#34678),
 .UNSPECIFIED.,.F.,.F.,(4,3,3,3,3,3,3,3,3,3,3,3,3,3,3,3,3,3,3,3,3,3,3,3,
3,3,3,3,3,3,3,3,3,3,3,3,3,3,3,3,3,3,3,3,3,3,3,3,3,3,3,3,3,3,3,3,3,3,3,3,
3,3,3,4),(-16.6018035946437,-16.5006122134358,-16.3993999728341,-16.2962730288087,
-16.1948628929016,-16.0908775448171,-15.9868921967327,-15.8863097542278,
-15.785873124552,-15.6855537844569,-15.5852985969477,-15.4850762127801,
-15.384855323902,-15.2845341914182,-15.1841648953368,-15.0836121282851,
-14.9877114344369,-14.8871289305195,-14.7866922386777,-14.6863728355818,
-14.5861175845928,-14.4858951365572,-14.3856741835129,-14.2853529868507,
-14.184983626479,-14.0844307957194,-13.9885306721411,-13.8879484924996,
-13.7875121256017,-13.6871930469416,-13.5869381199415,-13.4867159950122,
-13.3864953637554,-13.2861744845588,-13.1858054398181,-13.0852529178185,
-12.9893499098453,-12.8887672754061,-12.7883304552521,-12.6880109277277,
-12.587755554717,-12.4875329872103,-12.387311917392,-12.2869906089774,-12.1866211394074,
-12.0860682050563,-11.9901691475495,-11.8895862098247,-11.7891490804281,
-11.6888292362236,-11.5885735421607,-11.4883506497053,-11.388129251512,
-11.287807611706,-11.187437808555,-11.0868845409385,-10.9909883852537,-10.8905873154232,
-10.790327535112,-10.6901773093172,-10.5900985337102,-10.4900634929034,
-10.3900077170264,-10.3186182874641),.UNSPECIFIED.);
#1239=B_SPLINE_CURVE_WITH_KNOTS('',3,(#34679,#34680,#34681,#34682,#34683,
#34684,#34685,#34686,#34687,#34688,#34689,#34690,#34691,#34692,#34693,#34694,
#34695,#34696,#34697,#34698,#34699,#34700,#34701,#34702,#34703,#34704,#34705,
#34706,#34707,#34708,#34709,#34710,#34711,#34712,#34713,#34714,#34715,#34716,
#34717,#34718,#34719,#34720,#34721,#34722,#34723,#34724,#34725,#34726,#34727,
#34728,#34729,#34730,#34731,#34732,#34733,#34734,#34735,#34736,#34737,#34738,
#34739,#34740,#34741,#34742,#34743,#34744,#34745,#34746,#34747,#34748,#34749,
#34750,#34751,#34752,#34753,#34754,#34755,#34756,#34757,#34758,#34759,#34760,
#34761,#34762,#34763,#34764,#34765,#34766,#34767,#34768,#34769,#34770,#34771,
#34772,#34773,#34774,#34775,#34776,#34777,#34778,#34779,#34780,#34781,#34782,
#34783,#34784,#34785,#34786,#34787,#34788,#34789,#34790,#34791,#34792,#34793,
#34794,#34795,#34796,#34797,#34798,#34799,#34800,#34801,#34802,#34803,#34804,
#34805,#34806,#34807,#34808,#34809,#34810,#34811,#34812,#34813,#34814,#34815,
#34816,#34817,#34818,#34819,#34820,#34821,#34822,#34823,#34824,#34825,#34826,
#34827,#34828,#34829,#34830,#34831,#34832,#34833,#34834,#34835,#34836,#34837,
#34838,#34839,#34840,#34841,#34842,#34843,#34844,#34845,#34846,#34847,#34848,
#34849,#34850,#34851,#34852,#34853,#34854,#34855,#34856,#34857,#34858,#34859,
#34860,#34861,#34862,#34863,#34864,#34865,#34866,#34867,#34868),
 .UNSPECIFIED.,.F.,.F.,(4,3,3,3,3,3,3,3,3,3,3,3,3,3,3,3,3,3,3,3,3,3,3,3,
3,3,3,3,3,3,3,3,3,3,3,3,3,3,3,3,3,3,3,3,3,3,3,3,3,3,3,3,3,3,3,3,3,3,3,3,
3,3,3,4),(-10.3186182870443,-10.2011545560181,-10.0823918979535,-9.99180762295794,
-9.89122306431455,-9.79078432980569,-9.6904629114498,-9.59020566267282,
-9.48998123687609,-9.38975832867021,-9.28943522581426,-9.18906398281329,
-9.08850933164576,-8.99262686066215,-8.8920413763641,-8.79160167008605,
-8.6912792158045,-8.59102089266657,-8.49079535587881,-8.39057130182047,
-8.29024700692928,-8.18987454475535,-8.08931864337274,-7.99344609836635,
-7.89287868600335,-7.79245711482735,-7.69215280587807,-7.59191262656223,
-7.49170520752304,-7.39149922056677,-7.29119278659681,-7.19083810235733,
-7.09029962607513,-6.99426533607056,-6.89366269493674,-6.79320594127186,
-6.69286668158642,-6.59259170697504,-6.49234969393895,-6.39210936030836,
-6.29176920688027,-6.19138108976055,-6.09081006357693,-5.99508457377476,
-5.89448625755712,-5.79403347902593,-5.69369765531915,-5.59342578844064,
-5.49318655361032,-5.3929486670598,-5.29261042807389,-5.19222393808779,
-5.0916540362804,-4.99590381147897,-4.896050224785,-4.79634212419318,-4.69674938914012,
-4.59721866292036,-4.49771769171307,-4.39821426140152,-4.29861090058313,
-4.19895407607732,-4.09912709998999,-4.0354329805645),.UNSPECIFIED.);
#1240=B_SPLINE_CURVE_WITH_KNOTS('',3,(#34871,#34872,#34873,#34874,#34875,
#34876,#34877,#34878,#34879,#34880,#34881,#34882,#34883,#34884,#34885,#34886,
#34887,#34888,#34889,#34890,#34891,#34892,#34893,#34894,#34895,#34896,#34897,
#34898,#34899,#34900,#34901,#34902,#34903,#34904,#34905,#34906,#34907,#34908,
#34909,#34910,#34911,#34912,#34913,#34914,#34915,#34916,#34917,#34918,#34919,
#34920),.UNSPECIFIED.,.F.,.F.,(4,2,2,2,2,2,2,2,2,2,2,2,2,2,2,2,2,2,2,2,
2,2,2,2,4),(-0.242412075418231,-0.24068258493173,-0.23876015295065,-0.23726279880318,
-0.235498379397621,-0.232535044312713,-0.217554658625273,-0.175019001490325,
-0.150773707812734,-0.145414945615575,-0.142318515927924,-0.139655388881361,
-0.136404372732187,-0.130628635693296,-0.10322634121326,-0.0796420139484518,
-0.0505808179684192,-0.0474274175871481,-0.0454937459518301,-0.0439922154119611,
-0.0422271644585061,-0.0403423932910817,-0.0373729963661339,-0.0315833569543321,
-0.000576332490211338),.UNSPECIFIED.);
#1241=B_SPLINE_CURVE_WITH_KNOTS('',3,(#34922,#34923,#34924,#34925,#34926,
#34927,#34928,#34929,#34930,#34931,#34932,#34933,#34934,#34935,#34936,#34937,
#34938,#34939,#34940,#34941,#34942,#34943,#34944,#34945,#34946,#34947,#34948,
#34949,#34950,#34951,#34952,#34953,#34954,#34955,#34956,#34957,#34958,#34959,
#34960,#34961,#34962,#34963,#34964,#34965,#34966,#34967,#34968,#34969,#34970,
#34971,#34972,#34973,#34974,#34975,#34976,#34977,#34978,#34979,#34980,#34981,
#34982,#34983,#34984,#34985,#34986,#34987,#34988,#34989,#34990,#34991,#34992,
#34993,#34994,#34995,#34996,#34997,#34998,#34999,#35000,#35001,#35002,#35003,
#35004,#35005,#35006,#35007,#35008,#35009,#35010,#35011,#35012,#35013,#35014,
#35015,#35016,#35017,#35018,#35019,#35020,#35021,#35022,#35023,#35024,#35025,
#35026,#35027,#35028,#35029,#35030,#35031,#35032,#35033,#35034,#35035,#35036,
#35037,#35038,#35039),.UNSPECIFIED.,.F.,.F.,(4,3,3,3,3,3,3,3,3,3,3,3,3,
3,3,3,3,3,3,3,3,3,3,3,3,3,3,3,3,3,3,3,3,3,3,3,3,3,3,4),(128.805298797457,
128.909530301967,129.013684715498,129.117800270842,129.221915141085,129.326134956294,
129.430415400967,129.534872675319,129.575860238568,129.681560904871,129.787100864418,
129.892515952901,129.997864692822,130.103183758175,130.208509778359,130.313950456587,
130.419455685508,130.525146421068,130.575041000864,130.681053929543,130.78690594986,
130.892631297518,130.998288997924,131.103915267213,131.20954627527,131.315286538609,
131.421088702291,131.527069210927,131.57422176316,131.680115426827,131.785850999542,
131.891464565972,131.997013443811,132.102533989557,132.208062516701,132.313705829073,
132.419414064884,132.525306211834,132.573402525455,132.586742025829),
 .UNSPECIFIED.);
#1242=B_SPLINE_CURVE_WITH_KNOTS('',3,(#35043,#35044,#35045,#35046,#35047,
#35048,#35049,#35050,#35051,#35052,#35053,#35054,#35055,#35056,#35057,#35058,
#35059,#35060,#35061,#35062,#35063,#35064,#35065,#35066,#35067,#35068,#35069,
#35070,#35071,#35072,#35073,#35074,#35075,#35076,#35077,#35078,#35079,#35080,
#35081,#35082,#35083,#35084,#35085,#35086,#35087,#35088,#35089,#35090,#35091,
#35092,#35093,#35094,#35095,#35096,#35097,#35098,#35099,#35100,#35101,#35102,
#35103,#35104,#35105,#35106,#35107,#35108,#35109,#35110,#35111,#35112,#35113,
#35114,#35115),.UNSPECIFIED.,.F.,.F.,(4,3,3,3,3,3,3,3,3,3,3,3,3,3,3,3,3,
3,3,3,3,3,3,3,4),(128.805298797453,128.920686329815,129.036431940841,129.152706586493,
129.234468501037,129.339286844061,129.443944512182,129.54848134576,129.652954615654,
129.757402129115,129.861861652104,129.966449229204,130.071107485331,130.175969886253,
130.233649263333,130.342332107421,130.453644347197,130.561962326317,130.670177107086,
130.778318699004,130.89194653066,131.000061984321,131.108188597098,131.216390672611,
131.232830025629),.UNSPECIFIED.);
#1243=B_SPLINE_CURVE_WITH_KNOTS('',3,(#35116,#35117,#35118,#35119,#35120,
#35121,#35122,#35123,#35124,#35125,#35126,#35127,#35128,#35129,#35130,#35131,
#35132,#35133,#35134,#35135,#35136,#35137,#35138,#35139,#35140,#35141,#35142,
#35143,#35144,#35145,#35146,#35147,#35148,#35149,#35150,#35151,#35152,#35153,
#35154,#35155,#35156,#35157,#35158,#35159,#35160,#35161,#35162,#35163,#35164,
#35165,#35166,#35167,#35168,#35169),.UNSPECIFIED.,.F.,.F.,(4,2,2,2,2,2,
2,2,2,2,2,2,2,2,2,2,2,2,2,2,2,2,2,2,2,2,4),(-2.43052060028278,-2.42452327733995,
-2.41980014231107,-2.41714485996155,-2.41455047789507,-2.4116171269049,
-2.40697072271808,-2.39259337102949,-2.34514218860885,-2.33228857955003,
-2.32712859312713,-2.3232333540881,-2.32131082001195,-2.31993325557163,
-2.31817269023445,-2.31507196203576,-2.30138252764729,-2.24861046291519,
-2.23777801862789,-2.2322815284433,-2.22882458265371,-2.22563133019317,
-2.22300679682425,-2.21991811223185,-2.21463391519929,-2.19212759162886,
-2.18849108915717),.UNSPECIFIED.);
#1244=B_SPLINE_CURVE_WITH_KNOTS('',3,(#35173,#35174,#35175,#35176,#35177,
#35178,#35179,#35180,#35181,#35182,#35183,#35184,#35185,#35186,#35187,#35188,
#35189,#35190,#35191,#35192,#35193,#35194,#35195,#35196,#35197,#35198,#35199,
#35200,#35201,#35202,#35203,#35204,#35205,#35206,#35207,#35208,#35209,#35210,
#35211,#35212,#35213,#35214,#35215,#35216,#35217,#35218,#35219,#35220,#35221,
#35222,#35223,#35224,#35225,#35226,#35227,#35228,#35229,#35230,#35231,#35232,
#35233,#35234,#35235,#35236,#35237,#35238,#35239,#35240,#35241,#35242,#35243,
#35244,#35245,#35246,#35247,#35248,#35249,#35250,#35251),.UNSPECIFIED.,
 .F.,.F.,(4,3,3,3,3,3,3,3,3,3,3,3,3,3,3,3,3,3,3,3,3,3,3,3,3,3,4),(-0.423931964449299,
-0.398828895834902,-0.377505476130339,-0.372498818727613,-0.347705174956756,
-0.32990042178538,-0.325542832515127,-0.321200290882412,-0.297020641771167,
-0.273379185129757,-0.250225980523141,-0.239676135708419,-0.235939475515521,
-0.213014612686521,-0.205267149585748,-0.181769288410816,-0.159132288662692,
-0.153558814986012,-0.130782794694077,-0.108108185525988,-0.0856259844313709,
-0.0774184937638966,-0.0738810096236942,-0.0519894683140413,-0.030460990690467,
-0.00962200678755835,-1.16575970560916E-14),.UNSPECIFIED.);
#1245=B_SPLINE_CURVE_WITH_KNOTS('',3,(#35252,#35253,#35254,#35255,#35256,
#35257,#35258,#35259,#35260,#35261,#35262,#35263,#35264,#35265,#35266,#35267,
#35268,#35269,#35270,#35271,#35272,#35273,#35274,#35275,#35276,#35277,#35278,
#35279,#35280,#35281,#35282,#35283,#35284,#35285,#35286,#35287,#35288,#35289,
#35290,#35291,#35292,#35293,#35294,#35295,#35296,#35297,#35298,#35299,#35300,
#35301,#35302,#35303,#35304,#35305,#35306,#35307,#35308,#35309,#35310,#35311,
#35312,#35313,#35314,#35315,#35316,#35317,#35318,#35319,#35320,#35321,#35322,
#35323,#35324,#35325,#35326,#35327,#35328,#35329,#35330),.UNSPECIFIED.,
 .F.,.F.,(4,3,3,3,3,3,3,3,3,3,3,3,3,3,3,3,3,3,3,3,3,3,3,3,3,3,4),(-0.43028912773393,
-0.409095039634617,-0.389617234398967,-0.383301851779856,-0.361178803936431,
-0.343501455552783,-0.339161608446753,-0.316328762903765,-0.293495917360776,
-0.27693657759957,-0.264333174521167,-0.258637327723869,-0.234922334847588,
-0.227258558315955,-0.204133994215651,-0.181009430115347,-0.177044799294305,
-0.153366378725593,-0.129080143187624,-0.104793907649655,-0.0968425625095517,
-0.0919203420448217,-0.0878017623663734,-0.0627749710934861,-0.0377028824416867,
-0.0131606293708096,0.),.UNSPECIFIED.);
#1246=B_SPLINE_CURVE_WITH_KNOTS('',3,(#35835,#35836,#35837,#35838),
 .UNSPECIFIED.,.F.,.F.,(4,4),(-0.0446554005265974,0.),.UNSPECIFIED.);
#1247=B_SPLINE_CURVE_WITH_KNOTS('',3,(#35839,#35840,#35841,#35842,#35843,
#35844,#35845,#35846,#35847,#35848,#35849,#35850,#35851,#35852,#35853,#35854,
#35855,#35856,#35857,#35858,#35859,#35860,#35861,#35862,#35863,#35864,#35865,
#35866,#35867,#35868,#35869,#35870,#35871,#35872,#35873,#35874,#35875,#35876,
#35877,#35878,#35879,#35880,#35881,#35882,#35883,#35884,#35885,#35886,#35887,
#35888,#35889,#35890,#35891,#35892,#35893,#35894,#35895,#35896,#35897,#35898,
#35899,#35900,#35901,#35902,#35903,#35904,#35905,#35906,#35907,#35908,#35909,
#35910,#35911,#35912,#35913,#35914,#35915,#35916,#35917),.UNSPECIFIED.,
 .F.,.F.,(4,3,3,3,3,3,3,3,3,3,3,3,3,3,3,3,3,3,3,3,3,3,3,3,3,3,4),(-0.430284631122155,
-0.409090485009149,-0.389617069570191,-0.38330183976251,-0.361188616218542,
-0.343501442591732,-0.339161607595677,-0.316328764317089,-0.293495921038502,
-0.276936580357852,-0.26433317834727,-0.258637326590171,-0.234922332869949,
-0.227258558315902,-0.204375919054567,-0.181009440361364,-0.177044805514887,
-0.153366390422607,-0.129080158372962,-0.104793926323317,-0.0968425970791397,
-0.0919205100039578,-0.0878017655959253,-0.0628154480136494,-0.0378426001661505,
-0.0131606168603668,0.),.UNSPECIFIED.);
#1248=B_SPLINE_CURVE_WITH_KNOTS('',3,(#35922,#35923,#35924,#35925,#35926,
#35927,#35928,#35929,#35930,#35931,#35932,#35933,#35934,#35935,#35936,#35937,
#35938,#35939,#35940,#35941,#35942,#35943,#35944,#35945,#35946,#35947,#35948,
#35949,#35950,#35951,#35952,#35953,#35954,#35955,#35956,#35957,#35958,#35959,
#35960,#35961,#35962,#35963,#35964,#35965,#35966,#35967,#35968,#35969,#35970,
#35971,#35972,#35973,#35974,#35975,#35976,#35977,#35978,#35979,#35980,#35981,
#35982,#35983,#35984,#35985,#35986,#35987,#35988,#35989,#35990,#35991,#35992,
#35993,#35994,#35995,#35996,#35997,#35998,#35999,#36000),.UNSPECIFIED.,
 .F.,.F.,(4,3,3,3,3,3,3,3,3,3,3,3,3,3,3,3,3,3,3,3,3,3,3,3,3,3,4),(-0.423931917983707,
-0.398828849205038,-0.377505459037515,-0.372498795999555,-0.347705151353274,
-0.329900401132338,-0.325542781731763,-0.321200279025117,-0.297020628104016,
-0.273379162081259,-0.250225943592493,-0.239676120732133,-0.235939452644732,
-0.213014579934855,-0.205267149585788,-0.181769286159282,-0.159132282983792,
-0.153558817716272,-0.130782793604138,-0.108108193702964,-0.0856260055726251,
-0.0774185049266986,-0.0738810206053447,-0.0519894904181288,-0.0306843036419977,
-0.00962206573183614,-7.03132749747345E-15),.UNSPECIFIED.);
#1249=B_SPLINE_CURVE_WITH_KNOTS('',3,(#36506,#36507,#36508,#36509),
 .UNSPECIFIED.,.F.,.F.,(4,4),(-0.0447834994719192,0.),.UNSPECIFIED.);
#1559=FACE_BOUND('',#2963,.T.);
#1560=FACE_BOUND('',#3077,.T.);
#1652=PLANE('',#14141);
#1653=PLANE('',#14143);
#1654=PLANE('',#14149);
#1655=PLANE('',#14153);
#1656=PLANE('',#14154);
#1657=PLANE('',#14155);
#1658=PLANE('',#14156);
#1659=PLANE('',#14196);
#1660=PLANE('',#14197);
#1661=PLANE('',#14198);
#1662=PLANE('',#14200);
#1663=PLANE('',#14201);
#1664=PLANE('',#14202);
#1665=PLANE('',#14204);
#1666=PLANE('',#14205);
#1667=PLANE('',#14206);
#1668=PLANE('',#14208);
#1669=PLANE('',#14209);
#1670=PLANE('',#14210);
#1671=PLANE('',#14212);
#1672=PLANE('',#14213);
#1673=PLANE('',#14214);
#1674=PLANE('',#14216);
#1675=PLANE('',#14217);
#1676=PLANE('',#14218);
#1677=PLANE('',#14220);
#1678=PLANE('',#14221);
#1679=PLANE('',#14222);
#1680=PLANE('',#14224);
#1681=PLANE('',#14225);
#1682=PLANE('',#14226);
#1683=PLANE('',#14228);
#1684=PLANE('',#14229);
#1685=PLANE('',#14230);
#1686=PLANE('',#14232);
#1687=PLANE('',#14233);
#1688=PLANE('',#14234);
#1689=PLANE('',#14236);
#1690=PLANE('',#14237);
#1691=PLANE('',#14238);
#1692=PLANE('',#14240);
#1693=PLANE('',#14241);
#1694=PLANE('',#14242);
#1695=PLANE('',#14244);
#1696=PLANE('',#14245);
#1697=PLANE('',#14246);
#1698=PLANE('',#14248);
#1699=PLANE('',#14249);
#1700=PLANE('',#14250);
#1701=PLANE('',#14252);
#1702=PLANE('',#14253);
#1703=PLANE('',#14254);
#1704=PLANE('',#14256);
#1705=PLANE('',#14257);
#1706=PLANE('',#14258);
#1707=PLANE('',#14260);
#1708=PLANE('',#14261);
#1709=PLANE('',#14262);
#1710=PLANE('',#14265);
#1711=PLANE('',#14266);
#1712=PLANE('',#14267);
#1713=PLANE('',#14269);
#1714=PLANE('',#14270);
#1715=PLANE('',#14271);
#1716=PLANE('',#14273);
#1717=PLANE('',#14274);
#1718=PLANE('',#14275);
#1719=PLANE('',#14277);
#1720=PLANE('',#14278);
#1721=PLANE('',#14279);
#1722=PLANE('',#14281);
#1723=PLANE('',#14282);
#1724=PLANE('',#14283);
#1725=PLANE('',#14285);
#1726=PLANE('',#14286);
#1727=PLANE('',#14287);
#1728=PLANE('',#14289);
#1729=PLANE('',#14290);
#1730=PLANE('',#14291);
#1731=PLANE('',#14293);
#1732=PLANE('',#14294);
#1733=PLANE('',#14295);
#1734=PLANE('',#14297);
#1735=PLANE('',#14298);
#1736=PLANE('',#14299);
#1737=PLANE('',#14301);
#1738=PLANE('',#14302);
#1739=PLANE('',#14303);
#1740=PLANE('',#14305);
#1741=PLANE('',#14306);
#1742=PLANE('',#14307);
#1743=PLANE('',#14309);
#1744=PLANE('',#14310);
#1745=PLANE('',#14311);
#1746=PLANE('',#14313);
#1747=PLANE('',#14314);
#1748=PLANE('',#14315);
#1749=PLANE('',#14317);
#1750=PLANE('',#14318);
#1751=PLANE('',#14319);
#1752=PLANE('',#14321);
#1753=PLANE('',#14322);
#1754=PLANE('',#14323);
#1755=PLANE('',#14325);
#1756=PLANE('',#14326);
#1757=PLANE('',#14327);
#1758=PLANE('',#14329);
#1759=PLANE('',#14330);
#1760=PLANE('',#14331);
#1761=PLANE('',#14333);
#1762=PLANE('',#14334);
#1763=PLANE('',#14335);
#1764=PLANE('',#14338);
#1765=PLANE('',#14339);
#1766=PLANE('',#14341);
#1767=PLANE('',#14343);
#1768=PLANE('',#14345);
#1769=PLANE('',#14347);
#1770=PLANE('',#14349);
#1771=PLANE('',#14352);
#1772=PLANE('',#14353);
#1773=PLANE('',#14354);
#1774=PLANE('',#14355);
#1775=PLANE('',#14356);
#1776=PLANE('',#14357);
#2213=FACE_OUTER_BOUND('',#2936,.T.);
#2214=FACE_OUTER_BOUND('',#2937,.T.);
#2215=FACE_OUTER_BOUND('',#2938,.T.);
#2216=FACE_OUTER_BOUND('',#2939,.T.);
#2217=FACE_OUTER_BOUND('',#2940,.T.);
#2218=FACE_OUTER_BOUND('',#2941,.T.);
#2219=FACE_OUTER_BOUND('',#2942,.T.);
#2220=FACE_OUTER_BOUND('',#2943,.T.);
#2221=FACE_OUTER_BOUND('',#2944,.T.);
#2222=FACE_OUTER_BOUND('',#2945,.T.);
#2223=FACE_OUTER_BOUND('',#2946,.T.);
#2224=FACE_OUTER_BOUND('',#2947,.T.);
#2225=FACE_OUTER_BOUND('',#2948,.T.);
#2226=FACE_OUTER_BOUND('',#2949,.T.);
#2227=FACE_OUTER_BOUND('',#2950,.T.);
#2228=FACE_OUTER_BOUND('',#2951,.T.);
#2229=FACE_OUTER_BOUND('',#2952,.T.);
#2230=FACE_OUTER_BOUND('',#2953,.T.);
#2231=FACE_OUTER_BOUND('',#2954,.T.);
#2232=FACE_OUTER_BOUND('',#2955,.T.);
#2233=FACE_OUTER_BOUND('',#2956,.T.);
#2234=FACE_OUTER_BOUND('',#2957,.T.);
#2235=FACE_OUTER_BOUND('',#2958,.T.);
#2236=FACE_OUTER_BOUND('',#2959,.T.);
#2237=FACE_OUTER_BOUND('',#2960,.T.);
#2238=FACE_OUTER_BOUND('',#2961,.T.);
#2239=FACE_OUTER_BOUND('',#2962,.T.);
#2240=FACE_OUTER_BOUND('',#2964,.T.);
#2241=FACE_OUTER_BOUND('',#2965,.T.);
#2242=FACE_OUTER_BOUND('',#2966,.T.);
#2243=FACE_OUTER_BOUND('',#2967,.T.);
#2244=FACE_OUTER_BOUND('',#2968,.T.);
#2245=FACE_OUTER_BOUND('',#2969,.T.);
#2246=FACE_OUTER_BOUND('',#2970,.T.);
#2247=FACE_OUTER_BOUND('',#2971,.T.);
#2248=FACE_OUTER_BOUND('',#2972,.T.);
#2249=FACE_OUTER_BOUND('',#2973,.T.);
#2250=FACE_OUTER_BOUND('',#2974,.T.);
#2251=FACE_OUTER_BOUND('',#2975,.T.);
#2252=FACE_OUTER_BOUND('',#2976,.T.);
#2253=FACE_OUTER_BOUND('',#2977,.T.);
#2254=FACE_OUTER_BOUND('',#2978,.T.);
#2255=FACE_OUTER_BOUND('',#2979,.T.);
#2256=FACE_OUTER_BOUND('',#2980,.T.);
#2257=FACE_OUTER_BOUND('',#2981,.T.);
#2258=FACE_OUTER_BOUND('',#2982,.T.);
#2259=FACE_OUTER_BOUND('',#2983,.T.);
#2260=FACE_OUTER_BOUND('',#2984,.T.);
#2261=FACE_OUTER_BOUND('',#2985,.T.);
#2262=FACE_OUTER_BOUND('',#2986,.T.);
#2263=FACE_OUTER_BOUND('',#2987,.T.);
#2264=FACE_OUTER_BOUND('',#2988,.T.);
#2265=FACE_OUTER_BOUND('',#2989,.T.);
#2266=FACE_OUTER_BOUND('',#2990,.T.);
#2267=FACE_OUTER_BOUND('',#2991,.T.);
#2268=FACE_OUTER_BOUND('',#2992,.T.);
#2269=FACE_OUTER_BOUND('',#2993,.T.);
#2270=FACE_OUTER_BOUND('',#2994,.T.);
#2271=FACE_OUTER_BOUND('',#2995,.T.);
#2272=FACE_OUTER_BOUND('',#2996,.T.);
#2273=FACE_OUTER_BOUND('',#2997,.T.);
#2274=FACE_OUTER_BOUND('',#2998,.T.);
#2275=FACE_OUTER_BOUND('',#2999,.T.);
#2276=FACE_OUTER_BOUND('',#3000,.T.);
#2277=FACE_OUTER_BOUND('',#3001,.T.);
#2278=FACE_OUTER_BOUND('',#3002,.T.);
#2279=FACE_OUTER_BOUND('',#3003,.T.);
#2280=FACE_OUTER_BOUND('',#3004,.T.);
#2281=FACE_OUTER_BOUND('',#3005,.T.);
#2282=FACE_OUTER_BOUND('',#3006,.T.);
#2283=FACE_OUTER_BOUND('',#3007,.T.);
#2284=FACE_OUTER_BOUND('',#3008,.T.);
#2285=FACE_OUTER_BOUND('',#3009,.T.);
#2286=FACE_OUTER_BOUND('',#3010,.T.);
#2287=FACE_OUTER_BOUND('',#3011,.T.);
#2288=FACE_OUTER_BOUND('',#3012,.T.);
#2289=FACE_OUTER_BOUND('',#3013,.T.);
#2290=FACE_OUTER_BOUND('',#3014,.T.);
#2291=FACE_OUTER_BOUND('',#3015,.T.);
#2292=FACE_OUTER_BOUND('',#3016,.T.);
#2293=FACE_OUTER_BOUND('',#3017,.T.);
#2294=FACE_OUTER_BOUND('',#3018,.T.);
#2295=FACE_OUTER_BOUND('',#3019,.T.);
#2296=FACE_OUTER_BOUND('',#3020,.T.);
#2297=FACE_OUTER_BOUND('',#3021,.T.);
#2298=FACE_OUTER_BOUND('',#3022,.T.);
#2299=FACE_OUTER_BOUND('',#3023,.T.);
#2300=FACE_OUTER_BOUND('',#3024,.T.);
#2301=FACE_OUTER_BOUND('',#3025,.T.);
#2302=FACE_OUTER_BOUND('',#3026,.T.);
#2303=FACE_OUTER_BOUND('',#3027,.T.);
#2304=FACE_OUTER_BOUND('',#3028,.T.);
#2305=FACE_OUTER_BOUND('',#3029,.T.);
#2306=FACE_OUTER_BOUND('',#3030,.T.);
#2307=FACE_OUTER_BOUND('',#3031,.T.);
#2308=FACE_OUTER_BOUND('',#3032,.T.);
#2309=FACE_OUTER_BOUND('',#3033,.T.);
#2310=FACE_OUTER_BOUND('',#3034,.T.);
#2311=FACE_OUTER_BOUND('',#3035,.T.);
#2312=FACE_OUTER_BOUND('',#3036,.T.);
#2313=FACE_OUTER_BOUND('',#3037,.T.);
#2314=FACE_OUTER_BOUND('',#3038,.T.);
#2315=FACE_OUTER_BOUND('',#3039,.T.);
#2316=FACE_OUTER_BOUND('',#3040,.T.);
#2317=FACE_OUTER_BOUND('',#3041,.T.);
#2318=FACE_OUTER_BOUND('',#3042,.T.);
#2319=FACE_OUTER_BOUND('',#3043,.T.);
#2320=FACE_OUTER_BOUND('',#3044,.T.);
#2321=FACE_OUTER_BOUND('',#3045,.T.);
#2322=FACE_OUTER_BOUND('',#3046,.T.);
#2323=FACE_OUTER_BOUND('',#3047,.T.);
#2324=FACE_OUTER_BOUND('',#3048,.T.);
#2325=FACE_OUTER_BOUND('',#3049,.T.);
#2326=FACE_OUTER_BOUND('',#3050,.T.);
#2327=FACE_OUTER_BOUND('',#3051,.T.);
#2328=FACE_OUTER_BOUND('',#3052,.T.);
#2329=FACE_OUTER_BOUND('',#3053,.T.);
#2330=FACE_OUTER_BOUND('',#3054,.T.);
#2331=FACE_OUTER_BOUND('',#3055,.T.);
#2332=FACE_OUTER_BOUND('',#3056,.T.);
#2333=FACE_OUTER_BOUND('',#3057,.T.);
#2334=FACE_OUTER_BOUND('',#3058,.T.);
#2335=FACE_OUTER_BOUND('',#3059,.T.);
#2336=FACE_OUTER_BOUND('',#3060,.T.);
#2337=FACE_OUTER_BOUND('',#3061,.T.);
#2338=FACE_OUTER_BOUND('',#3062,.T.);
#2339=FACE_OUTER_BOUND('',#3063,.T.);
#2340=FACE_OUTER_BOUND('',#3064,.T.);
#2341=FACE_OUTER_BOUND('',#3065,.T.);
#2342=FACE_OUTER_BOUND('',#3066,.T.);
#2343=FACE_OUTER_BOUND('',#3067,.T.);
#2344=FACE_OUTER_BOUND('',#3068,.T.);
#2345=FACE_OUTER_BOUND('',#3069,.T.);
#2346=FACE_OUTER_BOUND('',#3070,.T.);
#2347=FACE_OUTER_BOUND('',#3071,.T.);
#2348=FACE_OUTER_BOUND('',#3072,.T.);
#2349=FACE_OUTER_BOUND('',#3073,.T.);
#2350=FACE_OUTER_BOUND('',#3074,.T.);
#2351=FACE_OUTER_BOUND('',#3075,.T.);
#2352=FACE_OUTER_BOUND('',#3076,.T.);
#2353=FACE_OUTER_BOUND('',#3078,.T.);
#2354=FACE_OUTER_BOUND('',#3079,.T.);
#2355=FACE_OUTER_BOUND('',#3080,.T.);
#2356=FACE_OUTER_BOUND('',#3081,.T.);
#2357=FACE_OUTER_BOUND('',#3082,.T.);
#2358=FACE_OUTER_BOUND('',#3083,.T.);
#2359=FACE_OUTER_BOUND('',#3084,.T.);
#2360=FACE_OUTER_BOUND('',#3085,.T.);
#2361=FACE_OUTER_BOUND('',#3086,.T.);
#2362=FACE_OUTER_BOUND('',#3087,.T.);
#2363=FACE_OUTER_BOUND('',#3088,.T.);
#2364=FACE_OUTER_BOUND('',#3089,.T.);
#2365=FACE_OUTER_BOUND('',#3090,.T.);
#2936=EDGE_LOOP('',(#9859,#9860,#9861,#9862));
#2937=EDGE_LOOP('',(#9863,#9864,#9865,#9866,#9867,#9868));
#2938=EDGE_LOOP('',(#9869,#9870,#9871,#9872));
#2939=EDGE_LOOP('',(#9873,#9874,#9875,#9876,#9877,#9878));
#2940=EDGE_LOOP('',(#9879,#9880,#9881,#9882));
#2941=EDGE_LOOP('',(#9883,#9884,#9885,#9886,#9887,#9888));
#2942=EDGE_LOOP('',(#9889,#9890,#9891,#9892));
#2943=EDGE_LOOP('',(#9893,#9894,#9895,#9896,#9897,#9898));
#2944=EDGE_LOOP('',(#9899,#9900,#9901,#9902,#9903));
#2945=EDGE_LOOP('',(#9904,#9905,#9906,#9907,#9908,#9909));
#2946=EDGE_LOOP('',(#9910,#9911,#9912,#9913,#9914));
#2947=EDGE_LOOP('',(#9915,#9916,#9917,#9918,#9919,#9920));
#2948=EDGE_LOOP('',(#9921,#9922,#9923,#9924));
#2949=EDGE_LOOP('',(#9925,#9926,#9927,#9928,#9929,#9930));
#2950=EDGE_LOOP('',(#9931,#9932,#9933,#9934));
#2951=EDGE_LOOP('',(#9935,#9936,#9937,#9938,#9939,#9940));
#2952=EDGE_LOOP('',(#9941,#9942,#9943,#9944));
#2953=EDGE_LOOP('',(#9945,#9946,#9947,#9948,#9949,#9950));
#2954=EDGE_LOOP('',(#9951,#9952,#9953,#9954));
#2955=EDGE_LOOP('',(#9955,#9956,#9957,#9958,#9959,#9960,#9961,#9962,#9963,
#9964,#9965,#9966,#9967,#9968,#9969,#9970,#9971,#9972,#9973,#9974,#9975,
#9976,#9977,#9978,#9979,#9980,#9981,#9982,#9983,#9984,#9985,#9986,#9987,
#9988,#9989,#9990,#9991,#9992,#9993,#9994,#9995,#9996,#9997,#9998));
#2956=EDGE_LOOP('',(#9999,#10000,#10001,#10002,#10003,#10004));
#2957=EDGE_LOOP('',(#10005,#10006,#10007,#10008));
#2958=EDGE_LOOP('',(#10009,#10010,#10011,#10012,#10013,#10014,#10015,#10016,
#10017,#10018,#10019,#10020,#10021,#10022,#10023,#10024,#10025,#10026,#10027,
#10028,#10029,#10030,#10031,#10032,#10033,#10034,#10035,#10036,#10037,#10038,
#10039,#10040,#10041,#10042,#10043,#10044,#10045,#10046,#10047,#10048,#10049,
#10050,#10051,#10052,#10053,#10054,#10055,#10056,#10057,#10058,#10059,#10060,
#10061,#10062,#10063));
#2959=EDGE_LOOP('',(#10064,#10065,#10066,#10067,#10068));
#2960=EDGE_LOOP('',(#10069,#10070,#10071,#10072,#10073,#10074,#10075,#10076,
#10077,#10078,#10079,#10080,#10081,#10082,#10083,#10084,#10085,#10086,#10087,
#10088,#10089,#10090,#10091,#10092,#10093,#10094,#10095,#10096,#10097,#10098,
#10099,#10100,#10101,#10102,#10103,#10104,#10105,#10106,#10107,#10108,#10109,
#10110,#10111,#10112,#10113,#10114,#10115,#10116,#10117,#10118,#10119,#10120,
#10121,#10122));
#2961=EDGE_LOOP('',(#10123,#10124,#10125,#10126,#10127,#10128,#10129));
#2962=EDGE_LOOP('',(#10130));
#2963=EDGE_LOOP('',(#10131));
#2964=EDGE_LOOP('',(#10132,#10133,#10134,#10135,#10136,#10137,#10138));
#2965=EDGE_LOOP('',(#10139));
#2966=EDGE_LOOP('',(#10140,#10141,#10142,#10143));
#2967=EDGE_LOOP('',(#10144,#10145,#10146,#10147));
#2968=EDGE_LOOP('',(#10148,#10149,#10150));
#2969=EDGE_LOOP('',(#10151,#10152,#10153,#10154,#10155,#10156,#10157,#10158,
#10159,#10160,#10161,#10162,#10163,#10164,#10165,#10166,#10167,#10168,#10169,
#10170,#10171,#10172,#10173,#10174,#10175,#10176,#10177,#10178,#10179,#10180,
#10181,#10182,#10183,#10184,#10185,#10186,#10187,#10188,#10189,#10190,#10191,
#10192,#10193,#10194,#10195,#10196,#10197,#10198,#10199,#10200,#10201,#10202,
#10203,#10204,#10205,#10206,#10207,#10208,#10209,#10210,#10211,#10212,#10213,
#10214,#10215,#10216,#10217,#10218,#10219,#10220,#10221,#10222,#10223,#10224,
#10225,#10226,#10227,#10228,#10229,#10230,#10231,#10232,#10233,#10234,#10235,
#10236,#10237,#10238,#10239,#10240,#10241,#10242,#10243,#10244,#10245,#10246,
#10247,#10248,#10249,#10250,#10251,#10252,#10253,#10254,#10255,#10256,#10257,
#10258,#10259,#10260,#10261));
#2970=EDGE_LOOP('',(#10262,#10263,#10264,#10265));
#2971=EDGE_LOOP('',(#10266,#10267,#10268,#10269));
#2972=EDGE_LOOP('',(#10270,#10271,#10272));
#2973=EDGE_LOOP('',(#10273,#10274,#10275,#10276));
#2974=EDGE_LOOP('',(#10277,#10278,#10279,#10280));
#2975=EDGE_LOOP('',(#10281,#10282,#10283));
#2976=EDGE_LOOP('',(#10284,#10285,#10286,#10287));
#2977=EDGE_LOOP('',(#10288,#10289,#10290,#10291));
#2978=EDGE_LOOP('',(#10292,#10293,#10294));
#2979=EDGE_LOOP('',(#10295,#10296,#10297,#10298));
#2980=EDGE_LOOP('',(#10299,#10300,#10301,#10302));
#2981=EDGE_LOOP('',(#10303,#10304,#10305));
#2982=EDGE_LOOP('',(#10306,#10307,#10308,#10309));
#2983=EDGE_LOOP('',(#10310,#10311,#10312,#10313));
#2984=EDGE_LOOP('',(#10314,#10315,#10316));
#2985=EDGE_LOOP('',(#10317,#10318,#10319,#10320));
#2986=EDGE_LOOP('',(#10321,#10322,#10323,#10324));
#2987=EDGE_LOOP('',(#10325,#10326,#10327));
#2988=EDGE_LOOP('',(#10328,#10329,#10330,#10331));
#2989=EDGE_LOOP('',(#10332,#10333,#10334,#10335));
#2990=EDGE_LOOP('',(#10336,#10337,#10338));
#2991=EDGE_LOOP('',(#10339,#10340,#10341,#10342));
#2992=EDGE_LOOP('',(#10343,#10344,#10345,#10346));
#2993=EDGE_LOOP('',(#10347,#10348,#10349));
#2994=EDGE_LOOP('',(#10350,#10351,#10352,#10353));
#2995=EDGE_LOOP('',(#10354,#10355,#10356,#10357));
#2996=EDGE_LOOP('',(#10358,#10359,#10360));
#2997=EDGE_LOOP('',(#10361,#10362,#10363,#10364));
#2998=EDGE_LOOP('',(#10365,#10366,#10367,#10368));
#2999=EDGE_LOOP('',(#10369,#10370,#10371));
#3000=EDGE_LOOP('',(#10372,#10373,#10374,#10375));
#3001=EDGE_LOOP('',(#10376,#10377,#10378,#10379));
#3002=EDGE_LOOP('',(#10380,#10381,#10382));
#3003=EDGE_LOOP('',(#10383,#10384,#10385,#10386));
#3004=EDGE_LOOP('',(#10387,#10388,#10389,#10390));
#3005=EDGE_LOOP('',(#10391,#10392,#10393));
#3006=EDGE_LOOP('',(#10394,#10395,#10396,#10397));
#3007=EDGE_LOOP('',(#10398,#10399,#10400,#10401));
#3008=EDGE_LOOP('',(#10402,#10403,#10404));
#3009=EDGE_LOOP('',(#10405,#10406,#10407,#10408));
#3010=EDGE_LOOP('',(#10409,#10410,#10411,#10412));
#3011=EDGE_LOOP('',(#10413,#10414,#10415));
#3012=EDGE_LOOP('',(#10416,#10417,#10418,#10419));
#3013=EDGE_LOOP('',(#10420,#10421,#10422,#10423));
#3014=EDGE_LOOP('',(#10424,#10425,#10426));
#3015=EDGE_LOOP('',(#10427,#10428,#10429,#10430));
#3016=EDGE_LOOP('',(#10431,#10432,#10433,#10434));
#3017=EDGE_LOOP('',(#10435,#10436,#10437));
#3018=EDGE_LOOP('',(#10438,#10439,#10440,#10441));
#3019=EDGE_LOOP('',(#10442,#10443,#10444,#10445));
#3020=EDGE_LOOP('',(#10446,#10447,#10448,#10449));
#3021=EDGE_LOOP('',(#10450,#10451,#10452,#10453));
#3022=EDGE_LOOP('',(#10454,#10455,#10456,#10457));
#3023=EDGE_LOOP('',(#10458,#10459,#10460));
#3024=EDGE_LOOP('',(#10461,#10462,#10463,#10464));
#3025=EDGE_LOOP('',(#10465,#10466,#10467,#10468));
#3026=EDGE_LOOP('',(#10469,#10470,#10471));
#3027=EDGE_LOOP('',(#10472,#10473,#10474,#10475));
#3028=EDGE_LOOP('',(#10476,#10477,#10478,#10479));
#3029=EDGE_LOOP('',(#10480,#10481,#10482));
#3030=EDGE_LOOP('',(#10483,#10484,#10485,#10486));
#3031=EDGE_LOOP('',(#10487,#10488,#10489,#10490));
#3032=EDGE_LOOP('',(#10491,#10492,#10493));
#3033=EDGE_LOOP('',(#10494,#10495,#10496,#10497));
#3034=EDGE_LOOP('',(#10498,#10499,#10500,#10501));
#3035=EDGE_LOOP('',(#10502,#10503,#10504));
#3036=EDGE_LOOP('',(#10505,#10506,#10507,#10508));
#3037=EDGE_LOOP('',(#10509,#10510,#10511,#10512));
#3038=EDGE_LOOP('',(#10513,#10514,#10515));
#3039=EDGE_LOOP('',(#10516,#10517,#10518,#10519));
#3040=EDGE_LOOP('',(#10520,#10521,#10522,#10523));
#3041=EDGE_LOOP('',(#10524,#10525,#10526));
#3042=EDGE_LOOP('',(#10527,#10528,#10529,#10530));
#3043=EDGE_LOOP('',(#10531,#10532,#10533,#10534));
#3044=EDGE_LOOP('',(#10535,#10536,#10537));
#3045=EDGE_LOOP('',(#10538,#10539,#10540,#10541));
#3046=EDGE_LOOP('',(#10542,#10543,#10544,#10545));
#3047=EDGE_LOOP('',(#10546,#10547,#10548));
#3048=EDGE_LOOP('',(#10549,#10550,#10551,#10552));
#3049=EDGE_LOOP('',(#10553,#10554,#10555,#10556));
#3050=EDGE_LOOP('',(#10557,#10558,#10559));
#3051=EDGE_LOOP('',(#10560,#10561,#10562,#10563));
#3052=EDGE_LOOP('',(#10564,#10565,#10566,#10567));
#3053=EDGE_LOOP('',(#10568,#10569,#10570));
#3054=EDGE_LOOP('',(#10571,#10572,#10573,#10574));
#3055=EDGE_LOOP('',(#10575,#10576,#10577,#10578));
#3056=EDGE_LOOP('',(#10579,#10580,#10581));
#3057=EDGE_LOOP('',(#10582,#10583,#10584,#10585));
#3058=EDGE_LOOP('',(#10586,#10587,#10588,#10589));
#3059=EDGE_LOOP('',(#10590,#10591,#10592));
#3060=EDGE_LOOP('',(#10593,#10594,#10595,#10596));
#3061=EDGE_LOOP('',(#10597,#10598,#10599,#10600));
#3062=EDGE_LOOP('',(#10601,#10602,#10603));
#3063=EDGE_LOOP('',(#10604,#10605,#10606,#10607));
#3064=EDGE_LOOP('',(#10608,#10609,#10610,#10611));
#3065=EDGE_LOOP('',(#10612,#10613,#10614));
#3066=EDGE_LOOP('',(#10615,#10616,#10617,#10618));
#3067=EDGE_LOOP('',(#10619,#10620,#10621,#10622));
#3068=EDGE_LOOP('',(#10623,#10624,#10625));
#3069=EDGE_LOOP('',(#10626,#10627,#10628,#10629));
#3070=EDGE_LOOP('',(#10630,#10631,#10632,#10633));
#3071=EDGE_LOOP('',(#10634,#10635,#10636));
#3072=EDGE_LOOP('',(#10637,#10638,#10639,#10640));
#3073=EDGE_LOOP('',(#10641,#10642,#10643,#10644));
#3074=EDGE_LOOP('',(#10645,#10646,#10647));
#3075=EDGE_LOOP('',(#10648,#10649,#10650,#10651,#10652,#10653,#10654,#10655,
#10656,#10657,#10658,#10659,#10660,#10661,#10662,#10663,#10664,#10665,#10666,
#10667,#10668,#10669,#10670,#10671,#10672,#10673,#10674,#10675,#10676,#10677,
#10678,#10679,#10680,#10681,#10682,#10683,#10684,#10685,#10686,#10687,#10688,
#10689,#10690,#10691,#10692,#10693,#10694,#10695,#10696,#10697,#10698,#10699,
#10700,#10701,#10702,#10703,#10704,#10705,#10706,#10707,#10708,#10709,#10710,
#10711,#10712,#10713,#10714,#10715,#10716,#10717,#10718,#10719,#10720,#10721,
#10722,#10723,#10724,#10725,#10726,#10727,#10728,#10729,#10730,#10731,#10732,
#10733,#10734,#10735,#10736,#10737,#10738,#10739,#10740,#10741,#10742,#10743,
#10744,#10745,#10746,#10747,#10748,#10749,#10750,#10751,#10752,#10753,#10754,
#10755,#10756,#10757,#10758,#10759,#10760,#10761,#10762,#10763,#10764,#10765,
#10766,#10767,#10768,#10769,#10770,#10771,#10772,#10773,#10774,#10775,#10776,
#10777,#10778,#10779,#10780,#10781,#10782,#10783,#10784,#10785,#10786,#10787,
#10788,#10789,#10790,#10791,#10792,#10793,#10794,#10795));
#3076=EDGE_LOOP('',(#10796));
#3077=EDGE_LOOP('',(#10797,#10798,#10799,#10800,#10801,#10802));
#3078=EDGE_LOOP('',(#10803,#10804));
#3079=EDGE_LOOP('',(#10805,#10806));
#3080=EDGE_LOOP('',(#10807,#10808));
#3081=EDGE_LOOP('',(#10809,#10810));
#3082=EDGE_LOOP('',(#10811,#10812));
#3083=EDGE_LOOP('',(#10813,#10814));
#3084=EDGE_LOOP('',(#10815,#10816,#10817,#10818,#10819,#10820,#10821,#10822));
#3085=EDGE_LOOP('',(#10823,#10824,#10825,#10826));
#3086=EDGE_LOOP('',(#10827,#10828,#10829,#10830));
#3087=EDGE_LOOP('',(#10831,#10832,#10833,#10834));
#3088=EDGE_LOOP('',(#10835,#10836,#10837,#10838));
#3089=EDGE_LOOP('',(#10839,#10840,#10841,#10842));
#3090=EDGE_LOOP('',(#10843,#10844,#10845,#10846));
#3562=CIRCLE('',#14116,1.92913);
#3563=CIRCLE('',#14136,2.36347);
#3564=CIRCLE('',#14137,2.36347);
#3565=CIRCLE('',#14138,2.36347);
#3566=CIRCLE('',#14140,1.92913);
#3567=CIRCLE('',#14142,2.36347);
#3568=CIRCLE('',#14144,2.36347);
#3569=CIRCLE('',#14145,2.36347);
#3570=CIRCLE('',#14147,2.56347);
#3571=CIRCLE('',#14148,0.2);
#3572=CIRCLE('',#14150,3.9624);
#3573=CIRCLE('',#14152,1.96347);
#3574=CIRCLE('',#14157,3.9624);
#3575=CIRCLE('',#14159,3.9624);
#3576=CIRCLE('',#14160,3.9624);
#3577=CIRCLE('',#14161,3.9624);
#3578=CIRCLE('',#14162,3.9624);
#3579=CIRCLE('',#14163,3.9624);
#3580=CIRCLE('',#14164,3.9624);
#3581=CIRCLE('',#14165,3.9624);
#3582=CIRCLE('',#14166,3.9624);
#3583=CIRCLE('',#14167,3.9624);
#3584=CIRCLE('',#14168,3.9624);
#3585=CIRCLE('',#14169,3.9624);
#3586=CIRCLE('',#14170,3.9624);
#3587=CIRCLE('',#14171,3.9624);
#3588=CIRCLE('',#14172,3.9624);
#3589=CIRCLE('',#14173,3.9624);
#3590=CIRCLE('',#14174,3.9624);
#3591=CIRCLE('',#14175,3.9624);
#3592=CIRCLE('',#14176,3.9624);
#3593=CIRCLE('',#14177,3.9624);
#3594=CIRCLE('',#14178,3.9624);
#3595=CIRCLE('',#14179,3.9624);
#3596=CIRCLE('',#14180,3.9624);
#3597=CIRCLE('',#14181,3.9624);
#3598=CIRCLE('',#14182,3.9624);
#3599=CIRCLE('',#14183,3.9624);
#3600=CIRCLE('',#14184,3.9624);
#3601=CIRCLE('',#14185,3.9624);
#3602=CIRCLE('',#14186,3.9624);
#3603=CIRCLE('',#14187,3.9624);
#3604=CIRCLE('',#14188,3.9624);
#3605=CIRCLE('',#14189,3.9624);
#3606=CIRCLE('',#14190,3.9624);
#3607=CIRCLE('',#14191,3.9624);
#3608=CIRCLE('',#14192,3.9624);
#3609=CIRCLE('',#14193,3.9624);
#3610=CIRCLE('',#14194,3.9624);
#3611=CIRCLE('',#14195,3.5624);
#3612=CIRCLE('',#14199,3.9624);
#3613=CIRCLE('',#14203,3.9624);
#3614=CIRCLE('',#14207,3.9624);
#3615=CIRCLE('',#14211,3.9624);
#3616=CIRCLE('',#14215,3.9624);
#3617=CIRCLE('',#14219,3.9624);
#3618=CIRCLE('',#14223,3.9624);
#3619=CIRCLE('',#14227,3.9624);
#3620=CIRCLE('',#14231,3.9624);
#3621=CIRCLE('',#14235,3.9624);
#3622=CIRCLE('',#14239,3.9624);
#3623=CIRCLE('',#14243,3.9624);
#3624=CIRCLE('',#14247,3.9624);
#3625=CIRCLE('',#14251,3.9624);
#3626=CIRCLE('',#14255,3.9624);
#3627=CIRCLE('',#14259,3.9624);
#3628=CIRCLE('',#14263,3.9624);
#3629=CIRCLE('',#14264,3.9624);
#3630=CIRCLE('',#14268,3.9624);
#3631=CIRCLE('',#14272,3.9624);
#3632=CIRCLE('',#14276,3.9624);
#3633=CIRCLE('',#14280,3.9624);
#3634=CIRCLE('',#14284,3.9624);
#3635=CIRCLE('',#14288,3.9624);
#3636=CIRCLE('',#14292,3.9624);
#3637=CIRCLE('',#14296,3.9624);
#3638=CIRCLE('',#14300,3.9624);
#3639=CIRCLE('',#14304,3.9624);
#3640=CIRCLE('',#14308,3.9624);
#3641=CIRCLE('',#14312,3.9624);
#3642=CIRCLE('',#14316,3.9624);
#3643=CIRCLE('',#14320,3.9624);
#3644=CIRCLE('',#14324,3.9624);
#3645=CIRCLE('',#14328,3.9624);
#3646=CIRCLE('',#14332,3.9624);
#3647=CIRCLE('',#14336,3.9624);
#3648=CIRCLE('',#14340,2.29135888084632);
#3649=CIRCLE('',#14342,2.29135888084632);
#3650=CIRCLE('',#14344,2.29135888084632);
#3651=CIRCLE('',#14346,2.29135888084632);
#3652=CIRCLE('',#14348,2.29135888084632);
#3653=CIRCLE('',#14350,2.29135888084632);
#4083=LINE('',#19895,#4994);
#4084=LINE('',#20117,#4995);
#4085=LINE('',#20543,#4996);
#4086=LINE('',#20965,#4997);
#4087=LINE('',#21427,#4998);
#4088=LINE('',#21847,#4999);
#4089=LINE('',#22311,#5000);
#4090=LINE('',#22733,#5001);
#4091=LINE('',#23232,#5002);
#4092=LINE('',#23492,#5003);
#4093=LINE('',#23796,#5004);
#4094=LINE('',#24185,#5005);
#4095=LINE('',#24610,#5006);
#4096=LINE('',#25046,#5007);
#4097=LINE('',#25484,#5008);
#4098=LINE('',#25912,#5009);
#4099=LINE('',#26354,#5010);
#4100=LINE('',#26786,#5011);
#4101=LINE('',#27252,#5012);
#4102=LINE('',#36519,#5013);
#4103=LINE('',#36525,#5014);
#4104=LINE('',#36527,#5015);
#4105=LINE('',#36529,#5016);
#4106=LINE('',#36536,#5017);
#4107=LINE('',#36540,#5018);
#4108=LINE('',#36896,#5019);
#4109=LINE('',#36900,#5020);
#4110=LINE('',#36902,#5021);
#4111=LINE('',#36903,#5022);
#4112=LINE('',#36906,#5023);
#4113=LINE('',#36907,#5024);
#4114=LINE('',#36912,#5025);
#4115=LINE('',#36914,#5026);
#4116=LINE('',#36915,#5027);
#4117=LINE('',#36918,#5028);
#4118=LINE('',#36919,#5029);
#4119=LINE('',#36924,#5030);
#4120=LINE('',#36926,#5031);
#4121=LINE('',#36927,#5032);
#4122=LINE('',#36930,#5033);
#4123=LINE('',#36931,#5034);
#4124=LINE('',#36936,#5035);
#4125=LINE('',#36938,#5036);
#4126=LINE('',#36939,#5037);
#4127=LINE('',#36942,#5038);
#4128=LINE('',#36943,#5039);
#4129=LINE('',#36948,#5040);
#4130=LINE('',#36950,#5041);
#4131=LINE('',#36951,#5042);
#4132=LINE('',#36954,#5043);
#4133=LINE('',#36955,#5044);
#4134=LINE('',#36960,#5045);
#4135=LINE('',#36962,#5046);
#4136=LINE('',#36963,#5047);
#4137=LINE('',#36966,#5048);
#4138=LINE('',#36967,#5049);
#4139=LINE('',#36972,#5050);
#4140=LINE('',#36974,#5051);
#4141=LINE('',#36975,#5052);
#4142=LINE('',#36978,#5053);
#4143=LINE('',#36979,#5054);
#4144=LINE('',#36984,#5055);
#4145=LINE('',#36986,#5056);
#4146=LINE('',#36987,#5057);
#4147=LINE('',#36990,#5058);
#4148=LINE('',#36991,#5059);
#4149=LINE('',#36996,#5060);
#4150=LINE('',#36998,#5061);
#4151=LINE('',#36999,#5062);
#4152=LINE('',#37002,#5063);
#4153=LINE('',#37003,#5064);
#4154=LINE('',#37008,#5065);
#4155=LINE('',#37010,#5066);
#4156=LINE('',#37011,#5067);
#4157=LINE('',#37014,#5068);
#4158=LINE('',#37015,#5069);
#4159=LINE('',#37020,#5070);
#4160=LINE('',#37022,#5071);
#4161=LINE('',#37023,#5072);
#4162=LINE('',#37026,#5073);
#4163=LINE('',#37027,#5074);
#4164=LINE('',#37032,#5075);
#4165=LINE('',#37034,#5076);
#4166=LINE('',#37035,#5077);
#4167=LINE('',#37038,#5078);
#4168=LINE('',#37039,#5079);
#4169=LINE('',#37044,#5080);
#4170=LINE('',#37046,#5081);
#4171=LINE('',#37047,#5082);
#4172=LINE('',#37050,#5083);
#4173=LINE('',#37051,#5084);
#4174=LINE('',#37056,#5085);
#4175=LINE('',#37058,#5086);
#4176=LINE('',#37059,#5087);
#4177=LINE('',#37062,#5088);
#4178=LINE('',#37063,#5089);
#4179=LINE('',#37068,#5090);
#4180=LINE('',#37070,#5091);
#4181=LINE('',#37071,#5092);
#4182=LINE('',#37074,#5093);
#4183=LINE('',#37075,#5094);
#4184=LINE('',#37080,#5095);
#4185=LINE('',#37082,#5096);
#4186=LINE('',#37083,#5097);
#4187=LINE('',#37086,#5098);
#4188=LINE('',#37087,#5099);
#4189=LINE('',#37092,#5100);
#4190=LINE('',#37094,#5101);
#4191=LINE('',#37095,#5102);
#4192=LINE('',#37098,#5103);
#4193=LINE('',#37099,#5104);
#4194=LINE('',#37106,#5105);
#4195=LINE('',#37108,#5106);
#4196=LINE('',#37109,#5107);
#4197=LINE('',#37112,#5108);
#4198=LINE('',#37113,#5109);
#4199=LINE('',#37118,#5110);
#4200=LINE('',#37120,#5111);
#4201=LINE('',#37121,#5112);
#4202=LINE('',#37124,#5113);
#4203=LINE('',#37125,#5114);
#4204=LINE('',#37130,#5115);
#4205=LINE('',#37132,#5116);
#4206=LINE('',#37133,#5117);
#4207=LINE('',#37136,#5118);
#4208=LINE('',#37137,#5119);
#4209=LINE('',#37142,#5120);
#4210=LINE('',#37144,#5121);
#4211=LINE('',#37145,#5122);
#4212=LINE('',#37148,#5123);
#4213=LINE('',#37149,#5124);
#4214=LINE('',#37154,#5125);
#4215=LINE('',#37156,#5126);
#4216=LINE('',#37157,#5127);
#4217=LINE('',#37160,#5128);
#4218=LINE('',#37161,#5129);
#4219=LINE('',#37166,#5130);
#4220=LINE('',#37168,#5131);
#4221=LINE('',#37169,#5132);
#4222=LINE('',#37172,#5133);
#4223=LINE('',#37173,#5134);
#4224=LINE('',#37178,#5135);
#4225=LINE('',#37180,#5136);
#4226=LINE('',#37181,#5137);
#4227=LINE('',#37184,#5138);
#4228=LINE('',#37185,#5139);
#4229=LINE('',#37190,#5140);
#4230=LINE('',#37192,#5141);
#4231=LINE('',#37193,#5142);
#4232=LINE('',#37196,#5143);
#4233=LINE('',#37197,#5144);
#4234=LINE('',#37202,#5145);
#4235=LINE('',#37204,#5146);
#4236=LINE('',#37205,#5147);
#4237=LINE('',#37208,#5148);
#4238=LINE('',#37209,#5149);
#4239=LINE('',#37214,#5150);
#4240=LINE('',#37216,#5151);
#4241=LINE('',#37217,#5152);
#4242=LINE('',#37220,#5153);
#4243=LINE('',#37221,#5154);
#4244=LINE('',#37226,#5155);
#4245=LINE('',#37228,#5156);
#4246=LINE('',#37229,#5157);
#4247=LINE('',#37232,#5158);
#4248=LINE('',#37233,#5159);
#4249=LINE('',#37238,#5160);
#4250=LINE('',#37240,#5161);
#4251=LINE('',#37241,#5162);
#4252=LINE('',#37244,#5163);
#4253=LINE('',#37245,#5164);
#4254=LINE('',#37250,#5165);
#4255=LINE('',#37252,#5166);
#4256=LINE('',#37253,#5167);
#4257=LINE('',#37256,#5168);
#4258=LINE('',#37257,#5169);
#4259=LINE('',#37262,#5170);
#4260=LINE('',#37264,#5171);
#4261=LINE('',#37265,#5172);
#4262=LINE('',#37268,#5173);
#4263=LINE('',#37269,#5174);
#4264=LINE('',#37274,#5175);
#4265=LINE('',#37276,#5176);
#4266=LINE('',#37277,#5177);
#4267=LINE('',#37280,#5178);
#4268=LINE('',#37281,#5179);
#4269=LINE('',#37286,#5180);
#4270=LINE('',#37288,#5181);
#4271=LINE('',#37289,#5182);
#4272=LINE('',#37292,#5183);
#4273=LINE('',#37293,#5184);
#4274=LINE('',#37298,#5185);
#4275=LINE('',#37300,#5186);
#4276=LINE('',#37301,#5187);
#4277=LINE('',#37304,#5188);
#4278=LINE('',#37305,#5189);
#4279=LINE('',#37310,#5190);
#4280=LINE('',#37312,#5191);
#4281=LINE('',#37313,#5192);
#4282=LINE('',#37316,#5193);
#4283=LINE('',#37317,#5194);
#4284=LINE('',#37321,#5195);
#4285=LINE('',#37325,#5196);
#4286=LINE('',#37327,#5197);
#4287=LINE('',#37329,#5198);
#4288=LINE('',#37331,#5199);
#4289=LINE('',#37333,#5200);
#4290=LINE('',#37334,#5201);
#4291=LINE('',#37338,#5202);
#4292=LINE('',#37342,#5203);
#4293=LINE('',#37346,#5204);
#4294=LINE('',#37350,#5205);
#4295=LINE('',#37354,#5206);
#4296=LINE('',#37357,#5207);
#4297=LINE('',#37361,#5208);
#4298=LINE('',#37363,#5209);
#4299=LINE('',#37364,#5210);
#4300=LINE('',#37366,#5211);
#4301=LINE('',#37368,#5212);
#4302=LINE('',#37370,#5213);
#4303=LINE('',#37372,#5214);
#4994=VECTOR('',#16008,1.92913);
#4995=VECTOR('',#16013,1.92913);
#4996=VECTOR('',#16016,1.92913);
#4997=VECTOR('',#16019,1.92913);
#4998=VECTOR('',#16022,1.92913);
#4999=VECTOR('',#16025,1.92913);
#5000=VECTOR('',#16028,1.92913);
#5001=VECTOR('',#16031,1.92913);
#5002=VECTOR('',#16034,1.92913);
#5003=VECTOR('',#16037,1.92913);
#5004=VECTOR('',#16040,1.92913);
#5005=VECTOR('',#16043,1.92913);
#5006=VECTOR('',#16046,1.92913);
#5007=VECTOR('',#16049,1.92913);
#5008=VECTOR('',#16052,1.92913);
#5009=VECTOR('',#16055,1.92913);
#5010=VECTOR('',#16058,1.92913);
#5011=VECTOR('',#16061,1.92913);
#5012=VECTOR('',#16064,1.92913);
#5013=VECTOR('',#16099,2.16347);
#5014=VECTOR('',#16106,10.);
#5015=VECTOR('',#16107,10.);
#5016=VECTOR('',#16108,10.);
#5017=VECTOR('',#16111,10.);
#5018=VECTOR('',#16112,10.);
#5019=VECTOR('',#16191,3.7624);
#5020=VECTOR('',#16196,10.);
#5021=VECTOR('',#16197,10.);
#5022=VECTOR('',#16198,10.);
#5023=VECTOR('',#16201,10.);
#5024=VECTOR('',#16202,10.);
#5025=VECTOR('',#16209,10.);
#5026=VECTOR('',#16210,10.);
#5027=VECTOR('',#16211,10.);
#5028=VECTOR('',#16214,10.);
#5029=VECTOR('',#16215,10.);
#5030=VECTOR('',#16222,10.);
#5031=VECTOR('',#16223,10.);
#5032=VECTOR('',#16224,10.);
#5033=VECTOR('',#16227,10.);
#5034=VECTOR('',#16228,10.);
#5035=VECTOR('',#16235,10.);
#5036=VECTOR('',#16236,10.);
#5037=VECTOR('',#16237,10.);
#5038=VECTOR('',#16240,10.);
#5039=VECTOR('',#16241,10.);
#5040=VECTOR('',#16248,10.);
#5041=VECTOR('',#16249,10.);
#5042=VECTOR('',#16250,10.);
#5043=VECTOR('',#16253,10.);
#5044=VECTOR('',#16254,10.);
#5045=VECTOR('',#16261,10.);
#5046=VECTOR('',#16262,10.);
#5047=VECTOR('',#16263,10.);
#5048=VECTOR('',#16266,10.);
#5049=VECTOR('',#16267,10.);
#5050=VECTOR('',#16274,10.);
#5051=VECTOR('',#16275,10.);
#5052=VECTOR('',#16276,10.);
#5053=VECTOR('',#16279,10.);
#5054=VECTOR('',#16280,10.);
#5055=VECTOR('',#16287,10.);
#5056=VECTOR('',#16288,10.);
#5057=VECTOR('',#16289,10.);
#5058=VECTOR('',#16292,10.);
#5059=VECTOR('',#16293,10.);
#5060=VECTOR('',#16300,10.);
#5061=VECTOR('',#16301,10.);
#5062=VECTOR('',#16302,10.);
#5063=VECTOR('',#16305,10.);
#5064=VECTOR('',#16306,10.);
#5065=VECTOR('',#16313,10.);
#5066=VECTOR('',#16314,10.);
#5067=VECTOR('',#16315,10.);
#5068=VECTOR('',#16318,10.);
#5069=VECTOR('',#16319,10.);
#5070=VECTOR('',#16326,10.);
#5071=VECTOR('',#16327,10.);
#5072=VECTOR('',#16328,10.);
#5073=VECTOR('',#16331,10.);
#5074=VECTOR('',#16332,10.);
#5075=VECTOR('',#16339,10.);
#5076=VECTOR('',#16340,10.);
#5077=VECTOR('',#16341,10.);
#5078=VECTOR('',#16344,10.);
#5079=VECTOR('',#16345,10.);
#5080=VECTOR('',#16352,10.);
#5081=VECTOR('',#16353,10.);
#5082=VECTOR('',#16354,10.);
#5083=VECTOR('',#16357,10.);
#5084=VECTOR('',#16358,10.);
#5085=VECTOR('',#16365,10.);
#5086=VECTOR('',#16366,10.);
#5087=VECTOR('',#16367,10.);
#5088=VECTOR('',#16370,10.);
#5089=VECTOR('',#16371,10.);
#5090=VECTOR('',#16378,10.);
#5091=VECTOR('',#16379,10.);
#5092=VECTOR('',#16380,10.);
#5093=VECTOR('',#16383,10.);
#5094=VECTOR('',#16384,10.);
#5095=VECTOR('',#16391,10.);
#5096=VECTOR('',#16392,10.);
#5097=VECTOR('',#16393,10.);
#5098=VECTOR('',#16396,10.);
#5099=VECTOR('',#16397,10.);
#5100=VECTOR('',#16404,10.);
#5101=VECTOR('',#16405,10.);
#5102=VECTOR('',#16406,10.);
#5103=VECTOR('',#16409,10.);
#5104=VECTOR('',#16410,10.);
#5105=VECTOR('',#16419,10.);
#5106=VECTOR('',#16420,10.);
#5107=VECTOR('',#16421,10.);
#5108=VECTOR('',#16424,10.);
#5109=VECTOR('',#16425,10.);
#5110=VECTOR('',#16432,10.);
#5111=VECTOR('',#16433,10.);
#5112=VECTOR('',#16434,10.);
#5113=VECTOR('',#16437,10.);
#5114=VECTOR('',#16438,10.);
#5115=VECTOR('',#16445,10.);
#5116=VECTOR('',#16446,10.);
#5117=VECTOR('',#16447,10.);
#5118=VECTOR('',#16450,10.);
#5119=VECTOR('',#16451,10.);
#5120=VECTOR('',#16458,10.);
#5121=VECTOR('',#16459,10.);
#5122=VECTOR('',#16460,10.);
#5123=VECTOR('',#16463,10.);
#5124=VECTOR('',#16464,10.);
#5125=VECTOR('',#16471,10.);
#5126=VECTOR('',#16472,10.);
#5127=VECTOR('',#16473,10.);
#5128=VECTOR('',#16476,10.);
#5129=VECTOR('',#16477,10.);
#5130=VECTOR('',#16484,10.);
#5131=VECTOR('',#16485,10.);
#5132=VECTOR('',#16486,10.);
#5133=VECTOR('',#16489,10.);
#5134=VECTOR('',#16490,10.);
#5135=VECTOR('',#16497,10.);
#5136=VECTOR('',#16498,10.);
#5137=VECTOR('',#16499,10.);
#5138=VECTOR('',#16502,10.);
#5139=VECTOR('',#16503,10.);
#5140=VECTOR('',#16510,10.);
#5141=VECTOR('',#16511,10.);
#5142=VECTOR('',#16512,10.);
#5143=VECTOR('',#16515,10.);
#5144=VECTOR('',#16516,10.);
#5145=VECTOR('',#16523,10.);
#5146=VECTOR('',#16524,10.);
#5147=VECTOR('',#16525,10.);
#5148=VECTOR('',#16528,10.);
#5149=VECTOR('',#16529,10.);
#5150=VECTOR('',#16536,10.);
#5151=VECTOR('',#16537,10.);
#5152=VECTOR('',#16538,10.);
#5153=VECTOR('',#16541,10.);
#5154=VECTOR('',#16542,10.);
#5155=VECTOR('',#16549,10.);
#5156=VECTOR('',#16550,10.);
#5157=VECTOR('',#16551,10.);
#5158=VECTOR('',#16554,10.);
#5159=VECTOR('',#16555,10.);
#5160=VECTOR('',#16562,10.);
#5161=VECTOR('',#16563,10.);
#5162=VECTOR('',#16564,10.);
#5163=VECTOR('',#16567,10.);
#5164=VECTOR('',#16568,10.);
#5165=VECTOR('',#16575,10.);
#5166=VECTOR('',#16576,10.);
#5167=VECTOR('',#16577,10.);
#5168=VECTOR('',#16580,10.);
#5169=VECTOR('',#16581,10.);
#5170=VECTOR('',#16588,10.);
#5171=VECTOR('',#16589,10.);
#5172=VECTOR('',#16590,10.);
#5173=VECTOR('',#16593,10.);
#5174=VECTOR('',#16594,10.);
#5175=VECTOR('',#16601,10.);
#5176=VECTOR('',#16602,10.);
#5177=VECTOR('',#16603,10.);
#5178=VECTOR('',#16606,10.);
#5179=VECTOR('',#16607,10.);
#5180=VECTOR('',#16614,10.);
#5181=VECTOR('',#16615,10.);
#5182=VECTOR('',#16616,10.);
#5183=VECTOR('',#16619,10.);
#5184=VECTOR('',#16620,10.);
#5185=VECTOR('',#16627,10.);
#5186=VECTOR('',#16628,10.);
#5187=VECTOR('',#16629,10.);
#5188=VECTOR('',#16632,10.);
#5189=VECTOR('',#16633,10.);
#5190=VECTOR('',#16640,10.);
#5191=VECTOR('',#16641,10.);
#5192=VECTOR('',#16642,10.);
#5193=VECTOR('',#16645,10.);
#5194=VECTOR('',#16646,10.);
#5195=VECTOR('',#16653,3.9624);
#5196=VECTOR('',#16656,10.);
#5197=VECTOR('',#16657,10.);
#5198=VECTOR('',#16658,10.);
#5199=VECTOR('',#16659,10.);
#5200=VECTOR('',#16660,10.);
#5201=VECTOR('',#16661,10.);
#5202=VECTOR('',#16664,10.);
#5203=VECTOR('',#16669,10.);
#5204=VECTOR('',#16674,10.);
#5205=VECTOR('',#16679,10.);
#5206=VECTOR('',#16684,10.);
#5207=VECTOR('',#16689,10.);
#5208=VECTOR('',#16694,2.29135888084632);
#5209=VECTOR('',#16697,10.);
#5210=VECTOR('',#16698,10.);
#5211=VECTOR('',#16701,10.);
#5212=VECTOR('',#16704,10.);
#5213=VECTOR('',#16707,10.);
#5214=VECTOR('',#16710,10.);
#5966=VERTEX_POINT('',#19893);
#5967=VERTEX_POINT('',#19894);
#5968=VERTEX_POINT('',#19896);
#5969=VERTEX_POINT('',#20027);
#5970=VERTEX_POINT('',#20115);
#5971=VERTEX_POINT('',#20116);
#5972=VERTEX_POINT('',#20118);
#5973=VERTEX_POINT('',#20333);
#5974=VERTEX_POINT('',#20541);
#5975=VERTEX_POINT('',#20542);
#5976=VERTEX_POINT('',#20963);
#5977=VERTEX_POINT('',#20964);
#5978=VERTEX_POINT('',#20966);
#5979=VERTEX_POINT('',#21183);
#5980=VERTEX_POINT('',#21425);
#5981=VERTEX_POINT('',#21426);
#5982=VERTEX_POINT('',#21845);
#5983=VERTEX_POINT('',#21846);
#5984=VERTEX_POINT('',#21848);
#5985=VERTEX_POINT('',#22087);
#5986=VERTEX_POINT('',#22309);
#5987=VERTEX_POINT('',#22310);
#5988=VERTEX_POINT('',#22731);
#5989=VERTEX_POINT('',#22732);
#5990=VERTEX_POINT('',#22734);
#5991=VERTEX_POINT('',#23033);
#5992=VERTEX_POINT('',#23230);
#5993=VERTEX_POINT('',#23231);
#5994=VERTEX_POINT('',#23439);
#5995=VERTEX_POINT('',#23490);
#5996=VERTEX_POINT('',#23491);
#5997=VERTEX_POINT('',#23493);
#5998=VERTEX_POINT('',#23611);
#5999=VERTEX_POINT('',#23794);
#6000=VERTEX_POINT('',#23795);
#6001=VERTEX_POINT('',#23797);
#6002=VERTEX_POINT('',#24183);
#6003=VERTEX_POINT('',#24184);
#6004=VERTEX_POINT('',#24186);
#6005=VERTEX_POINT('',#24398);
#6006=VERTEX_POINT('',#24608);
#6007=VERTEX_POINT('',#24609);
#6008=VERTEX_POINT('',#25044);
#6009=VERTEX_POINT('',#25045);
#6010=VERTEX_POINT('',#25047);
#6011=VERTEX_POINT('',#25264);
#6012=VERTEX_POINT('',#25482);
#6013=VERTEX_POINT('',#25483);
#6014=VERTEX_POINT('',#25910);
#6015=VERTEX_POINT('',#25911);
#6016=VERTEX_POINT('',#25913);
#6017=VERTEX_POINT('',#26130);
#6018=VERTEX_POINT('',#26352);
#6019=VERTEX_POINT('',#26353);
#6020=VERTEX_POINT('',#26784);
#6021=VERTEX_POINT('',#26785);
#6022=VERTEX_POINT('',#26787);
#6023=VERTEX_POINT('',#27008);
#6024=VERTEX_POINT('',#27250);
#6025=VERTEX_POINT('',#27251);
#6026=VERTEX_POINT('',#27668);
#6027=VERTEX_POINT('',#27669);
#6028=VERTEX_POINT('',#27737);
#6029=VERTEX_POINT('',#27739);
#6030=VERTEX_POINT('',#27745);
#6031=VERTEX_POINT('',#27939);
#6032=VERTEX_POINT('',#28130);
#6033=VERTEX_POINT('',#28321);
#6034=VERTEX_POINT('',#28512);
#6035=VERTEX_POINT('',#28703);
#6036=VERTEX_POINT('',#28897);
#6037=VERTEX_POINT('',#29088);
#6038=VERTEX_POINT('',#29279);
#6039=VERTEX_POINT('',#29470);
#6040=VERTEX_POINT('',#29661);
#6041=VERTEX_POINT('',#29852);
#6042=VERTEX_POINT('',#30046);
#6043=VERTEX_POINT('',#30237);
#6044=VERTEX_POINT('',#30425);
#6045=VERTEX_POINT('',#30616);
#6046=VERTEX_POINT('',#30807);
#6047=VERTEX_POINT('',#30998);
#6048=VERTEX_POINT('',#31192);
#6049=VERTEX_POINT('',#31386);
#6050=VERTEX_POINT('',#31403);
#6051=VERTEX_POINT('',#31405);
#6052=VERTEX_POINT('',#31407);
#6053=VERTEX_POINT('',#31417);
#6054=VERTEX_POINT('',#31608);
#6055=VERTEX_POINT('',#31799);
#6056=VERTEX_POINT('',#31993);
#6057=VERTEX_POINT('',#32187);
#6058=VERTEX_POINT('',#32378);
#6059=VERTEX_POINT('',#32569);
#6060=VERTEX_POINT('',#32760);
#6061=VERTEX_POINT('',#32951);
#6062=VERTEX_POINT('',#33145);
#6063=VERTEX_POINT('',#33339);
#6064=VERTEX_POINT('',#33530);
#6065=VERTEX_POINT('',#33721);
#6066=VERTEX_POINT('',#33912);
#6067=VERTEX_POINT('',#34106);
#6068=VERTEX_POINT('',#34297);
#6069=VERTEX_POINT('',#34488);
#6070=VERTEX_POINT('',#34870);
#6071=VERTEX_POINT('',#34921);
#6072=VERTEX_POINT('',#35040);
#6073=VERTEX_POINT('',#35042);
#6074=VERTEX_POINT('',#35171);
#6075=VERTEX_POINT('',#35919);
#6076=VERTEX_POINT('',#35920);
#6077=VERTEX_POINT('',#36511);
#6078=VERTEX_POINT('',#36515);
#6079=VERTEX_POINT('',#36518);
#6080=VERTEX_POINT('',#36523);
#6081=VERTEX_POINT('',#36524);
#6082=VERTEX_POINT('',#36526);
#6083=VERTEX_POINT('',#36528);
#6084=VERTEX_POINT('',#36534);
#6085=VERTEX_POINT('',#36535);
#6086=VERTEX_POINT('',#36544);
#6087=VERTEX_POINT('',#36545);
#6088=VERTEX_POINT('',#36549);
#6089=VERTEX_POINT('',#36551);
#6090=VERTEX_POINT('',#36555);
#6091=VERTEX_POINT('',#36559);
#6092=VERTEX_POINT('',#36561);
#6093=VERTEX_POINT('',#36565);
#6094=VERTEX_POINT('',#36569);
#6095=VERTEX_POINT('',#36571);
#6096=VERTEX_POINT('',#36575);
#6097=VERTEX_POINT('',#36579);
#6098=VERTEX_POINT('',#36581);
#6099=VERTEX_POINT('',#36585);
#6100=VERTEX_POINT('',#36589);
#6101=VERTEX_POINT('',#36591);
#6102=VERTEX_POINT('',#36595);
#6103=VERTEX_POINT('',#36599);
#6104=VERTEX_POINT('',#36601);
#6105=VERTEX_POINT('',#36605);
#6106=VERTEX_POINT('',#36609);
#6107=VERTEX_POINT('',#36611);
#6108=VERTEX_POINT('',#36615);
#6109=VERTEX_POINT('',#36619);
#6110=VERTEX_POINT('',#36621);
#6111=VERTEX_POINT('',#36625);
#6112=VERTEX_POINT('',#36629);
#6113=VERTEX_POINT('',#36631);
#6114=VERTEX_POINT('',#36635);
#6115=VERTEX_POINT('',#36639);
#6116=VERTEX_POINT('',#36641);
#6117=VERTEX_POINT('',#36645);
#6118=VERTEX_POINT('',#36649);
#6119=VERTEX_POINT('',#36651);
#6120=VERTEX_POINT('',#36655);
#6121=VERTEX_POINT('',#36659);
#6122=VERTEX_POINT('',#36661);
#6123=VERTEX_POINT('',#36665);
#6124=VERTEX_POINT('',#36669);
#6125=VERTEX_POINT('',#36671);
#6126=VERTEX_POINT('',#36675);
#6127=VERTEX_POINT('',#36679);
#6128=VERTEX_POINT('',#36681);
#6129=VERTEX_POINT('',#36685);
#6130=VERTEX_POINT('',#36689);
#6131=VERTEX_POINT('',#36691);
#6132=VERTEX_POINT('',#36695);
#6133=VERTEX_POINT('',#36699);
#6134=VERTEX_POINT('',#36701);
#6135=VERTEX_POINT('',#36705);
#6136=VERTEX_POINT('',#36709);
#6137=VERTEX_POINT('',#36711);
#6138=VERTEX_POINT('',#36715);
#6139=VERTEX_POINT('',#36719);
#6140=VERTEX_POINT('',#36721);
#6141=VERTEX_POINT('',#36725);
#6142=VERTEX_POINT('',#36730);
#6143=VERTEX_POINT('',#36732);
#6144=VERTEX_POINT('',#36736);
#6145=VERTEX_POINT('',#36740);
#6146=VERTEX_POINT('',#36742);
#6147=VERTEX_POINT('',#36746);
#6148=VERTEX_POINT('',#36750);
#6149=VERTEX_POINT('',#36752);
#6150=VERTEX_POINT('',#36756);
#6151=VERTEX_POINT('',#36760);
#6152=VERTEX_POINT('',#36762);
#6153=VERTEX_POINT('',#36766);
#6154=VERTEX_POINT('',#36770);
#6155=VERTEX_POINT('',#36772);
#6156=VERTEX_POINT('',#36776);
#6157=VERTEX_POINT('',#36780);
#6158=VERTEX_POINT('',#36782);
#6159=VERTEX_POINT('',#36786);
#6160=VERTEX_POINT('',#36790);
#6161=VERTEX_POINT('',#36792);
#6162=VERTEX_POINT('',#36796);
#6163=VERTEX_POINT('',#36800);
#6164=VERTEX_POINT('',#36802);
#6165=VERTEX_POINT('',#36806);
#6166=VERTEX_POINT('',#36810);
#6167=VERTEX_POINT('',#36812);
#6168=VERTEX_POINT('',#36816);
#6169=VERTEX_POINT('',#36820);
#6170=VERTEX_POINT('',#36822);
#6171=VERTEX_POINT('',#36826);
#6172=VERTEX_POINT('',#36830);
#6173=VERTEX_POINT('',#36832);
#6174=VERTEX_POINT('',#36836);
#6175=VERTEX_POINT('',#36840);
#6176=VERTEX_POINT('',#36842);
#6177=VERTEX_POINT('',#36846);
#6178=VERTEX_POINT('',#36850);
#6179=VERTEX_POINT('',#36852);
#6180=VERTEX_POINT('',#36856);
#6181=VERTEX_POINT('',#36860);
#6182=VERTEX_POINT('',#36862);
#6183=VERTEX_POINT('',#36866);
#6184=VERTEX_POINT('',#36870);
#6185=VERTEX_POINT('',#36872);
#6186=VERTEX_POINT('',#36876);
#6187=VERTEX_POINT('',#36880);
#6188=VERTEX_POINT('',#36882);
#6189=VERTEX_POINT('',#36886);
#6190=VERTEX_POINT('',#36890);
#6191=VERTEX_POINT('',#36895);
#6192=VERTEX_POINT('',#36899);
#6193=VERTEX_POINT('',#36901);
#6194=VERTEX_POINT('',#36905);
#6195=VERTEX_POINT('',#36911);
#6196=VERTEX_POINT('',#36913);
#6197=VERTEX_POINT('',#36917);
#6198=VERTEX_POINT('',#36923);
#6199=VERTEX_POINT('',#36925);
#6200=VERTEX_POINT('',#36929);
#6201=VERTEX_POINT('',#36935);
#6202=VERTEX_POINT('',#36937);
#6203=VERTEX_POINT('',#36941);
#6204=VERTEX_POINT('',#36947);
#6205=VERTEX_POINT('',#36949);
#6206=VERTEX_POINT('',#36953);
#6207=VERTEX_POINT('',#36959);
#6208=VERTEX_POINT('',#36961);
#6209=VERTEX_POINT('',#36965);
#6210=VERTEX_POINT('',#36971);
#6211=VERTEX_POINT('',#36973);
#6212=VERTEX_POINT('',#36977);
#6213=VERTEX_POINT('',#36983);
#6214=VERTEX_POINT('',#36985);
#6215=VERTEX_POINT('',#36989);
#6216=VERTEX_POINT('',#36995);
#6217=VERTEX_POINT('',#36997);
#6218=VERTEX_POINT('',#37001);
#6219=VERTEX_POINT('',#37007);
#6220=VERTEX_POINT('',#37009);
#6221=VERTEX_POINT('',#37013);
#6222=VERTEX_POINT('',#37019);
#6223=VERTEX_POINT('',#37021);
#6224=VERTEX_POINT('',#37025);
#6225=VERTEX_POINT('',#37031);
#6226=VERTEX_POINT('',#37033);
#6227=VERTEX_POINT('',#37037);
#6228=VERTEX_POINT('',#37043);
#6229=VERTEX_POINT('',#37045);
#6230=VERTEX_POINT('',#37049);
#6231=VERTEX_POINT('',#37055);
#6232=VERTEX_POINT('',#37057);
#6233=VERTEX_POINT('',#37061);
#6234=VERTEX_POINT('',#37067);
#6235=VERTEX_POINT('',#37069);
#6236=VERTEX_POINT('',#37073);
#6237=VERTEX_POINT('',#37079);
#6238=VERTEX_POINT('',#37081);
#6239=VERTEX_POINT('',#37085);
#6240=VERTEX_POINT('',#37091);
#6241=VERTEX_POINT('',#37093);
#6242=VERTEX_POINT('',#37097);
#6243=VERTEX_POINT('',#37101);
#6244=VERTEX_POINT('',#37105);
#6245=VERTEX_POINT('',#37107);
#6246=VERTEX_POINT('',#37111);
#6247=VERTEX_POINT('',#37117);
#6248=VERTEX_POINT('',#37119);
#6249=VERTEX_POINT('',#37123);
#6250=VERTEX_POINT('',#37129);
#6251=VERTEX_POINT('',#37131);
#6252=VERTEX_POINT('',#37135);
#6253=VERTEX_POINT('',#37141);
#6254=VERTEX_POINT('',#37143);
#6255=VERTEX_POINT('',#37147);
#6256=VERTEX_POINT('',#37153);
#6257=VERTEX_POINT('',#37155);
#6258=VERTEX_POINT('',#37159);
#6259=VERTEX_POINT('',#37165);
#6260=VERTEX_POINT('',#37167);
#6261=VERTEX_POINT('',#37171);
#6262=VERTEX_POINT('',#37177);
#6263=VERTEX_POINT('',#37179);
#6264=VERTEX_POINT('',#37183);
#6265=VERTEX_POINT('',#37189);
#6266=VERTEX_POINT('',#37191);
#6267=VERTEX_POINT('',#37195);
#6268=VERTEX_POINT('',#37201);
#6269=VERTEX_POINT('',#37203);
#6270=VERTEX_POINT('',#37207);
#6271=VERTEX_POINT('',#37213);
#6272=VERTEX_POINT('',#37215);
#6273=VERTEX_POINT('',#37219);
#6274=VERTEX_POINT('',#37225);
#6275=VERTEX_POINT('',#37227);
#6276=VERTEX_POINT('',#37231);
#6277=VERTEX_POINT('',#37237);
#6278=VERTEX_POINT('',#37239);
#6279=VERTEX_POINT('',#37243);
#6280=VERTEX_POINT('',#37249);
#6281=VERTEX_POINT('',#37251);
#6282=VERTEX_POINT('',#37255);
#6283=VERTEX_POINT('',#37261);
#6284=VERTEX_POINT('',#37263);
#6285=VERTEX_POINT('',#37267);
#6286=VERTEX_POINT('',#37273);
#6287=VERTEX_POINT('',#37275);
#6288=VERTEX_POINT('',#37279);
#6289=VERTEX_POINT('',#37285);
#6290=VERTEX_POINT('',#37287);
#6291=VERTEX_POINT('',#37291);
#6292=VERTEX_POINT('',#37297);
#6293=VERTEX_POINT('',#37299);
#6294=VERTEX_POINT('',#37303);
#6295=VERTEX_POINT('',#37309);
#6296=VERTEX_POINT('',#37311);
#6297=VERTEX_POINT('',#37315);
#6298=VERTEX_POINT('',#37323);
#6299=VERTEX_POINT('',#37324);
#6300=VERTEX_POINT('',#37326);
#6301=VERTEX_POINT('',#37328);
#6302=VERTEX_POINT('',#37330);
#6303=VERTEX_POINT('',#37332);
#6304=VERTEX_POINT('',#37336);
#6305=VERTEX_POINT('',#37337);
#6306=VERTEX_POINT('',#37341);
#6307=VERTEX_POINT('',#37345);
#6308=VERTEX_POINT('',#37349);
#6309=VERTEX_POINT('',#37353);
#6310=VERTEX_POINT('',#37360);
#7464=EDGE_CURVE('',#5966,#5967,#4083,.T.);
#7465=EDGE_CURVE('',#5968,#5966,#1141,.T.);
#7466=EDGE_CURVE('',#5969,#5968,#3562,.T.);
#7467=EDGE_CURVE('',#5969,#5967,#1142,.T.);
#7468=EDGE_CURVE('',#5970,#5971,#4084,.T.);
#7469=EDGE_CURVE('',#5972,#5970,#1143,.F.);
#7470=EDGE_CURVE('',#5966,#5972,#1144,.T.);
#7471=EDGE_CURVE('',#5967,#5973,#1145,.T.);
#7472=EDGE_CURVE('',#5973,#5971,#1146,.T.);
#7473=EDGE_CURVE('',#5974,#5975,#4085,.T.);
#7474=EDGE_CURVE('',#5970,#5974,#1147,.F.);
#7475=EDGE_CURVE('',#5971,#5975,#1148,.T.);
#7476=EDGE_CURVE('',#5976,#5977,#4086,.T.);
#7477=EDGE_CURVE('',#5978,#5976,#1149,.F.);
#7478=EDGE_CURVE('',#5974,#5978,#1150,.F.);
#7479=EDGE_CURVE('',#5975,#5979,#1151,.T.);
#7480=EDGE_CURVE('',#5979,#5977,#1152,.T.);
#7481=EDGE_CURVE('',#5980,#5981,#4087,.T.);
#7482=EDGE_CURVE('',#5976,#5980,#1153,.F.);
#7483=EDGE_CURVE('',#5977,#5981,#1154,.T.);
#7484=EDGE_CURVE('',#5982,#5983,#4088,.T.);
#7485=EDGE_CURVE('',#5984,#5982,#1155,.F.);
#7486=EDGE_CURVE('',#5980,#5984,#1156,.F.);
#7487=EDGE_CURVE('',#5981,#5985,#1157,.T.);
#7488=EDGE_CURVE('',#5985,#5983,#1158,.T.);
#7489=EDGE_CURVE('',#5986,#5987,#4089,.T.);
#7490=EDGE_CURVE('',#5982,#5986,#1159,.F.);
#7491=EDGE_CURVE('',#5983,#5987,#1160,.T.);
#7492=EDGE_CURVE('',#5988,#5989,#4090,.T.);
#7493=EDGE_CURVE('',#5990,#5988,#1161,.F.);
#7494=EDGE_CURVE('',#5986,#5990,#1162,.F.);
#7495=EDGE_CURVE('',#5987,#5991,#1163,.T.);
#7496=EDGE_CURVE('',#5991,#5989,#1164,.T.);
#7497=EDGE_CURVE('',#5992,#5993,#4091,.T.);
#7498=EDGE_CURVE('',#5988,#5992,#1165,.F.);
#7499=EDGE_CURVE('',#5989,#5994,#1166,.T.);
#7500=EDGE_CURVE('',#5994,#5993,#1167,.T.);
#7501=EDGE_CURVE('',#5995,#5996,#4092,.T.);
#7502=EDGE_CURVE('',#5997,#5995,#1168,.T.);
#7503=EDGE_CURVE('',#5992,#5997,#1169,.F.);
#7504=EDGE_CURVE('',#5993,#5998,#1170,.T.);
#7505=EDGE_CURVE('',#5998,#5996,#1171,.T.);
#7506=EDGE_CURVE('',#5999,#6000,#4093,.T.);
#7507=EDGE_CURVE('',#6001,#5999,#1172,.T.);
#7508=EDGE_CURVE('',#5995,#6001,#1173,.T.);
#7509=EDGE_CURVE('',#5996,#6000,#1174,.T.);
#7510=EDGE_CURVE('',#6002,#6003,#4094,.T.);
#7511=EDGE_CURVE('',#6004,#6002,#1175,.F.);
#7512=EDGE_CURVE('',#5999,#6004,#1176,.T.);
#7513=EDGE_CURVE('',#6000,#6005,#1177,.T.);
#7514=EDGE_CURVE('',#6005,#6003,#1178,.T.);
#7515=EDGE_CURVE('',#6006,#6007,#4095,.T.);
#7516=EDGE_CURVE('',#6002,#6006,#1179,.F.);
#7517=EDGE_CURVE('',#6003,#6007,#1180,.T.);
#7518=EDGE_CURVE('',#6008,#6009,#4096,.T.);
#7519=EDGE_CURVE('',#6010,#6008,#1181,.F.);
#7520=EDGE_CURVE('',#6006,#6010,#1182,.F.);
#7521=EDGE_CURVE('',#6007,#6011,#1183,.T.);
#7522=EDGE_CURVE('',#6011,#6009,#1184,.T.);
#7523=EDGE_CURVE('',#6012,#6013,#4097,.T.);
#7524=EDGE_CURVE('',#6008,#6012,#1185,.F.);
#7525=EDGE_CURVE('',#6009,#6013,#1186,.T.);
#7526=EDGE_CURVE('',#6014,#6015,#4098,.T.);
#7527=EDGE_CURVE('',#6016,#6014,#1187,.F.);
#7528=EDGE_CURVE('',#6012,#6016,#1188,.F.);
#7529=EDGE_CURVE('',#6013,#6017,#1189,.T.);
#7530=EDGE_CURVE('',#6017,#6015,#1190,.T.);
#7531=EDGE_CURVE('',#6018,#6019,#4099,.T.);
#7532=EDGE_CURVE('',#6014,#6018,#1191,.F.);
#7533=EDGE_CURVE('',#6015,#6019,#1192,.T.);
#7534=EDGE_CURVE('',#6020,#6021,#4100,.T.);
#7535=EDGE_CURVE('',#6022,#6020,#1193,.F.);
#7536=EDGE_CURVE('',#6018,#6022,#1194,.F.);
#7537=EDGE_CURVE('',#6019,#6023,#1195,.T.);
#7538=EDGE_CURVE('',#6023,#6021,#1196,.T.);
#7539=EDGE_CURVE('',#6024,#6025,#4101,.T.);
#7540=EDGE_CURVE('',#6020,#6024,#1197,.F.);
#7541=EDGE_CURVE('',#6021,#6025,#1198,.T.);
#7542=EDGE_CURVE('',#6026,#6027,#1199,.T.);
#7543=EDGE_CURVE('',#6028,#6027,#3563,.T.);
#7544=EDGE_CURVE('',#6028,#6029,#1200,.T.);
#7545=EDGE_CURVE('',#6029,#6030,#1201,.T.);
#7546=EDGE_CURVE('',#6030,#6031,#1202,.T.);
#7547=EDGE_CURVE('',#6031,#6032,#1203,.T.);
#7548=EDGE_CURVE('',#6032,#6033,#1204,.T.);
#7549=EDGE_CURVE('',#6033,#6034,#1205,.T.);
#7550=EDGE_CURVE('',#6034,#6035,#1206,.T.);
#7551=EDGE_CURVE('',#6035,#6036,#1207,.T.);
#7552=EDGE_CURVE('',#6036,#6037,#1208,.T.);
#7553=EDGE_CURVE('',#6037,#6038,#1209,.T.);
#7554=EDGE_CURVE('',#6038,#6039,#1210,.T.);
#7555=EDGE_CURVE('',#6039,#6040,#1211,.T.);
#7556=EDGE_CURVE('',#6040,#6041,#1212,.T.);
#7557=EDGE_CURVE('',#6041,#6042,#1213,.T.);
#7558=EDGE_CURVE('',#6042,#6043,#1214,.T.);
#7559=EDGE_CURVE('',#6043,#6044,#1215,.T.);
#7560=EDGE_CURVE('',#6044,#6045,#1216,.T.);
#7561=EDGE_CURVE('',#6045,#6046,#1217,.T.);
#7562=EDGE_CURVE('',#6046,#6047,#1218,.T.);
#7563=EDGE_CURVE('',#6047,#6048,#1219,.T.);
#7564=EDGE_CURVE('',#6048,#6049,#1220,.T.);
#7565=EDGE_CURVE('',#6050,#6049,#3564,.T.);
#7566=EDGE_CURVE('',#6051,#6050,#3565,.T.);
#7567=EDGE_CURVE('',#6051,#6052,#1221,.T.);
#7568=EDGE_CURVE('',#6052,#6053,#1222,.T.);
#7569=EDGE_CURVE('',#6053,#6054,#1223,.T.);
#7570=EDGE_CURVE('',#6054,#6055,#1224,.T.);
#7571=EDGE_CURVE('',#6055,#6056,#1225,.T.);
#7572=EDGE_CURVE('',#6056,#6057,#1226,.T.);
#7573=EDGE_CURVE('',#6057,#6058,#1227,.T.);
#7574=EDGE_CURVE('',#6058,#6059,#1228,.T.);
#7575=EDGE_CURVE('',#6059,#6060,#1229,.T.);
#7576=EDGE_CURVE('',#6060,#6061,#1230,.T.);
#7577=EDGE_CURVE('',#6061,#6062,#1231,.T.);
#7578=EDGE_CURVE('',#6062,#6063,#1232,.T.);
#7579=EDGE_CURVE('',#6063,#6064,#1233,.T.);
#7580=EDGE_CURVE('',#6064,#6065,#1234,.T.);
#7581=EDGE_CURVE('',#6065,#6066,#1235,.T.);
#7582=EDGE_CURVE('',#6066,#6067,#1236,.T.);
#7583=EDGE_CURVE('',#6067,#6068,#1237,.T.);
#7584=EDGE_CURVE('',#6068,#6069,#1238,.T.);
#7585=EDGE_CURVE('',#6069,#6026,#1239,.T.);
#7586=EDGE_CURVE('',#6025,#6070,#1240,.T.);
#7587=EDGE_CURVE('',#6070,#6071,#1241,.T.);
#7588=EDGE_CURVE('',#6072,#6071,#3566,.T.);
#7589=EDGE_CURVE('',#6073,#6072,#1242,.T.);
#7590=EDGE_CURVE('',#6024,#6073,#1243,.F.);
#7591=EDGE_CURVE('',#6074,#6051,#3567,.T.);
#7592=EDGE_CURVE('',#6074,#6072,#1244,.T.);
#7593=EDGE_CURVE('',#6071,#6051,#1245,.T.);
#7594=EDGE_CURVE('',#6049,#6074,#1246,.T.);
#7595=EDGE_CURVE('',#5968,#6028,#1247,.T.);
#7596=EDGE_CURVE('',#6075,#6076,#3568,.T.);
#7597=EDGE_CURVE('',#6075,#5969,#1248,.T.);
#7598=EDGE_CURVE('',#6076,#6028,#3569,.T.);
#7599=EDGE_CURVE('',#6027,#6075,#1249,.T.);
#7600=EDGE_CURVE('',#6077,#6077,#3570,.T.);
#7601=EDGE_CURVE('',#6077,#6076,#3571,.T.);
#7602=EDGE_CURVE('',#6078,#6078,#3572,.T.);
#7603=EDGE_CURVE('',#6050,#6079,#4102,.T.);
#7604=EDGE_CURVE('',#6079,#6079,#3573,.T.);
#7605=EDGE_CURVE('',#6080,#6081,#4103,.T.);
#7606=EDGE_CURVE('',#6080,#6082,#4104,.T.);
#7607=EDGE_CURVE('',#6083,#6082,#4105,.T.);
#7608=EDGE_CURVE('',#6081,#6083,#787,.T.);
#7609=EDGE_CURVE('',#6084,#6085,#4106,.T.);
#7610=EDGE_CURVE('',#6083,#6084,#788,.T.);
#7611=EDGE_CURVE('',#6082,#6085,#4107,.T.);
#7612=EDGE_CURVE('',#6085,#6080,#3574,.T.);
#7613=EDGE_CURVE('',#6086,#6087,#789,.T.);
#7614=EDGE_CURVE('',#6087,#6088,#3575,.T.);
#7615=EDGE_CURVE('',#6088,#6089,#790,.T.);
#7616=EDGE_CURVE('',#6089,#6090,#791,.T.);
#7617=EDGE_CURVE('',#6090,#6091,#3576,.T.);
#7618=EDGE_CURVE('',#6091,#6092,#792,.T.);
#7619=EDGE_CURVE('',#6092,#6093,#793,.T.);
#7620=EDGE_CURVE('',#6093,#6094,#3577,.T.);
#7621=EDGE_CURVE('',#6094,#6095,#794,.T.);
#7622=EDGE_CURVE('',#6095,#6096,#795,.T.);
#7623=EDGE_CURVE('',#6096,#6097,#3578,.T.);
#7624=EDGE_CURVE('',#6097,#6098,#796,.T.);
#7625=EDGE_CURVE('',#6098,#6099,#797,.T.);
#7626=EDGE_CURVE('',#6099,#6100,#3579,.T.);
#7627=EDGE_CURVE('',#6100,#6101,#798,.T.);
#7628=EDGE_CURVE('',#6101,#6102,#799,.T.);
#7629=EDGE_CURVE('',#6102,#6103,#3580,.T.);
#7630=EDGE_CURVE('',#6103,#6104,#800,.T.);
#7631=EDGE_CURVE('',#6104,#6105,#801,.T.);
#7632=EDGE_CURVE('',#6105,#6106,#3581,.T.);
#7633=EDGE_CURVE('',#6106,#6107,#802,.T.);
#7634=EDGE_CURVE('',#6107,#6108,#803,.T.);
#7635=EDGE_CURVE('',#6108,#6109,#3582,.T.);
#7636=EDGE_CURVE('',#6109,#6110,#804,.T.);
#7637=EDGE_CURVE('',#6110,#6111,#805,.T.);
#7638=EDGE_CURVE('',#6111,#6112,#3583,.T.);
#7639=EDGE_CURVE('',#6112,#6113,#806,.T.);
#7640=EDGE_CURVE('',#6113,#6114,#807,.T.);
#7641=EDGE_CURVE('',#6114,#6115,#3584,.T.);
#7642=EDGE_CURVE('',#6115,#6116,#808,.T.);
#7643=EDGE_CURVE('',#6116,#6117,#809,.T.);
#7644=EDGE_CURVE('',#6117,#6118,#3585,.T.);
#7645=EDGE_CURVE('',#6118,#6119,#810,.T.);
#7646=EDGE_CURVE('',#6119,#6120,#811,.T.);
#7647=EDGE_CURVE('',#6120,#6121,#3586,.T.);
#7648=EDGE_CURVE('',#6121,#6122,#812,.T.);
#7649=EDGE_CURVE('',#6122,#6123,#813,.T.);
#7650=EDGE_CURVE('',#6123,#6124,#3587,.T.);
#7651=EDGE_CURVE('',#6124,#6125,#814,.T.);
#7652=EDGE_CURVE('',#6125,#6126,#815,.T.);
#7653=EDGE_CURVE('',#6126,#6127,#3588,.T.);
#7654=EDGE_CURVE('',#6127,#6128,#816,.T.);
#7655=EDGE_CURVE('',#6128,#6129,#817,.T.);
#7656=EDGE_CURVE('',#6129,#6130,#3589,.T.);
#7657=EDGE_CURVE('',#6130,#6131,#818,.T.);
#7658=EDGE_CURVE('',#6131,#6132,#819,.T.);
#7659=EDGE_CURVE('',#6132,#6133,#3590,.T.);
#7660=EDGE_CURVE('',#6133,#6134,#820,.T.);
#7661=EDGE_CURVE('',#6134,#6135,#821,.T.);
#7662=EDGE_CURVE('',#6135,#6136,#3591,.T.);
#7663=EDGE_CURVE('',#6136,#6137,#822,.T.);
#7664=EDGE_CURVE('',#6137,#6138,#823,.T.);
#7665=EDGE_CURVE('',#6138,#6139,#3592,.T.);
#7666=EDGE_CURVE('',#6139,#6140,#824,.T.);
#7667=EDGE_CURVE('',#6140,#6141,#825,.T.);
#7668=EDGE_CURVE('',#6141,#6081,#3593,.T.);
#7669=EDGE_CURVE('',#6084,#6142,#3594,.T.);
#7670=EDGE_CURVE('',#6142,#6143,#826,.T.);
#7671=EDGE_CURVE('',#6143,#6144,#827,.T.);
#7672=EDGE_CURVE('',#6144,#6145,#3595,.T.);
#7673=EDGE_CURVE('',#6145,#6146,#828,.T.);
#7674=EDGE_CURVE('',#6146,#6147,#829,.T.);
#7675=EDGE_CURVE('',#6147,#6148,#3596,.T.);
#7676=EDGE_CURVE('',#6148,#6149,#830,.T.);
#7677=EDGE_CURVE('',#6149,#6150,#831,.T.);
#7678=EDGE_CURVE('',#6150,#6151,#3597,.T.);
#7679=EDGE_CURVE('',#6151,#6152,#832,.T.);
#7680=EDGE_CURVE('',#6152,#6153,#833,.T.);
#7681=EDGE_CURVE('',#6153,#6154,#3598,.T.);
#7682=EDGE_CURVE('',#6154,#6155,#834,.T.);
#7683=EDGE_CURVE('',#6155,#6156,#835,.T.);
#7684=EDGE_CURVE('',#6156,#6157,#3599,.T.);
#7685=EDGE_CURVE('',#6157,#6158,#836,.T.);
#7686=EDGE_CURVE('',#6158,#6159,#837,.T.);
#7687=EDGE_CURVE('',#6159,#6160,#3600,.T.);
#7688=EDGE_CURVE('',#6160,#6161,#838,.T.);
#7689=EDGE_CURVE('',#6161,#6162,#839,.T.);
#7690=EDGE_CURVE('',#6162,#6163,#3601,.T.);
#7691=EDGE_CURVE('',#6163,#6164,#840,.T.);
#7692=EDGE_CURVE('',#6164,#6165,#841,.T.);
#7693=EDGE_CURVE('',#6165,#6166,#3602,.T.);
#7694=EDGE_CURVE('',#6166,#6167,#842,.T.);
#7695=EDGE_CURVE('',#6167,#6168,#843,.T.);
#7696=EDGE_CURVE('',#6168,#6169,#3603,.T.);
#7697=EDGE_CURVE('',#6169,#6170,#844,.T.);
#7698=EDGE_CURVE('',#6170,#6171,#845,.T.);
#7699=EDGE_CURVE('',#6171,#6172,#3604,.T.);
#7700=EDGE_CURVE('',#6172,#6173,#846,.T.);
#7701=EDGE_CURVE('',#6173,#6174,#847,.T.);
#7702=EDGE_CURVE('',#6174,#6175,#3605,.T.);
#7703=EDGE_CURVE('',#6175,#6176,#848,.T.);
#7704=EDGE_CURVE('',#6176,#6177,#849,.T.);
#7705=EDGE_CURVE('',#6177,#6178,#3606,.T.);
#7706=EDGE_CURVE('',#6178,#6179,#850,.T.);
#7707=EDGE_CURVE('',#6179,#6180,#851,.T.);
#7708=EDGE_CURVE('',#6180,#6181,#3607,.T.);
#7709=EDGE_CURVE('',#6181,#6182,#852,.T.);
#7710=EDGE_CURVE('',#6182,#6183,#853,.T.);
#7711=EDGE_CURVE('',#6183,#6184,#3608,.T.);
#7712=EDGE_CURVE('',#6184,#6185,#854,.T.);
#7713=EDGE_CURVE('',#6185,#6186,#855,.T.);
#7714=EDGE_CURVE('',#6186,#6187,#3609,.T.);
#7715=EDGE_CURVE('',#6187,#6188,#856,.T.);
#7716=EDGE_CURVE('',#6188,#6189,#857,.T.);
#7717=EDGE_CURVE('',#6189,#6190,#3610,.T.);
#7718=EDGE_CURVE('',#6190,#6086,#858,.T.);
#7719=EDGE_CURVE('',#6086,#6191,#4108,.T.);
#7720=EDGE_CURVE('',#6191,#6191,#3611,.T.);
#7721=EDGE_CURVE('',#6192,#6142,#4109,.T.);
#7722=EDGE_CURVE('',#6192,#6193,#4110,.T.);
#7723=EDGE_CURVE('',#6143,#6193,#4111,.T.);
#7724=EDGE_CURVE('',#6144,#6194,#4112,.T.);
#7725=EDGE_CURVE('',#6193,#6194,#4113,.T.);
#7726=EDGE_CURVE('',#6194,#6192,#3612,.T.);
#7727=EDGE_CURVE('',#6195,#6145,#4114,.T.);
#7728=EDGE_CURVE('',#6195,#6196,#4115,.T.);
#7729=EDGE_CURVE('',#6146,#6196,#4116,.T.);
#7730=EDGE_CURVE('',#6147,#6197,#4117,.T.);
#7731=EDGE_CURVE('',#6196,#6197,#4118,.T.);
#7732=EDGE_CURVE('',#6197,#6195,#3613,.T.);
#7733=EDGE_CURVE('',#6198,#6148,#4119,.T.);
#7734=EDGE_CURVE('',#6198,#6199,#4120,.T.);
#7735=EDGE_CURVE('',#6149,#6199,#4121,.T.);
#7736=EDGE_CURVE('',#6150,#6200,#4122,.T.);
#7737=EDGE_CURVE('',#6199,#6200,#4123,.T.);
#7738=EDGE_CURVE('',#6200,#6198,#3614,.T.);
#7739=EDGE_CURVE('',#6201,#6151,#4124,.T.);
#7740=EDGE_CURVE('',#6201,#6202,#4125,.T.);
#7741=EDGE_CURVE('',#6152,#6202,#4126,.T.);
#7742=EDGE_CURVE('',#6153,#6203,#4127,.T.);
#7743=EDGE_CURVE('',#6202,#6203,#4128,.T.);
#7744=EDGE_CURVE('',#6203,#6201,#3615,.T.);
#7745=EDGE_CURVE('',#6204,#6154,#4129,.T.);
#7746=EDGE_CURVE('',#6204,#6205,#4130,.T.);
#7747=EDGE_CURVE('',#6155,#6205,#4131,.T.);
#7748=EDGE_CURVE('',#6156,#6206,#4132,.T.);
#7749=EDGE_CURVE('',#6205,#6206,#4133,.T.);
#7750=EDGE_CURVE('',#6206,#6204,#3616,.T.);
#7751=EDGE_CURVE('',#6207,#6157,#4134,.T.);
#7752=EDGE_CURVE('',#6207,#6208,#4135,.T.);
#7753=EDGE_CURVE('',#6158,#6208,#4136,.T.);
#7754=EDGE_CURVE('',#6159,#6209,#4137,.T.);
#7755=EDGE_CURVE('',#6208,#6209,#4138,.T.);
#7756=EDGE_CURVE('',#6209,#6207,#3617,.T.);
#7757=EDGE_CURVE('',#6210,#6160,#4139,.T.);
#7758=EDGE_CURVE('',#6210,#6211,#4140,.T.);
#7759=EDGE_CURVE('',#6161,#6211,#4141,.T.);
#7760=EDGE_CURVE('',#6162,#6212,#4142,.T.);
#7761=EDGE_CURVE('',#6211,#6212,#4143,.T.);
#7762=EDGE_CURVE('',#6212,#6210,#3618,.T.);
#7763=EDGE_CURVE('',#6213,#6163,#4144,.T.);
#7764=EDGE_CURVE('',#6213,#6214,#4145,.T.);
#7765=EDGE_CURVE('',#6164,#6214,#4146,.T.);
#7766=EDGE_CURVE('',#6165,#6215,#4147,.T.);
#7767=EDGE_CURVE('',#6214,#6215,#4148,.T.);
#7768=EDGE_CURVE('',#6215,#6213,#3619,.T.);
#7769=EDGE_CURVE('',#6216,#6166,#4149,.T.);
#7770=EDGE_CURVE('',#6216,#6217,#4150,.T.);
#7771=EDGE_CURVE('',#6167,#6217,#4151,.T.);
#7772=EDGE_CURVE('',#6168,#6218,#4152,.T.);
#7773=EDGE_CURVE('',#6217,#6218,#4153,.T.);
#7774=EDGE_CURVE('',#6218,#6216,#3620,.T.);
#7775=EDGE_CURVE('',#6219,#6169,#4154,.T.);
#7776=EDGE_CURVE('',#6219,#6220,#4155,.T.);
#7777=EDGE_CURVE('',#6170,#6220,#4156,.T.);
#7778=EDGE_CURVE('',#6171,#6221,#4157,.T.);
#7779=EDGE_CURVE('',#6220,#6221,#4158,.T.);
#7780=EDGE_CURVE('',#6221,#6219,#3621,.T.);
#7781=EDGE_CURVE('',#6222,#6172,#4159,.T.);
#7782=EDGE_CURVE('',#6222,#6223,#4160,.T.);
#7783=EDGE_CURVE('',#6173,#6223,#4161,.T.);
#7784=EDGE_CURVE('',#6174,#6224,#4162,.T.);
#7785=EDGE_CURVE('',#6223,#6224,#4163,.T.);
#7786=EDGE_CURVE('',#6224,#6222,#3622,.T.);
#7787=EDGE_CURVE('',#6225,#6175,#4164,.T.);
#7788=EDGE_CURVE('',#6225,#6226,#4165,.T.);
#7789=EDGE_CURVE('',#6176,#6226,#4166,.T.);
#7790=EDGE_CURVE('',#6177,#6227,#4167,.T.);
#7791=EDGE_CURVE('',#6226,#6227,#4168,.T.);
#7792=EDGE_CURVE('',#6227,#6225,#3623,.T.);
#7793=EDGE_CURVE('',#6228,#6178,#4169,.T.);
#7794=EDGE_CURVE('',#6228,#6229,#4170,.T.);
#7795=EDGE_CURVE('',#6179,#6229,#4171,.T.);
#7796=EDGE_CURVE('',#6180,#6230,#4172,.T.);
#7797=EDGE_CURVE('',#6229,#6230,#4173,.T.);
#7798=EDGE_CURVE('',#6230,#6228,#3624,.T.);
#7799=EDGE_CURVE('',#6231,#6181,#4174,.T.);
#7800=EDGE_CURVE('',#6231,#6232,#4175,.T.);
#7801=EDGE_CURVE('',#6182,#6232,#4176,.T.);
#7802=EDGE_CURVE('',#6183,#6233,#4177,.T.);
#7803=EDGE_CURVE('',#6232,#6233,#4178,.T.);
#7804=EDGE_CURVE('',#6233,#6231,#3625,.T.);
#7805=EDGE_CURVE('',#6234,#6184,#4179,.T.);
#7806=EDGE_CURVE('',#6234,#6235,#4180,.T.);
#7807=EDGE_CURVE('',#6185,#6235,#4181,.T.);
#7808=EDGE_CURVE('',#6186,#6236,#4182,.T.);
#7809=EDGE_CURVE('',#6235,#6236,#4183,.T.);
#7810=EDGE_CURVE('',#6236,#6234,#3626,.T.);
#7811=EDGE_CURVE('',#6237,#6187,#4184,.T.);
#7812=EDGE_CURVE('',#6237,#6238,#4185,.T.);
#7813=EDGE_CURVE('',#6188,#6238,#4186,.T.);
#7814=EDGE_CURVE('',#6189,#6239,#4187,.T.);
#7815=EDGE_CURVE('',#6238,#6239,#4188,.T.);
#7816=EDGE_CURVE('',#6239,#6237,#3627,.T.);
#7817=EDGE_CURVE('',#6240,#6190,#4189,.T.);
#7818=EDGE_CURVE('',#6240,#6241,#4190,.T.);
#7819=EDGE_CURVE('',#6086,#6241,#4191,.T.);
#7820=EDGE_CURVE('',#6087,#6242,#4192,.T.);
#7821=EDGE_CURVE('',#6241,#6242,#4193,.T.);
#7822=EDGE_CURVE('',#6242,#6243,#3628,.T.);
#7823=EDGE_CURVE('',#6243,#6240,#3629,.T.);
#7824=EDGE_CURVE('',#6244,#6088,#4194,.T.);
#7825=EDGE_CURVE('',#6244,#6245,#4195,.T.);
#7826=EDGE_CURVE('',#6089,#6245,#4196,.T.);
#7827=EDGE_CURVE('',#6090,#6246,#4197,.T.);
#7828=EDGE_CURVE('',#6245,#6246,#4198,.T.);
#7829=EDGE_CURVE('',#6246,#6244,#3630,.T.);
#7830=EDGE_CURVE('',#6247,#6091,#4199,.T.);
#7831=EDGE_CURVE('',#6247,#6248,#4200,.T.);
#7832=EDGE_CURVE('',#6092,#6248,#4201,.T.);
#7833=EDGE_CURVE('',#6093,#6249,#4202,.T.);
#7834=EDGE_CURVE('',#6248,#6249,#4203,.T.);
#7835=EDGE_CURVE('',#6249,#6247,#3631,.T.);
#7836=EDGE_CURVE('',#6250,#6094,#4204,.T.);
#7837=EDGE_CURVE('',#6250,#6251,#4205,.T.);
#7838=EDGE_CURVE('',#6095,#6251,#4206,.T.);
#7839=EDGE_CURVE('',#6096,#6252,#4207,.T.);
#7840=EDGE_CURVE('',#6251,#6252,#4208,.T.);
#7841=EDGE_CURVE('',#6252,#6250,#3632,.T.);
#7842=EDGE_CURVE('',#6253,#6097,#4209,.T.);
#7843=EDGE_CURVE('',#6253,#6254,#4210,.T.);
#7844=EDGE_CURVE('',#6098,#6254,#4211,.T.);
#7845=EDGE_CURVE('',#6099,#6255,#4212,.T.);
#7846=EDGE_CURVE('',#6254,#6255,#4213,.T.);
#7847=EDGE_CURVE('',#6255,#6253,#3633,.T.);
#7848=EDGE_CURVE('',#6256,#6100,#4214,.T.);
#7849=EDGE_CURVE('',#6256,#6257,#4215,.T.);
#7850=EDGE_CURVE('',#6101,#6257,#4216,.T.);
#7851=EDGE_CURVE('',#6102,#6258,#4217,.T.);
#7852=EDGE_CURVE('',#6257,#6258,#4218,.T.);
#7853=EDGE_CURVE('',#6258,#6256,#3634,.T.);
#7854=EDGE_CURVE('',#6259,#6103,#4219,.T.);
#7855=EDGE_CURVE('',#6259,#6260,#4220,.T.);
#7856=EDGE_CURVE('',#6104,#6260,#4221,.T.);
#7857=EDGE_CURVE('',#6105,#6261,#4222,.T.);
#7858=EDGE_CURVE('',#6260,#6261,#4223,.T.);
#7859=EDGE_CURVE('',#6261,#6259,#3635,.T.);
#7860=EDGE_CURVE('',#6262,#6106,#4224,.T.);
#7861=EDGE_CURVE('',#6262,#6263,#4225,.T.);
#7862=EDGE_CURVE('',#6107,#6263,#4226,.T.);
#7863=EDGE_CURVE('',#6108,#6264,#4227,.T.);
#7864=EDGE_CURVE('',#6263,#6264,#4228,.T.);
#7865=EDGE_CURVE('',#6264,#6262,#3636,.T.);
#7866=EDGE_CURVE('',#6265,#6109,#4229,.T.);
#7867=EDGE_CURVE('',#6265,#6266,#4230,.T.);
#7868=EDGE_CURVE('',#6110,#6266,#4231,.T.);
#7869=EDGE_CURVE('',#6111,#6267,#4232,.T.);
#7870=EDGE_CURVE('',#6266,#6267,#4233,.T.);
#7871=EDGE_CURVE('',#6267,#6265,#3637,.T.);
#7872=EDGE_CURVE('',#6268,#6112,#4234,.T.);
#7873=EDGE_CURVE('',#6268,#6269,#4235,.T.);
#7874=EDGE_CURVE('',#6113,#6269,#4236,.T.);
#7875=EDGE_CURVE('',#6114,#6270,#4237,.T.);
#7876=EDGE_CURVE('',#6269,#6270,#4238,.T.);
#7877=EDGE_CURVE('',#6270,#6268,#3638,.T.);
#7878=EDGE_CURVE('',#6271,#6115,#4239,.T.);
#7879=EDGE_CURVE('',#6271,#6272,#4240,.T.);
#7880=EDGE_CURVE('',#6116,#6272,#4241,.T.);
#7881=EDGE_CURVE('',#6117,#6273,#4242,.T.);
#7882=EDGE_CURVE('',#6272,#6273,#4243,.T.);
#7883=EDGE_CURVE('',#6273,#6271,#3639,.T.);
#7884=EDGE_CURVE('',#6274,#6118,#4244,.T.);
#7885=EDGE_CURVE('',#6274,#6275,#4245,.T.);
#7886=EDGE_CURVE('',#6119,#6275,#4246,.T.);
#7887=EDGE_CURVE('',#6120,#6276,#4247,.T.);
#7888=EDGE_CURVE('',#6275,#6276,#4248,.T.);
#7889=EDGE_CURVE('',#6276,#6274,#3640,.T.);
#7890=EDGE_CURVE('',#6277,#6121,#4249,.T.);
#7891=EDGE_CURVE('',#6277,#6278,#4250,.T.);
#7892=EDGE_CURVE('',#6122,#6278,#4251,.T.);
#7893=EDGE_CURVE('',#6123,#6279,#4252,.T.);
#7894=EDGE_CURVE('',#6278,#6279,#4253,.T.);
#7895=EDGE_CURVE('',#6279,#6277,#3641,.T.);
#7896=EDGE_CURVE('',#6280,#6124,#4254,.T.);
#7897=EDGE_CURVE('',#6280,#6281,#4255,.T.);
#7898=EDGE_CURVE('',#6125,#6281,#4256,.T.);
#7899=EDGE_CURVE('',#6126,#6282,#4257,.T.);
#7900=EDGE_CURVE('',#6281,#6282,#4258,.T.);
#7901=EDGE_CURVE('',#6282,#6280,#3642,.T.);
#7902=EDGE_CURVE('',#6283,#6127,#4259,.T.);
#7903=EDGE_CURVE('',#6283,#6284,#4260,.T.);
#7904=EDGE_CURVE('',#6128,#6284,#4261,.T.);
#7905=EDGE_CURVE('',#6129,#6285,#4262,.T.);
#7906=EDGE_CURVE('',#6284,#6285,#4263,.T.);
#7907=EDGE_CURVE('',#6285,#6283,#3643,.T.);
#7908=EDGE_CURVE('',#6286,#6130,#4264,.T.);
#7909=EDGE_CURVE('',#6286,#6287,#4265,.T.);
#7910=EDGE_CURVE('',#6131,#6287,#4266,.T.);
#7911=EDGE_CURVE('',#6132,#6288,#4267,.T.);
#7912=EDGE_CURVE('',#6287,#6288,#4268,.T.);
#7913=EDGE_CURVE('',#6288,#6286,#3644,.T.);
#7914=EDGE_CURVE('',#6289,#6133,#4269,.T.);
#7915=EDGE_CURVE('',#6289,#6290,#4270,.T.);
#7916=EDGE_CURVE('',#6134,#6290,#4271,.T.);
#7917=EDGE_CURVE('',#6135,#6291,#4272,.T.);
#7918=EDGE_CURVE('',#6290,#6291,#4273,.T.);
#7919=EDGE_CURVE('',#6291,#6289,#3645,.T.);
#7920=EDGE_CURVE('',#6292,#6136,#4274,.T.);
#7921=EDGE_CURVE('',#6292,#6293,#4275,.T.);
#7922=EDGE_CURVE('',#6137,#6293,#4276,.T.);
#7923=EDGE_CURVE('',#6138,#6294,#4277,.T.);
#7924=EDGE_CURVE('',#6293,#6294,#4278,.T.);
#7925=EDGE_CURVE('',#6294,#6292,#3646,.T.);
#7926=EDGE_CURVE('',#6295,#6139,#4279,.T.);
#7927=EDGE_CURVE('',#6295,#6296,#4280,.T.);
#7928=EDGE_CURVE('',#6140,#6296,#4281,.T.);
#7929=EDGE_CURVE('',#6141,#6297,#4282,.T.);
#7930=EDGE_CURVE('',#6296,#6297,#4283,.T.);
#7931=EDGE_CURVE('',#6297,#6295,#3647,.T.);
#7932=EDGE_CURVE('',#6243,#6078,#4284,.T.);
#7933=EDGE_CURVE('',#6298,#6299,#4285,.T.);
#7934=EDGE_CURVE('',#6299,#6300,#4286,.T.);
#7935=EDGE_CURVE('',#6300,#6301,#4287,.T.);
#7936=EDGE_CURVE('',#6301,#6302,#4288,.T.);
#7937=EDGE_CURVE('',#6302,#6303,#4289,.T.);
#7938=EDGE_CURVE('',#6303,#6298,#4290,.T.);
#7939=EDGE_CURVE('',#6304,#6305,#4291,.T.);
#7940=EDGE_CURVE('',#6304,#6305,#3648,.T.);
#7941=EDGE_CURVE('',#6305,#6306,#4292,.T.);
#7942=EDGE_CURVE('',#6305,#6306,#3649,.T.);
#7943=EDGE_CURVE('',#6306,#6307,#4293,.T.);
#7944=EDGE_CURVE('',#6306,#6307,#3650,.T.);
#7945=EDGE_CURVE('',#6307,#6308,#4294,.T.);
#7946=EDGE_CURVE('',#6307,#6308,#3651,.T.);
#7947=EDGE_CURVE('',#6308,#6309,#4295,.T.);
#7948=EDGE_CURVE('',#6308,#6309,#3652,.T.);
#7949=EDGE_CURVE('',#6309,#6304,#4296,.T.);
#7950=EDGE_CURVE('',#6309,#6304,#3653,.T.);
#7951=EDGE_CURVE('',#6310,#6304,#4297,.T.);
#7952=EDGE_CURVE('',#6298,#6304,#4298,.T.);
#7953=EDGE_CURVE('',#6299,#6305,#4299,.T.);
#7954=EDGE_CURVE('',#6303,#6309,#4300,.T.);
#7955=EDGE_CURVE('',#6302,#6308,#4301,.T.);
#7956=EDGE_CURVE('',#6301,#6307,#4302,.T.);
#7957=EDGE_CURVE('',#6300,#6306,#4303,.T.);
#9859=ORIENTED_EDGE('',*,*,#7464,.F.);
#9860=ORIENTED_EDGE('',*,*,#7465,.F.);
#9861=ORIENTED_EDGE('',*,*,#7466,.F.);
#9862=ORIENTED_EDGE('',*,*,#7467,.T.);
#9863=ORIENTED_EDGE('',*,*,#7468,.F.);
#9864=ORIENTED_EDGE('',*,*,#7469,.F.);
#9865=ORIENTED_EDGE('',*,*,#7470,.F.);
#9866=ORIENTED_EDGE('',*,*,#7464,.T.);
#9867=ORIENTED_EDGE('',*,*,#7471,.T.);
#9868=ORIENTED_EDGE('',*,*,#7472,.T.);
#9869=ORIENTED_EDGE('',*,*,#7473,.F.);
#9870=ORIENTED_EDGE('',*,*,#7474,.F.);
#9871=ORIENTED_EDGE('',*,*,#7468,.T.);
#9872=ORIENTED_EDGE('',*,*,#7475,.T.);
#9873=ORIENTED_EDGE('',*,*,#7476,.F.);
#9874=ORIENTED_EDGE('',*,*,#7477,.F.);
#9875=ORIENTED_EDGE('',*,*,#7478,.F.);
#9876=ORIENTED_EDGE('',*,*,#7473,.T.);
#9877=ORIENTED_EDGE('',*,*,#7479,.T.);
#9878=ORIENTED_EDGE('',*,*,#7480,.T.);
#9879=ORIENTED_EDGE('',*,*,#7481,.F.);
#9880=ORIENTED_EDGE('',*,*,#7482,.F.);
#9881=ORIENTED_EDGE('',*,*,#7476,.T.);
#9882=ORIENTED_EDGE('',*,*,#7483,.T.);
#9883=ORIENTED_EDGE('',*,*,#7484,.F.);
#9884=ORIENTED_EDGE('',*,*,#7485,.F.);
#9885=ORIENTED_EDGE('',*,*,#7486,.F.);
#9886=ORIENTED_EDGE('',*,*,#7481,.T.);
#9887=ORIENTED_EDGE('',*,*,#7487,.T.);
#9888=ORIENTED_EDGE('',*,*,#7488,.T.);
#9889=ORIENTED_EDGE('',*,*,#7489,.F.);
#9890=ORIENTED_EDGE('',*,*,#7490,.F.);
#9891=ORIENTED_EDGE('',*,*,#7484,.T.);
#9892=ORIENTED_EDGE('',*,*,#7491,.T.);
#9893=ORIENTED_EDGE('',*,*,#7492,.F.);
#9894=ORIENTED_EDGE('',*,*,#7493,.F.);
#9895=ORIENTED_EDGE('',*,*,#7494,.F.);
#9896=ORIENTED_EDGE('',*,*,#7489,.T.);
#9897=ORIENTED_EDGE('',*,*,#7495,.T.);
#9898=ORIENTED_EDGE('',*,*,#7496,.T.);
#9899=ORIENTED_EDGE('',*,*,#7497,.F.);
#9900=ORIENTED_EDGE('',*,*,#7498,.F.);
#9901=ORIENTED_EDGE('',*,*,#7492,.T.);
#9902=ORIENTED_EDGE('',*,*,#7499,.T.);
#9903=ORIENTED_EDGE('',*,*,#7500,.T.);
#9904=ORIENTED_EDGE('',*,*,#7501,.F.);
#9905=ORIENTED_EDGE('',*,*,#7502,.F.);
#9906=ORIENTED_EDGE('',*,*,#7503,.F.);
#9907=ORIENTED_EDGE('',*,*,#7497,.T.);
#9908=ORIENTED_EDGE('',*,*,#7504,.T.);
#9909=ORIENTED_EDGE('',*,*,#7505,.T.);
#9910=ORIENTED_EDGE('',*,*,#7506,.F.);
#9911=ORIENTED_EDGE('',*,*,#7507,.F.);
#9912=ORIENTED_EDGE('',*,*,#7508,.F.);
#9913=ORIENTED_EDGE('',*,*,#7501,.T.);
#9914=ORIENTED_EDGE('',*,*,#7509,.T.);
#9915=ORIENTED_EDGE('',*,*,#7510,.F.);
#9916=ORIENTED_EDGE('',*,*,#7511,.F.);
#9917=ORIENTED_EDGE('',*,*,#7512,.F.);
#9918=ORIENTED_EDGE('',*,*,#7506,.T.);
#9919=ORIENTED_EDGE('',*,*,#7513,.T.);
#9920=ORIENTED_EDGE('',*,*,#7514,.T.);
#9921=ORIENTED_EDGE('',*,*,#7515,.F.);
#9922=ORIENTED_EDGE('',*,*,#7516,.F.);
#9923=ORIENTED_EDGE('',*,*,#7510,.T.);
#9924=ORIENTED_EDGE('',*,*,#7517,.T.);
#9925=ORIENTED_EDGE('',*,*,#7518,.F.);
#9926=ORIENTED_EDGE('',*,*,#7519,.F.);
#9927=ORIENTED_EDGE('',*,*,#7520,.F.);
#9928=ORIENTED_EDGE('',*,*,#7515,.T.);
#9929=ORIENTED_EDGE('',*,*,#7521,.T.);
#9930=ORIENTED_EDGE('',*,*,#7522,.T.);
#9931=ORIENTED_EDGE('',*,*,#7523,.F.);
#9932=ORIENTED_EDGE('',*,*,#7524,.F.);
#9933=ORIENTED_EDGE('',*,*,#7518,.T.);
#9934=ORIENTED_EDGE('',*,*,#7525,.T.);
#9935=ORIENTED_EDGE('',*,*,#7526,.F.);
#9936=ORIENTED_EDGE('',*,*,#7527,.F.);
#9937=ORIENTED_EDGE('',*,*,#7528,.F.);
#9938=ORIENTED_EDGE('',*,*,#7523,.T.);
#9939=ORIENTED_EDGE('',*,*,#7529,.T.);
#9940=ORIENTED_EDGE('',*,*,#7530,.T.);
#9941=ORIENTED_EDGE('',*,*,#7531,.F.);
#9942=ORIENTED_EDGE('',*,*,#7532,.F.);
#9943=ORIENTED_EDGE('',*,*,#7526,.T.);
#9944=ORIENTED_EDGE('',*,*,#7533,.T.);
#9945=ORIENTED_EDGE('',*,*,#7534,.F.);
#9946=ORIENTED_EDGE('',*,*,#7535,.F.);
#9947=ORIENTED_EDGE('',*,*,#7536,.F.);
#9948=ORIENTED_EDGE('',*,*,#7531,.T.);
#9949=ORIENTED_EDGE('',*,*,#7537,.T.);
#9950=ORIENTED_EDGE('',*,*,#7538,.T.);
#9951=ORIENTED_EDGE('',*,*,#7539,.F.);
#9952=ORIENTED_EDGE('',*,*,#7540,.F.);
#9953=ORIENTED_EDGE('',*,*,#7534,.T.);
#9954=ORIENTED_EDGE('',*,*,#7541,.T.);
#9955=ORIENTED_EDGE('',*,*,#7542,.T.);
#9956=ORIENTED_EDGE('',*,*,#7543,.F.);
#9957=ORIENTED_EDGE('',*,*,#7544,.T.);
#9958=ORIENTED_EDGE('',*,*,#7545,.T.);
#9959=ORIENTED_EDGE('',*,*,#7546,.T.);
#9960=ORIENTED_EDGE('',*,*,#7547,.T.);
#9961=ORIENTED_EDGE('',*,*,#7548,.T.);
#9962=ORIENTED_EDGE('',*,*,#7549,.T.);
#9963=ORIENTED_EDGE('',*,*,#7550,.T.);
#9964=ORIENTED_EDGE('',*,*,#7551,.T.);
#9965=ORIENTED_EDGE('',*,*,#7552,.T.);
#9966=ORIENTED_EDGE('',*,*,#7553,.T.);
#9967=ORIENTED_EDGE('',*,*,#7554,.T.);
#9968=ORIENTED_EDGE('',*,*,#7555,.T.);
#9969=ORIENTED_EDGE('',*,*,#7556,.T.);
#9970=ORIENTED_EDGE('',*,*,#7557,.T.);
#9971=ORIENTED_EDGE('',*,*,#7558,.T.);
#9972=ORIENTED_EDGE('',*,*,#7559,.T.);
#9973=ORIENTED_EDGE('',*,*,#7560,.T.);
#9974=ORIENTED_EDGE('',*,*,#7561,.T.);
#9975=ORIENTED_EDGE('',*,*,#7562,.T.);
#9976=ORIENTED_EDGE('',*,*,#7563,.T.);
#9977=ORIENTED_EDGE('',*,*,#7564,.T.);
#9978=ORIENTED_EDGE('',*,*,#7565,.F.);
#9979=ORIENTED_EDGE('',*,*,#7566,.F.);
#9980=ORIENTED_EDGE('',*,*,#7567,.T.);
#9981=ORIENTED_EDGE('',*,*,#7568,.T.);
#9982=ORIENTED_EDGE('',*,*,#7569,.T.);
#9983=ORIENTED_EDGE('',*,*,#7570,.T.);
#9984=ORIENTED_EDGE('',*,*,#7571,.T.);
#9985=ORIENTED_EDGE('',*,*,#7572,.T.);
#9986=ORIENTED_EDGE('',*,*,#7573,.T.);
#9987=ORIENTED_EDGE('',*,*,#7574,.T.);
#9988=ORIENTED_EDGE('',*,*,#7575,.T.);
#9989=ORIENTED_EDGE('',*,*,#7576,.T.);
#9990=ORIENTED_EDGE('',*,*,#7577,.T.);
#9991=ORIENTED_EDGE('',*,*,#7578,.T.);
#9992=ORIENTED_EDGE('',*,*,#7579,.T.);
#9993=ORIENTED_EDGE('',*,*,#7580,.T.);
#9994=ORIENTED_EDGE('',*,*,#7581,.T.);
#9995=ORIENTED_EDGE('',*,*,#7582,.T.);
#9996=ORIENTED_EDGE('',*,*,#7583,.T.);
#9997=ORIENTED_EDGE('',*,*,#7584,.T.);
#9998=ORIENTED_EDGE('',*,*,#7585,.T.);
#9999=ORIENTED_EDGE('',*,*,#7539,.T.);
#10000=ORIENTED_EDGE('',*,*,#7586,.T.);
#10001=ORIENTED_EDGE('',*,*,#7587,.T.);
#10002=ORIENTED_EDGE('',*,*,#7588,.F.);
#10003=ORIENTED_EDGE('',*,*,#7589,.F.);
#10004=ORIENTED_EDGE('',*,*,#7590,.F.);
#10005=ORIENTED_EDGE('',*,*,#7591,.F.);
#10006=ORIENTED_EDGE('',*,*,#7592,.T.);
#10007=ORIENTED_EDGE('',*,*,#7588,.T.);
#10008=ORIENTED_EDGE('',*,*,#7593,.T.);
#10009=ORIENTED_EDGE('',*,*,#7592,.F.);
#10010=ORIENTED_EDGE('',*,*,#7594,.F.);
#10011=ORIENTED_EDGE('',*,*,#7564,.F.);
#10012=ORIENTED_EDGE('',*,*,#7563,.F.);
#10013=ORIENTED_EDGE('',*,*,#7562,.F.);
#10014=ORIENTED_EDGE('',*,*,#7561,.F.);
#10015=ORIENTED_EDGE('',*,*,#7560,.F.);
#10016=ORIENTED_EDGE('',*,*,#7559,.F.);
#10017=ORIENTED_EDGE('',*,*,#7558,.F.);
#10018=ORIENTED_EDGE('',*,*,#7557,.F.);
#10019=ORIENTED_EDGE('',*,*,#7556,.F.);
#10020=ORIENTED_EDGE('',*,*,#7555,.F.);
#10021=ORIENTED_EDGE('',*,*,#7554,.F.);
#10022=ORIENTED_EDGE('',*,*,#7553,.F.);
#10023=ORIENTED_EDGE('',*,*,#7552,.F.);
#10024=ORIENTED_EDGE('',*,*,#7551,.F.);
#10025=ORIENTED_EDGE('',*,*,#7550,.F.);
#10026=ORIENTED_EDGE('',*,*,#7549,.F.);
#10027=ORIENTED_EDGE('',*,*,#7548,.F.);
#10028=ORIENTED_EDGE('',*,*,#7547,.F.);
#10029=ORIENTED_EDGE('',*,*,#7546,.F.);
#10030=ORIENTED_EDGE('',*,*,#7545,.F.);
#10031=ORIENTED_EDGE('',*,*,#7544,.F.);
#10032=ORIENTED_EDGE('',*,*,#7595,.F.);
#10033=ORIENTED_EDGE('',*,*,#7465,.T.);
#10034=ORIENTED_EDGE('',*,*,#7470,.T.);
#10035=ORIENTED_EDGE('',*,*,#7469,.T.);
#10036=ORIENTED_EDGE('',*,*,#7474,.T.);
#10037=ORIENTED_EDGE('',*,*,#7478,.T.);
#10038=ORIENTED_EDGE('',*,*,#7477,.T.);
#10039=ORIENTED_EDGE('',*,*,#7482,.T.);
#10040=ORIENTED_EDGE('',*,*,#7486,.T.);
#10041=ORIENTED_EDGE('',*,*,#7485,.T.);
#10042=ORIENTED_EDGE('',*,*,#7490,.T.);
#10043=ORIENTED_EDGE('',*,*,#7494,.T.);
#10044=ORIENTED_EDGE('',*,*,#7493,.T.);
#10045=ORIENTED_EDGE('',*,*,#7498,.T.);
#10046=ORIENTED_EDGE('',*,*,#7503,.T.);
#10047=ORIENTED_EDGE('',*,*,#7502,.T.);
#10048=ORIENTED_EDGE('',*,*,#7508,.T.);
#10049=ORIENTED_EDGE('',*,*,#7507,.T.);
#10050=ORIENTED_EDGE('',*,*,#7512,.T.);
#10051=ORIENTED_EDGE('',*,*,#7511,.T.);
#10052=ORIENTED_EDGE('',*,*,#7516,.T.);
#10053=ORIENTED_EDGE('',*,*,#7520,.T.);
#10054=ORIENTED_EDGE('',*,*,#7519,.T.);
#10055=ORIENTED_EDGE('',*,*,#7524,.T.);
#10056=ORIENTED_EDGE('',*,*,#7528,.T.);
#10057=ORIENTED_EDGE('',*,*,#7527,.T.);
#10058=ORIENTED_EDGE('',*,*,#7532,.T.);
#10059=ORIENTED_EDGE('',*,*,#7536,.T.);
#10060=ORIENTED_EDGE('',*,*,#7535,.T.);
#10061=ORIENTED_EDGE('',*,*,#7540,.T.);
#10062=ORIENTED_EDGE('',*,*,#7590,.T.);
#10063=ORIENTED_EDGE('',*,*,#7589,.T.);
#10064=ORIENTED_EDGE('',*,*,#7596,.F.);
#10065=ORIENTED_EDGE('',*,*,#7597,.T.);
#10066=ORIENTED_EDGE('',*,*,#7466,.T.);
#10067=ORIENTED_EDGE('',*,*,#7595,.T.);
#10068=ORIENTED_EDGE('',*,*,#7598,.F.);
#10069=ORIENTED_EDGE('',*,*,#7593,.F.);
#10070=ORIENTED_EDGE('',*,*,#7587,.F.);
#10071=ORIENTED_EDGE('',*,*,#7586,.F.);
#10072=ORIENTED_EDGE('',*,*,#7541,.F.);
#10073=ORIENTED_EDGE('',*,*,#7538,.F.);
#10074=ORIENTED_EDGE('',*,*,#7537,.F.);
#10075=ORIENTED_EDGE('',*,*,#7533,.F.);
#10076=ORIENTED_EDGE('',*,*,#7530,.F.);
#10077=ORIENTED_EDGE('',*,*,#7529,.F.);
#10078=ORIENTED_EDGE('',*,*,#7525,.F.);
#10079=ORIENTED_EDGE('',*,*,#7522,.F.);
#10080=ORIENTED_EDGE('',*,*,#7521,.F.);
#10081=ORIENTED_EDGE('',*,*,#7517,.F.);
#10082=ORIENTED_EDGE('',*,*,#7514,.F.);
#10083=ORIENTED_EDGE('',*,*,#7513,.F.);
#10084=ORIENTED_EDGE('',*,*,#7509,.F.);
#10085=ORIENTED_EDGE('',*,*,#7505,.F.);
#10086=ORIENTED_EDGE('',*,*,#7504,.F.);
#10087=ORIENTED_EDGE('',*,*,#7500,.F.);
#10088=ORIENTED_EDGE('',*,*,#7499,.F.);
#10089=ORIENTED_EDGE('',*,*,#7496,.F.);
#10090=ORIENTED_EDGE('',*,*,#7495,.F.);
#10091=ORIENTED_EDGE('',*,*,#7491,.F.);
#10092=ORIENTED_EDGE('',*,*,#7488,.F.);
#10093=ORIENTED_EDGE('',*,*,#7487,.F.);
#10094=ORIENTED_EDGE('',*,*,#7483,.F.);
#10095=ORIENTED_EDGE('',*,*,#7480,.F.);
#10096=ORIENTED_EDGE('',*,*,#7479,.F.);
#10097=ORIENTED_EDGE('',*,*,#7475,.F.);
#10098=ORIENTED_EDGE('',*,*,#7472,.F.);
#10099=ORIENTED_EDGE('',*,*,#7471,.F.);
#10100=ORIENTED_EDGE('',*,*,#7467,.F.);
#10101=ORIENTED_EDGE('',*,*,#7597,.F.);
#10102=ORIENTED_EDGE('',*,*,#7599,.F.);
#10103=ORIENTED_EDGE('',*,*,#7542,.F.);
#10104=ORIENTED_EDGE('',*,*,#7585,.F.);
#10105=ORIENTED_EDGE('',*,*,#7584,.F.);
#10106=ORIENTED_EDGE('',*,*,#7583,.F.);
#10107=ORIENTED_EDGE('',*,*,#7582,.F.);
#10108=ORIENTED_EDGE('',*,*,#7581,.F.);
#10109=ORIENTED_EDGE('',*,*,#7580,.F.);
#10110=ORIENTED_EDGE('',*,*,#7579,.F.);
#10111=ORIENTED_EDGE('',*,*,#7578,.F.);
#10112=ORIENTED_EDGE('',*,*,#7577,.F.);
#10113=ORIENTED_EDGE('',*,*,#7576,.F.);
#10114=ORIENTED_EDGE('',*,*,#7575,.F.);
#10115=ORIENTED_EDGE('',*,*,#7574,.F.);
#10116=ORIENTED_EDGE('',*,*,#7573,.F.);
#10117=ORIENTED_EDGE('',*,*,#7572,.F.);
#10118=ORIENTED_EDGE('',*,*,#7571,.F.);
#10119=ORIENTED_EDGE('',*,*,#7570,.F.);
#10120=ORIENTED_EDGE('',*,*,#7569,.F.);
#10121=ORIENTED_EDGE('',*,*,#7568,.F.);
#10122=ORIENTED_EDGE('',*,*,#7567,.F.);
#10123=ORIENTED_EDGE('',*,*,#7600,.T.);
#10124=ORIENTED_EDGE('',*,*,#7601,.T.);
#10125=ORIENTED_EDGE('',*,*,#7598,.T.);
#10126=ORIENTED_EDGE('',*,*,#7543,.T.);
#10127=ORIENTED_EDGE('',*,*,#7599,.T.);
#10128=ORIENTED_EDGE('',*,*,#7596,.T.);
#10129=ORIENTED_EDGE('',*,*,#7601,.F.);
#10130=ORIENTED_EDGE('',*,*,#7602,.F.);
#10131=ORIENTED_EDGE('',*,*,#7600,.F.);
#10132=ORIENTED_EDGE('',*,*,#7566,.T.);
#10133=ORIENTED_EDGE('',*,*,#7603,.T.);
#10134=ORIENTED_EDGE('',*,*,#7604,.T.);
#10135=ORIENTED_EDGE('',*,*,#7603,.F.);
#10136=ORIENTED_EDGE('',*,*,#7565,.T.);
#10137=ORIENTED_EDGE('',*,*,#7594,.T.);
#10138=ORIENTED_EDGE('',*,*,#7591,.T.);
#10139=ORIENTED_EDGE('',*,*,#7604,.F.);
#10140=ORIENTED_EDGE('',*,*,#7605,.F.);
#10141=ORIENTED_EDGE('',*,*,#7606,.T.);
#10142=ORIENTED_EDGE('',*,*,#7607,.F.);
#10143=ORIENTED_EDGE('',*,*,#7608,.F.);
#10144=ORIENTED_EDGE('',*,*,#7609,.F.);
#10145=ORIENTED_EDGE('',*,*,#7610,.F.);
#10146=ORIENTED_EDGE('',*,*,#7607,.T.);
#10147=ORIENTED_EDGE('',*,*,#7611,.T.);
#10148=ORIENTED_EDGE('',*,*,#7612,.F.);
#10149=ORIENTED_EDGE('',*,*,#7611,.F.);
#10150=ORIENTED_EDGE('',*,*,#7606,.F.);
#10151=ORIENTED_EDGE('',*,*,#7613,.T.);
#10152=ORIENTED_EDGE('',*,*,#7614,.T.);
#10153=ORIENTED_EDGE('',*,*,#7615,.T.);
#10154=ORIENTED_EDGE('',*,*,#7616,.T.);
#10155=ORIENTED_EDGE('',*,*,#7617,.T.);
#10156=ORIENTED_EDGE('',*,*,#7618,.T.);
#10157=ORIENTED_EDGE('',*,*,#7619,.T.);
#10158=ORIENTED_EDGE('',*,*,#7620,.T.);
#10159=ORIENTED_EDGE('',*,*,#7621,.T.);
#10160=ORIENTED_EDGE('',*,*,#7622,.T.);
#10161=ORIENTED_EDGE('',*,*,#7623,.T.);
#10162=ORIENTED_EDGE('',*,*,#7624,.T.);
#10163=ORIENTED_EDGE('',*,*,#7625,.T.);
#10164=ORIENTED_EDGE('',*,*,#7626,.T.);
#10165=ORIENTED_EDGE('',*,*,#7627,.T.);
#10166=ORIENTED_EDGE('',*,*,#7628,.T.);
#10167=ORIENTED_EDGE('',*,*,#7629,.T.);
#10168=ORIENTED_EDGE('',*,*,#7630,.T.);
#10169=ORIENTED_EDGE('',*,*,#7631,.T.);
#10170=ORIENTED_EDGE('',*,*,#7632,.T.);
#10171=ORIENTED_EDGE('',*,*,#7633,.T.);
#10172=ORIENTED_EDGE('',*,*,#7634,.T.);
#10173=ORIENTED_EDGE('',*,*,#7635,.T.);
#10174=ORIENTED_EDGE('',*,*,#7636,.T.);
#10175=ORIENTED_EDGE('',*,*,#7637,.T.);
#10176=ORIENTED_EDGE('',*,*,#7638,.T.);
#10177=ORIENTED_EDGE('',*,*,#7639,.T.);
#10178=ORIENTED_EDGE('',*,*,#7640,.T.);
#10179=ORIENTED_EDGE('',*,*,#7641,.T.);
#10180=ORIENTED_EDGE('',*,*,#7642,.T.);
#10181=ORIENTED_EDGE('',*,*,#7643,.T.);
#10182=ORIENTED_EDGE('',*,*,#7644,.T.);
#10183=ORIENTED_EDGE('',*,*,#7645,.T.);
#10184=ORIENTED_EDGE('',*,*,#7646,.T.);
#10185=ORIENTED_EDGE('',*,*,#7647,.T.);
#10186=ORIENTED_EDGE('',*,*,#7648,.T.);
#10187=ORIENTED_EDGE('',*,*,#7649,.T.);
#10188=ORIENTED_EDGE('',*,*,#7650,.T.);
#10189=ORIENTED_EDGE('',*,*,#7651,.T.);
#10190=ORIENTED_EDGE('',*,*,#7652,.T.);
#10191=ORIENTED_EDGE('',*,*,#7653,.T.);
#10192=ORIENTED_EDGE('',*,*,#7654,.T.);
#10193=ORIENTED_EDGE('',*,*,#7655,.T.);
#10194=ORIENTED_EDGE('',*,*,#7656,.T.);
#10195=ORIENTED_EDGE('',*,*,#7657,.T.);
#10196=ORIENTED_EDGE('',*,*,#7658,.T.);
#10197=ORIENTED_EDGE('',*,*,#7659,.T.);
#10198=ORIENTED_EDGE('',*,*,#7660,.T.);
#10199=ORIENTED_EDGE('',*,*,#7661,.T.);
#10200=ORIENTED_EDGE('',*,*,#7662,.T.);
#10201=ORIENTED_EDGE('',*,*,#7663,.T.);
#10202=ORIENTED_EDGE('',*,*,#7664,.T.);
#10203=ORIENTED_EDGE('',*,*,#7665,.T.);
#10204=ORIENTED_EDGE('',*,*,#7666,.T.);
#10205=ORIENTED_EDGE('',*,*,#7667,.T.);
#10206=ORIENTED_EDGE('',*,*,#7668,.T.);
#10207=ORIENTED_EDGE('',*,*,#7608,.T.);
#10208=ORIENTED_EDGE('',*,*,#7610,.T.);
#10209=ORIENTED_EDGE('',*,*,#7669,.T.);
#10210=ORIENTED_EDGE('',*,*,#7670,.T.);
#10211=ORIENTED_EDGE('',*,*,#7671,.T.);
#10212=ORIENTED_EDGE('',*,*,#7672,.T.);
#10213=ORIENTED_EDGE('',*,*,#7673,.T.);
#10214=ORIENTED_EDGE('',*,*,#7674,.T.);
#10215=ORIENTED_EDGE('',*,*,#7675,.T.);
#10216=ORIENTED_EDGE('',*,*,#7676,.T.);
#10217=ORIENTED_EDGE('',*,*,#7677,.T.);
#10218=ORIENTED_EDGE('',*,*,#7678,.T.);
#10219=ORIENTED_EDGE('',*,*,#7679,.T.);
#10220=ORIENTED_EDGE('',*,*,#7680,.T.);
#10221=ORIENTED_EDGE('',*,*,#7681,.T.);
#10222=ORIENTED_EDGE('',*,*,#7682,.T.);
#10223=ORIENTED_EDGE('',*,*,#7683,.T.);
#10224=ORIENTED_EDGE('',*,*,#7684,.T.);
#10225=ORIENTED_EDGE('',*,*,#7685,.T.);
#10226=ORIENTED_EDGE('',*,*,#7686,.T.);
#10227=ORIENTED_EDGE('',*,*,#7687,.T.);
#10228=ORIENTED_EDGE('',*,*,#7688,.T.);
#10229=ORIENTED_EDGE('',*,*,#7689,.T.);
#10230=ORIENTED_EDGE('',*,*,#7690,.T.);
#10231=ORIENTED_EDGE('',*,*,#7691,.T.);
#10232=ORIENTED_EDGE('',*,*,#7692,.T.);
#10233=ORIENTED_EDGE('',*,*,#7693,.T.);
#10234=ORIENTED_EDGE('',*,*,#7694,.T.);
#10235=ORIENTED_EDGE('',*,*,#7695,.T.);
#10236=ORIENTED_EDGE('',*,*,#7696,.T.);
#10237=ORIENTED_EDGE('',*,*,#7697,.T.);
#10238=ORIENTED_EDGE('',*,*,#7698,.T.);
#10239=ORIENTED_EDGE('',*,*,#7699,.T.);
#10240=ORIENTED_EDGE('',*,*,#7700,.T.);
#10241=ORIENTED_EDGE('',*,*,#7701,.T.);
#10242=ORIENTED_EDGE('',*,*,#7702,.T.);
#10243=ORIENTED_EDGE('',*,*,#7703,.T.);
#10244=ORIENTED_EDGE('',*,*,#7704,.T.);
#10245=ORIENTED_EDGE('',*,*,#7705,.T.);
#10246=ORIENTED_EDGE('',*,*,#7706,.T.);
#10247=ORIENTED_EDGE('',*,*,#7707,.T.);
#10248=ORIENTED_EDGE('',*,*,#7708,.T.);
#10249=ORIENTED_EDGE('',*,*,#7709,.T.);
#10250=ORIENTED_EDGE('',*,*,#7710,.T.);
#10251=ORIENTED_EDGE('',*,*,#7711,.T.);
#10252=ORIENTED_EDGE('',*,*,#7712,.T.);
#10253=ORIENTED_EDGE('',*,*,#7713,.T.);
#10254=ORIENTED_EDGE('',*,*,#7714,.T.);
#10255=ORIENTED_EDGE('',*,*,#7715,.T.);
#10256=ORIENTED_EDGE('',*,*,#7716,.T.);
#10257=ORIENTED_EDGE('',*,*,#7717,.T.);
#10258=ORIENTED_EDGE('',*,*,#7718,.T.);
#10259=ORIENTED_EDGE('',*,*,#7719,.T.);
#10260=ORIENTED_EDGE('',*,*,#7720,.T.);
#10261=ORIENTED_EDGE('',*,*,#7719,.F.);
#10262=ORIENTED_EDGE('',*,*,#7721,.F.);
#10263=ORIENTED_EDGE('',*,*,#7722,.T.);
#10264=ORIENTED_EDGE('',*,*,#7723,.F.);
#10265=ORIENTED_EDGE('',*,*,#7670,.F.);
#10266=ORIENTED_EDGE('',*,*,#7724,.F.);
#10267=ORIENTED_EDGE('',*,*,#7671,.F.);
#10268=ORIENTED_EDGE('',*,*,#7723,.T.);
#10269=ORIENTED_EDGE('',*,*,#7725,.T.);
#10270=ORIENTED_EDGE('',*,*,#7726,.F.);
#10271=ORIENTED_EDGE('',*,*,#7725,.F.);
#10272=ORIENTED_EDGE('',*,*,#7722,.F.);
#10273=ORIENTED_EDGE('',*,*,#7727,.F.);
#10274=ORIENTED_EDGE('',*,*,#7728,.T.);
#10275=ORIENTED_EDGE('',*,*,#7729,.F.);
#10276=ORIENTED_EDGE('',*,*,#7673,.F.);
#10277=ORIENTED_EDGE('',*,*,#7730,.F.);
#10278=ORIENTED_EDGE('',*,*,#7674,.F.);
#10279=ORIENTED_EDGE('',*,*,#7729,.T.);
#10280=ORIENTED_EDGE('',*,*,#7731,.T.);
#10281=ORIENTED_EDGE('',*,*,#7732,.F.);
#10282=ORIENTED_EDGE('',*,*,#7731,.F.);
#10283=ORIENTED_EDGE('',*,*,#7728,.F.);
#10284=ORIENTED_EDGE('',*,*,#7733,.F.);
#10285=ORIENTED_EDGE('',*,*,#7734,.T.);
#10286=ORIENTED_EDGE('',*,*,#7735,.F.);
#10287=ORIENTED_EDGE('',*,*,#7676,.F.);
#10288=ORIENTED_EDGE('',*,*,#7736,.F.);
#10289=ORIENTED_EDGE('',*,*,#7677,.F.);
#10290=ORIENTED_EDGE('',*,*,#7735,.T.);
#10291=ORIENTED_EDGE('',*,*,#7737,.T.);
#10292=ORIENTED_EDGE('',*,*,#7738,.F.);
#10293=ORIENTED_EDGE('',*,*,#7737,.F.);
#10294=ORIENTED_EDGE('',*,*,#7734,.F.);
#10295=ORIENTED_EDGE('',*,*,#7739,.F.);
#10296=ORIENTED_EDGE('',*,*,#7740,.T.);
#10297=ORIENTED_EDGE('',*,*,#7741,.F.);
#10298=ORIENTED_EDGE('',*,*,#7679,.F.);
#10299=ORIENTED_EDGE('',*,*,#7742,.F.);
#10300=ORIENTED_EDGE('',*,*,#7680,.F.);
#10301=ORIENTED_EDGE('',*,*,#7741,.T.);
#10302=ORIENTED_EDGE('',*,*,#7743,.T.);
#10303=ORIENTED_EDGE('',*,*,#7744,.F.);
#10304=ORIENTED_EDGE('',*,*,#7743,.F.);
#10305=ORIENTED_EDGE('',*,*,#7740,.F.);
#10306=ORIENTED_EDGE('',*,*,#7745,.F.);
#10307=ORIENTED_EDGE('',*,*,#7746,.T.);
#10308=ORIENTED_EDGE('',*,*,#7747,.F.);
#10309=ORIENTED_EDGE('',*,*,#7682,.F.);
#10310=ORIENTED_EDGE('',*,*,#7748,.F.);
#10311=ORIENTED_EDGE('',*,*,#7683,.F.);
#10312=ORIENTED_EDGE('',*,*,#7747,.T.);
#10313=ORIENTED_EDGE('',*,*,#7749,.T.);
#10314=ORIENTED_EDGE('',*,*,#7750,.F.);
#10315=ORIENTED_EDGE('',*,*,#7749,.F.);
#10316=ORIENTED_EDGE('',*,*,#7746,.F.);
#10317=ORIENTED_EDGE('',*,*,#7751,.F.);
#10318=ORIENTED_EDGE('',*,*,#7752,.T.);
#10319=ORIENTED_EDGE('',*,*,#7753,.F.);
#10320=ORIENTED_EDGE('',*,*,#7685,.F.);
#10321=ORIENTED_EDGE('',*,*,#7754,.F.);
#10322=ORIENTED_EDGE('',*,*,#7686,.F.);
#10323=ORIENTED_EDGE('',*,*,#7753,.T.);
#10324=ORIENTED_EDGE('',*,*,#7755,.T.);
#10325=ORIENTED_EDGE('',*,*,#7756,.F.);
#10326=ORIENTED_EDGE('',*,*,#7755,.F.);
#10327=ORIENTED_EDGE('',*,*,#7752,.F.);
#10328=ORIENTED_EDGE('',*,*,#7757,.F.);
#10329=ORIENTED_EDGE('',*,*,#7758,.T.);
#10330=ORIENTED_EDGE('',*,*,#7759,.F.);
#10331=ORIENTED_EDGE('',*,*,#7688,.F.);
#10332=ORIENTED_EDGE('',*,*,#7760,.F.);
#10333=ORIENTED_EDGE('',*,*,#7689,.F.);
#10334=ORIENTED_EDGE('',*,*,#7759,.T.);
#10335=ORIENTED_EDGE('',*,*,#7761,.T.);
#10336=ORIENTED_EDGE('',*,*,#7762,.F.);
#10337=ORIENTED_EDGE('',*,*,#7761,.F.);
#10338=ORIENTED_EDGE('',*,*,#7758,.F.);
#10339=ORIENTED_EDGE('',*,*,#7763,.F.);
#10340=ORIENTED_EDGE('',*,*,#7764,.T.);
#10341=ORIENTED_EDGE('',*,*,#7765,.F.);
#10342=ORIENTED_EDGE('',*,*,#7691,.F.);
#10343=ORIENTED_EDGE('',*,*,#7766,.F.);
#10344=ORIENTED_EDGE('',*,*,#7692,.F.);
#10345=ORIENTED_EDGE('',*,*,#7765,.T.);
#10346=ORIENTED_EDGE('',*,*,#7767,.T.);
#10347=ORIENTED_EDGE('',*,*,#7768,.F.);
#10348=ORIENTED_EDGE('',*,*,#7767,.F.);
#10349=ORIENTED_EDGE('',*,*,#7764,.F.);
#10350=ORIENTED_EDGE('',*,*,#7769,.F.);
#10351=ORIENTED_EDGE('',*,*,#7770,.T.);
#10352=ORIENTED_EDGE('',*,*,#7771,.F.);
#10353=ORIENTED_EDGE('',*,*,#7694,.F.);
#10354=ORIENTED_EDGE('',*,*,#7772,.F.);
#10355=ORIENTED_EDGE('',*,*,#7695,.F.);
#10356=ORIENTED_EDGE('',*,*,#7771,.T.);
#10357=ORIENTED_EDGE('',*,*,#7773,.T.);
#10358=ORIENTED_EDGE('',*,*,#7774,.F.);
#10359=ORIENTED_EDGE('',*,*,#7773,.F.);
#10360=ORIENTED_EDGE('',*,*,#7770,.F.);
#10361=ORIENTED_EDGE('',*,*,#7775,.F.);
#10362=ORIENTED_EDGE('',*,*,#7776,.T.);
#10363=ORIENTED_EDGE('',*,*,#7777,.F.);
#10364=ORIENTED_EDGE('',*,*,#7697,.F.);
#10365=ORIENTED_EDGE('',*,*,#7778,.F.);
#10366=ORIENTED_EDGE('',*,*,#7698,.F.);
#10367=ORIENTED_EDGE('',*,*,#7777,.T.);
#10368=ORIENTED_EDGE('',*,*,#7779,.T.);
#10369=ORIENTED_EDGE('',*,*,#7780,.F.);
#10370=ORIENTED_EDGE('',*,*,#7779,.F.);
#10371=ORIENTED_EDGE('',*,*,#7776,.F.);
#10372=ORIENTED_EDGE('',*,*,#7781,.F.);
#10373=ORIENTED_EDGE('',*,*,#7782,.T.);
#10374=ORIENTED_EDGE('',*,*,#7783,.F.);
#10375=ORIENTED_EDGE('',*,*,#7700,.F.);
#10376=ORIENTED_EDGE('',*,*,#7784,.F.);
#10377=ORIENTED_EDGE('',*,*,#7701,.F.);
#10378=ORIENTED_EDGE('',*,*,#7783,.T.);
#10379=ORIENTED_EDGE('',*,*,#7785,.T.);
#10380=ORIENTED_EDGE('',*,*,#7786,.F.);
#10381=ORIENTED_EDGE('',*,*,#7785,.F.);
#10382=ORIENTED_EDGE('',*,*,#7782,.F.);
#10383=ORIENTED_EDGE('',*,*,#7787,.F.);
#10384=ORIENTED_EDGE('',*,*,#7788,.T.);
#10385=ORIENTED_EDGE('',*,*,#7789,.F.);
#10386=ORIENTED_EDGE('',*,*,#7703,.F.);
#10387=ORIENTED_EDGE('',*,*,#7790,.F.);
#10388=ORIENTED_EDGE('',*,*,#7704,.F.);
#10389=ORIENTED_EDGE('',*,*,#7789,.T.);
#10390=ORIENTED_EDGE('',*,*,#7791,.T.);
#10391=ORIENTED_EDGE('',*,*,#7792,.F.);
#10392=ORIENTED_EDGE('',*,*,#7791,.F.);
#10393=ORIENTED_EDGE('',*,*,#7788,.F.);
#10394=ORIENTED_EDGE('',*,*,#7793,.F.);
#10395=ORIENTED_EDGE('',*,*,#7794,.T.);
#10396=ORIENTED_EDGE('',*,*,#7795,.F.);
#10397=ORIENTED_EDGE('',*,*,#7706,.F.);
#10398=ORIENTED_EDGE('',*,*,#7796,.F.);
#10399=ORIENTED_EDGE('',*,*,#7707,.F.);
#10400=ORIENTED_EDGE('',*,*,#7795,.T.);
#10401=ORIENTED_EDGE('',*,*,#7797,.T.);
#10402=ORIENTED_EDGE('',*,*,#7798,.F.);
#10403=ORIENTED_EDGE('',*,*,#7797,.F.);
#10404=ORIENTED_EDGE('',*,*,#7794,.F.);
#10405=ORIENTED_EDGE('',*,*,#7799,.F.);
#10406=ORIENTED_EDGE('',*,*,#7800,.T.);
#10407=ORIENTED_EDGE('',*,*,#7801,.F.);
#10408=ORIENTED_EDGE('',*,*,#7709,.F.);
#10409=ORIENTED_EDGE('',*,*,#7802,.F.);
#10410=ORIENTED_EDGE('',*,*,#7710,.F.);
#10411=ORIENTED_EDGE('',*,*,#7801,.T.);
#10412=ORIENTED_EDGE('',*,*,#7803,.T.);
#10413=ORIENTED_EDGE('',*,*,#7804,.F.);
#10414=ORIENTED_EDGE('',*,*,#7803,.F.);
#10415=ORIENTED_EDGE('',*,*,#7800,.F.);
#10416=ORIENTED_EDGE('',*,*,#7805,.F.);
#10417=ORIENTED_EDGE('',*,*,#7806,.T.);
#10418=ORIENTED_EDGE('',*,*,#7807,.F.);
#10419=ORIENTED_EDGE('',*,*,#7712,.F.);
#10420=ORIENTED_EDGE('',*,*,#7808,.F.);
#10421=ORIENTED_EDGE('',*,*,#7713,.F.);
#10422=ORIENTED_EDGE('',*,*,#7807,.T.);
#10423=ORIENTED_EDGE('',*,*,#7809,.T.);
#10424=ORIENTED_EDGE('',*,*,#7810,.F.);
#10425=ORIENTED_EDGE('',*,*,#7809,.F.);
#10426=ORIENTED_EDGE('',*,*,#7806,.F.);
#10427=ORIENTED_EDGE('',*,*,#7811,.F.);
#10428=ORIENTED_EDGE('',*,*,#7812,.T.);
#10429=ORIENTED_EDGE('',*,*,#7813,.F.);
#10430=ORIENTED_EDGE('',*,*,#7715,.F.);
#10431=ORIENTED_EDGE('',*,*,#7814,.F.);
#10432=ORIENTED_EDGE('',*,*,#7716,.F.);
#10433=ORIENTED_EDGE('',*,*,#7813,.T.);
#10434=ORIENTED_EDGE('',*,*,#7815,.T.);
#10435=ORIENTED_EDGE('',*,*,#7816,.F.);
#10436=ORIENTED_EDGE('',*,*,#7815,.F.);
#10437=ORIENTED_EDGE('',*,*,#7812,.F.);
#10438=ORIENTED_EDGE('',*,*,#7817,.F.);
#10439=ORIENTED_EDGE('',*,*,#7818,.T.);
#10440=ORIENTED_EDGE('',*,*,#7819,.F.);
#10441=ORIENTED_EDGE('',*,*,#7718,.F.);
#10442=ORIENTED_EDGE('',*,*,#7820,.F.);
#10443=ORIENTED_EDGE('',*,*,#7613,.F.);
#10444=ORIENTED_EDGE('',*,*,#7819,.T.);
#10445=ORIENTED_EDGE('',*,*,#7821,.T.);
#10446=ORIENTED_EDGE('',*,*,#7822,.F.);
#10447=ORIENTED_EDGE('',*,*,#7821,.F.);
#10448=ORIENTED_EDGE('',*,*,#7818,.F.);
#10449=ORIENTED_EDGE('',*,*,#7823,.F.);
#10450=ORIENTED_EDGE('',*,*,#7824,.F.);
#10451=ORIENTED_EDGE('',*,*,#7825,.T.);
#10452=ORIENTED_EDGE('',*,*,#7826,.F.);
#10453=ORIENTED_EDGE('',*,*,#7615,.F.);
#10454=ORIENTED_EDGE('',*,*,#7827,.F.);
#10455=ORIENTED_EDGE('',*,*,#7616,.F.);
#10456=ORIENTED_EDGE('',*,*,#7826,.T.);
#10457=ORIENTED_EDGE('',*,*,#7828,.T.);
#10458=ORIENTED_EDGE('',*,*,#7829,.F.);
#10459=ORIENTED_EDGE('',*,*,#7828,.F.);
#10460=ORIENTED_EDGE('',*,*,#7825,.F.);
#10461=ORIENTED_EDGE('',*,*,#7830,.F.);
#10462=ORIENTED_EDGE('',*,*,#7831,.T.);
#10463=ORIENTED_EDGE('',*,*,#7832,.F.);
#10464=ORIENTED_EDGE('',*,*,#7618,.F.);
#10465=ORIENTED_EDGE('',*,*,#7833,.F.);
#10466=ORIENTED_EDGE('',*,*,#7619,.F.);
#10467=ORIENTED_EDGE('',*,*,#7832,.T.);
#10468=ORIENTED_EDGE('',*,*,#7834,.T.);
#10469=ORIENTED_EDGE('',*,*,#7835,.F.);
#10470=ORIENTED_EDGE('',*,*,#7834,.F.);
#10471=ORIENTED_EDGE('',*,*,#7831,.F.);
#10472=ORIENTED_EDGE('',*,*,#7836,.F.);
#10473=ORIENTED_EDGE('',*,*,#7837,.T.);
#10474=ORIENTED_EDGE('',*,*,#7838,.F.);
#10475=ORIENTED_EDGE('',*,*,#7621,.F.);
#10476=ORIENTED_EDGE('',*,*,#7839,.F.);
#10477=ORIENTED_EDGE('',*,*,#7622,.F.);
#10478=ORIENTED_EDGE('',*,*,#7838,.T.);
#10479=ORIENTED_EDGE('',*,*,#7840,.T.);
#10480=ORIENTED_EDGE('',*,*,#7841,.F.);
#10481=ORIENTED_EDGE('',*,*,#7840,.F.);
#10482=ORIENTED_EDGE('',*,*,#7837,.F.);
#10483=ORIENTED_EDGE('',*,*,#7842,.F.);
#10484=ORIENTED_EDGE('',*,*,#7843,.T.);
#10485=ORIENTED_EDGE('',*,*,#7844,.F.);
#10486=ORIENTED_EDGE('',*,*,#7624,.F.);
#10487=ORIENTED_EDGE('',*,*,#7845,.F.);
#10488=ORIENTED_EDGE('',*,*,#7625,.F.);
#10489=ORIENTED_EDGE('',*,*,#7844,.T.);
#10490=ORIENTED_EDGE('',*,*,#7846,.T.);
#10491=ORIENTED_EDGE('',*,*,#7847,.F.);
#10492=ORIENTED_EDGE('',*,*,#7846,.F.);
#10493=ORIENTED_EDGE('',*,*,#7843,.F.);
#10494=ORIENTED_EDGE('',*,*,#7848,.F.);
#10495=ORIENTED_EDGE('',*,*,#7849,.T.);
#10496=ORIENTED_EDGE('',*,*,#7850,.F.);
#10497=ORIENTED_EDGE('',*,*,#7627,.F.);
#10498=ORIENTED_EDGE('',*,*,#7851,.F.);
#10499=ORIENTED_EDGE('',*,*,#7628,.F.);
#10500=ORIENTED_EDGE('',*,*,#7850,.T.);
#10501=ORIENTED_EDGE('',*,*,#7852,.T.);
#10502=ORIENTED_EDGE('',*,*,#7853,.F.);
#10503=ORIENTED_EDGE('',*,*,#7852,.F.);
#10504=ORIENTED_EDGE('',*,*,#7849,.F.);
#10505=ORIENTED_EDGE('',*,*,#7854,.F.);
#10506=ORIENTED_EDGE('',*,*,#7855,.T.);
#10507=ORIENTED_EDGE('',*,*,#7856,.F.);
#10508=ORIENTED_EDGE('',*,*,#7630,.F.);
#10509=ORIENTED_EDGE('',*,*,#7857,.F.);
#10510=ORIENTED_EDGE('',*,*,#7631,.F.);
#10511=ORIENTED_EDGE('',*,*,#7856,.T.);
#10512=ORIENTED_EDGE('',*,*,#7858,.T.);
#10513=ORIENTED_EDGE('',*,*,#7859,.F.);
#10514=ORIENTED_EDGE('',*,*,#7858,.F.);
#10515=ORIENTED_EDGE('',*,*,#7855,.F.);
#10516=ORIENTED_EDGE('',*,*,#7860,.F.);
#10517=ORIENTED_EDGE('',*,*,#7861,.T.);
#10518=ORIENTED_EDGE('',*,*,#7862,.F.);
#10519=ORIENTED_EDGE('',*,*,#7633,.F.);
#10520=ORIENTED_EDGE('',*,*,#7863,.F.);
#10521=ORIENTED_EDGE('',*,*,#7634,.F.);
#10522=ORIENTED_EDGE('',*,*,#7862,.T.);
#10523=ORIENTED_EDGE('',*,*,#7864,.T.);
#10524=ORIENTED_EDGE('',*,*,#7865,.F.);
#10525=ORIENTED_EDGE('',*,*,#7864,.F.);
#10526=ORIENTED_EDGE('',*,*,#7861,.F.);
#10527=ORIENTED_EDGE('',*,*,#7866,.F.);
#10528=ORIENTED_EDGE('',*,*,#7867,.T.);
#10529=ORIENTED_EDGE('',*,*,#7868,.F.);
#10530=ORIENTED_EDGE('',*,*,#7636,.F.);
#10531=ORIENTED_EDGE('',*,*,#7869,.F.);
#10532=ORIENTED_EDGE('',*,*,#7637,.F.);
#10533=ORIENTED_EDGE('',*,*,#7868,.T.);
#10534=ORIENTED_EDGE('',*,*,#7870,.T.);
#10535=ORIENTED_EDGE('',*,*,#7871,.F.);
#10536=ORIENTED_EDGE('',*,*,#7870,.F.);
#10537=ORIENTED_EDGE('',*,*,#7867,.F.);
#10538=ORIENTED_EDGE('',*,*,#7872,.F.);
#10539=ORIENTED_EDGE('',*,*,#7873,.T.);
#10540=ORIENTED_EDGE('',*,*,#7874,.F.);
#10541=ORIENTED_EDGE('',*,*,#7639,.F.);
#10542=ORIENTED_EDGE('',*,*,#7875,.F.);
#10543=ORIENTED_EDGE('',*,*,#7640,.F.);
#10544=ORIENTED_EDGE('',*,*,#7874,.T.);
#10545=ORIENTED_EDGE('',*,*,#7876,.T.);
#10546=ORIENTED_EDGE('',*,*,#7877,.F.);
#10547=ORIENTED_EDGE('',*,*,#7876,.F.);
#10548=ORIENTED_EDGE('',*,*,#7873,.F.);
#10549=ORIENTED_EDGE('',*,*,#7878,.F.);
#10550=ORIENTED_EDGE('',*,*,#7879,.T.);
#10551=ORIENTED_EDGE('',*,*,#7880,.F.);
#10552=ORIENTED_EDGE('',*,*,#7642,.F.);
#10553=ORIENTED_EDGE('',*,*,#7881,.F.);
#10554=ORIENTED_EDGE('',*,*,#7643,.F.);
#10555=ORIENTED_EDGE('',*,*,#7880,.T.);
#10556=ORIENTED_EDGE('',*,*,#7882,.T.);
#10557=ORIENTED_EDGE('',*,*,#7883,.F.);
#10558=ORIENTED_EDGE('',*,*,#7882,.F.);
#10559=ORIENTED_EDGE('',*,*,#7879,.F.);
#10560=ORIENTED_EDGE('',*,*,#7884,.F.);
#10561=ORIENTED_EDGE('',*,*,#7885,.T.);
#10562=ORIENTED_EDGE('',*,*,#7886,.F.);
#10563=ORIENTED_EDGE('',*,*,#7645,.F.);
#10564=ORIENTED_EDGE('',*,*,#7887,.F.);
#10565=ORIENTED_EDGE('',*,*,#7646,.F.);
#10566=ORIENTED_EDGE('',*,*,#7886,.T.);
#10567=ORIENTED_EDGE('',*,*,#7888,.T.);
#10568=ORIENTED_EDGE('',*,*,#7889,.F.);
#10569=ORIENTED_EDGE('',*,*,#7888,.F.);
#10570=ORIENTED_EDGE('',*,*,#7885,.F.);
#10571=ORIENTED_EDGE('',*,*,#7890,.F.);
#10572=ORIENTED_EDGE('',*,*,#7891,.T.);
#10573=ORIENTED_EDGE('',*,*,#7892,.F.);
#10574=ORIENTED_EDGE('',*,*,#7648,.F.);
#10575=ORIENTED_EDGE('',*,*,#7893,.F.);
#10576=ORIENTED_EDGE('',*,*,#7649,.F.);
#10577=ORIENTED_EDGE('',*,*,#7892,.T.);
#10578=ORIENTED_EDGE('',*,*,#7894,.T.);
#10579=ORIENTED_EDGE('',*,*,#7895,.F.);
#10580=ORIENTED_EDGE('',*,*,#7894,.F.);
#10581=ORIENTED_EDGE('',*,*,#7891,.F.);
#10582=ORIENTED_EDGE('',*,*,#7896,.F.);
#10583=ORIENTED_EDGE('',*,*,#7897,.T.);
#10584=ORIENTED_EDGE('',*,*,#7898,.F.);
#10585=ORIENTED_EDGE('',*,*,#7651,.F.);
#10586=ORIENTED_EDGE('',*,*,#7899,.F.);
#10587=ORIENTED_EDGE('',*,*,#7652,.F.);
#10588=ORIENTED_EDGE('',*,*,#7898,.T.);
#10589=ORIENTED_EDGE('',*,*,#7900,.T.);
#10590=ORIENTED_EDGE('',*,*,#7901,.F.);
#10591=ORIENTED_EDGE('',*,*,#7900,.F.);
#10592=ORIENTED_EDGE('',*,*,#7897,.F.);
#10593=ORIENTED_EDGE('',*,*,#7902,.F.);
#10594=ORIENTED_EDGE('',*,*,#7903,.T.);
#10595=ORIENTED_EDGE('',*,*,#7904,.F.);
#10596=ORIENTED_EDGE('',*,*,#7654,.F.);
#10597=ORIENTED_EDGE('',*,*,#7905,.F.);
#10598=ORIENTED_EDGE('',*,*,#7655,.F.);
#10599=ORIENTED_EDGE('',*,*,#7904,.T.);
#10600=ORIENTED_EDGE('',*,*,#7906,.T.);
#10601=ORIENTED_EDGE('',*,*,#7907,.F.);
#10602=ORIENTED_EDGE('',*,*,#7906,.F.);
#10603=ORIENTED_EDGE('',*,*,#7903,.F.);
#10604=ORIENTED_EDGE('',*,*,#7908,.F.);
#10605=ORIENTED_EDGE('',*,*,#7909,.T.);
#10606=ORIENTED_EDGE('',*,*,#7910,.F.);
#10607=ORIENTED_EDGE('',*,*,#7657,.F.);
#10608=ORIENTED_EDGE('',*,*,#7911,.F.);
#10609=ORIENTED_EDGE('',*,*,#7658,.F.);
#10610=ORIENTED_EDGE('',*,*,#7910,.T.);
#10611=ORIENTED_EDGE('',*,*,#7912,.T.);
#10612=ORIENTED_EDGE('',*,*,#7913,.F.);
#10613=ORIENTED_EDGE('',*,*,#7912,.F.);
#10614=ORIENTED_EDGE('',*,*,#7909,.F.);
#10615=ORIENTED_EDGE('',*,*,#7914,.F.);
#10616=ORIENTED_EDGE('',*,*,#7915,.T.);
#10617=ORIENTED_EDGE('',*,*,#7916,.F.);
#10618=ORIENTED_EDGE('',*,*,#7660,.F.);
#10619=ORIENTED_EDGE('',*,*,#7917,.F.);
#10620=ORIENTED_EDGE('',*,*,#7661,.F.);
#10621=ORIENTED_EDGE('',*,*,#7916,.T.);
#10622=ORIENTED_EDGE('',*,*,#7918,.T.);
#10623=ORIENTED_EDGE('',*,*,#7919,.F.);
#10624=ORIENTED_EDGE('',*,*,#7918,.F.);
#10625=ORIENTED_EDGE('',*,*,#7915,.F.);
#10626=ORIENTED_EDGE('',*,*,#7920,.F.);
#10627=ORIENTED_EDGE('',*,*,#7921,.T.);
#10628=ORIENTED_EDGE('',*,*,#7922,.F.);
#10629=ORIENTED_EDGE('',*,*,#7663,.F.);
#10630=ORIENTED_EDGE('',*,*,#7923,.F.);
#10631=ORIENTED_EDGE('',*,*,#7664,.F.);
#10632=ORIENTED_EDGE('',*,*,#7922,.T.);
#10633=ORIENTED_EDGE('',*,*,#7924,.T.);
#10634=ORIENTED_EDGE('',*,*,#7925,.F.);
#10635=ORIENTED_EDGE('',*,*,#7924,.F.);
#10636=ORIENTED_EDGE('',*,*,#7921,.F.);
#10637=ORIENTED_EDGE('',*,*,#7926,.F.);
#10638=ORIENTED_EDGE('',*,*,#7927,.T.);
#10639=ORIENTED_EDGE('',*,*,#7928,.F.);
#10640=ORIENTED_EDGE('',*,*,#7666,.F.);
#10641=ORIENTED_EDGE('',*,*,#7929,.F.);
#10642=ORIENTED_EDGE('',*,*,#7667,.F.);
#10643=ORIENTED_EDGE('',*,*,#7928,.T.);
#10644=ORIENTED_EDGE('',*,*,#7930,.T.);
#10645=ORIENTED_EDGE('',*,*,#7931,.F.);
#10646=ORIENTED_EDGE('',*,*,#7930,.F.);
#10647=ORIENTED_EDGE('',*,*,#7927,.F.);
#10648=ORIENTED_EDGE('',*,*,#7822,.T.);
#10649=ORIENTED_EDGE('',*,*,#7932,.T.);
#10650=ORIENTED_EDGE('',*,*,#7602,.T.);
#10651=ORIENTED_EDGE('',*,*,#7932,.F.);
#10652=ORIENTED_EDGE('',*,*,#7823,.T.);
#10653=ORIENTED_EDGE('',*,*,#7817,.T.);
#10654=ORIENTED_EDGE('',*,*,#7717,.F.);
#10655=ORIENTED_EDGE('',*,*,#7814,.T.);
#10656=ORIENTED_EDGE('',*,*,#7816,.T.);
#10657=ORIENTED_EDGE('',*,*,#7811,.T.);
#10658=ORIENTED_EDGE('',*,*,#7714,.F.);
#10659=ORIENTED_EDGE('',*,*,#7808,.T.);
#10660=ORIENTED_EDGE('',*,*,#7810,.T.);
#10661=ORIENTED_EDGE('',*,*,#7805,.T.);
#10662=ORIENTED_EDGE('',*,*,#7711,.F.);
#10663=ORIENTED_EDGE('',*,*,#7802,.T.);
#10664=ORIENTED_EDGE('',*,*,#7804,.T.);
#10665=ORIENTED_EDGE('',*,*,#7799,.T.);
#10666=ORIENTED_EDGE('',*,*,#7708,.F.);
#10667=ORIENTED_EDGE('',*,*,#7796,.T.);
#10668=ORIENTED_EDGE('',*,*,#7798,.T.);
#10669=ORIENTED_EDGE('',*,*,#7793,.T.);
#10670=ORIENTED_EDGE('',*,*,#7705,.F.);
#10671=ORIENTED_EDGE('',*,*,#7790,.T.);
#10672=ORIENTED_EDGE('',*,*,#7792,.T.);
#10673=ORIENTED_EDGE('',*,*,#7787,.T.);
#10674=ORIENTED_EDGE('',*,*,#7702,.F.);
#10675=ORIENTED_EDGE('',*,*,#7784,.T.);
#10676=ORIENTED_EDGE('',*,*,#7786,.T.);
#10677=ORIENTED_EDGE('',*,*,#7781,.T.);
#10678=ORIENTED_EDGE('',*,*,#7699,.F.);
#10679=ORIENTED_EDGE('',*,*,#7778,.T.);
#10680=ORIENTED_EDGE('',*,*,#7780,.T.);
#10681=ORIENTED_EDGE('',*,*,#7775,.T.);
#10682=ORIENTED_EDGE('',*,*,#7696,.F.);
#10683=ORIENTED_EDGE('',*,*,#7772,.T.);
#10684=ORIENTED_EDGE('',*,*,#7774,.T.);
#10685=ORIENTED_EDGE('',*,*,#7769,.T.);
#10686=ORIENTED_EDGE('',*,*,#7693,.F.);
#10687=ORIENTED_EDGE('',*,*,#7766,.T.);
#10688=ORIENTED_EDGE('',*,*,#7768,.T.);
#10689=ORIENTED_EDGE('',*,*,#7763,.T.);
#10690=ORIENTED_EDGE('',*,*,#7690,.F.);
#10691=ORIENTED_EDGE('',*,*,#7760,.T.);
#10692=ORIENTED_EDGE('',*,*,#7762,.T.);
#10693=ORIENTED_EDGE('',*,*,#7757,.T.);
#10694=ORIENTED_EDGE('',*,*,#7687,.F.);
#10695=ORIENTED_EDGE('',*,*,#7754,.T.);
#10696=ORIENTED_EDGE('',*,*,#7756,.T.);
#10697=ORIENTED_EDGE('',*,*,#7751,.T.);
#10698=ORIENTED_EDGE('',*,*,#7684,.F.);
#10699=ORIENTED_EDGE('',*,*,#7748,.T.);
#10700=ORIENTED_EDGE('',*,*,#7750,.T.);
#10701=ORIENTED_EDGE('',*,*,#7745,.T.);
#10702=ORIENTED_EDGE('',*,*,#7681,.F.);
#10703=ORIENTED_EDGE('',*,*,#7742,.T.);
#10704=ORIENTED_EDGE('',*,*,#7744,.T.);
#10705=ORIENTED_EDGE('',*,*,#7739,.T.);
#10706=ORIENTED_EDGE('',*,*,#7678,.F.);
#10707=ORIENTED_EDGE('',*,*,#7736,.T.);
#10708=ORIENTED_EDGE('',*,*,#7738,.T.);
#10709=ORIENTED_EDGE('',*,*,#7733,.T.);
#10710=ORIENTED_EDGE('',*,*,#7675,.F.);
#10711=ORIENTED_EDGE('',*,*,#7730,.T.);
#10712=ORIENTED_EDGE('',*,*,#7732,.T.);
#10713=ORIENTED_EDGE('',*,*,#7727,.T.);
#10714=ORIENTED_EDGE('',*,*,#7672,.F.);
#10715=ORIENTED_EDGE('',*,*,#7724,.T.);
#10716=ORIENTED_EDGE('',*,*,#7726,.T.);
#10717=ORIENTED_EDGE('',*,*,#7721,.T.);
#10718=ORIENTED_EDGE('',*,*,#7669,.F.);
#10719=ORIENTED_EDGE('',*,*,#7609,.T.);
#10720=ORIENTED_EDGE('',*,*,#7612,.T.);
#10721=ORIENTED_EDGE('',*,*,#7605,.T.);
#10722=ORIENTED_EDGE('',*,*,#7668,.F.);
#10723=ORIENTED_EDGE('',*,*,#7929,.T.);
#10724=ORIENTED_EDGE('',*,*,#7931,.T.);
#10725=ORIENTED_EDGE('',*,*,#7926,.T.);
#10726=ORIENTED_EDGE('',*,*,#7665,.F.);
#10727=ORIENTED_EDGE('',*,*,#7923,.T.);
#10728=ORIENTED_EDGE('',*,*,#7925,.T.);
#10729=ORIENTED_EDGE('',*,*,#7920,.T.);
#10730=ORIENTED_EDGE('',*,*,#7662,.F.);
#10731=ORIENTED_EDGE('',*,*,#7917,.T.);
#10732=ORIENTED_EDGE('',*,*,#7919,.T.);
#10733=ORIENTED_EDGE('',*,*,#7914,.T.);
#10734=ORIENTED_EDGE('',*,*,#7659,.F.);
#10735=ORIENTED_EDGE('',*,*,#7911,.T.);
#10736=ORIENTED_EDGE('',*,*,#7913,.T.);
#10737=ORIENTED_EDGE('',*,*,#7908,.T.);
#10738=ORIENTED_EDGE('',*,*,#7656,.F.);
#10739=ORIENTED_EDGE('',*,*,#7905,.T.);
#10740=ORIENTED_EDGE('',*,*,#7907,.T.);
#10741=ORIENTED_EDGE('',*,*,#7902,.T.);
#10742=ORIENTED_EDGE('',*,*,#7653,.F.);
#10743=ORIENTED_EDGE('',*,*,#7899,.T.);
#10744=ORIENTED_EDGE('',*,*,#7901,.T.);
#10745=ORIENTED_EDGE('',*,*,#7896,.T.);
#10746=ORIENTED_EDGE('',*,*,#7650,.F.);
#10747=ORIENTED_EDGE('',*,*,#7893,.T.);
#10748=ORIENTED_EDGE('',*,*,#7895,.T.);
#10749=ORIENTED_EDGE('',*,*,#7890,.T.);
#10750=ORIENTED_EDGE('',*,*,#7647,.F.);
#10751=ORIENTED_EDGE('',*,*,#7887,.T.);
#10752=ORIENTED_EDGE('',*,*,#7889,.T.);
#10753=ORIENTED_EDGE('',*,*,#7884,.T.);
#10754=ORIENTED_EDGE('',*,*,#7644,.F.);
#10755=ORIENTED_EDGE('',*,*,#7881,.T.);
#10756=ORIENTED_EDGE('',*,*,#7883,.T.);
#10757=ORIENTED_EDGE('',*,*,#7878,.T.);
#10758=ORIENTED_EDGE('',*,*,#7641,.F.);
#10759=ORIENTED_EDGE('',*,*,#7875,.T.);
#10760=ORIENTED_EDGE('',*,*,#7877,.T.);
#10761=ORIENTED_EDGE('',*,*,#7872,.T.);
#10762=ORIENTED_EDGE('',*,*,#7638,.F.);
#10763=ORIENTED_EDGE('',*,*,#7869,.T.);
#10764=ORIENTED_EDGE('',*,*,#7871,.T.);
#10765=ORIENTED_EDGE('',*,*,#7866,.T.);
#10766=ORIENTED_EDGE('',*,*,#7635,.F.);
#10767=ORIENTED_EDGE('',*,*,#7863,.T.);
#10768=ORIENTED_EDGE('',*,*,#7865,.T.);
#10769=ORIENTED_EDGE('',*,*,#7860,.T.);
#10770=ORIENTED_EDGE('',*,*,#7632,.F.);
#10771=ORIENTED_EDGE('',*,*,#7857,.T.);
#10772=ORIENTED_EDGE('',*,*,#7859,.T.);
#10773=ORIENTED_EDGE('',*,*,#7854,.T.);
#10774=ORIENTED_EDGE('',*,*,#7629,.F.);
#10775=ORIENTED_EDGE('',*,*,#7851,.T.);
#10776=ORIENTED_EDGE('',*,*,#7853,.T.);
#10777=ORIENTED_EDGE('',*,*,#7848,.T.);
#10778=ORIENTED_EDGE('',*,*,#7626,.F.);
#10779=ORIENTED_EDGE('',*,*,#7845,.T.);
#10780=ORIENTED_EDGE('',*,*,#7847,.T.);
#10781=ORIENTED_EDGE('',*,*,#7842,.T.);
#10782=ORIENTED_EDGE('',*,*,#7623,.F.);
#10783=ORIENTED_EDGE('',*,*,#7839,.T.);
#10784=ORIENTED_EDGE('',*,*,#7841,.T.);
#10785=ORIENTED_EDGE('',*,*,#7836,.T.);
#10786=ORIENTED_EDGE('',*,*,#7620,.F.);
#10787=ORIENTED_EDGE('',*,*,#7833,.T.);
#10788=ORIENTED_EDGE('',*,*,#7835,.T.);
#10789=ORIENTED_EDGE('',*,*,#7830,.T.);
#10790=ORIENTED_EDGE('',*,*,#7617,.F.);
#10791=ORIENTED_EDGE('',*,*,#7827,.T.);
#10792=ORIENTED_EDGE('',*,*,#7829,.T.);
#10793=ORIENTED_EDGE('',*,*,#7824,.T.);
#10794=ORIENTED_EDGE('',*,*,#7614,.F.);
#10795=ORIENTED_EDGE('',*,*,#7820,.T.);
#10796=ORIENTED_EDGE('',*,*,#7720,.F.);
#10797=ORIENTED_EDGE('',*,*,#7933,.T.);
#10798=ORIENTED_EDGE('',*,*,#7934,.T.);
#10799=ORIENTED_EDGE('',*,*,#7935,.T.);
#10800=ORIENTED_EDGE('',*,*,#7936,.T.);
#10801=ORIENTED_EDGE('',*,*,#7937,.T.);
#10802=ORIENTED_EDGE('',*,*,#7938,.T.);
#10803=ORIENTED_EDGE('',*,*,#7939,.F.);
#10804=ORIENTED_EDGE('',*,*,#7940,.T.);
#10805=ORIENTED_EDGE('',*,*,#7941,.F.);
#10806=ORIENTED_EDGE('',*,*,#7942,.T.);
#10807=ORIENTED_EDGE('',*,*,#7943,.F.);
#10808=ORIENTED_EDGE('',*,*,#7944,.T.);
#10809=ORIENTED_EDGE('',*,*,#7945,.F.);
#10810=ORIENTED_EDGE('',*,*,#7946,.T.);
#10811=ORIENTED_EDGE('',*,*,#7947,.F.);
#10812=ORIENTED_EDGE('',*,*,#7948,.T.);
#10813=ORIENTED_EDGE('',*,*,#7949,.F.);
#10814=ORIENTED_EDGE('',*,*,#7950,.T.);
#10815=ORIENTED_EDGE('',*,*,#7951,.T.);
#10816=ORIENTED_EDGE('',*,*,#7950,.F.);
#10817=ORIENTED_EDGE('',*,*,#7948,.F.);
#10818=ORIENTED_EDGE('',*,*,#7946,.F.);
#10819=ORIENTED_EDGE('',*,*,#7944,.F.);
#10820=ORIENTED_EDGE('',*,*,#7942,.F.);
#10821=ORIENTED_EDGE('',*,*,#7940,.F.);
#10822=ORIENTED_EDGE('',*,*,#7951,.F.);
#10823=ORIENTED_EDGE('',*,*,#7933,.F.);
#10824=ORIENTED_EDGE('',*,*,#7952,.T.);
#10825=ORIENTED_EDGE('',*,*,#7939,.T.);
#10826=ORIENTED_EDGE('',*,*,#7953,.F.);
#10827=ORIENTED_EDGE('',*,*,#7938,.F.);
#10828=ORIENTED_EDGE('',*,*,#7954,.T.);
#10829=ORIENTED_EDGE('',*,*,#7949,.T.);
#10830=ORIENTED_EDGE('',*,*,#7952,.F.);
#10831=ORIENTED_EDGE('',*,*,#7937,.F.);
#10832=ORIENTED_EDGE('',*,*,#7955,.T.);
#10833=ORIENTED_EDGE('',*,*,#7947,.T.);
#10834=ORIENTED_EDGE('',*,*,#7954,.F.);
#10835=ORIENTED_EDGE('',*,*,#7936,.F.);
#10836=ORIENTED_EDGE('',*,*,#7956,.T.);
#10837=ORIENTED_EDGE('',*,*,#7945,.T.);
#10838=ORIENTED_EDGE('',*,*,#7955,.F.);
#10839=ORIENTED_EDGE('',*,*,#7935,.F.);
#10840=ORIENTED_EDGE('',*,*,#7957,.T.);
#10841=ORIENTED_EDGE('',*,*,#7943,.T.);
#10842=ORIENTED_EDGE('',*,*,#7956,.F.);
#10843=ORIENTED_EDGE('',*,*,#7934,.F.);
#10844=ORIENTED_EDGE('',*,*,#7953,.T.);
#10845=ORIENTED_EDGE('',*,*,#7941,.T.);
#10846=ORIENTED_EDGE('',*,*,#7957,.F.);
#12918=CYLINDRICAL_SURFACE('',#14115,1.92913);
#12919=CYLINDRICAL_SURFACE('',#14117,1.92913);
#12920=CYLINDRICAL_SURFACE('',#14118,1.92913);
#12921=CYLINDRICAL_SURFACE('',#14119,1.92913);
#12922=CYLINDRICAL_SURFACE('',#14120,1.92913);
#12923=CYLINDRICAL_SURFACE('',#14121,1.92913);
#12924=CYLINDRICAL_SURFACE('',#14122,1.92913);
#12925=CYLINDRICAL_SURFACE('',#14123,1.92913);
#12926=CYLINDRICAL_SURFACE('',#14124,1.92913);
#12927=CYLINDRICAL_SURFACE('',#14125,1.92913);
#12928=CYLINDRICAL_SURFACE('',#14126,1.92913);
#12929=CYLINDRICAL_SURFACE('',#14127,1.92913);
#12930=CYLINDRICAL_SURFACE('',#14128,1.92913);
#12931=CYLINDRICAL_SURFACE('',#14129,1.92913);
#12932=CYLINDRICAL_SURFACE('',#14130,1.92913);
#12933=CYLINDRICAL_SURFACE('',#14131,1.92913);
#12934=CYLINDRICAL_SURFACE('',#14132,1.92913);
#12935=CYLINDRICAL_SURFACE('',#14133,1.92913);
#12936=CYLINDRICAL_SURFACE('',#14134,1.92913);
#12937=CYLINDRICAL_SURFACE('',#14135,2.36347);
#12938=CYLINDRICAL_SURFACE('',#14139,1.92913);
#12939=CYLINDRICAL_SURFACE('',#14337,3.9624);
#13173=ADVANCED_FACE('',(#2213),#12918,.T.);
#13174=ADVANCED_FACE('',(#2214),#12919,.T.);
#13175=ADVANCED_FACE('',(#2215),#12920,.T.);
#13176=ADVANCED_FACE('',(#2216),#12921,.T.);
#13177=ADVANCED_FACE('',(#2217),#12922,.T.);
#13178=ADVANCED_FACE('',(#2218),#12923,.T.);
#13179=ADVANCED_FACE('',(#2219),#12924,.T.);
#13180=ADVANCED_FACE('',(#2220),#12925,.T.);
#13181=ADVANCED_FACE('',(#2221),#12926,.T.);
#13182=ADVANCED_FACE('',(#2222),#12927,.T.);
#13183=ADVANCED_FACE('',(#2223),#12928,.T.);
#13184=ADVANCED_FACE('',(#2224),#12929,.T.);
#13185=ADVANCED_FACE('',(#2225),#12930,.T.);
#13186=ADVANCED_FACE('',(#2226),#12931,.T.);
#13187=ADVANCED_FACE('',(#2227),#12932,.T.);
#13188=ADVANCED_FACE('',(#2228),#12933,.T.);
#13189=ADVANCED_FACE('',(#2229),#12934,.T.);
#13190=ADVANCED_FACE('',(#2230),#12935,.T.);
#13191=ADVANCED_FACE('',(#2231),#12936,.T.);
#13192=ADVANCED_FACE('',(#2232),#12937,.T.);
#13193=ADVANCED_FACE('',(#2233),#12938,.T.);
#13194=ADVANCED_FACE('',(#2234),#1652,.T.);
#13195=ADVANCED_FACE('',(#2235),#1006,.F.);
#13196=ADVANCED_FACE('',(#2236),#1653,.F.);
#13197=ADVANCED_FACE('',(#2237),#1007,.F.);
#13198=ADVANCED_FACE('',(#2238),#1003,.F.);
#13199=ADVANCED_FACE('',(#2239,#1559),#1654,.F.);
#13200=ADVANCED_FACE('',(#2240),#1094,.T.);
#13201=ADVANCED_FACE('',(#2241),#1655,.F.);
#13202=ADVANCED_FACE('',(#2242),#1656,.F.);
#13203=ADVANCED_FACE('',(#2243),#1657,.F.);
#13204=ADVANCED_FACE('',(#2244),#1658,.F.);
#13205=ADVANCED_FACE('',(#2245),#1095,.T.);
#13206=ADVANCED_FACE('',(#2246),#1659,.F.);
#13207=ADVANCED_FACE('',(#2247),#1660,.F.);
#13208=ADVANCED_FACE('',(#2248),#1661,.F.);
#13209=ADVANCED_FACE('',(#2249),#1662,.F.);
#13210=ADVANCED_FACE('',(#2250),#1663,.F.);
#13211=ADVANCED_FACE('',(#2251),#1664,.F.);
#13212=ADVANCED_FACE('',(#2252),#1665,.F.);
#13213=ADVANCED_FACE('',(#2253),#1666,.F.);
#13214=ADVANCED_FACE('',(#2254),#1667,.F.);
#13215=ADVANCED_FACE('',(#2255),#1668,.F.);
#13216=ADVANCED_FACE('',(#2256),#1669,.F.);
#13217=ADVANCED_FACE('',(#2257),#1670,.F.);
#13218=ADVANCED_FACE('',(#2258),#1671,.F.);
#13219=ADVANCED_FACE('',(#2259),#1672,.F.);
#13220=ADVANCED_FACE('',(#2260),#1673,.F.);
#13221=ADVANCED_FACE('',(#2261),#1674,.F.);
#13222=ADVANCED_FACE('',(#2262),#1675,.F.);
#13223=ADVANCED_FACE('',(#2263),#1676,.F.);
#13224=ADVANCED_FACE('',(#2264),#1677,.F.);
#13225=ADVANCED_FACE('',(#2265),#1678,.F.);
#13226=ADVANCED_FACE('',(#2266),#1679,.F.);
#13227=ADVANCED_FACE('',(#2267),#1680,.F.);
#13228=ADVANCED_FACE('',(#2268),#1681,.F.);
#13229=ADVANCED_FACE('',(#2269),#1682,.F.);
#13230=ADVANCED_FACE('',(#2270),#1683,.F.);
#13231=ADVANCED_FACE('',(#2271),#1684,.F.);
#13232=ADVANCED_FACE('',(#2272),#1685,.F.);
#13233=ADVANCED_FACE('',(#2273),#1686,.F.);
#13234=ADVANCED_FACE('',(#2274),#1687,.F.);
#13235=ADVANCED_FACE('',(#2275),#1688,.F.);
#13236=ADVANCED_FACE('',(#2276),#1689,.F.);
#13237=ADVANCED_FACE('',(#2277),#1690,.F.);
#13238=ADVANCED_FACE('',(#2278),#1691,.F.);
#13239=ADVANCED_FACE('',(#2279),#1692,.F.);
#13240=ADVANCED_FACE('',(#2280),#1693,.F.);
#13241=ADVANCED_FACE('',(#2281),#1694,.F.);
#13242=ADVANCED_FACE('',(#2282),#1695,.F.);
#13243=ADVANCED_FACE('',(#2283),#1696,.F.);
#13244=ADVANCED_FACE('',(#2284),#1697,.F.);
#13245=ADVANCED_FACE('',(#2285),#1698,.F.);
#13246=ADVANCED_FACE('',(#2286),#1699,.F.);
#13247=ADVANCED_FACE('',(#2287),#1700,.F.);
#13248=ADVANCED_FACE('',(#2288),#1701,.F.);
#13249=ADVANCED_FACE('',(#2289),#1702,.F.);
#13250=ADVANCED_FACE('',(#2290),#1703,.F.);
#13251=ADVANCED_FACE('',(#2291),#1704,.F.);
#13252=ADVANCED_FACE('',(#2292),#1705,.F.);
#13253=ADVANCED_FACE('',(#2293),#1706,.F.);
#13254=ADVANCED_FACE('',(#2294),#1707,.F.);
#13255=ADVANCED_FACE('',(#2295),#1708,.F.);
#13256=ADVANCED_FACE('',(#2296),#1709,.F.);
#13257=ADVANCED_FACE('',(#2297),#1710,.F.);
#13258=ADVANCED_FACE('',(#2298),#1711,.F.);
#13259=ADVANCED_FACE('',(#2299),#1712,.F.);
#13260=ADVANCED_FACE('',(#2300),#1713,.F.);
#13261=ADVANCED_FACE('',(#2301),#1714,.F.);
#13262=ADVANCED_FACE('',(#2302),#1715,.F.);
#13263=ADVANCED_FACE('',(#2303),#1716,.F.);
#13264=ADVANCED_FACE('',(#2304),#1717,.F.);
#13265=ADVANCED_FACE('',(#2305),#1718,.F.);
#13266=ADVANCED_FACE('',(#2306),#1719,.F.);
#13267=ADVANCED_FACE('',(#2307),#1720,.F.);
#13268=ADVANCED_FACE('',(#2308),#1721,.F.);
#13269=ADVANCED_FACE('',(#2309),#1722,.F.);
#13270=ADVANCED_FACE('',(#2310),#1723,.F.);
#13271=ADVANCED_FACE('',(#2311),#1724,.F.);
#13272=ADVANCED_FACE('',(#2312),#1725,.F.);
#13273=ADVANCED_FACE('',(#2313),#1726,.F.);
#13274=ADVANCED_FACE('',(#2314),#1727,.F.);
#13275=ADVANCED_FACE('',(#2315),#1728,.F.);
#13276=ADVANCED_FACE('',(#2316),#1729,.F.);
#13277=ADVANCED_FACE('',(#2317),#1730,.F.);
#13278=ADVANCED_FACE('',(#2318),#1731,.F.);
#13279=ADVANCED_FACE('',(#2319),#1732,.F.);
#13280=ADVANCED_FACE('',(#2320),#1733,.F.);
#13281=ADVANCED_FACE('',(#2321),#1734,.F.);
#13282=ADVANCED_FACE('',(#2322),#1735,.F.);
#13283=ADVANCED_FACE('',(#2323),#1736,.F.);
#13284=ADVANCED_FACE('',(#2324),#1737,.F.);
#13285=ADVANCED_FACE('',(#2325),#1738,.F.);
#13286=ADVANCED_FACE('',(#2326),#1739,.F.);
#13287=ADVANCED_FACE('',(#2327),#1740,.F.);
#13288=ADVANCED_FACE('',(#2328),#1741,.F.);
#13289=ADVANCED_FACE('',(#2329),#1742,.F.);
#13290=ADVANCED_FACE('',(#2330),#1743,.F.);
#13291=ADVANCED_FACE('',(#2331),#1744,.F.);
#13292=ADVANCED_FACE('',(#2332),#1745,.F.);
#13293=ADVANCED_FACE('',(#2333),#1746,.F.);
#13294=ADVANCED_FACE('',(#2334),#1747,.F.);
#13295=ADVANCED_FACE('',(#2335),#1748,.F.);
#13296=ADVANCED_FACE('',(#2336),#1749,.F.);
#13297=ADVANCED_FACE('',(#2337),#1750,.F.);
#13298=ADVANCED_FACE('',(#2338),#1751,.F.);
#13299=ADVANCED_FACE('',(#2339),#1752,.F.);
#13300=ADVANCED_FACE('',(#2340),#1753,.F.);
#13301=ADVANCED_FACE('',(#2341),#1754,.F.);
#13302=ADVANCED_FACE('',(#2342),#1755,.F.);
#13303=ADVANCED_FACE('',(#2343),#1756,.F.);
#13304=ADVANCED_FACE('',(#2344),#1757,.F.);
#13305=ADVANCED_FACE('',(#2345),#1758,.F.);
#13306=ADVANCED_FACE('',(#2346),#1759,.F.);
#13307=ADVANCED_FACE('',(#2347),#1760,.F.);
#13308=ADVANCED_FACE('',(#2348),#1761,.F.);
#13309=ADVANCED_FACE('',(#2349),#1762,.F.);
#13310=ADVANCED_FACE('',(#2350),#1763,.F.);
#13311=ADVANCED_FACE('',(#2351),#12939,.T.);
#13312=ADVANCED_FACE('',(#2352,#1560),#1764,.T.);
#13313=ADVANCED_FACE('',(#2353),#1765,.F.);
#13314=ADVANCED_FACE('',(#2354),#1766,.F.);
#13315=ADVANCED_FACE('',(#2355),#1767,.F.);
#13316=ADVANCED_FACE('',(#2356),#1768,.F.);
#13317=ADVANCED_FACE('',(#2357),#1769,.F.);
#13318=ADVANCED_FACE('',(#2358),#1770,.F.);
#13319=ADVANCED_FACE('',(#2359),#1096,.F.);
#13320=ADVANCED_FACE('',(#2360),#1771,.F.);
#13321=ADVANCED_FACE('',(#2361),#1772,.F.);
#13322=ADVANCED_FACE('',(#2362),#1773,.F.);
#13323=ADVANCED_FACE('',(#2363),#1774,.F.);
#13324=ADVANCED_FACE('',(#2364),#1775,.F.);
#13325=ADVANCED_FACE('',(#2365),#1776,.F.);
#13642=CLOSED_SHELL('',(#13173,#13174,#13175,#13176,#13177,#13178,#13179,
#13180,#13181,#13182,#13183,#13184,#13185,#13186,#13187,#13188,#13189,#13190,
#13191,#13192,#13193,#13194,#13195,#13196,#13197,#13198,#13199,#13200,#13201,
#13202,#13203,#13204,#13205,#13206,#13207,#13208,#13209,#13210,#13211,#13212,
#13213,#13214,#13215,#13216,#13217,#13218,#13219,#13220,#13221,#13222,#13223,
#13224,#13225,#13226,#13227,#13228,#13229,#13230,#13231,#13232,#13233,#13234,
#13235,#13236,#13237,#13238,#13239,#13240,#13241,#13242,#13243,#13244,#13245,
#13246,#13247,#13248,#13249,#13250,#13251,#13252,#13253,#13254,#13255,#13256,
#13257,#13258,#13259,#13260,#13261,#13262,#13263,#13264,#13265,#13266,#13267,
#13268,#13269,#13270,#13271,#13272,#13273,#13274,#13275,#13276,#13277,#13278,
#13279,#13280,#13281,#13282,#13283,#13284,#13285,#13286,#13287,#13288,#13289,
#13290,#13291,#13292,#13293,#13294,#13295,#13296,#13297,#13298,#13299,#13300,
#13301,#13302,#13303,#13304,#13305,#13306,#13307,#13308,#13309,#13310,#13311,
#13312,#13313,#13314,#13315,#13316,#13317,#13318,#13319,#13320,#13321,#13322,
#13323,#13324,#13325));
#14114=AXIS2_PLACEMENT_3D('',#19891,#16004,#16005);
#14115=AXIS2_PLACEMENT_3D('',#19892,#16006,#16007);
#14116=AXIS2_PLACEMENT_3D('',#20028,#16009,#16010);
#14117=AXIS2_PLACEMENT_3D('',#20114,#16011,#16012);
#14118=AXIS2_PLACEMENT_3D('',#20540,#16014,#16015);
#14119=AXIS2_PLACEMENT_3D('',#20962,#16017,#16018);
#14120=AXIS2_PLACEMENT_3D('',#21424,#16020,#16021);
#14121=AXIS2_PLACEMENT_3D('',#21844,#16023,#16024);
#14122=AXIS2_PLACEMENT_3D('',#22308,#16026,#16027);
#14123=AXIS2_PLACEMENT_3D('',#22730,#16029,#16030);
#14124=AXIS2_PLACEMENT_3D('',#23229,#16032,#16033);
#14125=AXIS2_PLACEMENT_3D('',#23489,#16035,#16036);
#14126=AXIS2_PLACEMENT_3D('',#23793,#16038,#16039);
#14127=AXIS2_PLACEMENT_3D('',#24182,#16041,#16042);
#14128=AXIS2_PLACEMENT_3D('',#24607,#16044,#16045);
#14129=AXIS2_PLACEMENT_3D('',#25043,#16047,#16048);
#14130=AXIS2_PLACEMENT_3D('',#25481,#16050,#16051);
#14131=AXIS2_PLACEMENT_3D('',#25909,#16053,#16054);
#14132=AXIS2_PLACEMENT_3D('',#26351,#16056,#16057);
#14133=AXIS2_PLACEMENT_3D('',#26783,#16059,#16060);
#14134=AXIS2_PLACEMENT_3D('',#27249,#16062,#16063);
#14135=AXIS2_PLACEMENT_3D('',#27667,#16065,#16066);
#14136=AXIS2_PLACEMENT_3D('',#27738,#16067,#16068);
#14137=AXIS2_PLACEMENT_3D('',#31404,#16069,#16070);
#14138=AXIS2_PLACEMENT_3D('',#31406,#16071,#16072);
#14139=AXIS2_PLACEMENT_3D('',#34869,#16073,#16074);
#14140=AXIS2_PLACEMENT_3D('',#35041,#16075,#16076);
#14141=AXIS2_PLACEMENT_3D('',#35170,#16077,#16078);
#14142=AXIS2_PLACEMENT_3D('',#35172,#16079,#16080);
#14143=AXIS2_PLACEMENT_3D('',#35918,#16081,#16082);
#14144=AXIS2_PLACEMENT_3D('',#35921,#16083,#16084);
#14145=AXIS2_PLACEMENT_3D('',#36001,#16085,#16086);
#14146=AXIS2_PLACEMENT_3D('',#36510,#16087,#16088);
#14147=AXIS2_PLACEMENT_3D('',#36512,#16089,#16090);
#14148=AXIS2_PLACEMENT_3D('',#36513,#16091,#16092);
#14149=AXIS2_PLACEMENT_3D('',#36514,#16093,#16094);
#14150=AXIS2_PLACEMENT_3D('',#36516,#16095,#16096);
#14151=AXIS2_PLACEMENT_3D('',#36517,#16097,#16098);
#14152=AXIS2_PLACEMENT_3D('',#36520,#16100,#16101);
#14153=AXIS2_PLACEMENT_3D('',#36521,#16102,#16103);
#14154=AXIS2_PLACEMENT_3D('',#36522,#16104,#16105);
#14155=AXIS2_PLACEMENT_3D('',#36533,#16109,#16110);
#14156=AXIS2_PLACEMENT_3D('',#36541,#16113,#16114);
#14157=AXIS2_PLACEMENT_3D('',#36542,#16115,#16116);
#14158=AXIS2_PLACEMENT_3D('',#36543,#16117,#16118);
#14159=AXIS2_PLACEMENT_3D('',#36550,#16119,#16120);
#14160=AXIS2_PLACEMENT_3D('',#36560,#16121,#16122);
#14161=AXIS2_PLACEMENT_3D('',#36570,#16123,#16124);
#14162=AXIS2_PLACEMENT_3D('',#36580,#16125,#16126);
#14163=AXIS2_PLACEMENT_3D('',#36590,#16127,#16128);
#14164=AXIS2_PLACEMENT_3D('',#36600,#16129,#16130);
#14165=AXIS2_PLACEMENT_3D('',#36610,#16131,#16132);
#14166=AXIS2_PLACEMENT_3D('',#36620,#16133,#16134);
#14167=AXIS2_PLACEMENT_3D('',#36630,#16135,#16136);
#14168=AXIS2_PLACEMENT_3D('',#36640,#16137,#16138);
#14169=AXIS2_PLACEMENT_3D('',#36650,#16139,#16140);
#14170=AXIS2_PLACEMENT_3D('',#36660,#16141,#16142);
#14171=AXIS2_PLACEMENT_3D('',#36670,#16143,#16144);
#14172=AXIS2_PLACEMENT_3D('',#36680,#16145,#16146);
#14173=AXIS2_PLACEMENT_3D('',#36690,#16147,#16148);
#14174=AXIS2_PLACEMENT_3D('',#36700,#16149,#16150);
#14175=AXIS2_PLACEMENT_3D('',#36710,#16151,#16152);
#14176=AXIS2_PLACEMENT_3D('',#36720,#16153,#16154);
#14177=AXIS2_PLACEMENT_3D('',#36729,#16155,#16156);
#14178=AXIS2_PLACEMENT_3D('',#36731,#16157,#16158);
#14179=AXIS2_PLACEMENT_3D('',#36741,#16159,#16160);
#14180=AXIS2_PLACEMENT_3D('',#36751,#16161,#16162);
#14181=AXIS2_PLACEMENT_3D('',#36761,#16163,#16164);
#14182=AXIS2_PLACEMENT_3D('',#36771,#16165,#16166);
#14183=AXIS2_PLACEMENT_3D('',#36781,#16167,#16168);
#14184=AXIS2_PLACEMENT_3D('',#36791,#16169,#16170);
#14185=AXIS2_PLACEMENT_3D('',#36801,#16171,#16172);
#14186=AXIS2_PLACEMENT_3D('',#36811,#16173,#16174);
#14187=AXIS2_PLACEMENT_3D('',#36821,#16175,#16176);
#14188=AXIS2_PLACEMENT_3D('',#36831,#16177,#16178);
#14189=AXIS2_PLACEMENT_3D('',#36841,#16179,#16180);
#14190=AXIS2_PLACEMENT_3D('',#36851,#16181,#16182);
#14191=AXIS2_PLACEMENT_3D('',#36861,#16183,#16184);
#14192=AXIS2_PLACEMENT_3D('',#36871,#16185,#16186);
#14193=AXIS2_PLACEMENT_3D('',#36881,#16187,#16188);
#14194=AXIS2_PLACEMENT_3D('',#36891,#16189,#16190);
#14195=AXIS2_PLACEMENT_3D('',#36897,#16192,#16193);
#14196=AXIS2_PLACEMENT_3D('',#36898,#16194,#16195);
#14197=AXIS2_PLACEMENT_3D('',#36904,#16199,#16200);
#14198=AXIS2_PLACEMENT_3D('',#36908,#16203,#16204);
#14199=AXIS2_PLACEMENT_3D('',#36909,#16205,#16206);
#14200=AXIS2_PLACEMENT_3D('',#36910,#16207,#16208);
#14201=AXIS2_PLACEMENT_3D('',#36916,#16212,#16213);
#14202=AXIS2_PLACEMENT_3D('',#36920,#16216,#16217);
#14203=AXIS2_PLACEMENT_3D('',#36921,#16218,#16219);
#14204=AXIS2_PLACEMENT_3D('',#36922,#16220,#16221);
#14205=AXIS2_PLACEMENT_3D('',#36928,#16225,#16226);
#14206=AXIS2_PLACEMENT_3D('',#36932,#16229,#16230);
#14207=AXIS2_PLACEMENT_3D('',#36933,#16231,#16232);
#14208=AXIS2_PLACEMENT_3D('',#36934,#16233,#16234);
#14209=AXIS2_PLACEMENT_3D('',#36940,#16238,#16239);
#14210=AXIS2_PLACEMENT_3D('',#36944,#16242,#16243);
#14211=AXIS2_PLACEMENT_3D('',#36945,#16244,#16245);
#14212=AXIS2_PLACEMENT_3D('',#36946,#16246,#16247);
#14213=AXIS2_PLACEMENT_3D('',#36952,#16251,#16252);
#14214=AXIS2_PLACEMENT_3D('',#36956,#16255,#16256);
#14215=AXIS2_PLACEMENT_3D('',#36957,#16257,#16258);
#14216=AXIS2_PLACEMENT_3D('',#36958,#16259,#16260);
#14217=AXIS2_PLACEMENT_3D('',#36964,#16264,#16265);
#14218=AXIS2_PLACEMENT_3D('',#36968,#16268,#16269);
#14219=AXIS2_PLACEMENT_3D('',#36969,#16270,#16271);
#14220=AXIS2_PLACEMENT_3D('',#36970,#16272,#16273);
#14221=AXIS2_PLACEMENT_3D('',#36976,#16277,#16278);
#14222=AXIS2_PLACEMENT_3D('',#36980,#16281,#16282);
#14223=AXIS2_PLACEMENT_3D('',#36981,#16283,#16284);
#14224=AXIS2_PLACEMENT_3D('',#36982,#16285,#16286);
#14225=AXIS2_PLACEMENT_3D('',#36988,#16290,#16291);
#14226=AXIS2_PLACEMENT_3D('',#36992,#16294,#16295);
#14227=AXIS2_PLACEMENT_3D('',#36993,#16296,#16297);
#14228=AXIS2_PLACEMENT_3D('',#36994,#16298,#16299);
#14229=AXIS2_PLACEMENT_3D('',#37000,#16303,#16304);
#14230=AXIS2_PLACEMENT_3D('',#37004,#16307,#16308);
#14231=AXIS2_PLACEMENT_3D('',#37005,#16309,#16310);
#14232=AXIS2_PLACEMENT_3D('',#37006,#16311,#16312);
#14233=AXIS2_PLACEMENT_3D('',#37012,#16316,#16317);
#14234=AXIS2_PLACEMENT_3D('',#37016,#16320,#16321);
#14235=AXIS2_PLACEMENT_3D('',#37017,#16322,#16323);
#14236=AXIS2_PLACEMENT_3D('',#37018,#16324,#16325);
#14237=AXIS2_PLACEMENT_3D('',#37024,#16329,#16330);
#14238=AXIS2_PLACEMENT_3D('',#37028,#16333,#16334);
#14239=AXIS2_PLACEMENT_3D('',#37029,#16335,#16336);
#14240=AXIS2_PLACEMENT_3D('',#37030,#16337,#16338);
#14241=AXIS2_PLACEMENT_3D('',#37036,#16342,#16343);
#14242=AXIS2_PLACEMENT_3D('',#37040,#16346,#16347);
#14243=AXIS2_PLACEMENT_3D('',#37041,#16348,#16349);
#14244=AXIS2_PLACEMENT_3D('',#37042,#16350,#16351);
#14245=AXIS2_PLACEMENT_3D('',#37048,#16355,#16356);
#14246=AXIS2_PLACEMENT_3D('',#37052,#16359,#16360);
#14247=AXIS2_PLACEMENT_3D('',#37053,#16361,#16362);
#14248=AXIS2_PLACEMENT_3D('',#37054,#16363,#16364);
#14249=AXIS2_PLACEMENT_3D('',#37060,#16368,#16369);
#14250=AXIS2_PLACEMENT_3D('',#37064,#16372,#16373);
#14251=AXIS2_PLACEMENT_3D('',#37065,#16374,#16375);
#14252=AXIS2_PLACEMENT_3D('',#37066,#16376,#16377);
#14253=AXIS2_PLACEMENT_3D('',#37072,#16381,#16382);
#14254=AXIS2_PLACEMENT_3D('',#37076,#16385,#16386);
#14255=AXIS2_PLACEMENT_3D('',#37077,#16387,#16388);
#14256=AXIS2_PLACEMENT_3D('',#37078,#16389,#16390);
#14257=AXIS2_PLACEMENT_3D('',#37084,#16394,#16395);
#14258=AXIS2_PLACEMENT_3D('',#37088,#16398,#16399);
#14259=AXIS2_PLACEMENT_3D('',#37089,#16400,#16401);
#14260=AXIS2_PLACEMENT_3D('',#37090,#16402,#16403);
#14261=AXIS2_PLACEMENT_3D('',#37096,#16407,#16408);
#14262=AXIS2_PLACEMENT_3D('',#37100,#16411,#16412);
#14263=AXIS2_PLACEMENT_3D('',#37102,#16413,#16414);
#14264=AXIS2_PLACEMENT_3D('',#37103,#16415,#16416);
#14265=AXIS2_PLACEMENT_3D('',#37104,#16417,#16418);
#14266=AXIS2_PLACEMENT_3D('',#37110,#16422,#16423);
#14267=AXIS2_PLACEMENT_3D('',#37114,#16426,#16427);
#14268=AXIS2_PLACEMENT_3D('',#37115,#16428,#16429);
#14269=AXIS2_PLACEMENT_3D('',#37116,#16430,#16431);
#14270=AXIS2_PLACEMENT_3D('',#37122,#16435,#16436);
#14271=AXIS2_PLACEMENT_3D('',#37126,#16439,#16440);
#14272=AXIS2_PLACEMENT_3D('',#37127,#16441,#16442);
#14273=AXIS2_PLACEMENT_3D('',#37128,#16443,#16444);
#14274=AXIS2_PLACEMENT_3D('',#37134,#16448,#16449);
#14275=AXIS2_PLACEMENT_3D('',#37138,#16452,#16453);
#14276=AXIS2_PLACEMENT_3D('',#37139,#16454,#16455);
#14277=AXIS2_PLACEMENT_3D('',#37140,#16456,#16457);
#14278=AXIS2_PLACEMENT_3D('',#37146,#16461,#16462);
#14279=AXIS2_PLACEMENT_3D('',#37150,#16465,#16466);
#14280=AXIS2_PLACEMENT_3D('',#37151,#16467,#16468);
#14281=AXIS2_PLACEMENT_3D('',#37152,#16469,#16470);
#14282=AXIS2_PLACEMENT_3D('',#37158,#16474,#16475);
#14283=AXIS2_PLACEMENT_3D('',#37162,#16478,#16479);
#14284=AXIS2_PLACEMENT_3D('',#37163,#16480,#16481);
#14285=AXIS2_PLACEMENT_3D('',#37164,#16482,#16483);
#14286=AXIS2_PLACEMENT_3D('',#37170,#16487,#16488);
#14287=AXIS2_PLACEMENT_3D('',#37174,#16491,#16492);
#14288=AXIS2_PLACEMENT_3D('',#37175,#16493,#16494);
#14289=AXIS2_PLACEMENT_3D('',#37176,#16495,#16496);
#14290=AXIS2_PLACEMENT_3D('',#37182,#16500,#16501);
#14291=AXIS2_PLACEMENT_3D('',#37186,#16504,#16505);
#14292=AXIS2_PLACEMENT_3D('',#37187,#16506,#16507);
#14293=AXIS2_PLACEMENT_3D('',#37188,#16508,#16509);
#14294=AXIS2_PLACEMENT_3D('',#37194,#16513,#16514);
#14295=AXIS2_PLACEMENT_3D('',#37198,#16517,#16518);
#14296=AXIS2_PLACEMENT_3D('',#37199,#16519,#16520);
#14297=AXIS2_PLACEMENT_3D('',#37200,#16521,#16522);
#14298=AXIS2_PLACEMENT_3D('',#37206,#16526,#16527);
#14299=AXIS2_PLACEMENT_3D('',#37210,#16530,#16531);
#14300=AXIS2_PLACEMENT_3D('',#37211,#16532,#16533);
#14301=AXIS2_PLACEMENT_3D('',#37212,#16534,#16535);
#14302=AXIS2_PLACEMENT_3D('',#37218,#16539,#16540);
#14303=AXIS2_PLACEMENT_3D('',#37222,#16543,#16544);
#14304=AXIS2_PLACEMENT_3D('',#37223,#16545,#16546);
#14305=AXIS2_PLACEMENT_3D('',#37224,#16547,#16548);
#14306=AXIS2_PLACEMENT_3D('',#37230,#16552,#16553);
#14307=AXIS2_PLACEMENT_3D('',#37234,#16556,#16557);
#14308=AXIS2_PLACEMENT_3D('',#37235,#16558,#16559);
#14309=AXIS2_PLACEMENT_3D('',#37236,#16560,#16561);
#14310=AXIS2_PLACEMENT_3D('',#37242,#16565,#16566);
#14311=AXIS2_PLACEMENT_3D('',#37246,#16569,#16570);
#14312=AXIS2_PLACEMENT_3D('',#37247,#16571,#16572);
#14313=AXIS2_PLACEMENT_3D('',#37248,#16573,#16574);
#14314=AXIS2_PLACEMENT_3D('',#37254,#16578,#16579);
#14315=AXIS2_PLACEMENT_3D('',#37258,#16582,#16583);
#14316=AXIS2_PLACEMENT_3D('',#37259,#16584,#16585);
#14317=AXIS2_PLACEMENT_3D('',#37260,#16586,#16587);
#14318=AXIS2_PLACEMENT_3D('',#37266,#16591,#16592);
#14319=AXIS2_PLACEMENT_3D('',#37270,#16595,#16596);
#14320=AXIS2_PLACEMENT_3D('',#37271,#16597,#16598);
#14321=AXIS2_PLACEMENT_3D('',#37272,#16599,#16600);
#14322=AXIS2_PLACEMENT_3D('',#37278,#16604,#16605);
#14323=AXIS2_PLACEMENT_3D('',#37282,#16608,#16609);
#14324=AXIS2_PLACEMENT_3D('',#37283,#16610,#16611);
#14325=AXIS2_PLACEMENT_3D('',#37284,#16612,#16613);
#14326=AXIS2_PLACEMENT_3D('',#37290,#16617,#16618);
#14327=AXIS2_PLACEMENT_3D('',#37294,#16621,#16622);
#14328=AXIS2_PLACEMENT_3D('',#37295,#16623,#16624);
#14329=AXIS2_PLACEMENT_3D('',#37296,#16625,#16626);
#14330=AXIS2_PLACEMENT_3D('',#37302,#16630,#16631);
#14331=AXIS2_PLACEMENT_3D('',#37306,#16634,#16635);
#14332=AXIS2_PLACEMENT_3D('',#37307,#16636,#16637);
#14333=AXIS2_PLACEMENT_3D('',#37308,#16638,#16639);
#14334=AXIS2_PLACEMENT_3D('',#37314,#16643,#16644);
#14335=AXIS2_PLACEMENT_3D('',#37318,#16647,#16648);
#14336=AXIS2_PLACEMENT_3D('',#37319,#16649,#16650);
#14337=AXIS2_PLACEMENT_3D('',#37320,#16651,#16652);
#14338=AXIS2_PLACEMENT_3D('',#37322,#16654,#16655);
#14339=AXIS2_PLACEMENT_3D('',#37335,#16662,#16663);
#14340=AXIS2_PLACEMENT_3D('',#37339,#16665,#16666);
#14341=AXIS2_PLACEMENT_3D('',#37340,#16667,#16668);
#14342=AXIS2_PLACEMENT_3D('',#37343,#16670,#16671);
#14343=AXIS2_PLACEMENT_3D('',#37344,#16672,#16673);
#14344=AXIS2_PLACEMENT_3D('',#37347,#16675,#16676);
#14345=AXIS2_PLACEMENT_3D('',#37348,#16677,#16678);
#14346=AXIS2_PLACEMENT_3D('',#37351,#16680,#16681);
#14347=AXIS2_PLACEMENT_3D('',#37352,#16682,#16683);
#14348=AXIS2_PLACEMENT_3D('',#37355,#16685,#16686);
#14349=AXIS2_PLACEMENT_3D('',#37356,#16687,#16688);
#14350=AXIS2_PLACEMENT_3D('',#37358,#16690,#16691);
#14351=AXIS2_PLACEMENT_3D('',#37359,#16692,#16693);
#14352=AXIS2_PLACEMENT_3D('',#37362,#16695,#16696);
#14353=AXIS2_PLACEMENT_3D('',#37365,#16699,#16700);
#14354=AXIS2_PLACEMENT_3D('',#37367,#16702,#16703);
#14355=AXIS2_PLACEMENT_3D('',#37369,#16705,#16706);
#14356=AXIS2_PLACEMENT_3D('',#37371,#16708,#16709);
#14357=AXIS2_PLACEMENT_3D('',#37373,#16711,#16712);
#16004=DIRECTION('axis',(0.,0.,1.));
#16005=DIRECTION('refdir',(1.,0.,0.));
#16006=DIRECTION('center_axis',(0.,-1.,0.));
#16007=DIRECTION('ref_axis',(0.314059274495562,0.,-0.94940337691801));
#16008=DIRECTION('',(0.,1.,0.));
#16009=DIRECTION('center_axis',(0.,1.,0.));
#16010=DIRECTION('ref_axis',(1.,0.,1.05892830722154E-13));
#16011=DIRECTION('center_axis',(0.,-1.,0.));
#16012=DIRECTION('ref_axis',(0.314059274495562,0.,-0.94940337691801));
#16013=DIRECTION('',(0.,1.,0.));
#16014=DIRECTION('center_axis',(0.,-1.,0.));
#16015=DIRECTION('ref_axis',(0.314059274495562,0.,-0.94940337691801));
#16016=DIRECTION('',(0.,1.,0.));
#16017=DIRECTION('center_axis',(0.,-1.,0.));
#16018=DIRECTION('ref_axis',(0.314059274495562,0.,-0.94940337691801));
#16019=DIRECTION('',(0.,1.,0.));
#16020=DIRECTION('center_axis',(0.,-1.,0.));
#16021=DIRECTION('ref_axis',(0.314059274495562,0.,-0.94940337691801));
#16022=DIRECTION('',(0.,1.,0.));
#16023=DIRECTION('center_axis',(0.,-1.,0.));
#16024=DIRECTION('ref_axis',(0.314059274495562,0.,-0.94940337691801));
#16025=DIRECTION('',(0.,1.,0.));
#16026=DIRECTION('center_axis',(0.,-1.,0.));
#16027=DIRECTION('ref_axis',(0.314059274495562,0.,-0.94940337691801));
#16028=DIRECTION('',(0.,1.,0.));
#16029=DIRECTION('center_axis',(0.,-1.,0.));
#16030=DIRECTION('ref_axis',(0.314059274495562,0.,-0.94940337691801));
#16031=DIRECTION('',(0.,1.,0.));
#16032=DIRECTION('center_axis',(0.,-1.,0.));
#16033=DIRECTION('ref_axis',(0.314059274495562,0.,-0.94940337691801));
#16034=DIRECTION('',(0.,1.,0.));
#16035=DIRECTION('center_axis',(0.,-1.,0.));
#16036=DIRECTION('ref_axis',(0.314059274495562,0.,-0.94940337691801));
#16037=DIRECTION('',(0.,1.,0.));
#16038=DIRECTION('center_axis',(0.,-1.,0.));
#16039=DIRECTION('ref_axis',(0.314059274495562,0.,-0.94940337691801));
#16040=DIRECTION('',(0.,1.,0.));
#16041=DIRECTION('center_axis',(0.,-1.,0.));
#16042=DIRECTION('ref_axis',(0.314059274495562,0.,-0.94940337691801));
#16043=DIRECTION('',(0.,1.,0.));
#16044=DIRECTION('center_axis',(0.,-1.,0.));
#16045=DIRECTION('ref_axis',(0.314059274495562,0.,-0.94940337691801));
#16046=DIRECTION('',(0.,1.,0.));
#16047=DIRECTION('center_axis',(0.,-1.,0.));
#16048=DIRECTION('ref_axis',(0.314059274495562,0.,-0.94940337691801));
#16049=DIRECTION('',(0.,1.,0.));
#16050=DIRECTION('center_axis',(0.,-1.,0.));
#16051=DIRECTION('ref_axis',(0.314059274495562,0.,-0.94940337691801));
#16052=DIRECTION('',(0.,1.,0.));
#16053=DIRECTION('center_axis',(0.,-1.,0.));
#16054=DIRECTION('ref_axis',(0.314059274495562,0.,-0.94940337691801));
#16055=DIRECTION('',(0.,1.,0.));
#16056=DIRECTION('center_axis',(0.,-1.,0.));
#16057=DIRECTION('ref_axis',(0.314059274495562,0.,-0.94940337691801));
#16058=DIRECTION('',(0.,1.,0.));
#16059=DIRECTION('center_axis',(0.,-1.,0.));
#16060=DIRECTION('ref_axis',(0.314059274495562,0.,-0.94940337691801));
#16061=DIRECTION('',(0.,1.,0.));
#16062=DIRECTION('center_axis',(0.,-1.,0.));
#16063=DIRECTION('ref_axis',(0.314059274495562,0.,-0.94940337691801));
#16064=DIRECTION('',(0.,1.,0.));
#16065=DIRECTION('center_axis',(0.,-1.,0.));
#16066=DIRECTION('ref_axis',(1.,0.,0.));
#16067=DIRECTION('center_axis',(0.,1.,0.));
#16068=DIRECTION('ref_axis',(1.,0.,0.));
#16069=DIRECTION('center_axis',(0.,-1.,0.));
#16070=DIRECTION('ref_axis',(1.,0.,0.));
#16071=DIRECTION('center_axis',(0.,-1.,0.));
#16072=DIRECTION('ref_axis',(1.,0.,0.));
#16073=DIRECTION('center_axis',(0.,-1.,0.));
#16074=DIRECTION('ref_axis',(-0.3010495107773,0.,-0.953608510899912));
#16075=DIRECTION('center_axis',(0.,-1.,0.));
#16076=DIRECTION('ref_axis',(1.,0.,1.05892830722154E-13));
#16077=DIRECTION('center_axis',(0.,1.,0.));
#16078=DIRECTION('ref_axis',(0.,0.,1.));
#16079=DIRECTION('center_axis',(0.,-1.,0.));
#16080=DIRECTION('ref_axis',(1.,0.,0.));
#16081=DIRECTION('center_axis',(0.,1.,0.));
#16082=DIRECTION('ref_axis',(0.,0.,1.));
#16083=DIRECTION('center_axis',(0.,1.,0.));
#16084=DIRECTION('ref_axis',(1.,0.,0.));
#16085=DIRECTION('center_axis',(0.,1.,0.));
#16086=DIRECTION('ref_axis',(1.,0.,0.));
#16087=DIRECTION('center_axis',(0.,1.,0.));
#16088=DIRECTION('ref_axis',(0.,0.,1.));
#16089=DIRECTION('center_axis',(0.,-1.,0.));
#16090=DIRECTION('ref_axis',(1.,0.,0.));
#16091=DIRECTION('center_axis',(1.,0.,0.));
#16092=DIRECTION('ref_axis',(0.,0.,-1.));
#16093=DIRECTION('center_axis',(0.,1.,0.));
#16094=DIRECTION('ref_axis',(1.,0.,0.));
#16095=DIRECTION('center_axis',(0.,1.,0.));
#16096=DIRECTION('ref_axis',(1.,0.,0.));
#16097=DIRECTION('center_axis',(0.,1.,0.));
#16098=DIRECTION('ref_axis',(1.,0.,0.));
#16099=DIRECTION('',(0.707106781186547,-0.707106781186548,-8.65956056235493E-17));
#16100=DIRECTION('center_axis',(0.,1.,0.));
#16101=DIRECTION('ref_axis',(1.,0.,0.));
#16102=DIRECTION('center_axis',(0.,1.,0.));
#16103=DIRECTION('ref_axis',(1.,0.,0.));
#16104=DIRECTION('center_axis',(-0.241286600017026,0.,0.970453902383943));
#16105=DIRECTION('ref_axis',(-0.970453902383943,0.,-0.241286600017026));
#16106=DIRECTION('',(0.,1.,0.));
#16107=DIRECTION('',(-0.970453902383943,0.,-0.241286600017026));
#16108=DIRECTION('',(0.,-1.,0.));
#16109=DIRECTION('center_axis',(-0.558650020314832,0.,-0.829403493362693));
#16110=DIRECTION('ref_axis',(0.829403493362693,0.,-0.558650020314832));
#16111=DIRECTION('',(0.,-1.,0.));
#16112=DIRECTION('',(0.829403493362693,0.,-0.558650020314832));
#16113=DIRECTION('center_axis',(0.,-1.,0.));
#16114=DIRECTION('ref_axis',(-0.17364817766693,0.,-0.984807753012208));
#16115=DIRECTION('center_axis',(0.,-1.,0.));
#16116=DIRECTION('ref_axis',(1.,0.,0.));
#16117=DIRECTION('center_axis',(0.,-1.,0.));
#16118=DIRECTION('ref_axis',(1.,0.,0.));
#16119=DIRECTION('center_axis',(0.,1.,0.));
#16120=DIRECTION('ref_axis',(1.,0.,0.));
#16121=DIRECTION('center_axis',(0.,1.,0.));
#16122=DIRECTION('ref_axis',(1.,0.,0.));
#16123=DIRECTION('center_axis',(0.,1.,0.));
#16124=DIRECTION('ref_axis',(1.,0.,0.));
#16125=DIRECTION('center_axis',(0.,1.,0.));
#16126=DIRECTION('ref_axis',(1.,0.,0.));
#16127=DIRECTION('center_axis',(0.,1.,0.));
#16128=DIRECTION('ref_axis',(1.,0.,0.));
#16129=DIRECTION('center_axis',(0.,1.,0.));
#16130=DIRECTION('ref_axis',(1.,0.,0.));
#16131=DIRECTION('center_axis',(0.,1.,0.));
#16132=DIRECTION('ref_axis',(1.,0.,0.));
#16133=DIRECTION('center_axis',(0.,1.,0.));
#16134=DIRECTION('ref_axis',(1.,0.,0.));
#16135=DIRECTION('center_axis',(0.,1.,0.));
#16136=DIRECTION('ref_axis',(1.,0.,0.));
#16137=DIRECTION('center_axis',(0.,1.,0.));
#16138=DIRECTION('ref_axis',(1.,0.,0.));
#16139=DIRECTION('center_axis',(0.,1.,0.));
#16140=DIRECTION('ref_axis',(1.,0.,0.));
#16141=DIRECTION('center_axis',(0.,1.,0.));
#16142=DIRECTION('ref_axis',(1.,0.,0.));
#16143=DIRECTION('center_axis',(0.,1.,0.));
#16144=DIRECTION('ref_axis',(1.,0.,0.));
#16145=DIRECTION('center_axis',(0.,1.,0.));
#16146=DIRECTION('ref_axis',(1.,0.,0.));
#16147=DIRECTION('center_axis',(0.,1.,0.));
#16148=DIRECTION('ref_axis',(1.,0.,0.));
#16149=DIRECTION('center_axis',(0.,1.,0.));
#16150=DIRECTION('ref_axis',(1.,0.,0.));
#16151=DIRECTION('center_axis',(0.,1.,0.));
#16152=DIRECTION('ref_axis',(1.,0.,0.));
#16153=DIRECTION('center_axis',(0.,1.,0.));
#16154=DIRECTION('ref_axis',(1.,0.,0.));
#16155=DIRECTION('center_axis',(0.,1.,0.));
#16156=DIRECTION('ref_axis',(1.,0.,0.));
#16157=DIRECTION('center_axis',(0.,1.,0.));
#16158=DIRECTION('ref_axis',(1.,0.,0.));
#16159=DIRECTION('center_axis',(0.,1.,0.));
#16160=DIRECTION('ref_axis',(1.,0.,0.));
#16161=DIRECTION('center_axis',(0.,1.,0.));
#16162=DIRECTION('ref_axis',(1.,0.,0.));
#16163=DIRECTION('center_axis',(0.,1.,0.));
#16164=DIRECTION('ref_axis',(1.,0.,0.));
#16165=DIRECTION('center_axis',(0.,1.,0.));
#16166=DIRECTION('ref_axis',(1.,0.,0.));
#16167=DIRECTION('center_axis',(0.,1.,0.));
#16168=DIRECTION('ref_axis',(1.,0.,0.));
#16169=DIRECTION('center_axis',(0.,1.,0.));
#16170=DIRECTION('ref_axis',(1.,0.,0.));
#16171=DIRECTION('center_axis',(0.,1.,0.));
#16172=DIRECTION('ref_axis',(1.,0.,0.));
#16173=DIRECTION('center_axis',(0.,1.,0.));
#16174=DIRECTION('ref_axis',(1.,0.,0.));
#16175=DIRECTION('center_axis',(0.,1.,0.));
#16176=DIRECTION('ref_axis',(1.,0.,0.));
#16177=DIRECTION('center_axis',(0.,1.,0.));
#16178=DIRECTION('ref_axis',(1.,0.,0.));
#16179=DIRECTION('center_axis',(0.,1.,0.));
#16180=DIRECTION('ref_axis',(1.,0.,0.));
#16181=DIRECTION('center_axis',(0.,1.,0.));
#16182=DIRECTION('ref_axis',(1.,0.,0.));
#16183=DIRECTION('center_axis',(0.,1.,0.));
#16184=DIRECTION('ref_axis',(1.,0.,0.));
#16185=DIRECTION('center_axis',(0.,1.,0.));
#16186=DIRECTION('ref_axis',(1.,0.,0.));
#16187=DIRECTION('center_axis',(0.,1.,0.));
#16188=DIRECTION('ref_axis',(1.,0.,0.));
#16189=DIRECTION('center_axis',(0.,1.,0.));
#16190=DIRECTION('ref_axis',(1.,0.,0.));
#16191=DIRECTION('',(0.707106781186547,0.707106781186548,8.65956056235493E-17));
#16192=DIRECTION('center_axis',(0.,-1.,0.));
#16193=DIRECTION('ref_axis',(1.,0.,0.));
#16194=DIRECTION('center_axis',(-0.0691033627359896,0.,0.997609505397066));
#16195=DIRECTION('ref_axis',(-0.997609505397066,0.,-0.0691033627359896));
#16196=DIRECTION('',(0.,1.,0.));
#16197=DIRECTION('',(-0.997609505397066,0.,-0.0691033627359896));
#16198=DIRECTION('',(0.,-1.,0.));
#16199=DIRECTION('center_axis',(-0.694187276399492,0.,-0.719794432657725));
#16200=DIRECTION('ref_axis',(0.719794432657725,0.,-0.694187276399492));
#16201=DIRECTION('',(0.,-1.,0.));
#16202=DIRECTION('',(0.719794432657725,0.,-0.694187276399492));
#16203=DIRECTION('center_axis',(0.,-1.,0.));
#16204=DIRECTION('ref_axis',(-0.342020143325669,0.,-0.939692620785908));
#16205=DIRECTION('center_axis',(0.,-1.,0.));
#16206=DIRECTION('ref_axis',(1.,0.,0.));
#16207=DIRECTION('center_axis',(0.10517954525379,0.,0.994453248403466));
#16208=DIRECTION('ref_axis',(-0.994453248403466,0.,0.10517954525379));
#16209=DIRECTION('',(0.,1.,0.));
#16210=DIRECTION('',(-0.994453248403466,0.,0.10517954525379));
#16211=DIRECTION('',(0.,-1.,0.));
#16212=DIRECTION('center_axis',(-0.808632003366464,0.,-0.58831478235001));
#16213=DIRECTION('ref_axis',(0.58831478235001,0.,-0.808632003366464));
#16214=DIRECTION('',(0.,-1.,0.));
#16215=DIRECTION('',(0.58831478235001,0.,-0.808632003366464));
#16216=DIRECTION('center_axis',(0.,-1.,0.));
#16217=DIRECTION('ref_axis',(-0.5,0.,-0.866025403784438));
#16218=DIRECTION('center_axis',(0.,-1.,0.));
#16219=DIRECTION('ref_axis',(1.,0.,0.));
#16220=DIRECTION('center_axis',(0.276266625984452,0.,0.961081032674752));
#16221=DIRECTION('ref_axis',(-0.961081032674752,0.,0.276266625984452));
#16222=DIRECTION('',(0.,1.,0.));
#16223=DIRECTION('',(-0.961081032674752,0.,0.276266625984452));
#16224=DIRECTION('',(0.,-1.,0.));
#16225=DIRECTION('center_axis',(-0.898506856098683,0.,-0.438959485082234));
#16226=DIRECTION('ref_axis',(0.438959485082234,0.,-0.898506856098683));
#16227=DIRECTION('',(0.,-1.,0.));
#16228=DIRECTION('',(0.438959485082234,0.,-0.898506856098683));
#16229=DIRECTION('center_axis',(0.,-1.,0.));
#16230=DIRECTION('ref_axis',(-0.64278760968654,0.,-0.766044443118978));
#16231=DIRECTION('center_axis',(0.,-1.,0.));
#16232=DIRECTION('ref_axis',(1.,0.,0.));
#16233=DIRECTION('center_axis',(0.438959485082234,0.,0.898506856098683));
#16234=DIRECTION('ref_axis',(-0.898506856098683,0.,0.438959485082234));
#16235=DIRECTION('',(0.,1.,0.));
#16236=DIRECTION('',(-0.898506856098683,0.,0.438959485082234));
#16237=DIRECTION('',(0.,-1.,0.));
#16238=DIRECTION('center_axis',(-0.961081032674752,0.,-0.276266625984452));
#16239=DIRECTION('ref_axis',(0.276266625984452,0.,-0.961081032674752));
#16240=DIRECTION('',(0.,-1.,0.));
#16241=DIRECTION('',(0.276266625984452,0.,-0.961081032674752));
#16242=DIRECTION('center_axis',(0.,-1.,0.));
#16243=DIRECTION('ref_axis',(-0.766044443118978,0.,-0.642787609686539));
#16244=DIRECTION('center_axis',(0.,-1.,0.));
#16245=DIRECTION('ref_axis',(1.,0.,0.));
#16246=DIRECTION('center_axis',(0.58831478235001,0.,0.808632003366464));
#16247=DIRECTION('ref_axis',(-0.808632003366464,0.,0.58831478235001));
#16248=DIRECTION('',(0.,1.,0.));
#16249=DIRECTION('',(-0.808632003366464,0.,0.58831478235001));
#16250=DIRECTION('',(0.,-1.,0.));
#16251=DIRECTION('center_axis',(-0.994453248403466,0.,-0.10517954525379));
#16252=DIRECTION('ref_axis',(0.10517954525379,0.,-0.994453248403466));
#16253=DIRECTION('',(0.,-1.,0.));
#16254=DIRECTION('',(0.10517954525379,0.,-0.994453248403466));
#16255=DIRECTION('center_axis',(0.,-1.,0.));
#16256=DIRECTION('ref_axis',(-0.866025403784439,0.,-0.5));
#16257=DIRECTION('center_axis',(0.,-1.,0.));
#16258=DIRECTION('ref_axis',(1.,0.,0.));
#16259=DIRECTION('center_axis',(0.719794432657726,0.,0.694187276399491));
#16260=DIRECTION('ref_axis',(-0.694187276399491,0.,0.719794432657726));
#16261=DIRECTION('',(0.,1.,0.));
#16262=DIRECTION('',(-0.694187276399491,0.,0.719794432657726));
#16263=DIRECTION('',(0.,-1.,0.));
#16264=DIRECTION('center_axis',(-0.997609505397066,0.,0.0691033627359909));
#16265=DIRECTION('ref_axis',(-0.0691033627359909,0.,-0.997609505397066));
#16266=DIRECTION('',(0.,-1.,0.));
#16267=DIRECTION('',(-0.0691033627359909,0.,-0.997609505397066));
#16268=DIRECTION('center_axis',(0.,-1.,0.));
#16269=DIRECTION('ref_axis',(-0.939692620785909,0.,-0.342020143325668));
#16270=DIRECTION('center_axis',(0.,-1.,0.));
#16271=DIRECTION('ref_axis',(1.,0.,0.));
#16272=DIRECTION('center_axis',(0.829403493362693,0.,0.558650020314831));
#16273=DIRECTION('ref_axis',(-0.558650020314831,0.,0.829403493362693));
#16274=DIRECTION('',(0.,1.,0.));
#16275=DIRECTION('',(-0.558650020314831,0.,0.829403493362693));
#16276=DIRECTION('',(0.,-1.,0.));
#16277=DIRECTION('center_axis',(-0.970453902383943,0.,0.241286600017027));
#16278=DIRECTION('ref_axis',(-0.241286600017027,0.,-0.970453902383943));
#16279=DIRECTION('',(0.,-1.,0.));
#16280=DIRECTION('',(-0.241286600017027,0.,-0.970453902383943));
#16281=DIRECTION('center_axis',(0.,-1.,0.));
#16282=DIRECTION('ref_axis',(-0.984807753012208,0.,-0.17364817766693));
#16283=DIRECTION('center_axis',(0.,-1.,0.));
#16284=DIRECTION('ref_axis',(1.,0.,0.));
#16285=DIRECTION('center_axis',(0.913811548620253,0.,0.406138466053456));
#16286=DIRECTION('ref_axis',(-0.406138466053456,0.,0.913811548620253));
#16287=DIRECTION('',(0.,1.,0.));
#16288=DIRECTION('',(-0.406138466053456,0.,0.913811548620253));
#16289=DIRECTION('',(0.,-1.,0.));
#16290=DIRECTION('center_axis',(-0.913811548620253,0.,0.406138466053456));
#16291=DIRECTION('ref_axis',(-0.406138466053456,0.,-0.913811548620253));
#16292=DIRECTION('',(0.,-1.,0.));
#16293=DIRECTION('',(-0.406138466053456,0.,-0.913811548620253));
#16294=DIRECTION('center_axis',(0.,-1.,0.));
#16295=DIRECTION('ref_axis',(-1.,0.,1.83697019872103E-16));
#16296=DIRECTION('center_axis',(0.,-1.,0.));
#16297=DIRECTION('ref_axis',(1.,0.,0.));
#16298=DIRECTION('center_axis',(0.970453902383943,0.,0.241286600017026));
#16299=DIRECTION('ref_axis',(-0.241286600017026,0.,0.970453902383943));
#16300=DIRECTION('',(0.,1.,0.));
#16301=DIRECTION('',(-0.241286600017026,0.,0.970453902383943));
#16302=DIRECTION('',(0.,-1.,0.));
#16303=DIRECTION('center_axis',(-0.829403493362693,0.,0.558650020314831));
#16304=DIRECTION('ref_axis',(-0.558650020314831,0.,-0.829403493362693));
#16305=DIRECTION('',(0.,-1.,0.));
#16306=DIRECTION('',(-0.558650020314831,0.,-0.829403493362693));
#16307=DIRECTION('center_axis',(0.,-1.,0.));
#16308=DIRECTION('ref_axis',(-0.984807753012208,0.,0.17364817766693));
#16309=DIRECTION('center_axis',(0.,-1.,0.));
#16310=DIRECTION('ref_axis',(1.,0.,0.));
#16311=DIRECTION('center_axis',(0.997609505397066,0.,0.0691033627359897));
#16312=DIRECTION('ref_axis',(-0.0691033627359897,0.,0.997609505397066));
#16313=DIRECTION('',(0.,1.,0.));
#16314=DIRECTION('',(-0.0691033627359897,0.,0.997609505397066));
#16315=DIRECTION('',(0.,-1.,0.));
#16316=DIRECTION('center_axis',(-0.719794432657725,0.,0.694187276399492));
#16317=DIRECTION('ref_axis',(-0.694187276399492,0.,-0.719794432657725));
#16318=DIRECTION('',(0.,-1.,0.));
#16319=DIRECTION('',(-0.694187276399492,0.,-0.719794432657725));
#16320=DIRECTION('center_axis',(0.,-1.,0.));
#16321=DIRECTION('ref_axis',(-0.939692620785908,0.,0.342020143325669));
#16322=DIRECTION('center_axis',(0.,-1.,0.));
#16323=DIRECTION('ref_axis',(1.,0.,0.));
#16324=DIRECTION('center_axis',(0.994453248403466,0.,-0.10517954525379));
#16325=DIRECTION('ref_axis',(0.10517954525379,0.,0.994453248403466));
#16326=DIRECTION('',(0.,1.,0.));
#16327=DIRECTION('',(0.10517954525379,0.,0.994453248403466));
#16328=DIRECTION('',(0.,-1.,0.));
#16329=DIRECTION('center_axis',(-0.58831478235001,0.,0.808632003366464));
#16330=DIRECTION('ref_axis',(-0.808632003366464,0.,-0.58831478235001));
#16331=DIRECTION('',(0.,-1.,0.));
#16332=DIRECTION('',(-0.808632003366464,0.,-0.58831478235001));
#16333=DIRECTION('center_axis',(0.,-1.,0.));
#16334=DIRECTION('ref_axis',(-0.866025403784438,0.,0.5));
#16335=DIRECTION('center_axis',(0.,-1.,0.));
#16336=DIRECTION('ref_axis',(1.,0.,0.));
#16337=DIRECTION('center_axis',(0.961081032674752,0.,-0.276266625984452));
#16338=DIRECTION('ref_axis',(0.276266625984452,0.,0.961081032674752));
#16339=DIRECTION('',(0.,1.,0.));
#16340=DIRECTION('',(0.276266625984452,0.,0.961081032674752));
#16341=DIRECTION('',(0.,-1.,0.));
#16342=DIRECTION('center_axis',(-0.438959485082234,0.,0.898506856098683));
#16343=DIRECTION('ref_axis',(-0.898506856098683,0.,-0.438959485082234));
#16344=DIRECTION('',(0.,-1.,0.));
#16345=DIRECTION('',(-0.898506856098683,0.,-0.438959485082234));
#16346=DIRECTION('center_axis',(0.,-1.,0.));
#16347=DIRECTION('ref_axis',(-0.766044443118978,0.,0.642787609686539));
#16348=DIRECTION('center_axis',(0.,-1.,0.));
#16349=DIRECTION('ref_axis',(1.,0.,0.));
#16350=DIRECTION('center_axis',(0.898506856098683,0.,-0.438959485082234));
#16351=DIRECTION('ref_axis',(0.438959485082234,0.,0.898506856098683));
#16352=DIRECTION('',(0.,1.,0.));
#16353=DIRECTION('',(0.438959485082234,0.,0.898506856098683));
#16354=DIRECTION('',(0.,-1.,0.));
#16355=DIRECTION('center_axis',(-0.276266625984452,0.,0.961081032674752));
#16356=DIRECTION('ref_axis',(-0.961081032674752,0.,-0.276266625984452));
#16357=DIRECTION('',(0.,-1.,0.));
#16358=DIRECTION('',(-0.961081032674752,0.,-0.276266625984452));
#16359=DIRECTION('center_axis',(0.,-1.,0.));
#16360=DIRECTION('ref_axis',(-0.642787609686539,0.,0.766044443118978));
#16361=DIRECTION('center_axis',(0.,-1.,0.));
#16362=DIRECTION('ref_axis',(1.,0.,0.));
#16363=DIRECTION('center_axis',(0.808632003366463,0.,-0.58831478235001));
#16364=DIRECTION('ref_axis',(0.58831478235001,0.,0.808632003366463));
#16365=DIRECTION('',(0.,1.,0.));
#16366=DIRECTION('',(0.58831478235001,0.,0.808632003366463));
#16367=DIRECTION('',(0.,-1.,0.));
#16368=DIRECTION('center_axis',(-0.10517954525379,0.,0.994453248403466));
#16369=DIRECTION('ref_axis',(-0.994453248403466,0.,-0.10517954525379));
#16370=DIRECTION('',(0.,-1.,0.));
#16371=DIRECTION('',(-0.994453248403466,0.,-0.10517954525379));
#16372=DIRECTION('center_axis',(0.,-1.,0.));
#16373=DIRECTION('ref_axis',(-0.5,0.,0.866025403784439));
#16374=DIRECTION('center_axis',(0.,-1.,0.));
#16375=DIRECTION('ref_axis',(1.,0.,0.));
#16376=DIRECTION('center_axis',(0.694187276399491,0.,-0.719794432657725));
#16377=DIRECTION('ref_axis',(0.719794432657725,0.,0.694187276399491));
#16378=DIRECTION('',(0.,1.,0.));
#16379=DIRECTION('',(0.719794432657725,0.,0.694187276399491));
#16380=DIRECTION('',(0.,-1.,0.));
#16381=DIRECTION('center_axis',(0.0691033627359905,0.,0.997609505397066));
#16382=DIRECTION('ref_axis',(-0.997609505397066,0.,0.0691033627359905));
#16383=DIRECTION('',(0.,-1.,0.));
#16384=DIRECTION('',(-0.997609505397066,0.,0.0691033627359905));
#16385=DIRECTION('center_axis',(0.,-1.,0.));
#16386=DIRECTION('ref_axis',(-0.342020143325669,0.,0.939692620785908));
#16387=DIRECTION('center_axis',(0.,-1.,0.));
#16388=DIRECTION('ref_axis',(1.,0.,0.));
#16389=DIRECTION('center_axis',(0.558650020314831,0.,-0.829403493362693));
#16390=DIRECTION('ref_axis',(0.829403493362693,0.,0.558650020314831));
#16391=DIRECTION('',(0.,1.,0.));
#16392=DIRECTION('',(0.829403493362693,0.,0.558650020314831));
#16393=DIRECTION('',(0.,-1.,0.));
#16394=DIRECTION('center_axis',(0.241286600017027,0.,0.970453902383943));
#16395=DIRECTION('ref_axis',(-0.970453902383943,0.,0.241286600017027));
#16396=DIRECTION('',(0.,-1.,0.));
#16397=DIRECTION('',(-0.970453902383943,0.,0.241286600017027));
#16398=DIRECTION('center_axis',(0.,-1.,0.));
#16399=DIRECTION('ref_axis',(-0.17364817766693,0.,0.984807753012208));
#16400=DIRECTION('center_axis',(0.,-1.,0.));
#16401=DIRECTION('ref_axis',(1.,0.,0.));
#16402=DIRECTION('center_axis',(0.406138466053456,0.,-0.913811548620253));
#16403=DIRECTION('ref_axis',(0.913811548620253,0.,0.406138466053456));
#16404=DIRECTION('',(0.,1.,0.));
#16405=DIRECTION('',(0.913811548620253,0.,0.406138466053456));
#16406=DIRECTION('',(0.,-1.,0.));
#16407=DIRECTION('center_axis',(0.406138466053456,0.,0.913811548620253));
#16408=DIRECTION('ref_axis',(-0.913811548620253,0.,0.406138466053456));
#16409=DIRECTION('',(0.,-1.,0.));
#16410=DIRECTION('',(-0.913811548620253,0.,0.406138466053456));
#16411=DIRECTION('center_axis',(0.,-1.,0.));
#16412=DIRECTION('ref_axis',(1.22464679914735E-16,0.,1.));
#16413=DIRECTION('center_axis',(0.,-1.,0.));
#16414=DIRECTION('ref_axis',(1.,0.,0.));
#16415=DIRECTION('center_axis',(0.,-1.,0.));
#16416=DIRECTION('ref_axis',(1.,0.,0.));
#16417=DIRECTION('center_axis',(0.241286600017026,0.,-0.970453902383943));
#16418=DIRECTION('ref_axis',(0.970453902383943,0.,0.241286600017026));
#16419=DIRECTION('',(0.,1.,0.));
#16420=DIRECTION('',(0.970453902383943,0.,0.241286600017026));
#16421=DIRECTION('',(0.,-1.,0.));
#16422=DIRECTION('center_axis',(0.558650020314832,0.,0.829403493362693));
#16423=DIRECTION('ref_axis',(-0.829403493362693,0.,0.558650020314832));
#16424=DIRECTION('',(0.,-1.,0.));
#16425=DIRECTION('',(-0.829403493362692,0.,0.558650020314832));
#16426=DIRECTION('center_axis',(0.,-1.,0.));
#16427=DIRECTION('ref_axis',(0.173648177666931,0.,0.984807753012208));
#16428=DIRECTION('center_axis',(0.,-1.,0.));
#16429=DIRECTION('ref_axis',(1.,0.,0.));
#16430=DIRECTION('center_axis',(0.0691033627359902,0.,-0.997609505397066));
#16431=DIRECTION('ref_axis',(0.997609505397066,0.,0.0691033627359902));
#16432=DIRECTION('',(0.,1.,0.));
#16433=DIRECTION('',(0.997609505397066,0.,0.0691033627359902));
#16434=DIRECTION('',(0.,-1.,0.));
#16435=DIRECTION('center_axis',(0.694187276399491,0.,0.719794432657725));
#16436=DIRECTION('ref_axis',(-0.719794432657725,0.,0.694187276399491));
#16437=DIRECTION('',(0.,-1.,0.));
#16438=DIRECTION('',(-0.719794432657725,0.,0.694187276399491));
#16439=DIRECTION('center_axis',(0.,-1.,0.));
#16440=DIRECTION('ref_axis',(0.342020143325669,0.,0.939692620785908));
#16441=DIRECTION('center_axis',(0.,-1.,0.));
#16442=DIRECTION('ref_axis',(1.,0.,0.));
#16443=DIRECTION('center_axis',(-0.10517954525379,0.,-0.994453248403466));
#16444=DIRECTION('ref_axis',(0.994453248403466,0.,-0.10517954525379));
#16445=DIRECTION('',(0.,1.,0.));
#16446=DIRECTION('',(0.994453248403466,0.,-0.10517954525379));
#16447=DIRECTION('',(0.,-1.,0.));
#16448=DIRECTION('center_axis',(0.808632003366463,0.,0.58831478235001));
#16449=DIRECTION('ref_axis',(-0.58831478235001,0.,0.808632003366463));
#16450=DIRECTION('',(0.,-1.,0.));
#16451=DIRECTION('',(-0.58831478235001,0.,0.808632003366463));
#16452=DIRECTION('center_axis',(0.,-1.,0.));
#16453=DIRECTION('ref_axis',(0.5,0.,0.866025403784439));
#16454=DIRECTION('center_axis',(0.,-1.,0.));
#16455=DIRECTION('ref_axis',(1.,0.,0.));
#16456=DIRECTION('center_axis',(-0.276266625984452,0.,-0.961081032674752));
#16457=DIRECTION('ref_axis',(0.961081032674752,0.,-0.276266625984452));
#16458=DIRECTION('',(0.,1.,0.));
#16459=DIRECTION('',(0.961081032674752,0.,-0.276266625984452));
#16460=DIRECTION('',(0.,-1.,0.));
#16461=DIRECTION('center_axis',(0.898506856098683,0.,0.438959485082234));
#16462=DIRECTION('ref_axis',(-0.438959485082234,0.,0.898506856098683));
#16463=DIRECTION('',(0.,-1.,0.));
#16464=DIRECTION('',(-0.438959485082234,0.,0.898506856098683));
#16465=DIRECTION('center_axis',(0.,-1.,0.));
#16466=DIRECTION('ref_axis',(0.642787609686539,0.,0.766044443118978));
#16467=DIRECTION('center_axis',(0.,-1.,0.));
#16468=DIRECTION('ref_axis',(1.,0.,0.));
#16469=DIRECTION('center_axis',(-0.438959485082234,0.,-0.898506856098683));
#16470=DIRECTION('ref_axis',(0.898506856098683,0.,-0.438959485082234));
#16471=DIRECTION('',(0.,1.,0.));
#16472=DIRECTION('',(0.898506856098683,0.,-0.438959485082234));
#16473=DIRECTION('',(0.,-1.,0.));
#16474=DIRECTION('center_axis',(0.961081032674752,0.,0.276266625984452));
#16475=DIRECTION('ref_axis',(-0.276266625984452,0.,0.961081032674752));
#16476=DIRECTION('',(0.,-1.,0.));
#16477=DIRECTION('',(-0.276266625984452,0.,0.961081032674752));
#16478=DIRECTION('center_axis',(0.,-1.,0.));
#16479=DIRECTION('ref_axis',(0.766044443118978,0.,0.642787609686539));
#16480=DIRECTION('center_axis',(0.,-1.,0.));
#16481=DIRECTION('ref_axis',(1.,0.,0.));
#16482=DIRECTION('center_axis',(-0.58831478235001,0.,-0.808632003366463));
#16483=DIRECTION('ref_axis',(0.808632003366463,0.,-0.58831478235001));
#16484=DIRECTION('',(0.,1.,0.));
#16485=DIRECTION('',(0.808632003366463,0.,-0.58831478235001));
#16486=DIRECTION('',(0.,-1.,0.));
#16487=DIRECTION('center_axis',(0.994453248403466,0.,0.10517954525379));
#16488=DIRECTION('ref_axis',(-0.10517954525379,0.,0.994453248403466));
#16489=DIRECTION('',(0.,-1.,0.));
#16490=DIRECTION('',(-0.10517954525379,0.,0.994453248403466));
#16491=DIRECTION('center_axis',(0.,-1.,0.));
#16492=DIRECTION('ref_axis',(0.866025403784439,0.,0.5));
#16493=DIRECTION('center_axis',(0.,-1.,0.));
#16494=DIRECTION('ref_axis',(1.,0.,0.));
#16495=DIRECTION('center_axis',(-0.719794432657725,0.,-0.694187276399491));
#16496=DIRECTION('ref_axis',(0.694187276399491,0.,-0.719794432657725));
#16497=DIRECTION('',(0.,1.,0.));
#16498=DIRECTION('',(0.694187276399491,0.,-0.719794432657725));
#16499=DIRECTION('',(0.,-1.,0.));
#16500=DIRECTION('center_axis',(0.997609505397066,0.,-0.0691033627359904));
#16501=DIRECTION('ref_axis',(0.0691033627359904,0.,0.997609505397066));
#16502=DIRECTION('',(0.,-1.,0.));
#16503=DIRECTION('',(0.0691033627359904,0.,0.997609505397066));
#16504=DIRECTION('center_axis',(0.,-1.,0.));
#16505=DIRECTION('ref_axis',(0.939692620785908,0.,0.342020143325669));
#16506=DIRECTION('center_axis',(0.,-1.,0.));
#16507=DIRECTION('ref_axis',(1.,0.,0.));
#16508=DIRECTION('center_axis',(-0.829403493362693,0.,-0.558650020314831));
#16509=DIRECTION('ref_axis',(0.558650020314831,0.,-0.829403493362693));
#16510=DIRECTION('',(0.,1.,0.));
#16511=DIRECTION('',(0.558650020314831,0.,-0.829403493362693));
#16512=DIRECTION('',(0.,-1.,0.));
#16513=DIRECTION('center_axis',(0.970453902383943,0.,-0.241286600017027));
#16514=DIRECTION('ref_axis',(0.241286600017027,0.,0.970453902383943));
#16515=DIRECTION('',(0.,-1.,0.));
#16516=DIRECTION('',(0.241286600017026,0.,0.970453902383943));
#16517=DIRECTION('center_axis',(0.,-1.,0.));
#16518=DIRECTION('ref_axis',(0.984807753012208,0.,0.17364817766693));
#16519=DIRECTION('center_axis',(0.,-1.,0.));
#16520=DIRECTION('ref_axis',(1.,0.,0.));
#16521=DIRECTION('center_axis',(-0.913811548620253,0.,-0.406138466053456));
#16522=DIRECTION('ref_axis',(0.406138466053456,0.,-0.913811548620253));
#16523=DIRECTION('',(0.,1.,0.));
#16524=DIRECTION('',(0.406138466053456,0.,-0.913811548620253));
#16525=DIRECTION('',(0.,-1.,0.));
#16526=DIRECTION('center_axis',(0.913811548620253,0.,-0.406138466053456));
#16527=DIRECTION('ref_axis',(0.406138466053456,0.,0.913811548620253));
#16528=DIRECTION('',(0.,-1.,0.));
#16529=DIRECTION('',(0.406138466053456,0.,0.913811548620253));
#16530=DIRECTION('center_axis',(0.,-1.,0.));
#16531=DIRECTION('ref_axis',(1.,0.,-6.12323399573677E-17));
#16532=DIRECTION('center_axis',(0.,-1.,0.));
#16533=DIRECTION('ref_axis',(1.,0.,0.));
#16534=DIRECTION('center_axis',(-0.970453902383943,0.,-0.241286600017026));
#16535=DIRECTION('ref_axis',(0.241286600017026,0.,-0.970453902383943));
#16536=DIRECTION('',(0.,1.,0.));
#16537=DIRECTION('',(0.241286600017026,0.,-0.970453902383943));
#16538=DIRECTION('',(0.,-1.,0.));
#16539=DIRECTION('center_axis',(0.829403493362693,0.,-0.558650020314832));
#16540=DIRECTION('ref_axis',(0.558650020314832,0.,0.829403493362693));
#16541=DIRECTION('',(0.,-1.,0.));
#16542=DIRECTION('',(0.558650020314832,0.,0.829403493362693));
#16543=DIRECTION('center_axis',(0.,-1.,0.));
#16544=DIRECTION('ref_axis',(0.984807753012208,0.,-0.17364817766693));
#16545=DIRECTION('center_axis',(0.,-1.,0.));
#16546=DIRECTION('ref_axis',(1.,0.,0.));
#16547=DIRECTION('center_axis',(-0.997609505397066,0.,-0.0691033627359903));
#16548=DIRECTION('ref_axis',(0.0691033627359903,0.,-0.997609505397066));
#16549=DIRECTION('',(0.,1.,0.));
#16550=DIRECTION('',(0.0691033627359903,0.,-0.997609505397066));
#16551=DIRECTION('',(0.,-1.,0.));
#16552=DIRECTION('center_axis',(0.719794432657725,0.,-0.694187276399491));
#16553=DIRECTION('ref_axis',(0.694187276399491,0.,0.719794432657725));
#16554=DIRECTION('',(0.,-1.,0.));
#16555=DIRECTION('',(0.694187276399491,0.,0.719794432657725));
#16556=DIRECTION('center_axis',(0.,-1.,0.));
#16557=DIRECTION('ref_axis',(0.939692620785908,0.,-0.342020143325669));
#16558=DIRECTION('center_axis',(0.,-1.,0.));
#16559=DIRECTION('ref_axis',(1.,0.,0.));
#16560=DIRECTION('center_axis',(-0.994453248403466,0.,0.10517954525379));
#16561=DIRECTION('ref_axis',(-0.10517954525379,0.,-0.994453248403466));
#16562=DIRECTION('',(0.,1.,0.));
#16563=DIRECTION('',(-0.10517954525379,0.,-0.994453248403466));
#16564=DIRECTION('',(0.,-1.,0.));
#16565=DIRECTION('center_axis',(0.58831478235001,0.,-0.808632003366464));
#16566=DIRECTION('ref_axis',(0.808632003366464,0.,0.58831478235001));
#16567=DIRECTION('',(0.,-1.,0.));
#16568=DIRECTION('',(0.808632003366464,0.,0.58831478235001));
#16569=DIRECTION('center_axis',(0.,-1.,0.));
#16570=DIRECTION('ref_axis',(0.866025403784439,0.,-0.5));
#16571=DIRECTION('center_axis',(0.,-1.,0.));
#16572=DIRECTION('ref_axis',(1.,0.,0.));
#16573=DIRECTION('center_axis',(-0.961081032674752,0.,0.276266625984452));
#16574=DIRECTION('ref_axis',(-0.276266625984452,0.,-0.961081032674752));
#16575=DIRECTION('',(0.,1.,0.));
#16576=DIRECTION('',(-0.276266625984452,0.,-0.961081032674752));
#16577=DIRECTION('',(0.,-1.,0.));
#16578=DIRECTION('center_axis',(0.438959485082234,0.,-0.898506856098683));
#16579=DIRECTION('ref_axis',(0.898506856098683,0.,0.438959485082234));
#16580=DIRECTION('',(0.,-1.,0.));
#16581=DIRECTION('',(0.898506856098683,0.,0.438959485082234));
#16582=DIRECTION('center_axis',(0.,-1.,0.));
#16583=DIRECTION('ref_axis',(0.766044443118978,0.,-0.642787609686539));
#16584=DIRECTION('center_axis',(0.,-1.,0.));
#16585=DIRECTION('ref_axis',(1.,0.,0.));
#16586=DIRECTION('center_axis',(-0.898506856098683,0.,0.438959485082234));
#16587=DIRECTION('ref_axis',(-0.438959485082234,0.,-0.898506856098683));
#16588=DIRECTION('',(0.,1.,0.));
#16589=DIRECTION('',(-0.438959485082234,0.,-0.898506856098683));
#16590=DIRECTION('',(0.,-1.,0.));
#16591=DIRECTION('center_axis',(0.276266625984452,0.,-0.961081032674752));
#16592=DIRECTION('ref_axis',(0.961081032674752,0.,0.276266625984452));
#16593=DIRECTION('',(0.,-1.,0.));
#16594=DIRECTION('',(0.961081032674752,0.,0.276266625984452));
#16595=DIRECTION('center_axis',(0.,-1.,0.));
#16596=DIRECTION('ref_axis',(0.642787609686539,0.,-0.766044443118978));
#16597=DIRECTION('center_axis',(0.,-1.,0.));
#16598=DIRECTION('ref_axis',(1.,0.,0.));
#16599=DIRECTION('center_axis',(-0.808632003366463,0.,0.58831478235001));
#16600=DIRECTION('ref_axis',(-0.58831478235001,0.,-0.808632003366463));
#16601=DIRECTION('',(0.,1.,0.));
#16602=DIRECTION('',(-0.58831478235001,0.,-0.808632003366463));
#16603=DIRECTION('',(0.,-1.,0.));
#16604=DIRECTION('center_axis',(0.10517954525379,0.,-0.994453248403466));
#16605=DIRECTION('ref_axis',(0.994453248403466,0.,0.10517954525379));
#16606=DIRECTION('',(0.,-1.,0.));
#16607=DIRECTION('',(0.994453248403466,0.,0.10517954525379));
#16608=DIRECTION('center_axis',(0.,-1.,0.));
#16609=DIRECTION('ref_axis',(0.5,0.,-0.866025403784439));
#16610=DIRECTION('center_axis',(0.,-1.,0.));
#16611=DIRECTION('ref_axis',(1.,0.,0.));
#16612=DIRECTION('center_axis',(-0.694187276399491,0.,0.719794432657725));
#16613=DIRECTION('ref_axis',(-0.719794432657725,0.,-0.694187276399491));
#16614=DIRECTION('',(0.,1.,0.));
#16615=DIRECTION('',(-0.719794432657725,0.,-0.694187276399491));
#16616=DIRECTION('',(0.,-1.,0.));
#16617=DIRECTION('center_axis',(-0.0691033627359904,0.,-0.997609505397066));
#16618=DIRECTION('ref_axis',(0.997609505397066,0.,-0.0691033627359904));
#16619=DIRECTION('',(0.,-1.,0.));
#16620=DIRECTION('',(0.997609505397066,0.,-0.0691033627359904));
#16621=DIRECTION('center_axis',(0.,-1.,0.));
#16622=DIRECTION('ref_axis',(0.342020143325669,0.,-0.939692620785908));
#16623=DIRECTION('center_axis',(0.,-1.,0.));
#16624=DIRECTION('ref_axis',(1.,0.,0.));
#16625=DIRECTION('center_axis',(-0.558650020314831,0.,0.829403493362693));
#16626=DIRECTION('ref_axis',(-0.829403493362693,0.,-0.558650020314831));
#16627=DIRECTION('',(0.,1.,0.));
#16628=DIRECTION('',(-0.829403493362693,0.,-0.558650020314831));
#16629=DIRECTION('',(0.,-1.,0.));
#16630=DIRECTION('center_axis',(-0.241286600017026,0.,-0.970453902383943));
#16631=DIRECTION('ref_axis',(0.970453902383943,0.,-0.241286600017026));
#16632=DIRECTION('',(0.,-1.,0.));
#16633=DIRECTION('',(0.970453902383943,0.,-0.241286600017026));
#16634=DIRECTION('center_axis',(0.,-1.,0.));
#16635=DIRECTION('ref_axis',(0.17364817766693,0.,-0.984807753012208));
#16636=DIRECTION('center_axis',(0.,-1.,0.));
#16637=DIRECTION('ref_axis',(1.,0.,0.));
#16638=DIRECTION('center_axis',(-0.406138466053456,0.,0.913811548620253));
#16639=DIRECTION('ref_axis',(-0.913811548620253,0.,-0.406138466053456));
#16640=DIRECTION('',(0.,1.,0.));
#16641=DIRECTION('',(-0.913811548620253,0.,-0.406138466053456));
#16642=DIRECTION('',(0.,-1.,0.));
#16643=DIRECTION('center_axis',(-0.406138466053456,0.,-0.913811548620253));
#16644=DIRECTION('ref_axis',(0.913811548620253,0.,-0.406138466053456));
#16645=DIRECTION('',(0.,-1.,0.));
#16646=DIRECTION('',(0.913811548620253,0.,-0.406138466053456));
#16647=DIRECTION('center_axis',(0.,-1.,0.));
#16648=DIRECTION('ref_axis',(0.,0.,-1.));
#16649=DIRECTION('center_axis',(0.,-1.,0.));
#16650=DIRECTION('ref_axis',(1.,0.,0.));
#16651=DIRECTION('center_axis',(0.,1.,0.));
#16652=DIRECTION('ref_axis',(1.,0.,0.));
#16653=DIRECTION('',(0.,-1.,0.));
#16654=DIRECTION('center_axis',(0.,1.,0.));
#16655=DIRECTION('ref_axis',(1.,0.,0.));
#16656=DIRECTION('',(0.499999999999998,0.,-0.86602540378444));
#16657=DIRECTION('',(1.,0.,0.));
#16658=DIRECTION('',(0.499999999999998,0.,0.86602540378444));
#16659=DIRECTION('',(-0.499999999999998,0.,0.86602540378444));
#16660=DIRECTION('',(-1.,0.,0.));
#16661=DIRECTION('',(-0.499999999999998,0.,-0.86602540378444));
#16662=DIRECTION('center_axis',(0.,1.,0.));
#16663=DIRECTION('ref_axis',(0.,0.,1.));
#16664=DIRECTION('',(0.499999999999998,0.,-0.86602540378444));
#16665=DIRECTION('center_axis',(0.,-1.,0.));
#16666=DIRECTION('ref_axis',(1.,0.,0.));
#16667=DIRECTION('center_axis',(0.,1.,0.));
#16668=DIRECTION('ref_axis',(0.,0.,1.));
#16669=DIRECTION('',(1.,0.,0.));
#16670=DIRECTION('center_axis',(0.,-1.,0.));
#16671=DIRECTION('ref_axis',(1.,0.,0.));
#16672=DIRECTION('center_axis',(0.,1.,0.));
#16673=DIRECTION('ref_axis',(0.,0.,1.));
#16674=DIRECTION('',(0.499999999999998,0.,0.86602540378444));
#16675=DIRECTION('center_axis',(0.,-1.,0.));
#16676=DIRECTION('ref_axis',(1.,0.,0.));
#16677=DIRECTION('center_axis',(0.,1.,0.));
#16678=DIRECTION('ref_axis',(0.,0.,1.));
#16679=DIRECTION('',(-0.499999999999998,0.,0.86602540378444));
#16680=DIRECTION('center_axis',(0.,-1.,0.));
#16681=DIRECTION('ref_axis',(1.,0.,0.));
#16682=DIRECTION('center_axis',(0.,1.,0.));
#16683=DIRECTION('ref_axis',(0.,0.,1.));
#16684=DIRECTION('',(-1.,0.,0.));
#16685=DIRECTION('center_axis',(0.,-1.,0.));
#16686=DIRECTION('ref_axis',(1.,0.,0.));
#16687=DIRECTION('center_axis',(0.,1.,0.));
#16688=DIRECTION('ref_axis',(0.,0.,1.));
#16689=DIRECTION('',(-0.499999999999998,0.,-0.86602540378444));
#16690=DIRECTION('center_axis',(0.,-1.,0.));
#16691=DIRECTION('ref_axis',(1.,0.,0.));
#16692=DIRECTION('center_axis',(0.,1.,0.));
#16693=DIRECTION('ref_axis',(1.,0.,0.));
#16694=DIRECTION('',(-0.85716730070211,0.515038074910058,1.04972719113862E-16));
#16695=DIRECTION('center_axis',(-0.86602540378444,0.,-0.499999999999998));
#16696=DIRECTION('ref_axis',(0.499999999999998,0.,-0.86602540378444));
#16697=DIRECTION('',(0.,-1.,0.));
#16698=DIRECTION('',(0.,-1.,0.));
#16699=DIRECTION('center_axis',(-0.86602540378444,0.,0.499999999999998));
#16700=DIRECTION('ref_axis',(-0.499999999999998,0.,-0.86602540378444));
#16701=DIRECTION('',(0.,-1.,0.));
#16702=DIRECTION('center_axis',(0.,0.,1.));
#16703=DIRECTION('ref_axis',(-1.,0.,0.));
#16704=DIRECTION('',(0.,-1.,0.));
#16705=DIRECTION('center_axis',(0.86602540378444,0.,0.499999999999998));
#16706=DIRECTION('ref_axis',(-0.499999999999998,0.,0.86602540378444));
#16707=DIRECTION('',(0.,-1.,0.));
#16708=DIRECTION('center_axis',(0.86602540378444,0.,-0.499999999999998));
#16709=DIRECTION('ref_axis',(0.499999999999998,0.,0.86602540378444));
#16710=DIRECTION('',(0.,-1.,0.));
#16711=DIRECTION('center_axis',(0.,0.,-1.));
#16712=DIRECTION('ref_axis',(1.,0.,0.));
#19891=CARTESIAN_POINT('',(0.,0.,0.));
#19892=CARTESIAN_POINT('Origin',(42.4,48.4493818343519,48.));
#19893=CARTESIAN_POINT('',(41.7941388317924,46.4519835383214,49.8315225365138));
#19894=CARTESIAN_POINT('',(41.7941388317924,46.6231654538532,49.8315225365138));
#19895=CARTESIAN_POINT('',(41.7941388317924,48.4493818343519,49.8315225365138));
#19896=CARTESIAN_POINT('',(41.191723663621,46.9748,46.4961346962422));
#19897=CARTESIAN_POINT('Ctrl Pts',(41.191723663621,46.9748,46.4961346962422));
#19898=CARTESIAN_POINT('Ctrl Pts',(41.1983691281237,46.9742382770361,46.4907954165322));
#19899=CARTESIAN_POINT('Ctrl Pts',(41.2050496865336,46.9736765540721,46.4855004235829));
#19900=CARTESIAN_POINT('Ctrl Pts',(41.2117649567869,46.9731148311082,46.480250007738));
#19901=CARTESIAN_POINT('Ctrl Pts',(41.2650801043383,46.968655093588,46.438564910204));
#19902=CARTESIAN_POINT('Ctrl Pts',(41.3206975739893,46.9641953560677,46.3996058162976));
#19903=CARTESIAN_POINT('Ctrl Pts',(41.3783074070676,46.9597356185475,46.3636361032927));
#19904=CARTESIAN_POINT('Ctrl Pts',(41.4358295661938,46.955282668112,46.3277211310625));
#19905=CARTESIAN_POINT('Ctrl Pts',(41.4953376565687,46.9508297176764,46.2947867697778));
#19906=CARTESIAN_POINT('Ctrl Pts',(41.5564898960424,46.9463767672408,46.2650552569545));
#19907=CARTESIAN_POINT('Ctrl Pts',(41.617568923949,46.9419291478852,46.2353593387498));
#19908=CARTESIAN_POINT('Ctrl Pts',(41.6802877505718,46.9374815285296,46.2088588680115));
#19909=CARTESIAN_POINT('Ctrl Pts',(41.74427854964,46.933033909174,46.1857310187192));
#19910=CARTESIAN_POINT('Ctrl Pts',(41.8082284267617,46.9285891340592,46.1626179596253));
#19911=CARTESIAN_POINT('Ctrl Pts',(41.8734482003687,46.9241443589444,46.142873410735));
#19912=CARTESIAN_POINT('Ctrl Pts',(41.939549990011,46.9196995838296,46.126626480063));
#19913=CARTESIAN_POINT('Ctrl Pts',(42.0056322514933,46.9152561218151,46.1103843491501));
#19914=CARTESIAN_POINT('Ctrl Pts',(42.0725955334245,46.9108126598006,46.0976379027819));
#19915=CARTESIAN_POINT('Ctrl Pts',(42.1400384824014,46.9063691977861,46.0884659128679));
#19916=CARTESIAN_POINT('Ctrl Pts',(42.2074847113698,46.9019255196702,46.0792934768873));
#19917=CARTESIAN_POINT('Ctrl Pts',(42.2754101650517,46.8974818415542,46.0736959063333));
#19918=CARTESIAN_POINT('Ctrl Pts',(42.3434068477991,46.8930381634383,46.0717002898865));
#19919=CARTESIAN_POINT('Ctrl Pts',(42.4114747425737,46.888589831517,46.0697025834569));
#19920=CARTESIAN_POINT('Ctrl Pts',(42.4796135217653,46.8841414995957,46.071314373904));
#19921=CARTESIAN_POINT('Ctrl Pts',(42.5474146977834,46.8796931676744,46.0765106021146));
#19922=CARTESIAN_POINT('Ctrl Pts',(42.6152559711119,46.8752422050296,46.0817099033512));
#19923=CARTESIAN_POINT('Ctrl Pts',(42.6827587551109,46.8707912423849,46.0904977979093));
#19924=CARTESIAN_POINT('Ctrl Pts',(42.7495220026355,46.8663402797401,46.1027976052688));
#19925=CARTESIAN_POINT('Ctrl Pts',(42.8163991049541,46.8618817266401,46.1151183881214));
#19926=CARTESIAN_POINT('Ctrl Pts',(42.8825336747408,46.8574231735402,46.1309629220749));
#19927=CARTESIAN_POINT('Ctrl Pts',(42.9475380138215,46.8529646204403,46.1502041517183));
#19928=CARTESIAN_POINT('Ctrl Pts',(42.9770644780014,46.8509394431943,46.1589439602583));
#19929=CARTESIAN_POINT('Ctrl Pts',(43.0063580080931,46.8489142659483,46.1683839025424));
#19930=CARTESIAN_POINT('Ctrl Pts',(43.0353837115926,46.8468890887023,46.1785088262792));
#19931=CARTESIAN_POINT('Ctrl Pts',(43.0993551412968,46.8424256832301,46.200823732345));
#19932=CARTESIAN_POINT('Ctrl Pts',(43.1622728061311,46.837962277758,46.2265557417306));
#19933=CARTESIAN_POINT('Ctrl Pts',(43.2237472171988,46.8334988722859,46.2555851757517));
#19934=CARTESIAN_POINT('Ctrl Pts',(43.285130739502,46.8290420658751,46.2845716902987));
#19935=CARTESIAN_POINT('Ctrl Pts',(43.3450748018767,46.8245852594642,46.3168457449076));
#19936=CARTESIAN_POINT('Ctrl Pts',(43.4032074881356,46.8201284530534,46.3522387027701));
#19937=CARTESIAN_POINT('Ctrl Pts',(43.4612740279245,46.8156767178346,46.3875913886381));
#19938=CARTESIAN_POINT('Ctrl Pts',(43.517532866745,46.8112249826158,46.4260556750136));
#19939=CARTESIAN_POINT('Ctrl Pts',(43.571636046414,46.8067732473969,46.4674167129832));
#19940=CARTESIAN_POINT('Ctrl Pts',(43.62570659323,46.802324197285,46.508752803645));
#19941=CARTESIAN_POINT('Ctrl Pts',(43.6776236703527,46.7978751471731,46.5529818816755));
#19942=CARTESIAN_POINT('Ctrl Pts',(43.7270690426102,46.7934260970611,46.5998463252037));
#19943=CARTESIAN_POINT('Ctrl Pts',(43.7765015193754,46.788978207274,46.646698546353));
#19944=CARTESIAN_POINT('Ctrl Pts',(43.8234632143047,46.7845303174869,46.696184430213));
#19945=CARTESIAN_POINT('Ctrl Pts',(43.8676710594111,46.7800824276997,46.748007900078));
#19946=CARTESIAN_POINT('Ctrl Pts',(43.9118825092414,46.77563417523,46.7998355956478));
#19947=CARTESIAN_POINT('Ctrl Pts',(43.9533393462278,46.7711859227603,46.8540008797944));
#19948=CARTESIAN_POINT('Ctrl Pts',(43.9917984724335,46.7667376702906,46.9101742432579));
#19949=CARTESIAN_POINT('Ctrl Pts',(44.0302994859557,46.7622845730577,46.9664087872965));
#19950=CARTESIAN_POINT('Ctrl Pts',(44.0657959949355,46.7578314758248,47.0246553685409));
#19951=CARTESIAN_POINT('Ctrl Pts',(44.0980885597473,46.7533783785919,47.0845559546562));
#19952=CARTESIAN_POINT('Ctrl Pts',(44.130401043843,46.748922534519,47.1444934897343));
#19953=CARTESIAN_POINT('Ctrl Pts',(44.1595054403871,46.7444666904462,47.2060866154888));
#19954=CARTESIAN_POINT('Ctrl Pts',(44.1852498026584,46.7400108463733,47.2689557475719));
#19955=CARTESIAN_POINT('Ctrl Pts',(44.2110387609674,46.7355472836011,47.3319337856032));
#19956=CARTESIAN_POINT('Ctrl Pts',(44.2334559068194,46.731083720829,47.3961917773044));
#19957=CARTESIAN_POINT('Ctrl Pts',(44.2523989130009,46.7266201580569,47.4613342186354));
#19958=CARTESIAN_POINT('Ctrl Pts',(44.2608256584626,46.7246345541367,47.490312658836));
#19959=CARTESIAN_POINT('Ctrl Pts',(44.2685655868985,46.7226489502166,47.5194659812589));
#19960=CARTESIAN_POINT('Ctrl Pts',(44.2756129660321,46.7206633462965,47.5487588687272));
#19961=CARTESIAN_POINT('Ctrl Pts',(44.2914115935473,46.7162120721231,47.6144268864664));
#19962=CARTESIAN_POINT('Ctrl Pts',(44.3037895859002,46.7117607979497,47.6810596925127));
#19963=CARTESIAN_POINT('Ctrl Pts',(44.3126351888968,46.7073095237764,47.7482676200929));
#19964=CARTESIAN_POINT('Ctrl Pts',(44.3214672302742,46.7028650740655,47.8153725079679));
#19965=CARTESIAN_POINT('Ctrl Pts',(44.3267775648675,46.6984206243546,47.8830502810582));
#19966=CARTESIAN_POINT('Ctrl Pts',(44.3285050353862,46.6939761746436,47.9508992322864));
#19967=CARTESIAN_POINT('Ctrl Pts',(44.3302304290408,46.6895370683051,48.0186666116147));
#19968=CARTESIAN_POINT('Ctrl Pts',(44.3283814998983,46.6850979619664,48.0866042680409));
#19969=CARTESIAN_POINT('Ctrl Pts',(44.3229488844025,46.6806588556279,48.1543053624323));
#19970=CARTESIAN_POINT('Ctrl Pts',(44.3175197527825,46.6762225960388,48.221963040865));
#19971=CARTESIAN_POINT('Ctrl Pts',(44.3085115324534,46.6717863364497,48.2893839659275));
#19972=CARTESIAN_POINT('Ctrl Pts',(44.2959669172311,46.6673500768606,48.3561628920383));
#19973=CARTESIAN_POINT('Ctrl Pts',(44.2834259846457,46.6629151195939,48.4229222143167));
#19974=CARTESIAN_POINT('Ctrl Pts',(44.2673508091051,46.6584801623272,48.4890394255097));
#19975=CARTESIAN_POINT('Ctrl Pts',(44.2478354859469,46.6540452050604,48.5541178338364));
#19976=CARTESIAN_POINT('Ctrl Pts',(44.2283191059579,46.6496100076235,48.6191997664122));
#19977=CARTESIAN_POINT('Ctrl Pts',(44.2053623532084,46.6451748101866,48.6832423110911));
#19978=CARTESIAN_POINT('Ctrl Pts',(44.1791091169869,46.6407396127497,48.7458641342458));
#19979=CARTESIAN_POINT('Ctrl Pts',(44.1528277688164,46.6362996661061,48.8085530128095));
#19980=CARTESIAN_POINT('Ctrl Pts',(44.1232430846532,46.6318597194626,48.8698176765481));
#19981=CARTESIAN_POINT('Ctrl Pts',(44.0905466184338,46.627419772819,48.9292979542656));
#19982=CARTESIAN_POINT('Ctrl Pts',(44.0578304684092,46.6229771532553,48.9888140400788));
#19983=CARTESIAN_POINT('Ctrl Pts',(44.0219990696359,46.6185345336915,49.0465431816973));
#19984=CARTESIAN_POINT('Ctrl Pts',(43.9832878497896,46.6140919141278,49.1021534111043));
#19985=CARTESIAN_POINT('Ctrl Pts',(43.944509152903,46.6096415506898,49.1578605740024));
#19986=CARTESIAN_POINT('Ctrl Pts',(43.9028409206391,46.6051911872518,49.2114410632156));
#19987=CARTESIAN_POINT('Ctrl Pts',(43.8585588644388,46.6007408238138,49.2625959749132));
#19988=CARTESIAN_POINT('Ctrl Pts',(43.8376527412443,46.5986397505061,49.2867468607962));
#19989=CARTESIAN_POINT('Ctrl Pts',(43.8161645536072,46.5965386771983,49.3103576451171));
#19990=CARTESIAN_POINT('Ctrl Pts',(43.7941259842674,46.5944376038905,49.3333999013388));
#19991=CARTESIAN_POINT('Ctrl Pts',(43.7473774321868,46.5899807748905,49.3822774894631));
#19992=CARTESIAN_POINT('Ctrl Pts',(43.697961986577,46.5855239458904,49.4287911969137));
#19993=CARTESIAN_POINT('Ctrl Pts',(43.6461482113789,46.5810671168903,49.4726361370608));
#19994=CARTESIAN_POINT('Ctrl Pts',(43.594412953924,46.5766170416957,49.5164146353063));
#19995=CARTESIAN_POINT('Ctrl Pts',(43.5402869531792,46.572166966501,49.5575320759062));
#19996=CARTESIAN_POINT('Ctrl Pts',(43.4840761815292,46.5677168913064,49.595719708953));
#19997=CARTESIAN_POINT('Ctrl Pts',(43.4279319327049,46.5632720825681,49.6338621487179));
#19998=CARTESIAN_POINT('Ctrl Pts',(43.369708219006,46.5588272738298,49.6690813906766));
#19999=CARTESIAN_POINT('Ctrl Pts',(43.3097432645744,46.5543824650915,49.7011495376544));
#20000=CARTESIAN_POINT('Ctrl Pts',(43.249816114471,46.5499404585401,49.7331974675776));
#20001=CARTESIAN_POINT('Ctrl Pts',(43.1881503353395,46.5454984519887,49.7620980108258));
#20002=CARTESIAN_POINT('Ctrl Pts',(43.1251108919607,46.5410564454373,49.7876679644889));
#20003=CARTESIAN_POINT('Ctrl Pts',(43.0620894213714,46.5366157053192,49.8132306280593));
#20004=CARTESIAN_POINT('Ctrl Pts',(42.9976955211072,46.5321749652011,49.835464401591));
#20005=CARTESIAN_POINT('Ctrl Pts',(42.9323146994587,46.527734225083,49.8542339705766));
#20006=CARTESIAN_POINT('Ctrl Pts',(42.8669299404626,46.5232932175357,49.8730046698985));
#20007=CARTESIAN_POINT('Ctrl Pts',(42.8005586171901,46.5188522099884,49.8883106168319));
#20008=CARTESIAN_POINT('Ctrl Pts',(42.7336002041476,46.5144112024411,49.9000666990116));
#20009=CARTESIAN_POINT('Ctrl Pts',(42.6665701630067,46.5099654441701,49.9118353571436));
#20010=CARTESIAN_POINT('Ctrl Pts',(42.5989522658176,46.5055196858991,49.9200464867793));
#20011=CARTESIAN_POINT('Ctrl Pts',(42.5311539333469,46.501073927628,49.9246665172615));
#20012=CARTESIAN_POINT('Ctrl Pts',(42.463314692732,46.4966254868762,49.9292893353768));
#20013=CARTESIAN_POINT('Ctrl Pts',(42.3952952937105,46.4921770461244,49.9303167347623));
#20014=CARTESIAN_POINT('Ctrl Pts',(42.3275031536886,46.4877286053727,49.9277673003179));
#20015=CARTESIAN_POINT('Ctrl Pts',(42.2595937096817,46.4832724672709,49.925213454465));
#20016=CARTESIAN_POINT('Ctrl Pts',(42.1919128006937,46.4788163291692,49.9190704673553));
#20017=CARTESIAN_POINT('Ctrl Pts',(42.1248618177861,46.4743601910674,49.9094086879419));
#20018=CARTESIAN_POINT('Ctrl Pts',(42.0940240884677,46.4723107478732,49.9049650940472));
#20019=CARTESIAN_POINT('Ctrl Pts',(42.0633194436199,46.4702613046789,49.8997779097643));
#20020=CARTESIAN_POINT('Ctrl Pts',(42.0327859245322,46.4682118614847,49.8938575394359));
#20021=CARTESIAN_POINT('Ctrl Pts',(41.9663867181945,46.4637550741376,49.8809829051726));
#20022=CARTESIAN_POINT('Ctrl Pts',(41.9005331589857,46.4592982867905,49.8645864316223));
#20023=CARTESIAN_POINT('Ctrl Pts',(41.8356269390523,46.4548414994434,49.8447291413583));
#20024=CARTESIAN_POINT('Ctrl Pts',(41.821753010091,46.4538888457361,49.8404845768964));
#20025=CARTESIAN_POINT('Ctrl Pts',(41.8079223464408,46.4529361920287,49.8360820743412));
#20026=CARTESIAN_POINT('Ctrl Pts',(41.7941388317924,46.4519835383214,49.8315225365139));
#20027=CARTESIAN_POINT('',(43.6084517554458,46.9748,46.4962756530334));
#20028=CARTESIAN_POINT('Origin',(42.4,46.9748,48.));
#20029=CARTESIAN_POINT('Ctrl Pts',(43.6084517554457,46.9748,46.4962756530334));
#20030=CARTESIAN_POINT('Ctrl Pts',(43.6626868745532,46.97024365882,46.5398611180319));
#20031=CARTESIAN_POINT('Ctrl Pts',(43.714603934413,46.9656873176399,46.5864184202764));
#20032=CARTESIAN_POINT('Ctrl Pts',(43.7638757919844,46.9611309764599,46.6356740195471));
#20033=CARTESIAN_POINT('Ctrl Pts',(43.8145915454213,46.9564411131738,46.6863730382389));
#20034=CARTESIAN_POINT('Ctrl Pts',(43.8625042214584,46.9517512498878,46.7399306831323));
#20035=CARTESIAN_POINT('Ctrl Pts',(43.907295865415,46.9470613866017,46.7960059256778));
#20036=CARTESIAN_POINT('Ctrl Pts',(43.9507783555296,46.9425085969302,46.8504422214749));
#20037=CARTESIAN_POINT('Ctrl Pts',(43.9913194768775,46.9379558072587,46.9072505616738));
#20038=CARTESIAN_POINT('Ctrl Pts',(44.0286688300753,46.9334030175871,46.9660849170066));
#20039=CARTESIAN_POINT('Ctrl Pts',(44.0660184763803,46.9288501921866,47.0249197340549));
#20040=CARTESIAN_POINT('Ctrl Pts',(44.1001760571108,46.9242973667861,47.0857802079187));
#20041=CARTESIAN_POINT('Ctrl Pts',(44.1309352046544,46.9197445413856,47.1482923775215));
#20042=CARTESIAN_POINT('Ctrl Pts',(44.1617030842414,46.9151904235088,47.2108222933565));
#20043=CARTESIAN_POINT('Ctrl Pts',(44.1890704094519,46.910636305632,47.2750044223297));
#20044=CARTESIAN_POINT('Ctrl Pts',(44.212877998293,46.9060821877551,47.3404426331202));
#20045=CARTESIAN_POINT('Ctrl Pts',(44.237930877054,46.9012898602417,47.4093036829401));
#20046=CARTESIAN_POINT('Ctrl Pts',(44.2590412424677,46.8964975327283,47.4795552736269));
#20047=CARTESIAN_POINT('Ctrl Pts',(44.2760831146131,46.8917052052149,47.5507175677107));
#20048=CARTESIAN_POINT('Ctrl Pts',(44.2923129273951,46.8871412360882,47.6184889193717));
#20049=CARTESIAN_POINT('Ctrl Pts',(44.3048531194064,46.8825772669614,47.6870856827015));
#20050=CARTESIAN_POINT('Ctrl Pts',(44.3136478030715,46.8780132978347,47.7560847632889));
#20051=CARTESIAN_POINT('Ctrl Pts',(44.3224506437573,46.8734450956517,47.8251478401448));
#20052=CARTESIAN_POINT('Ctrl Pts',(44.3275010239818,46.8688768934686,47.8946135174533));
#20053=CARTESIAN_POINT('Ctrl Pts',(44.32879511488,46.8643086912856,47.9640561310493));
#20054=CARTESIAN_POINT('Ctrl Pts',(44.3300915836412,46.8597320951334,48.0336263438916));
#20055=CARTESIAN_POINT('Ctrl Pts',(44.3276180036356,46.8551554989812,48.1031729479443));
#20056=CARTESIAN_POINT('Ctrl Pts',(44.3214224949418,46.850578902829,48.1722734826715));
#20057=CARTESIAN_POINT('Ctrl Pts',(44.3205179072987,46.8499106877507,48.182362644504));
#20058=CARTESIAN_POINT('Ctrl Pts',(44.3195340645117,46.8492424726725,48.1924423136961));
#20059=CARTESIAN_POINT('Ctrl Pts',(44.3184712072634,46.8485742575942,48.2025111942618));
#20060=CARTESIAN_POINT('Ctrl Pts',(44.3114461192161,46.8441576063768,48.2690627209386));
#20061=CARTESIAN_POINT('Ctrl Pts',(44.3009370448108,46.8397409551594,48.3354066300998));
#20062=CARTESIAN_POINT('Ctrl Pts',(44.2869621236117,46.8353243039421,48.4011439903015));
#20063=CARTESIAN_POINT('Ctrl Pts',(44.2730105785239,46.8309150405396,48.4667713903945));
#20064=CARTESIAN_POINT('Ctrl Pts',(44.2556047870564,46.8265057771371,48.5317937659605));
#20065=CARTESIAN_POINT('Ctrl Pts',(44.2348146748757,46.8220965137346,48.5958168055374));
#20066=CARTESIAN_POINT('Ctrl Pts',(44.2140529332195,46.8176932672845,48.6597524782355));
#20067=CARTESIAN_POINT('Ctrl Pts',(44.1899161925483,46.8132900208344,48.7226910456546));
#20068=CARTESIAN_POINT('Ctrl Pts',(44.1625250745046,46.8088867743843,48.7842499082835));
#20069=CARTESIAN_POINT('Ctrl Pts',(44.1351541789645,46.8044867787933,48.8457633228104));
#20070=CARTESIAN_POINT('Ctrl Pts',(44.1045338724111,46.8000867832024,48.9058985926058));
#20071=CARTESIAN_POINT('Ctrl Pts',(44.0708335511412,46.7956867876115,48.9642913466795));
#20072=CARTESIAN_POINT('Ctrl Pts',(44.037145927091,46.7912884498004,49.0226621002024));
#20073=CARTESIAN_POINT('Ctrl Pts',(44.0003808416171,46.7868901119892,49.0792912040808));
#20074=CARTESIAN_POINT('Ctrl Pts',(43.9607535563198,46.7824917741781,49.1338390067973));
#20075=CARTESIAN_POINT('Ctrl Pts',(43.9211268759037,46.7780935035043,49.1883859768819));
#20076=CARTESIAN_POINT('Ctrl Pts',(43.8786383805713,46.7736952328306,49.2408513026502));
#20077=CARTESIAN_POINT('Ctrl Pts',(43.8335454064445,46.7692969621568,49.2909260724619));
#20078=CARTESIAN_POINT('Ctrl Pts',(43.7884060269328,46.7648941652027,49.3410523744471));
#20079=CARTESIAN_POINT('Ctrl Pts',(43.7406571573197,46.7604913682486,49.3887828354145));
#20080=CARTESIAN_POINT('Ctrl Pts',(43.6905942279537,46.7560885712944,49.4338441671509));
#20081=CARTESIAN_POINT('Ctrl Pts',(43.6405030602585,46.7516832909134,49.4789309160319));
#20082=CARTESIAN_POINT('Ctrl Pts',(43.5880956285632,46.7472780105323,49.5213452243093));
#20083=CARTESIAN_POINT('Ctrl Pts',(43.5336994733685,46.7428727301512,49.5608549134958));
#20084=CARTESIAN_POINT('Ctrl Pts',(43.4792064486823,46.7384596047805,49.6004349621312));
#20085=CARTESIAN_POINT('Ctrl Pts',(43.4227180557824,46.7340464794098,49.6370997956782));
#20086=CARTESIAN_POINT('Ctrl Pts',(43.3645889023727,46.7296333540392,49.6706617869334));
#20087=CARTESIAN_POINT('Ctrl Pts',(43.3326038970716,46.7272050744222,49.6891289485079));
#20088=CARTESIAN_POINT('Ctrl Pts',(43.3001225346997,46.7247767948053,49.7066575081409));
#20089=CARTESIAN_POINT('Ctrl Pts',(43.267206383005,46.7223485151883,49.7232224598627));
#20090=CARTESIAN_POINT('Ctrl Pts',(43.2067712897334,46.7178901171805,49.7536362339769));
#20091=CARTESIAN_POINT('Ctrl Pts',(43.1446140584476,46.7134317191727,49.78092739701));
#20092=CARTESIAN_POINT('Ctrl Pts',(43.0810899461359,46.7089733211649,49.8048986237938));
#20093=CARTESIAN_POINT('Ctrl Pts',(43.0176540189975,46.7045211123755,49.8288365733429));
#20094=CARTESIAN_POINT('Ctrl Pts',(42.9528554307497,46.700068903586,49.8494635543898));
#20095=CARTESIAN_POINT('Ctrl Pts',(42.8870727057927,46.6956166947966,49.8666287087077));
#20096=CARTESIAN_POINT('Ctrl Pts',(42.8213586597274,46.69116913423,49.8837759421539));
#20097=CARTESIAN_POINT('Ctrl Pts',(42.7546629897453,46.6867215736633,49.8974683956888));
#20098=CARTESIAN_POINT('Ctrl Pts',(42.6873810988408,46.6822740130967,49.9076044298882));
#20099=CARTESIAN_POINT('Ctrl Pts',(42.6201462984294,46.677829565371,49.9177333698927));
#20100=CARTESIAN_POINT('Ctrl Pts',(42.5523265776817,46.6733851176453,49.9243107586995));
#20101=CARTESIAN_POINT('Ctrl Pts',(42.4843275100686,46.6689406699196,49.9272860265009));
#20102=CARTESIAN_POINT('Ctrl Pts',(42.4163336383048,46.6644965617967,49.9302610669604));
#20103=CARTESIAN_POINT('Ctrl Pts',(42.3481609384597,46.6600524536739,49.9296344979394));
#20104=CARTESIAN_POINT('Ctrl Pts',(42.2802185983989,46.6556083455511,49.9254077419421));
#20105=CARTESIAN_POINT('Ctrl Pts',(42.2122796417916,46.6511644587399,49.9211811964325));
#20106=CARTESIAN_POINT('Ctrl Pts',(42.1445715136807,46.6467205719288,49.9133548591172));
#20107=CARTESIAN_POINT('Ctrl Pts',(42.077499663665,46.6422766851176,49.9019821476459));
#20108=CARTESIAN_POINT('Ctrl Pts',(42.0103781655728,46.6378295088425,49.8906010178405));
#20109=CARTESIAN_POINT('Ctrl Pts',(41.9438943701589,46.6333823325674,49.8756683666818));
#20110=CARTESIAN_POINT('Ctrl Pts',(41.8784436240851,46.6289351562923,49.8572887507446));
#20111=CARTESIAN_POINT('Ctrl Pts',(41.8501386723655,46.6270119221459,49.8493402677565));
#20112=CARTESIAN_POINT('Ctrl Pts',(41.8220267426197,46.6250886879995,49.8407477586424));
#20113=CARTESIAN_POINT('Ctrl Pts',(41.7941388317924,46.6231654538532,49.8315225365138));
#20114=CARTESIAN_POINT('Origin',(42.4,48.4493818343519,48.));
#20115=CARTESIAN_POINT('',(41.7941388553004,45.6566247686891,49.8315225442902));
#20116=CARTESIAN_POINT('',(41.7941388200938,45.8276962776015,49.831522532644));
#20117=CARTESIAN_POINT('',(41.7941388317924,48.4493818343519,49.8315225365138));
#20118=CARTESIAN_POINT('',(40.4708703631671,46.2939681656965,48.0011837199365));
#20119=CARTESIAN_POINT('Ctrl Pts',(41.7941388553004,45.6566247686891,49.8315225442902));
#20120=CARTESIAN_POINT('Ctrl Pts',(41.8667773820973,45.6618057094251,49.8555511106498));
#20121=CARTESIAN_POINT('Ctrl Pts',(41.9407833165274,45.6671213473477,49.8752379473992));
#20122=CARTESIAN_POINT('Ctrl Pts',(42.163798922572,45.6831907125301,49.9205651215141));
#20123=CARTESIAN_POINT('Ctrl Pts',(42.3148481722396,45.6941784801436,49.933160764554));
#20124=CARTESIAN_POINT('Ctrl Pts',(42.4915432862791,45.7063529406678,49.9271286627289));
#20125=CARTESIAN_POINT('Ctrl Pts',(42.5172487699093,45.708105795493,49.9257356877976));
#20126=CARTESIAN_POINT('Ctrl Pts',(42.5514406513741,45.7104064074252,49.9231955921762));
#20127=CARTESIAN_POINT('Ctrl Pts',(42.5599570597291,45.7109768727416,49.9225059954215));
#20128=CARTESIAN_POINT('Ctrl Pts',(42.5738205620841,45.7119010266578,49.9212906679015));
#20129=CARTESIAN_POINT('Ctrl Pts',(42.5791704236636,45.7122565647407,49.9207991512443));
#20130=CARTESIAN_POINT('Ctrl Pts',(42.5896336402088,45.712949700618,49.9197937514975));
#20131=CARTESIAN_POINT('Ctrl Pts',(42.5947470824736,45.7132873930716,49.9192817772434));
#20132=CARTESIAN_POINT('Ctrl Pts',(42.607262953155,45.7141115047742,49.917978114168));
#20133=CARTESIAN_POINT('Ctrl Pts',(42.6146630639592,45.7145966789292,49.9171639866282));
#20134=CARTESIAN_POINT('Ctrl Pts',(42.6415435548888,45.7163520574611,49.914049120686));
#20135=CARTESIAN_POINT('Ctrl Pts',(42.6609940294344,45.7176088764566,49.9114940528079));
#20136=CARTESIAN_POINT('Ctrl Pts',(42.7099017374203,45.7207430747346,49.904308909853));
#20137=CARTESIAN_POINT('Ctrl Pts',(42.739297635972,45.7226029760218,49.8992916624861));
#20138=CARTESIAN_POINT('Ctrl Pts',(42.8753828009737,45.7311506314811,49.872804212946));
#20139=CARTESIAN_POINT('Ctrl Pts',(42.9802553459919,45.7375670261326,49.8430115451974));
#20140=CARTESIAN_POINT('Ctrl Pts',(43.1919143385604,45.7510930623965,49.7630104419844));
#20141=CARTESIAN_POINT('Ctrl Pts',(43.297730851187,45.7581957959159,49.7115513754023));
#20142=CARTESIAN_POINT('Ctrl Pts',(43.4128454085964,45.7667400469537,49.6419438002967));
#20143=CARTESIAN_POINT('Ctrl Pts',(43.4273668852352,45.767833400047,49.6328969710675));
#20144=CARTESIAN_POINT('Ctrl Pts',(43.4510482080652,45.7696432095943,49.617702647737));
#20145=CARTESIAN_POINT('Ctrl Pts',(43.4602792570892,45.7703555039366,49.6116674845667));
#20146=CARTESIAN_POINT('Ctrl Pts',(43.4768407465366,45.7716460848175,49.6006358904844));
#20147=CARTESIAN_POINT('Ctrl Pts',(43.4841894858888,45.772223308108,49.5956673843802));
#20148=CARTESIAN_POINT('Ctrl Pts',(43.4998595479494,45.7734641069394,49.5849145815395));
#20149=CARTESIAN_POINT('Ctrl Pts',(43.5081700514879,45.7741282513336,49.5791150643047));
#20150=CARTESIAN_POINT('Ctrl Pts',(43.5307441189072,45.7759492575661,49.5630957048825));
#20151=CARTESIAN_POINT('Ctrl Pts',(43.5449142635461,45.7771110754136,49.5527465148691));
#20152=CARTESIAN_POINT('Ctrl Pts',(43.6258229299448,45.7838558533716,49.4919450555198));
#20153=CARTESIAN_POINT('Ctrl Pts',(43.6893552659555,45.7896000345881,49.4373939781315));
#20154=CARTESIAN_POINT('Ctrl Pts',(43.8280745170499,45.8032152007495,49.3016685120338));
#20155=CARTESIAN_POINT('Ctrl Pts',(43.9002284775379,45.811160177054,49.2178052421473));
#20156=CARTESIAN_POINT('Ctrl Pts',(44.0094480011836,45.8244327431891,49.0663235900971));
#20157=CARTESIAN_POINT('Ctrl Pts',(44.0503806153536,45.8297952656205,49.0018060615622));
#20158=CARTESIAN_POINT('Ctrl Pts',(44.0924439243999,45.8356546707957,48.9258968836376));
#20159=CARTESIAN_POINT('Ctrl Pts',(44.0974283197573,45.8363552918139,48.9167271063238));
#20160=CARTESIAN_POINT('Ctrl Pts',(44.1053551849102,45.8374792884526,48.9018577386052));
#20161=CARTESIAN_POINT('Ctrl Pts',(44.108343998255,45.8379054101292,48.8961832814476));
#20162=CARTESIAN_POINT('Ctrl Pts',(44.1136052465023,45.8386595396243,48.8860724905562));
#20163=CARTESIAN_POINT('Ctrl Pts',(44.11588884507,45.8389882347199,48.8816421454806));
#20164=CARTESIAN_POINT('Ctrl Pts',(44.1208197829061,45.8397009691612,48.871984040447));
#20165=CARTESIAN_POINT('Ctrl Pts',(44.1234604871542,45.8400845958303,48.8667530464358));
#20166=CARTESIAN_POINT('Ctrl Pts',(44.1308873316673,45.8411692855527,48.8518730010199));
#20167=CARTESIAN_POINT('Ctrl Pts',(44.1356166465556,45.8418669200859,48.8421956031449));
#20168=CARTESIAN_POINT('Ctrl Pts',(44.1672825819906,45.8465894448482,48.7759991903492));
#20169=CARTESIAN_POINT('Ctrl Pts',(44.1915379209984,45.8504665523758,48.7182312241847));
#20170=CARTESIAN_POINT('Ctrl Pts',(44.2563329770538,45.8619940556464,48.5400793803369));
#20171=CARTESIAN_POINT('Ctrl Pts',(44.2878427137848,45.8694188045737,48.4167853804526));
#20172=CARTESIAN_POINT('Ctrl Pts',(44.3192963450539,45.8820215632709,48.210862351945));
#20173=CARTESIAN_POINT('Ctrl Pts',(44.3264795799396,45.8870308556702,48.1297514046474));
#20174=CARTESIAN_POINT('Ctrl Pts',(44.3289694501331,45.8933372653506,48.0306140795009));
#20175=CARTESIAN_POINT('Ctrl Pts',(44.329169976939,45.8944782417602,48.0127877788413));
#20176=CARTESIAN_POINT('Ctrl Pts',(44.3290965247083,45.8962905197872,47.9846633791191));
#20177=CARTESIAN_POINT('Ctrl Pts',(44.3289871651644,45.8969566601649,47.9743655820161));
#20178=CARTESIAN_POINT('Ctrl Pts',(44.3286304185727,45.898200462519,47.9552150643824));
#20179=CARTESIAN_POINT('Ctrl Pts',(44.3284045119398,45.8987774345346,47.9463621791805));
#20180=CARTESIAN_POINT('Ctrl Pts',(44.3277675385058,45.9000629162437,47.9267080744489));
#20181=CARTESIAN_POINT('Ctrl Pts',(44.3273266323984,45.9007723449724,47.9159081881672));
#20182=CARTESIAN_POINT('Ctrl Pts',(44.3257743046911,45.9028521901391,47.8843863806755));
#20183=CARTESIAN_POINT('Ctrl Pts',(44.324419284977,45.9042301828235,47.8636785425948));
#20184=CARTESIAN_POINT('Ctrl Pts',(44.3205852726379,45.9073822709052,47.8167253958323));
#20185=CARTESIAN_POINT('Ctrl Pts',(44.3179018728869,45.9091624325726,47.7905014050236));
#20186=CARTESIAN_POINT('Ctrl Pts',(44.3071442517798,45.9151626978326,47.7030976412943));
#20187=CARTESIAN_POINT('Ctrl Pts',(44.2966729435862,45.9194511780744,47.6422560960795));
#20188=CARTESIAN_POINT('Ctrl Pts',(44.2729714913163,45.9271587243291,47.5354622887866));
#20189=CARTESIAN_POINT('Ctrl Pts',(44.2609144470359,45.9305512245677,47.489299886513));
#20190=CARTESIAN_POINT('Ctrl Pts',(44.2119857711351,45.9426592758852,47.3268547189059));
#20191=CARTESIAN_POINT('Ctrl Pts',(44.1658142057005,45.951428728634,47.2136653319055));
#20192=CARTESIAN_POINT('Ctrl Pts',(44.1018918143267,45.9608075272988,47.091507115101));
#20193=CARTESIAN_POINT('Ctrl Pts',(44.0943503647751,45.9618798451371,47.0775185903944));
#20194=CARTESIAN_POINT('Ctrl Pts',(44.0835502060202,45.9633671080864,47.0580649207555));
#20195=CARTESIAN_POINT('Ctrl Pts',(44.0804362601628,45.9637905095421,47.0525207294839));
#20196=CARTESIAN_POINT('Ctrl Pts',(44.0749968940717,45.9645206737539,47.0429474410594));
#20197=CARTESIAN_POINT('Ctrl Pts',(44.0726842319738,45.96482823164,47.0389112127462));
#20198=CARTESIAN_POINT('Ctrl Pts',(44.0677506554542,45.9654781951372,47.0303725208013));
#20199=CARTESIAN_POINT('Ctrl Pts',(44.0651260554681,45.9658203513396,47.0258722271055));
#20200=CARTESIAN_POINT('Ctrl Pts',(44.0585289953391,45.9666715556365,47.0146650879303));
#20201=CARTESIAN_POINT('Ctrl Pts',(44.0545340049802,45.967179163553,47.0079714979918));
#20202=CARTESIAN_POINT('Ctrl Pts',(44.0390527350458,45.9691171294027,46.9823863695682));
#20203=CARTESIAN_POINT('Ctrl Pts',(44.0272820706572,45.9705301891106,46.9636677498552));
#20204=CARTESIAN_POINT('Ctrl Pts',(43.9959630396975,45.9741491133502,46.9157116801642));
#20205=CARTESIAN_POINT('Ctrl Pts',(43.9759318279895,45.9763298248796,46.8867981518588));
#20206=CARTESIAN_POINT('Ctrl Pts',(43.8996140899327,45.984229705434,46.782831684283));
#20207=CARTESIAN_POINT('Ctrl Pts',(43.8386639034537,45.9897811464425,46.7113614646491));
#20208=CARTESIAN_POINT('Ctrl Pts',(43.6856272587649,46.0027877866331,46.5563648316089));
#20209=CARTESIAN_POINT('Ctrl Pts',(43.590209373986,46.0102638299392,46.4767417427015));
#20210=CARTESIAN_POINT('Ctrl Pts',(43.4737487735197,46.01922156021,46.3972222869714));
#20211=CARTESIAN_POINT('Ctrl Pts',(43.4595522659272,46.0203104333083,46.3878021858034));
#20212=CARTESIAN_POINT('Ctrl Pts',(43.4359817098638,46.0221143472094,46.3726077265948));
#20213=CARTESIAN_POINT('Ctrl Pts',(43.4266795027096,46.0228252730752,46.366723261316));
#20214=CARTESIAN_POINT('Ctrl Pts',(43.4097920020359,46.0241143857542,46.356241705648));
#20215=CARTESIAN_POINT('Ctrl Pts',(43.4022243435893,46.0246915202163,46.3516166773702));
#20216=CARTESIAN_POINT('Ctrl Pts',(43.3859288005859,46.0259332503235,46.3418112392476));
#20217=CARTESIAN_POINT('Ctrl Pts',(43.3771914190204,46.0265984230905,46.3366472142057));
#20218=CARTESIAN_POINT('Ctrl Pts',(43.3531769689252,46.0284251734035,46.3227085525852));
#20219=CARTESIAN_POINT('Ctrl Pts',(43.3378201183847,46.0295917594998,46.3140740455062));
#20220=CARTESIAN_POINT('Ctrl Pts',(43.2476104723796,46.0364372790108,46.2649668870141));
#20221=CARTESIAN_POINT('Ctrl Pts',(43.1702741269578,46.0422832705227,46.2292776725919));
#20222=CARTESIAN_POINT('Ctrl Pts',(42.9813282326039,46.0564902560166,46.1568076039486));
#20223=CARTESIAN_POINT('Ctrl Pts',(42.8682119539161,46.0649456452814,46.124879865722));
#20224=CARTESIAN_POINT('Ctrl Pts',(42.6859905278963,46.0780816973697,46.0909727782788));
#20225=CARTESIAN_POINT('Ctrl Pts',(42.6184533488154,46.0828437093803,46.0820699415558));
#20226=CARTESIAN_POINT('Ctrl Pts',(42.5402670456198,46.0881377491668,46.075948357268));
#20227=CARTESIAN_POINT('Ctrl Pts',(42.5299473831055,46.08883210117,46.075223842332));
#20228=CARTESIAN_POINT('Ctrl Pts',(42.5132480335645,46.0899480651109,46.0741863471328));
#20229=CARTESIAN_POINT('Ctrl Pts',(42.5068719079531,46.0903723614325,46.0738219861943));
#20230=CARTESIAN_POINT('Ctrl Pts',(42.495517170928,46.0911246142364,46.0732296807967));
#20231=CARTESIAN_POINT('Ctrl Pts',(42.4905393713068,46.0914532427062,46.0729893573087));
#20232=CARTESIAN_POINT('Ctrl Pts',(42.4796827908146,46.0921674562491,46.0725073734404));
#20233=CARTESIAN_POINT('Ctrl Pts',(42.4738038103962,46.0925526162157,46.0722733149012));
#20234=CARTESIAN_POINT('Ctrl Pts',(42.4570569256685,46.0936454741309,46.0716832991742));
#20235=CARTESIAN_POINT('Ctrl Pts',(42.4461867476324,46.0943496658085,46.0713923185081));
#20236=CARTESIAN_POINT('Ctrl Pts',(42.3699953405961,46.0992529352522,46.0699973354233));
#20237=CARTESIAN_POINT('Ctrl Pts',(42.3046499611367,46.1032910748266,46.0721201064787));
#20238=CARTESIAN_POINT('Ctrl Pts',(42.1098528306854,46.1151579926013,46.0883800309589));
#20239=CARTESIAN_POINT('Ctrl Pts',(41.9816010256449,46.1227646625686,46.1122975347731));
#20240=CARTESIAN_POINT('Ctrl Pts',(41.7841648662026,46.1352491303514,46.1702434568717));
#20241=CARTESIAN_POINT('Ctrl Pts',(41.7129219812569,46.1399188927578,46.1957872283272));
#20242=CARTESIAN_POINT('Ctrl Pts',(41.62720463498,46.1458468374139,46.2323352684189));
#20243=CARTESIAN_POINT('Ctrl Pts',(41.6111373411609,46.1469716954382,46.2394469754652));
#20244=CARTESIAN_POINT('Ctrl Pts',(41.5858611883222,46.1487641513322,46.251050182646));
#20245=CARTESIAN_POINT('Ctrl Pts',(41.5765868643382,46.149426782356,46.2553973892012));
#20246=CARTESIAN_POINT('Ctrl Pts',(41.5595118850458,46.150656134477,46.2635675239652));
#20247=CARTESIAN_POINT('Ctrl Pts',(41.5517015491145,46.1512221221055,46.2673697020795));
#20248=CARTESIAN_POINT('Ctrl Pts',(41.5344715870287,46.1524789889194,46.2759019103531));
#20249=CARTESIAN_POINT('Ctrl Pts',(41.5250645661024,46.1531707204732,46.2806566266772));
#20250=CARTESIAN_POINT('Ctrl Pts',(41.5055594783753,46.1546167333823,46.2907168689194));
#20251=CARTESIAN_POINT('Ctrl Pts',(41.4954685841182,46.1553714522756,46.2960353357381));
#20252=CARTESIAN_POINT('Ctrl Pts',(41.469487169611,46.157332121533,46.3100248186557));
#20253=CARTESIAN_POINT('Ctrl Pts',(41.4536707705822,46.1585427881257,46.3188304092879));
#20254=CARTESIAN_POINT('Ctrl Pts',(41.4071462348321,46.162155785298,46.3455969504621));
#20255=CARTESIAN_POINT('Ctrl Pts',(41.3768097755785,46.1645797823264,46.3641853586077));
#20256=CARTESIAN_POINT('Ctrl Pts',(41.205262518966,46.1786855298452,46.4759388274663));
#20257=CARTESIAN_POINT('Ctrl Pts',(41.0762883891773,46.1909742825748,46.5865173654446));
#20258=CARTESIAN_POINT('Ctrl Pts',(40.9279603339567,46.206612720103,46.7520163552216));
#20259=CARTESIAN_POINT('Ctrl Pts',(40.8941542568313,46.2102978522744,46.7930229208938));
#20260=CARTESIAN_POINT('Ctrl Pts',(40.8556297705303,46.2146002309119,46.843895616358));
#20261=CARTESIAN_POINT('Ctrl Pts',(40.8492491898741,46.2153164410881,46.8524684364828));
#20262=CARTESIAN_POINT('Ctrl Pts',(40.8394523048512,46.2164212671498,46.8658622887984));
#20263=CARTESIAN_POINT('Ctrl Pts',(40.8359864729835,46.2168131431537,46.870646580369));
#20264=CARTESIAN_POINT('Ctrl Pts',(40.8296411320068,46.2175323831199,46.8794910276876));
#20265=CARTESIAN_POINT('Ctrl Pts',(40.8267553565651,46.2178601624578,46.8835464074671));
#20266=CARTESIAN_POINT('Ctrl Pts',(40.8202268490702,46.2186032897646,46.8927964956614));
#20267=CARTESIAN_POINT('Ctrl Pts',(40.8165940252868,46.2190179635082,46.89799803517));
#20268=CARTESIAN_POINT('Ctrl Pts',(40.8055056070785,46.2202875649612,46.9140426613678));
#20269=CARTESIAN_POINT('Ctrl Pts',(40.7981350544288,46.221136972461,46.9249444527828));
#20270=CARTESIAN_POINT('Ctrl Pts',(40.7811727483579,46.2231069568287,46.9505952283035));
#20271=CARTESIAN_POINT('Ctrl Pts',(40.7716699154517,46.2242224034717,46.9654018999921));
#20272=CARTESIAN_POINT('Ctrl Pts',(40.7387771931728,46.2281337404714,47.0182292473946));
#20273=CARTESIAN_POINT('Ctrl Pts',(40.7165043999262,46.2308760644686,47.0569315369129));
#20274=CARTESIAN_POINT('Ctrl Pts',(40.629871036275,46.2420985689469,47.2203382254642));
#20275=CARTESIAN_POINT('Ctrl Pts',(40.5778687477796,46.250277495711,47.3511018331962));
#20276=CARTESIAN_POINT('Ctrl Pts',(40.5241453152251,46.2625830210372,47.5455898767062));
#20277=CARTESIAN_POINT('Ctrl Pts',(40.5106235816986,46.26639096728,47.6055700443864));
#20278=CARTESIAN_POINT('Ctrl Pts',(40.4968945368282,46.2714233410843,47.6836907565701));
#20279=CARTESIAN_POINT('Ctrl Pts',(40.4940460341359,46.2725644777965,47.7013339870714));
#20280=CARTESIAN_POINT('Ctrl Pts',(40.4898039573857,46.274436801096,47.730147659409));
#20281=CARTESIAN_POINT('Ctrl Pts',(40.4882622667632,46.2751632992933,47.7412954631389));
#20282=CARTESIAN_POINT('Ctrl Pts',(40.4856781407055,46.2764689072934,47.7612672717363));
#20283=CARTESIAN_POINT('Ctrl Pts',(40.4845989544873,46.277046836753,47.7700862619979));
#20284=CARTESIAN_POINT('Ctrl Pts',(40.4826279140193,46.278169330505,47.787171515488));
#20285=CARTESIAN_POINT('Ctrl Pts',(40.481728501575,46.2787136420374,47.7954367223339));
#20286=CARTESIAN_POINT('Ctrl Pts',(40.4798858795933,46.2799029464669,47.813451703841));
#20287=CARTESIAN_POINT('Ctrl Pts',(40.4789634486876,46.2805485803986,47.8232033239643));
#20288=CARTESIAN_POINT('Ctrl Pts',(40.4761992387617,46.2826605122948,47.8550073051383));
#20289=CARTESIAN_POINT('Ctrl Pts',(40.4746626862145,46.2841363078213,47.8770837311232));
#20290=CARTESIAN_POINT('Ctrl Pts',(40.4717266466095,46.2879129183618,47.9331868341155));
#20291=CARTESIAN_POINT('Ctrl Pts',(40.4708478359641,46.2902291322323,47.967231647312));
#20292=CARTESIAN_POINT('Ctrl Pts',(40.4708704245423,46.2925701609289,48.0012798415654));
#20293=CARTESIAN_POINT('Ctrl Pts',(41.7941388317924,46.4519835383214,49.8315225365139));
#20294=CARTESIAN_POINT('Ctrl Pts',(41.727826215268,46.4474003125196,49.8095865578331));
#20295=CARTESIAN_POINT('Ctrl Pts',(41.6626060745432,46.4428170867179,49.7840113396514));
#20296=CARTESIAN_POINT('Ctrl Pts',(41.5989029229069,46.4382338609161,49.7549319160506));
#20297=CARTESIAN_POINT('Ctrl Pts',(41.5371339006962,46.4337897891696,49.7267353901937));
#20298=CARTESIAN_POINT('Ctrl Pts',(41.4767915503687,46.4293457174232,49.6952446309924));
#20299=CARTESIAN_POINT('Ctrl Pts',(41.4182454283156,46.4249016456767,49.6606325655836));
#20300=CARTESIAN_POINT('Ctrl Pts',(41.3597310685853,46.420459984919,49.6260392778419));
#20301=CARTESIAN_POINT('Ctrl Pts',(41.3030114280562,46.4160183241613,49.588328293954));
#20302=CARTESIAN_POINT('Ctrl Pts',(41.248431409697,46.4115766634036,49.5477184300536));
#20303=CARTESIAN_POINT('Ctrl Pts',(41.1938621552395,46.4071358786002,49.5071165749556));
#20304=CARTESIAN_POINT('Ctrl Pts',(41.1414320807568,46.4026950937967,49.4636172698326));
#20305=CARTESIAN_POINT('Ctrl Pts',(41.0914555183565,46.3982543089933,49.4174815330227));
#20306=CARTESIAN_POINT('Ctrl Pts',(41.0414715553891,46.3938128665951,49.371338964398));
#20307=CARTESIAN_POINT('Ctrl Pts',(40.9939421862332,46.3893714241968,49.3225595260854));
#20308=CARTESIAN_POINT('Ctrl Pts',(40.9491458165153,46.3849299817986,49.2714419747535));
#20309=CARTESIAN_POINT('Ctrl Pts',(40.9042989929577,46.3804835370347,49.2202668500788));
#20310=CARTESIAN_POINT('Ctrl Pts',(40.862191634198,46.3760370922708,49.166748731578));
#20311=CARTESIAN_POINT('Ctrl Pts',(40.8230619659899,46.3715906475069,49.1112195974659));
#20312=CARTESIAN_POINT('Ctrl Pts',(40.7839056121508,46.3671411703589,49.0556525936237));
#20313=CARTESIAN_POINT('Ctrl Pts',(40.7477312506203,46.3626916932108,48.9980722635646));
#20314=CARTESIAN_POINT('Ctrl Pts',(40.7147323498353,46.3582422160628,48.9388373150915));
#20315=CARTESIAN_POINT('Ctrl Pts',(40.6816785786209,46.3537853403435,48.8795038710027));
#20316=CARTESIAN_POINT('Ctrl Pts',(40.6518110148748,46.3493284646241,48.8185107635707));
#20317=CARTESIAN_POINT('Ctrl Pts',(40.6252755672461,46.3448715889048,48.7562378889518));
#20318=CARTESIAN_POINT('Ctrl Pts',(40.6195490420395,46.3439097656295,48.7427989904948));
#20319=CARTESIAN_POINT('Ctrl Pts',(40.6139775172925,46.3429479423542,48.729300546802));
#20320=CARTESIAN_POINT('Ctrl Pts',(40.6085621529345,46.3419861190789,48.7157464613962));
#20321=CARTESIAN_POINT('Ctrl Pts',(40.580284191365,46.3369636681749,48.644969708278));
#20322=CARTESIAN_POINT('Ctrl Pts',(40.556173274459,46.3319412172709,48.5724370836976));
#20323=CARTESIAN_POINT('Ctrl Pts',(40.5364232936375,46.3269187663669,48.4986225189492));
#20324=CARTESIAN_POINT('Ctrl Pts',(40.5167501656455,46.3219158592573,48.425095187804));
#20325=CARTESIAN_POINT('Ctrl Pts',(40.5014042471389,46.3169129521476,48.3502961023876));
#20326=CARTESIAN_POINT('Ctrl Pts',(40.4905304824803,46.3119100450379,48.2747157049807));
#20327=CARTESIAN_POINT('Ctrl Pts',(40.4797262149631,46.3069391128471,48.1996183621309));
#20328=CARTESIAN_POINT('Ctrl Pts',(40.4733372415611,46.3019681806564,48.1237499091596));
#20329=CARTESIAN_POINT('Ctrl Pts',(40.4714575774903,46.2969972484656,48.0476096784313));
#20330=CARTESIAN_POINT('Ctrl Pts',(40.4710757806877,46.2959875542092,48.0321440975915));
#20331=CARTESIAN_POINT('Ctrl Pts',(40.470879863975,46.2949778599529,48.0166673571739));
#20332=CARTESIAN_POINT('Ctrl Pts',(40.4708703631671,46.2939681656965,48.0011837199365));
#20333=CARTESIAN_POINT('',(40.4708700795635,46.4650068343519,48.0005540547159));
#20334=CARTESIAN_POINT('Ctrl Pts',(41.7941388317924,46.6231654538532,49.8315225365138));
#20335=CARTESIAN_POINT('Ctrl Pts',(41.7287833055596,46.6186583403414,49.8099031599117));
#20336=CARTESIAN_POINT('Ctrl Pts',(41.6646598591436,46.6141512268296,49.7848056142629));
#20337=CARTESIAN_POINT('Ctrl Pts',(41.6021507757283,46.6096441133178,49.7564108779636));
#20338=CARTESIAN_POINT('Ctrl Pts',(41.5396416923129,46.605136999806,49.7280161416644));
#20339=CARTESIAN_POINT('Ctrl Pts',(41.4787474022242,46.6006298862943,49.6963245113389));
#20340=CARTESIAN_POINT('Ctrl Pts',(41.4198212647442,46.5961227727825,49.6615631808187));
#20341=CARTESIAN_POINT('Ctrl Pts',(41.3614665912009,46.5916593691241,49.6271389646527));
#20342=CARTESIAN_POINT('Ctrl Pts',(41.3048151949058,46.5871959654657,49.5895705731172));
#20343=CARTESIAN_POINT('Ctrl Pts',(41.250225540661,46.5827325618073,49.5490517259122));
#20344=CARTESIAN_POINT('Ctrl Pts',(41.1957165968945,46.5782757572646,49.5085927855813));
#20345=CARTESIAN_POINT('Ctrl Pts',(41.1432637369315,46.5738189527219,49.4651923385466));
#20346=CARTESIAN_POINT('Ctrl Pts',(41.0931985951083,46.5693621481793,49.4190886670935));
#20347=CARTESIAN_POINT('Ctrl Pts',(41.0431904209025,46.5649104149003,49.3730374556198));
#20348=CARTESIAN_POINT('Ctrl Pts',(40.9955649291494,46.5604586816213,49.324289460263));
#20349=CARTESIAN_POINT('Ctrl Pts',(40.9506212007339,46.5560069483423,49.2731235812512));
#20350=CARTESIAN_POINT('Ctrl Pts',(40.905704581011,46.5515579002136,49.2219885639444));
#20351=CARTESIAN_POINT('Ctrl Pts',(40.8634668395876,46.547108852085,49.1684389249248));
#20352=CARTESIAN_POINT('Ctrl Pts',(40.8241695250672,46.5426598039564,49.1127896796669));
#20353=CARTESIAN_POINT('Ctrl Pts',(40.78488245976,46.5382119161931,49.0571549484027));
#20354=CARTESIAN_POINT('Ctrl Pts',(40.7485345823357,46.5337640284298,48.9994220997049));
#20355=CARTESIAN_POINT('Ctrl Pts',(40.7153454172212,46.5293161406666,48.9399369625791));
#20356=CARTESIAN_POINT('Ctrl Pts',(40.6821535461303,46.5248678902585,48.8804469755157));
#20357=CARTESIAN_POINT('Ctrl Pts',(40.6521211360122,46.5204196398504,48.8192048471323));
#20358=CARTESIAN_POINT('Ctrl Pts',(40.6254219621436,46.5159713894423,48.756581353496));
#20359=CARTESIAN_POINT('Ctrl Pts',(40.5986937094228,46.5115182943144,48.6938896547785));
#20360=CARTESIAN_POINT('Ctrl Pts',(40.5753061307835,46.5070651991865,48.629814041767));
#20361=CARTESIAN_POINT('Ctrl Pts',(40.5553845982352,46.5026121040586,48.5647447002603));
#20362=CARTESIAN_POINT('Ctrl Pts',(40.5354507774457,46.4981562621186,48.4996352218936));
#20363=CARTESIAN_POINT('Ctrl Pts',(40.5189873765866,46.4937004201785,48.4335312723801));
#20364=CARTESIAN_POINT('Ctrl Pts',(40.5060689709932,46.4892445782385,48.3668348596646));
#20365=CARTESIAN_POINT('Ctrl Pts',(40.493128187358,46.4847810176202,48.3000229113981));
#20366=CARTESIAN_POINT('Ctrl Pts',(40.4837447224647,46.4803174570019,48.2326169384692));
#20367=CARTESIAN_POINT('Ctrl Pts',(40.4779413739301,46.4758538963836,48.1650248310114));
#20368=CARTESIAN_POINT('Ctrl Pts',(40.4753597451538,46.4738682743813,48.1349563750796));
#20369=CARTESIAN_POINT('Ctrl Pts',(40.4734859041685,46.471882652379,48.1048510896329));
#20370=CARTESIAN_POINT('Ctrl Pts',(40.4723185475692,46.4698970303766,48.0747447312809));
#20371=CARTESIAN_POINT('Ctrl Pts',(40.4713602244183,46.4682669650351,48.0500293870446));
#20372=CARTESIAN_POINT('Ctrl Pts',(40.47087718529,46.4666368996935,48.0252950581875));
#20373=CARTESIAN_POINT('Ctrl Pts',(40.4708700795635,46.4650068343519,48.0005540547159));
#20374=CARTESIAN_POINT('Ctrl Pts',(40.4708701150492,46.4632498880547,48.0006662504151));
#20375=CARTESIAN_POINT('Ctrl Pts',(40.4708552840327,46.460507586754,47.9577230019347));
#20376=CARTESIAN_POINT('Ctrl Pts',(40.4722743616713,46.4578329855591,47.9147871563977));
#20377=CARTESIAN_POINT('Ctrl Pts',(40.4865662148564,46.4446308769824,47.6999814642341));
#20378=CARTESIAN_POINT('Ctrl Pts',(40.5209937658437,46.4347081789134,47.530337677286));
#20379=CARTESIAN_POINT('Ctrl Pts',(40.5951923604088,46.4207891607846,47.3165354800588));
#20380=CARTESIAN_POINT('Ctrl Pts',(40.6150138033227,46.4174174900997,47.266325807559));
#20381=CARTESIAN_POINT('Ctrl Pts',(40.6431677001459,46.4129912787833,47.2029301328526));
#20382=CARTESIAN_POINT('Ctrl Pts',(40.6495916749533,46.4120022547676,47.1889199940303));
#20383=CARTESIAN_POINT('Ctrl Pts',(40.660300513753,46.4103859051362,47.166284840379));
#20384=CARTESIAN_POINT('Ctrl Pts',(40.6644833878878,46.4097621385383,47.1576121123378));
#20385=CARTESIAN_POINT('Ctrl Pts',(40.6726595190762,46.4085570646184,47.1409792055157));
#20386=CARTESIAN_POINT('Ctrl Pts',(40.6766433236021,46.4079761017127,47.1330146346165));
#20387=CARTESIAN_POINT('Ctrl Pts',(40.6859209663589,46.4066370447662,47.1147830456223));
#20388=CARTESIAN_POINT('Ctrl Pts',(40.6912521191776,46.4058776421258,47.1045355061669));
#20389=CARTESIAN_POINT('Ctrl Pts',(40.7081867888205,46.4034958406936,47.0726856492009));
#20390=CARTESIAN_POINT('Ctrl Pts',(40.7201099752349,46.4018620918835,47.0512570125377));
#20391=CARTESIAN_POINT('Ctrl Pts',(40.805821197561,46.3904026808009,46.9038982882746));
#20392=CARTESIAN_POINT('Ctrl Pts',(40.893271933691,46.3800615731715,46.7864927129354));
#20393=CARTESIAN_POINT('Ctrl Pts',(41.047707628527,46.3639232627292,46.6218785812438));
#20394=CARTESIAN_POINT('Ctrl Pts',(41.1058815170792,46.3582164254853,46.5671105782759));
#20395=CARTESIAN_POINT('Ctrl Pts',(41.1867019593298,46.3509008272281,46.4999707734454));
#20396=CARTESIAN_POINT('Ctrl Pts',(41.2064355536179,46.3491590650644,46.4842216991207));
#20397=CARTESIAN_POINT('Ctrl Pts',(41.2359194179308,46.346627730218,46.4616240404142));
#20398=CARTESIAN_POINT('Ctrl Pts',(41.2454323531625,46.345821565881,46.4544716890596));
#20399=CARTESIAN_POINT('Ctrl Pts',(41.2606977153002,46.3445454324041,46.4432139565821));
#20400=CARTESIAN_POINT('Ctrl Pts',(41.2664073929846,46.3440719693008,46.4390514787571));
#20401=CARTESIAN_POINT('Ctrl Pts',(41.2771912670167,46.3431851458396,46.4312801801213));
#20402=CARTESIAN_POINT('Ctrl Pts',(41.2822602985823,46.3427713336254,46.4276643848327));
#20403=CARTESIAN_POINT('Ctrl Pts',(41.2913076407346,46.3420382782745,46.4212766811355));
#20404=CARTESIAN_POINT('Ctrl Pts',(41.2952789741683,46.3417183893128,46.4184951717373));
#20405=CARTESIAN_POINT('Ctrl Pts',(41.3039411618193,46.3410247574061,46.4124767531489));
#20406=CARTESIAN_POINT('Ctrl Pts',(41.3086358880727,46.3406514062176,46.4092456464545));
#20407=CARTESIAN_POINT('Ctrl Pts',(41.3214191017703,46.3396416000418,46.4005309338823));
#20408=CARTESIAN_POINT('Ctrl Pts',(41.3295351781033,46.3390078011307,46.3950878147536));
#20409=CARTESIAN_POINT('Ctrl Pts',(41.3702073480632,46.3358661096318,46.3682564629621));
#20410=CARTESIAN_POINT('Ctrl Pts',(41.4033670899543,46.3334139538375,46.3477944422935));
#20411=CARTESIAN_POINT('Ctrl Pts',(41.5380249657494,46.3237890605195,46.2702312815312));
#20412=CARTESIAN_POINT('Ctrl Pts',(41.6439863349158,46.3169361054216,46.2213632729674));
#20413=CARTESIAN_POINT('Ctrl Pts',(41.8592105471828,46.3032767390657,46.1448381501431));
#20414=CARTESIAN_POINT('Ctrl Pts',(41.9677566965841,46.2965019188156,46.1165882636696));
#20415=CARTESIAN_POINT('Ctrl Pts',(42.099027387672,46.2880679421048,46.0943748592831));
#20416=CARTESIAN_POINT('Ctrl Pts',(42.1199792489612,46.2867152793351,46.0911836095156));
#20417=CARTESIAN_POINT('Ctrl Pts',(42.1517897084826,46.2846498068543,46.0868734412592));
#20418=CARTESIAN_POINT('Ctrl Pts',(42.1626126699525,46.2839450149413,46.0855003718904));
#20419=CARTESIAN_POINT('Ctrl Pts',(42.1822605533313,46.2826615730958,46.083176882453));
#20420=CARTESIAN_POINT('Ctrl Pts',(42.1910815536594,46.2820839192053,46.0821954195086));
#20421=CARTESIAN_POINT('Ctrl Pts',(42.2101047262249,46.2808349054589,46.0802116190892));
#20422=CARTESIAN_POINT('Ctrl Pts',(42.2203087040767,46.2801629219421,46.0792296665749));
#20423=CARTESIAN_POINT('Ctrl Pts',(42.2480238825849,46.2783320361356,46.0767853498229));
#20424=CARTESIAN_POINT('Ctrl Pts',(42.2655476681068,46.2771682256669,46.0754808739473));
#20425=CARTESIAN_POINT('Ctrl Pts',(42.3592648261936,46.270909488596,46.069790748067));
#20426=CARTESIAN_POINT('Ctrl Pts',(42.4356408428096,46.2656825054002,46.0696906456074));
#20427=CARTESIAN_POINT('Ctrl Pts',(42.6407527808226,46.2513188618444,46.0815991318318));
#20428=CARTESIAN_POINT('Ctrl Pts',(42.7686100326898,46.2419975556876,46.1020152387178));
#20429=CARTESIAN_POINT('Ctrl Pts',(42.9561618963193,46.2282753272947,46.151640133866));
#20430=CARTESIAN_POINT('Ctrl Pts',(43.0180011237031,46.2237487159198,46.1713866711326));
#20431=CARTESIAN_POINT('Ctrl Pts',(43.0889124536931,46.2186412460737,46.1980398364184));
#20432=CARTESIAN_POINT('Ctrl Pts',(43.0990589248348,46.2179125068184,46.2019517712064));
#20433=CARTESIAN_POINT('Ctrl Pts',(43.114651996241,46.2167963765403,46.2081155720415));
#20434=CARTESIAN_POINT('Ctrl Pts',(43.1201220697898,46.2164055613946,46.2103068738502));
#20435=CARTESIAN_POINT('Ctrl Pts',(43.1302073933846,46.2156864605986,46.2144007622343));
#20436=CARTESIAN_POINT('Ctrl Pts',(43.1348253009995,46.2153577749367,46.2162961979812));
#20437=CARTESIAN_POINT('Ctrl Pts',(43.1453481982665,46.2146100792474,46.2206631587664));
#20438=CARTESIAN_POINT('Ctrl Pts',(43.1512482805549,46.214191766579,46.2231461638364));
#20439=CARTESIAN_POINT('Ctrl Pts',(43.166688881263,46.2130991568552,46.2297348813172));
#20440=CARTESIAN_POINT('Ctrl Pts',(43.1762089422018,46.2124276302207,46.2338884178587));
#20441=CARTESIAN_POINT('Ctrl Pts',(43.2525176021799,46.2070585405321,46.2679175848093));
#20442=CARTESIAN_POINT('Ctrl Pts',(43.317599017047,46.2025625092259,46.3014976049751));
#20443=CARTESIAN_POINT('Ctrl Pts',(43.4778469462884,46.191318972357,46.396087673145));
#20444=CARTESIAN_POINT('Ctrl Pts',(43.5698467549764,46.1846858618212,46.4619010824607));
#20445=CARTESIAN_POINT('Ctrl Pts',(43.7195425691231,46.1727664267429,46.5902300419548));
#20446=CARTESIAN_POINT('Ctrl Pts',(43.7798511681422,46.1675811720529,46.6492031789765));
#20447=CARTESIAN_POINT('Ctrl Pts',(43.8478445496594,46.1611011175132,46.7250106967588));
#20448=CARTESIAN_POINT('Ctrl Pts',(43.8594019872309,46.1599754040952,46.738256218486));
#20449=CARTESIAN_POINT('Ctrl Pts',(43.877339452542,46.1581883652133,46.7593898434653));
#20450=CARTESIAN_POINT('Ctrl Pts',(43.8838412148424,46.1575320641356,46.7671737100688));
#20451=CARTESIAN_POINT('Ctrl Pts',(43.8959146901998,46.1562969448355,46.7818618701515));
#20452=CARTESIAN_POINT('Ctrl Pts',(43.9015007599331,46.1557187314165,46.7887540599727));
#20453=CARTESIAN_POINT('Ctrl Pts',(43.9139198585538,46.1544178075405,46.8042948922488));
#20454=CARTESIAN_POINT('Ctrl Pts',(43.9207266591163,46.1536940724038,46.8129640011806));
#20455=CARTESIAN_POINT('Ctrl Pts',(43.9378928225782,46.1518410059216,46.8352167389674));
#20456=CARTESIAN_POINT('Ctrl Pts',(43.9481465462219,46.1507075758894,46.8488802763014));
#20457=CARTESIAN_POINT('Ctrl Pts',(44.0242677010004,46.1420869247016,46.953172000813));
#20458=CARTESIAN_POINT('Ctrl Pts',(44.0822980429427,46.1343003987884,47.04923195623));
#20459=CARTESIAN_POINT('Ctrl Pts',(44.1944689927516,46.1162361746765,47.2776894348219));
#20460=CARTESIAN_POINT('Ctrl Pts',(44.2429110816477,46.105900733293,47.4121792535044));
#20461=CARTESIAN_POINT('Ctrl Pts',(44.2809943344811,46.0947049451618,47.5712285788929));
#20462=CARTESIAN_POINT('Ctrl Pts',(44.2855559377303,46.0932797267022,47.5917555718817));
#20463=CARTESIAN_POINT('Ctrl Pts',(44.2913176355134,46.0913599927763,47.6198439561263));
#20464=CARTESIAN_POINT('Ctrl Pts',(44.2928095117034,46.0908504021819,47.6273430889051));
#20465=CARTESIAN_POINT('Ctrl Pts',(44.2952368644038,46.0899998818677,47.6399352908648));
#20466=CARTESIAN_POINT('Ctrl Pts',(44.296196480144,46.0896576129552,47.6450235533307));
#20467=CARTESIAN_POINT('Ctrl Pts',(44.297983297468,46.089008665436,47.6547119987486));
#20468=CARTESIAN_POINT('Ctrl Pts',(44.2988142841292,46.0887017667262,47.6593114078387));
#20469=CARTESIAN_POINT('Ctrl Pts',(44.3007533065816,46.0879731721839,47.6702711646044));
#20470=CARTESIAN_POINT('Ctrl Pts',(44.3018461546069,46.0875523279078,47.6766341939783));
#20471=CARTESIAN_POINT('Ctrl Pts',(44.3056160557135,46.0860628734684,47.6992645805628));
#20472=CARTESIAN_POINT('Ctrl Pts',(44.3081165955785,46.0850036634006,47.7155611740648));
#20473=CARTESIAN_POINT('Ctrl Pts',(44.3247345871394,46.0773911685787,47.8339713894062));
#20474=CARTESIAN_POINT('Ctrl Pts',(44.3308578064202,46.071209084178,47.9370524185077));
#20475=CARTESIAN_POINT('Ctrl Pts',(44.3264794976112,46.0586467317207,48.1474271025378));
#20476=CARTESIAN_POINT('Ctrl Pts',(44.3152990680754,46.0522858907156,48.2543340425677));
#20477=CARTESIAN_POINT('Ctrl Pts',(44.2849069673674,46.042271368237,48.4144484971756));
#20478=CARTESIAN_POINT('Ctrl Pts',(44.2721633146581,46.0387952519515,48.4686634857562));
#20479=CARTESIAN_POINT('Ctrl Pts',(44.2528655649094,46.0342470983823,48.5372855510325));
#20480=CARTESIAN_POINT('Ctrl Pts',(44.2484543780888,46.0332447615468,48.5522707251424));
#20481=CARTESIAN_POINT('Ctrl Pts',(44.241007556239,46.0316098728776,48.5764789451563));
#20482=CARTESIAN_POINT('Ctrl Pts',(44.2380833586545,46.0309809837329,48.5857357401003));
#20483=CARTESIAN_POINT('Ctrl Pts',(44.2323307493011,46.0297681788473,48.6034787423235));
#20484=CARTESIAN_POINT('Ctrl Pts',(44.2295129293274,46.0291846262352,48.6119681398054));
#20485=CARTESIAN_POINT('Ctrl Pts',(44.2229194993601,46.0278426240446,48.6313799220639));
#20486=CARTESIAN_POINT('Ctrl Pts',(44.2191046083557,46.0270828871039,48.6422885029913));
#20487=CARTESIAN_POINT('Ctrl Pts',(44.2066279741783,46.024649767361,48.6769621189402));
#20488=CARTESIAN_POINT('Ctrl Pts',(44.1975970492132,46.0229641677198,48.7005905311966));
#20489=CARTESIAN_POINT('Ctrl Pts',(44.1373302123194,46.0121654241522,48.8494280982201));
#20490=CARTESIAN_POINT('Ctrl Pts',(44.0735155958563,46.0026203357195,48.969111649272));
#20491=CARTESIAN_POINT('Ctrl Pts',(43.9562593991378,45.9876772060383,49.1423984061069));
#20492=CARTESIAN_POINT('Ctrl Pts',(43.9113000960647,45.9823794645922,49.201245268887));
#20493=CARTESIAN_POINT('Ctrl Pts',(43.8407992349202,45.9747807173391,49.2832800448694));
#20494=CARTESIAN_POINT('Ctrl Pts',(43.8178423605574,45.9724032487436,49.3085997964914));
#20495=CARTESIAN_POINT('Ctrl Pts',(43.7792581395926,45.9685785780702,49.3489471498493));
#20496=CARTESIAN_POINT('Ctrl Pts',(43.7640293725413,45.9671099460054,49.3643443102512));
#20497=CARTESIAN_POINT('Ctrl Pts',(43.7430175918665,45.9651422122111,49.3848848430884));
#20498=CARTESIAN_POINT('Ctrl Pts',(43.7374588396382,45.9646270503943,49.3902539832684));
#20499=CARTESIAN_POINT('Ctrl Pts',(43.7281119385911,45.96377004313,49.3991741101396));
#20500=CARTESIAN_POINT('Ctrl Pts',(43.7243414957307,45.9634268112735,49.4027434251052));
#20501=CARTESIAN_POINT('Ctrl Pts',(43.717159191793,45.9627777500421,49.4094878292393));
#20502=CARTESIAN_POINT('Ctrl Pts',(43.713750173869,45.9624716885591,49.4126658341993));
#20503=CARTESIAN_POINT('Ctrl Pts',(43.7056351133436,45.9617477737817,49.4201761941979));
#20504=CARTESIAN_POINT('Ctrl Pts',(43.7009189381864,45.9613307444905,49.424497592443));
#20505=CARTESIAN_POINT('Ctrl Pts',(43.6842415877539,45.9598685792411,49.439627027631));
#20506=CARTESIAN_POINT('Ctrl Pts',(43.6721661282368,45.9588323915648,49.4503088697083));
#20507=CARTESIAN_POINT('Ctrl Pts',(43.5721064605865,45.9504149280176,49.5366092719332));
#20508=CARTESIAN_POINT('Ctrl Pts',(43.4775865689455,45.9435081149933,49.6043117570513));
#20509=CARTESIAN_POINT('Ctrl Pts',(43.2556401245294,45.9281528071371,49.7347671176079));
#20510=CARTESIAN_POINT('Ctrl Pts',(43.1262459069658,45.9197209442377,49.7927903907055));
#20511=CARTESIAN_POINT('Ctrl Pts',(42.971863046181,45.909441680981,49.8425386709255));
#20512=CARTESIAN_POINT('Ctrl Pts',(42.9519434963435,45.9081123185111,49.8486033702171));
#20513=CARTESIAN_POINT('Ctrl Pts',(42.9215261486687,45.9060759294906,49.8573287771559));
#20514=CARTESIAN_POINT('Ctrl Pts',(42.9110972565773,45.9053765979035,49.860225603688));
#20515=CARTESIAN_POINT('Ctrl Pts',(42.8920909661993,45.9040997799575,49.8653330769768));
#20516=CARTESIAN_POINT('Ctrl Pts',(42.883521613515,45.903523253257,49.8675727166403));
#20517=CARTESIAN_POINT('Ctrl Pts',(42.8649659909922,45.9022728997538,49.8722860426369));
#20518=CARTESIAN_POINT('Ctrl Pts',(42.8549747884349,45.9015984219757,49.8747390040079));
#20519=CARTESIAN_POINT('Ctrl Pts',(42.827665385168,45.8997512544549,49.8812126286772));
#20520=CARTESIAN_POINT('Ctrl Pts',(42.8103108184844,45.8985734896732,49.8850739062596));
#20521=CARTESIAN_POINT('Ctrl Pts',(42.7142400244263,45.8920302070028,49.9050595489422));
#20522=CARTESIAN_POINT('Ctrl Pts',(42.6346392862302,45.8865171976895,49.9164915909003));
#20523=CARTESIAN_POINT('Ctrl Pts',(42.4273863164452,45.8719478317822,49.9331507666779));
#20524=CARTESIAN_POINT('Ctrl Pts',(42.2995080821002,45.8627327477398,49.9307303290074));
#20525=CARTESIAN_POINT('Ctrl Pts',(42.1103304009486,45.8492658560347,49.9082960729596));
#20526=CARTESIAN_POINT('Ctrl Pts',(42.0482340021057,45.8448784174493,49.8978316008014));
#20527=CARTESIAN_POINT('Ctrl Pts',(41.9762203374174,45.8399081365241,49.8820386963221));
#20528=CARTESIAN_POINT('Ctrl Pts',(41.9657056821016,45.8391854442231,49.8796402090588));
#20529=CARTESIAN_POINT('Ctrl Pts',(41.9495059548467,45.8380772443336,49.8758017091104));
#20530=CARTESIAN_POINT('Ctrl Pts',(41.943806608933,45.8376883654177,49.8744237858168));
#20531=CARTESIAN_POINT('Ctrl Pts',(41.9332744837574,45.8369717093823,49.8718265651099));
#20532=CARTESIAN_POINT('Ctrl Pts',(41.9284401570581,45.836643543229,49.8706145281224));
#20533=CARTESIAN_POINT('Ctrl Pts',(41.9173997080052,45.8358958385496,49.8678010046056));
#20534=CARTESIAN_POINT('Ctrl Pts',(41.9111968286981,45.8354770066366,49.8661873156985));
#20535=CARTESIAN_POINT('Ctrl Pts',(41.8949264291925,45.8343814082306,49.8618678569942));
#20536=CARTESIAN_POINT('Ctrl Pts',(41.8848724392048,45.8337074435762,49.8591113028894));
#20537=CARTESIAN_POINT('Ctrl Pts',(41.8477587930746,45.8312291232269,49.8486114673626));
#20538=CARTESIAN_POINT('Ctrl Pts',(41.8208516596979,45.8294512529434,49.840359045563));
#20539=CARTESIAN_POINT('Ctrl Pts',(41.7941388200938,45.8276962776015,49.831522532644));
#20540=CARTESIAN_POINT('Origin',(42.4,48.4493818343519,48.));
#20541=CARTESIAN_POINT('',(41.7941389732838,44.8639880114013,49.8315225833187));
#20542=CARTESIAN_POINT('',(41.7941386463292,45.0367815693785,49.8315224751633));
#20543=CARTESIAN_POINT('',(41.7941388317924,48.4493818343519,49.8315225365138));
#20544=CARTESIAN_POINT('Ctrl Pts',(41.7941389732838,44.8639880114013,49.8315225833187));
#20545=CARTESIAN_POINT('Ctrl Pts',(41.8398698956634,44.8668818440374,49.846650206553));
#20546=CARTESIAN_POINT('Ctrl Pts',(41.8861705002305,44.8697991318275,49.8600661076338));
#20547=CARTESIAN_POINT('Ctrl Pts',(41.987195043301,44.8761965318852,49.8852747529153));
#20548=CARTESIAN_POINT('Ctrl Pts',(42.0420030289712,44.8796874134856,49.8964456470235));
#20549=CARTESIAN_POINT('Ctrl Pts',(42.1126738968819,44.8842529772068,49.9076769320419));
#20550=CARTESIAN_POINT('Ctrl Pts',(42.1281616255028,44.885257362061,49.9099454027151));
#20551=CARTESIAN_POINT('Ctrl Pts',(42.1533100192657,44.8868951995562,49.9133167836511));
#20552=CARTESIAN_POINT('Ctrl Pts',(42.1629546314003,44.8875249740215,49.9145355960799));
#20553=CARTESIAN_POINT('Ctrl Pts',(42.1814988482933,44.8887392262738,49.9167368015385));
#20554=CARTESIAN_POINT('Ctrl Pts',(42.1903969080519,44.8893233383791,49.9177302362292));
#20555=CARTESIAN_POINT('Ctrl Pts',(42.2108006020702,44.8906662690512,49.9198645323047));
#20556=CARTESIAN_POINT('Ctrl Pts',(42.2223101304359,44.8914263733883,49.9209639598153));
#20557=CARTESIAN_POINT('Ctrl Pts',(42.2590193849076,44.8938592523921,49.9241378174312));
#20558=CARTESIAN_POINT('Ctrl Pts',(42.2842494384544,44.895544220105,49.9258202351666));
#20559=CARTESIAN_POINT('Ctrl Pts',(42.4449077647045,44.9063602266949,49.9333650423089));
#20560=CARTESIAN_POINT('Ctrl Pts',(42.5805804297497,44.9159247602421,49.9254337762438));
#20561=CARTESIAN_POINT('Ctrl Pts',(42.7593907784112,44.9288673617393,49.895909178815));
#20562=CARTESIAN_POINT('Ctrl Pts',(42.8042264033753,44.9321375976747,49.8868583536638));
#20563=CARTESIAN_POINT('Ctrl Pts',(42.9173064871559,44.9404014453769,49.8598152675831));
#20564=CARTESIAN_POINT('Ctrl Pts',(42.9849703497119,44.9453623117601,49.8396550121707));
#20565=CARTESIAN_POINT('Ctrl Pts',(43.0659262760286,44.9512060781462,49.8106141096855));
#20566=CARTESIAN_POINT('Ctrl Pts',(43.0804062625858,44.95224755208,49.8052225941129));
#20567=CARTESIAN_POINT('Ctrl Pts',(43.1011378809499,44.9537316834185,49.7972184306798));
#20568=CARTESIAN_POINT('Ctrl Pts',(43.1074425310783,44.9541820811108,49.7947460779557));
#20569=CARTESIAN_POINT('Ctrl Pts',(43.1184018790699,44.9549632048007,49.7903816744217));
#20570=CARTESIAN_POINT('Ctrl Pts',(43.1230623923128,44.9552948062442,49.7885045650316));
#20571=CARTESIAN_POINT('Ctrl Pts',(43.132939267181,44.9559962884962,49.7844815494626));
#20572=CARTESIAN_POINT('Ctrl Pts',(43.1381535870893,44.9563658846647,49.7823309607466));
#20573=CARTESIAN_POINT('Ctrl Pts',(43.1523623512064,44.9573711935071,49.7763976625225));
#20574=CARTESIAN_POINT('Ctrl Pts',(43.1613377958191,44.958004229339,49.7725694720773));
#20575=CARTESIAN_POINT('Ctrl Pts',(43.204591086721,44.9610469837814,49.753732007587));
#20576=CARTESIAN_POINT('Ctrl Pts',(43.2384588597062,44.9634054542435,49.7377945640908));
#20577=CARTESIAN_POINT('Ctrl Pts',(43.3037695258554,44.9679469868955,49.704706439237));
#20578=CARTESIAN_POINT('Ctrl Pts',(43.3352402502694,44.9701323076176,49.687646086652));
#20579=CARTESIAN_POINT('Ctrl Pts',(43.4661496168624,44.9792840951103,49.6118925269568));
#20580=CARTESIAN_POINT('Ctrl Pts',(43.5606875930777,44.9860608158762,49.5452113235434));
#20581=CARTESIAN_POINT('Ctrl Pts',(43.7133358743848,44.9981628238264,49.4155855601737));
#20582=CARTESIAN_POINT('Ctrl Pts',(43.7742775071717,45.0033789981259,49.3565000032995));
#20583=CARTESIAN_POINT('Ctrl Pts',(43.8429345203681,45.009893874573,49.280543786691));
#20584=CARTESIAN_POINT('Ctrl Pts',(43.8545587634623,45.0110210802375,49.2673244219021));
#20585=CARTESIAN_POINT('Ctrl Pts',(43.8725951222502,45.0128098567852,49.2462379802009));
#20586=CARTESIAN_POINT('Ctrl Pts',(43.8791290314647,45.0134663816525,49.2384759986026));
#20587=CARTESIAN_POINT('Ctrl Pts',(43.8912592133246,45.0147015357312,49.2238329853458));
#20588=CARTESIAN_POINT('Ctrl Pts',(43.8968698714679,45.015279556801,49.2169641740026));
#20589=CARTESIAN_POINT('Ctrl Pts',(43.909339580745,45.0165795360476,49.2014815140065));
#20590=CARTESIAN_POINT('Ctrl Pts',(43.9161726023265,45.0173025145723,49.192847194696));
#20591=CARTESIAN_POINT('Ctrl Pts',(43.9333973444211,45.0191526479047,49.1706946071235));
#20592=CARTESIAN_POINT('Ctrl Pts',(43.9436842617619,45.0202838823947,49.1570964294876));
#20593=CARTESIAN_POINT('Ctrl Pts',(44.0188823405807,45.0287544838903,49.0549050312242));
#20594=CARTESIAN_POINT('Ctrl Pts',(44.0762912976276,45.0363808800105,48.9610643696934));
#20595=CARTESIAN_POINT('Ctrl Pts',(44.190009037151,45.0544133392815,48.7336725165721));
#20596=CARTESIAN_POINT('Ctrl Pts',(44.2399044534812,45.064895377592,48.5976303356733));
#20597=CARTESIAN_POINT('Ctrl Pts',(44.2791559136267,45.0762321124881,48.4367631672591));
#20598=CARTESIAN_POINT('Ctrl Pts',(44.2838272226617,45.0776645053495,48.416153935323));
#20599=CARTESIAN_POINT('Ctrl Pts',(44.2897297771956,45.0795922974452,48.3879724506852));
#20600=CARTESIAN_POINT('Ctrl Pts',(44.2912557022966,45.0801029279679,48.3804643567441));
#20601=CARTESIAN_POINT('Ctrl Pts',(44.2937386974416,45.0809547573062,48.3678629581893));
#20602=CARTESIAN_POINT('Ctrl Pts',(44.2947200348704,45.0812973032588,48.3627745880688));
#20603=CARTESIAN_POINT('Ctrl Pts',(44.296547800727,45.0819466513567,48.353087607425));
#20604=CARTESIAN_POINT('Ctrl Pts',(44.2973980300129,45.0822536748889,48.3484897930068));
#20605=CARTESIAN_POINT('Ctrl Pts',(44.2993818293171,45.082982183284,48.3375394228986));
#20606=CARTESIAN_POINT('Ctrl Pts',(44.3005002682169,45.0834028197149,48.3311841315293));
#20607=CARTESIAN_POINT('Ctrl Pts',(44.3043565644849,45.0848897192833,48.3086085232795));
#20608=CARTESIAN_POINT('Ctrl Pts',(44.3069189175436,45.0859466357359,48.292358394215));
#20609=CARTESIAN_POINT('Ctrl Pts',(44.3242207553804,45.0936442291906,48.1727035328114));
#20610=CARTESIAN_POINT('Ctrl Pts',(44.3307502617323,45.0999036508947,48.0682727491889));
#20611=CARTESIAN_POINT('Ctrl Pts',(44.3268654816146,45.1122671283403,47.8611978901689));
#20612=CARTESIAN_POINT('Ctrl Pts',(44.3167544488062,45.1183552977951,47.7589035174432));
#20613=CARTESIAN_POINT('Ctrl Pts',(44.2881772097921,45.1282390460147,47.6003073763412));
#20614=CARTESIAN_POINT('Ctrl Pts',(44.2751848995508,45.1318877252281,47.5432200318192));
#20615=CARTESIAN_POINT('Ctrl Pts',(44.2553946794159,45.1366326841936,47.4715065336293));
#20616=CARTESIAN_POINT('Ctrl Pts',(44.2509812895333,45.1376514500592,47.4562509753491));
#20617=CARTESIAN_POINT('Ctrl Pts',(44.2435490814129,45.1393069480025,47.4317000659151));
#20618=CARTESIAN_POINT('Ctrl Pts',(44.240647036601,45.1399398509009,47.422369918148));
#20619=CARTESIAN_POINT('Ctrl Pts',(44.2349547552747,45.1411562109915,47.4045476517151));
#20620=CARTESIAN_POINT('Ctrl Pts',(44.2321761233734,45.1417392723439,47.3960520706386));
#20621=CARTESIAN_POINT('Ctrl Pts',(44.225700997738,45.143074264455,47.37671056611));
#20622=CARTESIAN_POINT('Ctrl Pts',(44.2219667386075,45.1438274296275,47.3658777363236));
#20623=CARTESIAN_POINT('Ctrl Pts',(44.2098735791232,45.1462154013271,47.3317851696141));
#20624=CARTESIAN_POINT('Ctrl Pts',(44.2011643454327,45.1478617745234,47.3086532448387));
#20625=CARTESIAN_POINT('Ctrl Pts',(44.1375653207158,45.1594056495137,47.1490989193369));
#20626=CARTESIAN_POINT('Ctrl Pts',(44.0676873412533,45.1698235696639,47.0191997957208));
#20627=CARTESIAN_POINT('Ctrl Pts',(43.9660478771651,45.1825406483707,46.8730578478913));
#20628=CARTESIAN_POINT('Ctrl Pts',(43.9477267553262,45.184756026245,46.8480249589085));
#20629=CARTESIAN_POINT('Ctrl Pts',(43.8949592907188,45.1909123904709,46.7794592000886));
#20630=CARTESIAN_POINT('Ctrl Pts',(43.8592238160372,45.1948328481501,46.7369521738713));
#20631=CARTESIAN_POINT('Ctrl Pts',(43.8012738187346,45.2007603701703,46.6737693665352));
#20632=CARTESIAN_POINT('Ctrl Pts',(43.780322902934,45.2028245805512,46.6519773964961));
#20633=CARTESIAN_POINT('Ctrl Pts',(43.752668615284,45.2054399702573,46.6245341028403));
#20634=CARTESIAN_POINT('Ctrl Pts',(43.746428216339,45.2060232392672,46.6184248545794));
#20635=CARTESIAN_POINT('Ctrl Pts',(43.7362521307988,45.2069629153701,46.6085970712434));
#20636=CARTESIAN_POINT('Ctrl Pts',(43.7323419845155,45.207321286438,46.6048524431727));
#20637=CARTESIAN_POINT('Ctrl Pts',(43.7247503434539,45.2080117828091,46.5976431838188));
#20638=CARTESIAN_POINT('Ctrl Pts',(43.7210709392342,45.2083440580805,46.59417650947));
#20639=CARTESIAN_POINT('Ctrl Pts',(43.712898802311,45.2090769073386,46.5865372712635));
#20640=CARTESIAN_POINT('Ctrl Pts',(43.7083996761453,45.2094769643848,46.5823715435207));
#20641=CARTESIAN_POINT('Ctrl Pts',(43.6923501818983,45.2108923429771,46.5676528580662));
#20642=CARTESIAN_POINT('Ctrl Pts',(43.6806910166339,45.2118991493485,46.5572186980029));
#20643=CARTESIAN_POINT('Ctrl Pts',(43.5696242051618,45.2213052624814,46.4602288497678));
#20644=CARTESIAN_POINT('Ctrl Pts',(43.4617034051146,45.2290836469037,46.3839207644328));
#20645=CARTESIAN_POINT('Ctrl Pts',(43.2367002990596,45.2444939674408,46.2571711885206));
#20646=CARTESIAN_POINT('Ctrl Pts',(43.1207562332192,45.2520884585251,46.2061147256893));
#20647=CARTESIAN_POINT('Ctrl Pts',(42.9806556589149,45.2614289947194,46.1602106864278));
#20648=CARTESIAN_POINT('Ctrl Pts',(42.9605455471921,45.2627727428097,46.1539841965971));
#20649=CARTESIAN_POINT('Ctrl Pts',(42.9299027869332,45.2648266811414,46.1450434610457));
#20650=CARTESIAN_POINT('Ctrl Pts',(42.9194420228465,45.2655289666295,46.1420870036765));
#20651=CARTESIAN_POINT('Ctrl Pts',(42.9004111326687,45.2668088848935,46.1368817131461));
#20652=CARTESIAN_POINT('Ctrl Pts',(42.8918493814899,45.2673855341446,46.1346031966285));
#20653=CARTESIAN_POINT('Ctrl Pts',(42.8733483998171,45.2686335387352,46.1298158035444));
#20654=CARTESIAN_POINT('Ctrl Pts',(42.8634042985811,45.2693055255943,46.1273270212236));
#20655=CARTESIAN_POINT('Ctrl Pts',(42.836320049723,45.2711392637996,46.1207773842127));
#20656=CARTESIAN_POINT('Ctrl Pts',(42.8191437063512,45.2723059699003,46.1168719258258));
#20657=CARTESIAN_POINT('Ctrl Pts',(42.7263409440724,45.2786316853696,46.0971035178727));
#20658=CARTESIAN_POINT('Ctrl Pts',(42.6498760283478,45.2839265978606,46.0855620508922));
#20659=CARTESIAN_POINT('Ctrl Pts',(42.4437516039078,45.2984055918514,46.0670097080172));
#20660=CARTESIAN_POINT('Ctrl Pts',(42.3137299875012,45.3077734802555,46.068441327191));
#20661=CARTESIAN_POINT('Ctrl Pts',(42.1210276436757,45.3214899659038,46.0900676012835));
#20662=CARTESIAN_POINT('Ctrl Pts',(42.05759392552,45.3259712159887,46.1004139302229));
#20663=CARTESIAN_POINT('Ctrl Pts',(41.984198889962,45.3310326835872,46.1161822519496));
#20664=CARTESIAN_POINT('Ctrl Pts',(41.9736284047895,45.3317585785719,46.118546533356));
#20665=CARTESIAN_POINT('Ctrl Pts',(41.9573578297607,45.3328705877415,46.1223299127065));
#20666=CARTESIAN_POINT('Ctrl Pts',(41.9516435718611,45.3332601110679,46.123686176777));
#20667=CARTESIAN_POINT('Ctrl Pts',(41.941092378712,45.3339773593169,46.126241428692));
#20668=CARTESIAN_POINT('Ctrl Pts',(41.9362539046264,45.3343054786297,46.1274330590362));
#20669=CARTESIAN_POINT('Ctrl Pts',(41.9252154842975,45.3350522851958,46.1301970346632));
#20670=CARTESIAN_POINT('Ctrl Pts',(41.9190187001121,45.3354702725699,46.1317814748847));
#20671=CARTESIAN_POINT('Ctrl Pts',(41.9027879344318,45.3365620512477,46.1360175894782));
#20672=CARTESIAN_POINT('Ctrl Pts',(41.8927671132211,45.3372330724177,46.1387195066591));
#20673=CARTESIAN_POINT('Ctrl Pts',(41.8124288367972,45.3425919004022,46.1610781569515));
#20674=CARTESIAN_POINT('Ctrl Pts',(41.7432485468824,45.3470787376706,46.1846340526797));
#20675=CARTESIAN_POINT('Ctrl Pts',(41.5707376055398,45.3583252030467,46.2545319286104));
#20676=CARTESIAN_POINT('Ctrl Pts',(41.469850011165,45.3649689275563,46.3061414331288));
#20677=CARTESIAN_POINT('Ctrl Pts',(41.3026373631626,45.3769035993675,46.4111477645204));
#20678=CARTESIAN_POINT('Ctrl Pts',(41.234237734677,45.3820928212337,46.4606326341144));
#20679=CARTESIAN_POINT('Ctrl Pts',(41.15576186563,45.3885773448957,46.525644855577));
#20680=CARTESIAN_POINT('Ctrl Pts',(41.14237800653,45.3897031330683,46.5370445954906));
#20681=CARTESIAN_POINT('Ctrl Pts',(41.1215225280144,45.3914901699157,46.5553060003055));
#20682=CARTESIAN_POINT('Ctrl Pts',(41.1139458138287,45.392146389433,46.5620465853046));
#20683=CARTESIAN_POINT('Ctrl Pts',(41.0998426445514,45.3933812784833,46.5747940224455));
#20684=CARTESIAN_POINT('Ctrl Pts',(41.0933037633589,45.3939593425192,46.5807867784933));
#20685=CARTESIAN_POINT('Ctrl Pts',(41.0787353997711,45.3952598270551,46.5943244301228));
#20686=CARTESIAN_POINT('Ctrl Pts',(41.070728815373,45.3959832713719,46.6018934015217));
#20687=CARTESIAN_POINT('Ctrl Pts',(41.0504815651611,45.3978353961448,46.6213651492942));
#20688=CARTESIAN_POINT('Ctrl Pts',(41.0383334891037,45.3989681713086,46.6333623967398));
#20689=CARTESIAN_POINT('Ctrl Pts',(40.9478693913633,45.4075703633746,46.7251069955365));
#20690=CARTESIAN_POINT('Ctrl Pts',(40.8764711158507,45.415337690854,46.8113505889491));
#20691=CARTESIAN_POINT('Ctrl Pts',(40.7318838554259,45.4333869109945,47.0205801787319));
#20692=CARTESIAN_POINT('Ctrl Pts',(40.6640738924162,45.4437280551725,47.1465141219001));
#20693=CARTESIAN_POINT('Ctrl Pts',(40.6028994213088,45.4549293865162,47.2982776550209));
#20694=CARTESIAN_POINT('Ctrl Pts',(40.5953568393628,45.4563547774798,47.3179091763951));
#20695=CARTESIAN_POINT('Ctrl Pts',(40.5855108314491,45.458274765749,47.3448434580625));
#20696=CARTESIAN_POINT('Ctrl Pts',(40.5829279363366,45.4587844399407,47.3520415464154));
#20697=CARTESIAN_POINT('Ctrl Pts',(40.5786676517651,45.4596351228711,47.3641400644745));
#20698=CARTESIAN_POINT('Ctrl Pts',(40.57696709049,45.4599774710929,47.3690321772976));
#20699=CARTESIAN_POINT('Ctrl Pts',(40.5737679546114,45.4606267876403,47.3783562437979));
#20700=CARTESIAN_POINT('Ctrl Pts',(40.5722657729137,45.4609339750591,47.3827868767312));
#20701=CARTESIAN_POINT('Ctrl Pts',(40.5687267477025,45.4616633089054,47.3933513343301));
#20702=CARTESIAN_POINT('Ctrl Pts',(40.5667045658399,45.4620846023614,47.3994900648957));
#20703=CARTESIAN_POINT('Ctrl Pts',(40.5596265980289,45.463576027856,47.4213456367223));
#20704=CARTESIAN_POINT('Ctrl Pts',(40.5547415929671,45.4646367393974,47.4371176091156));
#20705=CARTESIAN_POINT('Ctrl Pts',(40.5221195590718,45.4719605146159,47.5474346375059));
#20706=CARTESIAN_POINT('Ctrl Pts',(40.5014554624994,45.47788559347,47.6439326661028));
#20707=CARTESIAN_POINT('Ctrl Pts',(40.476742447857,45.4889088324802,47.8267677989799));
#20708=CARTESIAN_POINT('Ctrl Pts',(40.4709350396174,45.4940039414054,47.9126108422634));
#20709=CARTESIAN_POINT('Ctrl Pts',(40.4708124784275,45.5039038220345,48.075923570566));
#20710=CARTESIAN_POINT('Ctrl Pts',(40.4754090259402,45.5086773032843,48.1532199463386));
#20711=CARTESIAN_POINT('Ctrl Pts',(40.4867339793363,45.514718890139,48.2475200081008));
#20712=CARTESIAN_POINT('Ctrl Pts',(40.4890744726845,45.5158468482015,48.2649841811214));
#20713=CARTESIAN_POINT('Ctrl Pts',(40.4931546312366,45.5176430285859,48.2925549525971));
#20714=CARTESIAN_POINT('Ctrl Pts',(40.4947362608742,45.5183062448043,48.3026842220854));
#20715=CARTESIAN_POINT('Ctrl Pts',(40.4978350721116,45.5195474011195,48.3215425885675));
#20716=CARTESIAN_POINT('Ctrl Pts',(40.4993318027835,45.5201246761939,48.3302748080384));
#20717=CARTESIAN_POINT('Ctrl Pts',(40.5027985178214,45.521414444566,48.3496958998813));
#20718=CARTESIAN_POINT('Ctrl Pts',(40.5047987807237,45.5221278867066,48.3603789902236));
#20719=CARTESIAN_POINT('Ctrl Pts',(40.5109365138345,45.5242311736102,48.3916944021243));
#20720=CARTESIAN_POINT('Ctrl Pts',(40.515321310221,45.5256288560924,48.4122760432403));
#20721=CARTESIAN_POINT('Ctrl Pts',(40.5480012623231,45.5353790668902,48.55423449777));
#20722=CARTESIAN_POINT('Ctrl Pts',(40.5876591792554,45.5441016591821,48.6726704756848));
#20723=CARTESIAN_POINT('Ctrl Pts',(40.693027897489,45.5625175856761,48.9086875280277));
#20724=CARTESIAN_POINT('Ctrl Pts',(40.7601877728224,45.5721842801089,49.0249330887395));
#20725=CARTESIAN_POINT('Ctrl Pts',(40.847931341814,45.5823327182408,49.1458029629038));
#20726=CARTESIAN_POINT('Ctrl Pts',(40.8571635717543,45.583374836433,49.1582043612549));
#20727=CARTESIAN_POINT('Ctrl Pts',(40.8702465856935,45.5848148615061,49.1753443249718));
#20728=CARTESIAN_POINT('Ctrl Pts',(40.8739719874032,45.5852208686908,49.1801772316496));
#20729=CARTESIAN_POINT('Ctrl Pts',(40.8808210891446,45.5859598430739,49.1889758094864));
#20730=CARTESIAN_POINT('Ctrl Pts',(40.8839375426987,45.5862933085585,49.1929470510635));
#20731=CARTESIAN_POINT('Ctrl Pts',(40.8904371595074,45.5869829664163,49.201162789556));
#20732=CARTESIAN_POINT('Ctrl Pts',(40.8938226897472,45.5873389861354,49.2054052962811));
#20733=CARTESIAN_POINT('Ctrl Pts',(40.9027409297488,45.5882686227461,49.2164847660254));
#20734=CARTESIAN_POINT('Ctrl Pts',(40.9083026444419,45.5888402038468,49.2232983757347));
#20735=CARTESIAN_POINT('Ctrl Pts',(40.9335853435197,45.5914032329968,49.2538431622364));
#20736=CARTESIAN_POINT('Ctrl Pts',(40.9538285760658,45.5933598586195,49.2771386338879));
#20737=CARTESIAN_POINT('Ctrl Pts',(41.0132396447128,45.5988706950909,49.3422825298116));
#20738=CARTESIAN_POINT('Ctrl Pts',(41.0537265186962,45.6023544840896,49.3828866008304));
#20739=CARTESIAN_POINT('Ctrl Pts',(41.1903645942287,45.613506546293,49.5082222576587));
#20740=CARTESIAN_POINT('Ctrl Pts',(41.2931519328122,45.6210213861649,49.585193767332));
#20741=CARTESIAN_POINT('Ctrl Pts',(41.4548054575174,45.6325787446976,49.68280693578));
#20742=CARTESIAN_POINT('Ctrl Pts',(41.5082504530253,45.6363581631205,49.7117282288967));
#20743=CARTESIAN_POINT('Ctrl Pts',(41.578001678198,45.6412903976384,49.7453193950468));
#20744=CARTESIAN_POINT('Ctrl Pts',(41.5931295142146,45.642359986001,49.7523644092311));
#20745=CARTESIAN_POINT('Ctrl Pts',(41.6174174375653,45.6440779445414,49.7632940863347));
#20746=CARTESIAN_POINT('Ctrl Pts',(41.6265196983154,45.6447219326147,49.7673057796177));
#20747=CARTESIAN_POINT('Ctrl Pts',(41.6438219097779,45.6459465636218,49.7747722167485));
#20748=CARTESIAN_POINT('Ctrl Pts',(41.6520155563738,45.6465267082801,49.7782409828505));
#20749=CARTESIAN_POINT('Ctrl Pts',(41.6706870478752,45.6478493449199,49.7859936473494));
#20750=CARTESIAN_POINT('Ctrl Pts',(41.6811791120757,45.6485930122819,49.7902422216799));
#20751=CARTESIAN_POINT('Ctrl Pts',(41.7134026637587,45.6508786629668,49.8029616348139));
#20752=CARTESIAN_POINT('Ctrl Pts',(41.7352502195506,45.6524306791987,49.811130643188));
#20753=CARTESIAN_POINT('Ctrl Pts',(41.7694986777515,45.6548682623836,49.823233306061));
#20754=CARTESIAN_POINT('Ctrl Pts',(41.7817990312338,45.6557446311092,49.8274405743698));
#20755=CARTESIAN_POINT('Ctrl Pts',(41.7941388553004,45.6566247686891,49.8315225442902));
#20756=CARTESIAN_POINT('Ctrl Pts',(41.7941388200938,45.8276962776015,49.831522532644));
#20757=CARTESIAN_POINT('Ctrl Pts',(41.7489977681372,45.8247306088719,49.8165900322171));
#20758=CARTESIAN_POINT('Ctrl Pts',(41.7044115598008,45.8218301431025,49.7999895810198));
#20759=CARTESIAN_POINT('Ctrl Pts',(41.5580371350285,45.8122670972022,49.7392359799271));
#20760=CARTESIAN_POINT('Ctrl Pts',(41.4594588335036,45.805747466061,49.6879651314237));
#20761=CARTESIAN_POINT('Ctrl Pts',(41.2950929966855,45.7939753970559,49.5835860715604));
#20762=CARTESIAN_POINT('Ctrl Pts',(41.2273653028119,45.7888183151641,49.5341087327945));
#20763=CARTESIAN_POINT('Ctrl Pts',(41.1496054568406,45.7823701883531,49.4691371783181));
#20764=CARTESIAN_POINT('Ctrl Pts',(41.1362923021391,45.7812463033521,49.457701404249));
#20765=CARTESIAN_POINT('Ctrl Pts',(41.1155416898174,45.77946171098,49.4393790612813));
#20766=CARTESIAN_POINT('Ctrl Pts',(41.1079990952252,45.7788060107802,49.4326126092577));
#20767=CARTESIAN_POINT('Ctrl Pts',(41.0939561691918,45.7775717500974,49.4198136174763));
#20768=CARTESIAN_POINT('Ctrl Pts',(41.0874434241676,45.776993791775,49.4137950442593));
#20769=CARTESIAN_POINT('Ctrl Pts',(41.0729289061825,45.7756930858404,49.4001951188175));
#20770=CARTESIAN_POINT('Ctrl Pts',(41.0649502044251,45.7749693110674,49.3925897075417));
#20771=CARTESIAN_POINT('Ctrl Pts',(41.0447652354103,45.7731154485877,49.3730162083826));
#20772=CARTESIAN_POINT('Ctrl Pts',(41.0326522821825,45.7719812515221,49.3609536957905));
#20773=CARTESIAN_POINT('Ctrl Pts',(40.9416560245141,45.7632913007043,49.2678951898616));
#20774=CARTESIAN_POINT('Ctrl Pts',(40.8698837376074,45.7554303064388,49.1802802796323));
#20775=CARTESIAN_POINT('Ctrl Pts',(40.7265461758084,45.7373683076527,48.9700948195896));
#20776=CARTESIAN_POINT('Ctrl Pts',(40.6599691194015,45.7271186641324,48.8448829963908));
#20777=CARTESIAN_POINT('Ctrl Pts',(40.5999204901637,45.7160055748317,48.6940429483817));
#20778=CARTESIAN_POINT('Ctrl Pts',(40.5924858079949,45.714584924637,48.6744437636442));
#20779=CARTESIAN_POINT('Ctrl Pts',(40.5827800386299,45.712670323389,48.6475434192508));
#20780=CARTESIAN_POINT('Ctrl Pts',(40.58023102428,45.7121613976206,48.640345022382));
#20781=CARTESIAN_POINT('Ctrl Pts',(40.5760261330969,45.7113116896684,48.6282425307444));
#20782=CARTESIAN_POINT('Ctrl Pts',(40.574347147764,45.710969573438,48.6233466209235));
#20783=CARTESIAN_POINT('Ctrl Pts',(40.5711881457038,45.710320503492,48.6140127384059));
#20784=CARTESIAN_POINT('Ctrl Pts',(40.5697045414466,45.7100133321267,48.6095760632656));
#20785=CARTESIAN_POINT('Ctrl Pts',(40.5662086038631,45.7092837849661,48.5989937308895));
#20786=CARTESIAN_POINT('Ctrl Pts',(40.564210987921,45.7088622642186,48.5928432172652));
#20787=CARTESIAN_POINT('Ctrl Pts',(40.5572145463655,45.7073687434576,48.5709271951168));
#20788=CARTESIAN_POINT('Ctrl Pts',(40.5523874076705,45.7063062012436,48.5551070554506));
#20789=CARTESIAN_POINT('Ctrl Pts',(40.5203611666367,45.699012211015,48.4450972738243));
#20790=CARTESIAN_POINT('Ctrl Pts',(40.5001697562934,45.6931151635944,48.3490038090651));
#20791=CARTESIAN_POINT('Ctrl Pts',(40.4764463287328,45.6822542611877,48.1687912774779));
#20792=CARTESIAN_POINT('Ctrl Pts',(40.47093461263,45.6772914720765,48.085179266282));
#20793=CARTESIAN_POINT('Ctrl Pts',(40.4708094838832,45.6673906846146,47.9216505663629));
#20794=CARTESIAN_POINT('Ctrl Pts',(40.475702984479,45.6624718590081,47.8419070117054));
#20795=CARTESIAN_POINT('Ctrl Pts',(40.4877035742627,45.656267122446,47.7450883727929));
#20796=CARTESIAN_POINT('Ctrl Pts',(40.4901296537454,45.6551311012319,47.7275063591347));
#20797=CARTESIAN_POINT('Ctrl Pts',(40.4943432878256,45.6533250808875,47.699798893423));
#20798=CARTESIAN_POINT('Ctrl Pts',(40.4959698308078,45.6526601847964,47.6896496865439));
#20799=CARTESIAN_POINT('Ctrl Pts',(40.4991483174403,45.6514177228355,47.6707829985948));
#20800=CARTESIAN_POINT('Ctrl Pts',(40.5006793288481,45.6508408377371,47.6620622293506));
#20801=CARTESIAN_POINT('Ctrl Pts',(40.5042156487209,45.6495542969478,47.6427025689079));
#20802=CARTESIAN_POINT('Ctrl Pts',(40.5062505783723,45.6488437124804,47.6320694620345));
#20803=CARTESIAN_POINT('Ctrl Pts',(40.5124652258416,45.6467564699514,47.6010143447037));
#20804=CARTESIAN_POINT('Ctrl Pts',(40.5168864683117,45.6453721507834,47.5806428188978));
#20805=CARTESIAN_POINT('Ctrl Pts',(40.5276790478715,45.6422031985392,47.5345327916235));
#20806=CARTESIAN_POINT('Ctrl Pts',(40.5342525579553,45.6404124040772,47.5088464234966));
#20807=CARTESIAN_POINT('Ctrl Pts',(40.558027952774,45.6343629303525,47.4233220039839));
#20808=CARTESIAN_POINT('Ctrl Pts',(40.5775952014722,45.6300346199068,47.3641871325198));
#20809=CARTESIAN_POINT('Ctrl Pts',(40.6495160875748,45.6159416073177,47.1776187010271));
#20810=CARTESIAN_POINT('Ctrl Pts',(40.7126590167087,45.6059566083774,47.0548102430191));
#20811=CARTESIAN_POINT('Ctrl Pts',(40.81081958499,45.5934885436024,46.9055952513964));
#20812=CARTESIAN_POINT('Ctrl Pts',(40.8343864089518,45.5906716136456,46.8721388424947));
#20813=CARTESIAN_POINT('Ctrl Pts',(40.8649789972531,45.5872481534987,46.8315173034448));
#20814=CARTESIAN_POINT('Ctrl Pts',(40.8710180937537,45.5865829558754,46.8236260663398));
#20815=CARTESIAN_POINT('Ctrl Pts',(40.8806392180626,45.5855402262731,46.8112534862332));
#20816=CARTESIAN_POINT('Ctrl Pts',(40.8841806207593,45.5851599724916,46.8067409873243));
#20817=CARTESIAN_POINT('Ctrl Pts',(40.8905355334103,45.5844840406398,46.7987174259746));
#20818=CARTESIAN_POINT('Ctrl Pts',(40.8933411902295,45.5841878306637,46.7952004191194));
#20819=CARTESIAN_POINT('Ctrl Pts',(40.9001131840279,45.5834781154442,46.7867720961225));
#20820=CARTESIAN_POINT('Ctrl Pts',(40.9040913511106,45.5830654649129,46.781870399162));
#20821=CARTESIAN_POINT('Ctrl Pts',(40.9163258306319,45.5818090525843,46.766946014074));
#20822=CARTESIAN_POINT('Ctrl Pts',(40.9246595387772,45.5809706381401,46.7569868388791));
#20823=CARTESIAN_POINT('Ctrl Pts',(40.944323590172,45.579030372814,46.7339637661276));
#20824=CARTESIAN_POINT('Ctrl Pts',(40.9557304350497,45.5779334347124,46.7209663708862));
#20825=CARTESIAN_POINT('Ctrl Pts',(40.9964310881122,45.5741110696445,46.6758294039647));
#20826=CARTESIAN_POINT('Ctrl Pts',(41.0266368444325,45.5714365422141,46.6445267970164));
#20827=CARTESIAN_POINT('Ctrl Pts',(41.1511360491969,45.5609083055487,46.5239453851308));
#20828=CARTESIAN_POINT('Ctrl Pts',(41.2532761570946,45.5533199073216,46.4432646421649));
#20829=CARTESIAN_POINT('Ctrl Pts',(41.4277418456405,45.5407746083559,46.332007670501));
#20830=CARTESIAN_POINT('Ctrl Pts',(41.495152913795,45.5360182048485,46.2944989036598));
#20831=CARTESIAN_POINT('Ctrl Pts',(41.5804869479239,45.5299959864769,46.2535033004219));
#20832=CARTESIAN_POINT('Ctrl Pts',(41.5964555366025,45.5288691984128,46.2460990260106));
#20833=CARTESIAN_POINT('Ctrl Pts',(41.6218765272562,45.5270745653844,46.2347319171563));
#20834=CARTESIAN_POINT('Ctrl Pts',(41.63126328474,45.5264117132499,46.2306240085761));
#20835=CARTESIAN_POINT('Ctrl Pts',(41.6488248249132,45.5251710452032,46.223104710125));
#20836=CARTESIAN_POINT('Ctrl Pts',(41.6569912749836,45.5245938922403,46.2196744553361));
#20837=CARTESIAN_POINT('Ctrl Pts',(41.675231641057,45.5233041496136,46.2121600901749));
#20838=CARTESIAN_POINT('Ctrl Pts',(41.6853169737672,45.5225906095605,46.2081046679377));
#20839=CARTESIAN_POINT('Ctrl Pts',(41.715038898919,45.5204862375377,46.196443992078));
#20840=CARTESIAN_POINT('Ctrl Pts',(41.7347658445182,45.5190875539711,46.1890749761293));
#20841=CARTESIAN_POINT('Ctrl Pts',(41.8757045399072,45.5090771493632,46.1390408054126));
#20842=CARTESIAN_POINT('Ctrl Pts',(42.000770137031,45.5000700780431,46.1082655919083));
#20843=CARTESIAN_POINT('Ctrl Pts',(42.2561085335451,45.4816810415333,46.0718927286004));
#20844=CARTESIAN_POINT('Ctrl Pts',(42.3857958121912,45.4723477900513,46.0665818330857));
#20845=CARTESIAN_POINT('Ctrl Pts',(42.5304771985306,45.4624946242331,46.0752254011924));
#20846=CARTESIAN_POINT('Ctrl Pts',(42.5458982312289,45.4614519024199,46.0763328513661));
#20847=CARTESIAN_POINT('Ctrl Pts',(42.5675668540677,45.4599988110093,46.0781510478549));
#20848=CARTESIAN_POINT('Ctrl Pts',(42.573826343241,45.4595804713035,46.0787070888152));
#20849=CARTESIAN_POINT('Ctrl Pts',(42.5851541006439,45.4588261112817,46.0797691657242));
#20850=CARTESIAN_POINT('Ctrl Pts',(42.5902232876689,45.4584895171886,46.0802647055171));
#20851=CARTESIAN_POINT('Ctrl Pts',(42.6006092098813,45.4578019859752,46.0813215270133));
#20852=CARTESIAN_POINT('Ctrl Pts',(42.6059256638783,45.4574511642822,46.081884841704));
#20853=CARTESIAN_POINT('Ctrl Pts',(42.619618840437,45.4565503054413,46.0833933156804));
#20854=CARTESIAN_POINT('Ctrl Pts',(42.6279919413212,45.4560020790462,46.0843713046243));
#20855=CARTESIAN_POINT('Ctrl Pts',(42.6634995861571,45.453687369906,46.0887547548131));
#20856=CARTESIAN_POINT('Ctrl Pts',(42.6905679904396,45.4519479713485,46.0926822902659));
#20857=CARTESIAN_POINT('Ctrl Pts',(42.7646240909343,45.4472358358481,46.1050409072191));
#20858=CARTESIAN_POINT('Ctrl Pts',(42.8113984083784,45.444311379968,46.1146425615657));
#20859=CARTESIAN_POINT('Ctrl Pts',(43.0035449543937,45.4323386791839,46.1615784116989));
#20860=CARTESIAN_POINT('Ctrl Pts',(43.144662755547,45.4236015350582,46.2140718997319));
#20861=CARTESIAN_POINT('Ctrl Pts',(43.3262628813893,45.4110603700198,46.3069303546737));
#20862=CARTESIAN_POINT('Ctrl Pts',(43.3731994891942,45.4076941509458,46.3334677644867));
#20863=CARTESIAN_POINT('Ctrl Pts',(43.4325736486908,45.4032352545222,46.3704015101339));
#20864=CARTESIAN_POINT('Ctrl Pts',(43.4460802380752,45.4022069742332,46.3790386529662));
#20865=CARTESIAN_POINT('Ctrl Pts',(43.4676688787885,45.4005399064253,46.3932262745587));
#20866=CARTESIAN_POINT('Ctrl Pts',(43.4758191912984,45.3999050501457,46.398671894573));
#20867=CARTESIAN_POINT('Ctrl Pts',(43.4913117944252,45.3986875439046,46.4091949182841));
#20868=CARTESIAN_POINT('Ctrl Pts',(43.4986610548828,45.3981053098013,46.4142616474892));
#20869=CARTESIAN_POINT('Ctrl Pts',(43.515462585929,45.3967632773241,46.4260178314029));
#20870=CARTESIAN_POINT('Ctrl Pts',(43.5248902415259,45.3960021714471,46.4327416989466));
#20871=CARTESIAN_POINT('Ctrl Pts',(43.5542449384474,45.3936065263311,46.4540789782047));
#20872=CARTESIAN_POINT('Ctrl Pts',(43.5739514148156,45.3919604951448,46.4689901494618));
#20873=CARTESIAN_POINT('Ctrl Pts',(43.6725807221521,45.3835238981142,46.5466432882947));
#20874=CARTESIAN_POINT('Ctrl Pts',(43.7467729208159,45.37650581243,46.6151156927379));
#20875=CARTESIAN_POINT('Ctrl Pts',(43.8881086712195,45.3617527021093,46.7676992699086));
#20876=CARTESIAN_POINT('Ctrl Pts',(43.9542684869372,45.3540253734483,46.8522709551391));
#20877=CARTESIAN_POINT('Ctrl Pts',(44.0415902873666,45.3428296613133,46.9853920178565));
#20878=CARTESIAN_POINT('Ctrl Pts',(44.0683515555887,45.3392233670434,47.030024653293));
#20879=CARTESIAN_POINT('Ctrl Pts',(44.0983698816432,45.3349998218833,47.085016266002));
#20880=CARTESIAN_POINT('Ctrl Pts',(44.1033845808426,45.3342876447707,47.0943861359691));
#20881=CARTESIAN_POINT('Ctrl Pts',(44.1110594187255,45.3331877933222,47.109015740703));
#20882=CARTESIAN_POINT('Ctrl Pts',(44.1137732235806,45.3327969021908,47.1142468599179));
#20883=CARTESIAN_POINT('Ctrl Pts',(44.1187358001713,45.332078519209,47.123920893659));
#20884=CARTESIAN_POINT('Ctrl Pts',(44.120991339839,45.3317506208461,47.1283600740341));
#20885=CARTESIAN_POINT('Ctrl Pts',(44.1260907057081,45.3310060767611,47.1384932164202));
#20886=CARTESIAN_POINT('Ctrl Pts',(44.1289235608454,45.3305901150827,47.1441925531458));
#20887=CARTESIAN_POINT('Ctrl Pts',(44.1375674299662,45.3293132745692,47.1618009944639));
#20888=CARTESIAN_POINT('Ctrl Pts',(44.1432841331289,45.3284579993905,47.1737563305823));
#20889=CARTESIAN_POINT('Ctrl Pts',(44.1563689329494,45.3264723093262,47.2018610565474));
#20890=CARTESIAN_POINT('Ctrl Pts',(44.1636383415871,45.3253471308104,47.2180553407334));
#20891=CARTESIAN_POINT('Ctrl Pts',(44.1886366498586,45.3213893528808,47.275867645118));
#20892=CARTESIAN_POINT('Ctrl Pts',(44.2051251860031,45.3186116335538,47.3180085415979));
#20893=CARTESIAN_POINT('Ctrl Pts',(44.2645540311461,45.307734891404,47.4872034281112));
#20894=CARTESIAN_POINT('Ctrl Pts',(44.295679724053,45.2999042048776,47.618002197373));
#20895=CARTESIAN_POINT('Ctrl Pts',(44.322143666168,45.287433565727,47.821295973615));
#20896=CARTESIAN_POINT('Ctrl Pts',(44.3274124934296,45.2830440644208,47.8920611610014));
#20897=CARTESIAN_POINT('Ctrl Pts',(44.3291048587296,45.2774356689934,47.9801647132384));
#20898=CARTESIAN_POINT('Ctrl Pts',(44.3292050461932,45.2763330349727,47.9973820917729));
#20899=CARTESIAN_POINT('Ctrl Pts',(44.3289978932785,45.2745683623532,48.0247564996777));
#20900=CARTESIAN_POINT('Ctrl Pts',(44.3288407820625,45.2739110362639,48.0349140006813));
#20901=CARTESIAN_POINT('Ctrl Pts',(44.3283963518383,45.2726753780757,48.0539319003905));
#20902=CARTESIAN_POINT('Ctrl Pts',(44.3281281688722,45.2720976623275,48.0627925126045));
#20903=CARTESIAN_POINT('Ctrl Pts',(44.3273909172916,45.2707996919707,48.0826286071421));
#20904=CARTESIAN_POINT('Ctrl Pts',(44.3268891508784,45.2700784287953,48.0936024919549));
#20905=CARTESIAN_POINT('Ctrl Pts',(44.3251211584243,45.2679281089409,48.1261704397063));
#20906=CARTESIAN_POINT('Ctrl Pts',(44.32358546829,45.2664906714876,48.1477475401696));
#20907=CARTESIAN_POINT('Ctrl Pts',(44.309487861616,45.2557309063079,48.3077725119865));
#20908=CARTESIAN_POINT('Ctrl Pts',(44.282358252401,45.2459408543432,48.4445011344404));
#20909=CARTESIAN_POINT('Ctrl Pts',(44.2057510946412,45.2276560812585,48.6888554031354));
#20910=CARTESIAN_POINT('Ctrl Pts',(44.1606086885483,45.2192499903552,48.797195512021));
#20911=CARTESIAN_POINT('Ctrl Pts',(44.0984035199583,45.2101851302243,48.9150009324215));
#20912=CARTESIAN_POINT('Ctrl Pts',(44.0907158883632,45.2090996016342,48.9291291886891));
#20913=CARTESIAN_POINT('Ctrl Pts',(44.0797278534584,45.2075971985535,48.9487348063231));
#20914=CARTESIAN_POINT('Ctrl Pts',(44.076575811688,45.2071716466355,48.954293951014));
#20915=CARTESIAN_POINT('Ctrl Pts',(44.0710780736071,45.2064388474913,48.9638787968176));
#20916=CARTESIAN_POINT('Ctrl Pts',(44.0687453346064,45.2061307912994,48.9679118102561));
#20917=CARTESIAN_POINT('Ctrl Pts',(44.0637790958118,45.2054810748599,48.9764264933086));
#20918=CARTESIAN_POINT('Ctrl Pts',(44.0611420482365,45.205139656731,48.9809060471412));
#20919=CARTESIAN_POINT('Ctrl Pts',(44.0545314160587,45.2042924862137,48.9920324178202));
#20920=CARTESIAN_POINT('Ctrl Pts',(44.0505358027342,45.203788145542,48.9986661572501));
#20921=CARTESIAN_POINT('Ctrl Pts',(44.0351714953321,45.2018771466587,49.0238307303909));
#20922=CARTESIAN_POINT('Ctrl Pts',(44.0235292984774,45.2004871776679,49.0421937905191));
#20923=CARTESIAN_POINT('Ctrl Pts',(43.9926964132392,45.1969411641667,49.0890550040385));
#20924=CARTESIAN_POINT('Ctrl Pts',(43.9730499196481,45.1948090219009,49.1172452265651));
#20925=CARTESIAN_POINT('Ctrl Pts',(43.9082961687356,45.1881195133178,49.2050614472613));
#20926=CARTESIAN_POINT('Ctrl Pts',(43.860470482017,45.183662345675,49.2625995486546));
#20927=CARTESIAN_POINT('Ctrl Pts',(43.717904714341,45.1712090064643,49.4151448160633));
#20928=CARTESIAN_POINT('Ctrl Pts',(43.6164413348958,45.1632180832521,49.5032540561617));
#20929=CARTESIAN_POINT('Ctrl Pts',(43.4859211967136,45.1531706934503,49.5946659543404));
#20930=CARTESIAN_POINT('Ctrl Pts',(43.4648871807527,45.1515591450046,49.6087882235412));
#20931=CARTESIAN_POINT('Ctrl Pts',(43.4338520340445,45.1491890314014,49.6287499393738));
#20932=CARTESIAN_POINT('Ctrl Pts',(43.4240662209804,45.1484427960548,49.6349204135836));
#20933=CARTESIAN_POINT('Ctrl Pts',(43.4066104754436,45.1471132972055,49.6457089812219));
#20934=CARTESIAN_POINT('Ctrl Pts',(43.3989627180196,45.1465313585298,49.6503624400774));
#20935=CARTESIAN_POINT('Ctrl Pts',(43.3829497462801,45.1453138735764,49.6599538275377));
#20936=CARTESIAN_POINT('Ctrl Pts',(43.3745790892171,45.1446779968262,49.6648821298427));
#20937=CARTESIAN_POINT('Ctrl Pts',(43.3526465185876,45.1430131288837,49.6775730524158));
#20938=CARTESIAN_POINT('Ctrl Pts',(43.3390271023177,45.1419805192434,49.6852343493212));
#20939=CARTESIAN_POINT('Ctrl Pts',(43.2764859092685,45.1372431103501,49.7194219773386));
#20940=CARTESIAN_POINT('Ctrl Pts',(43.2265279131259,45.1334699055616,49.7439868200236));
#20941=CARTESIAN_POINT('Ctrl Pts',(43.0774150120444,45.1222336249694,49.8094601941863));
#20942=CARTESIAN_POINT('Ctrl Pts',(42.9758352934972,45.1145999424436,49.8443010347653));
#20943=CARTESIAN_POINT('Ctrl Pts',(42.7718302572124,45.0995693186419,49.8957679647394));
#20944=CARTESIAN_POINT('Ctrl Pts',(42.6698857023353,45.0922009072282,49.9129453151854));
#20945=CARTESIAN_POINT('Ctrl Pts',(42.5506247950813,45.0840505529895,49.9233113329774));
#20946=CARTESIAN_POINT('Ctrl Pts',(42.5341834004405,45.0829374128404,49.9245282985785));
#20947=CARTESIAN_POINT('Ctrl Pts',(42.5112819606707,45.0814032999862,49.9259284996786));
#20948=CARTESIAN_POINT('Ctrl Pts',(42.5048341004224,45.0809731796702,49.9262902364359));
#20949=CARTESIAN_POINT('Ctrl Pts',(42.4937144086169,45.0802346665316,49.9268580727464));
#20950=CARTESIAN_POINT('Ctrl Pts',(42.4890434708682,45.0799254357074,49.9270795739557));
#20951=CARTESIAN_POINT('Ctrl Pts',(42.4791981290499,45.079275792214,49.9275105785724));
#20952=CARTESIAN_POINT('Ctrl Pts',(42.4740236063068,45.0789356074953,49.9277162345491));
#20953=CARTESIAN_POINT('Ctrl Pts',(42.4612038369691,45.0780957795509,49.9281740479059));
#20954=CARTESIAN_POINT('Ctrl Pts',(42.4535576966618,45.0775974950056,49.9284015781585));
#20955=CARTESIAN_POINT('Ctrl Pts',(42.4248635830673,45.075736691758,49.9290846462127));
#20956=CARTESIAN_POINT('Ctrl Pts',(42.4038090765643,45.0743897555934,49.9292411329202));
#20957=CARTESIAN_POINT('Ctrl Pts',(42.2397012633488,45.064005512162,49.9277740885052));
#20958=CARTESIAN_POINT('Ctrl Pts',(42.0972143712163,45.0556417455269,49.9105864390193));
#20959=CARTESIAN_POINT('Ctrl Pts',(41.9026455049927,45.0436772849884,49.8647804534868));
#20960=CARTESIAN_POINT('Ctrl Pts',(41.8479982187459,45.0402578482943,49.8493390370101));
#20961=CARTESIAN_POINT('Ctrl Pts',(41.7941386463292,45.0367815693785,49.8315224751633));
#20962=CARTESIAN_POINT('Origin',(42.4,48.4493818343519,48.));
#20963=CARTESIAN_POINT('',(41.7941388317924,44.0726550104672,49.8315225365138));
#20964=CARTESIAN_POINT('',(41.7941385063105,44.2430936274184,49.8315224288456));
#20965=CARTESIAN_POINT('',(41.7941388317924,48.4493818343519,49.8315225365138));
#20966=CARTESIAN_POINT('',(40.4708695925604,44.7082214075913,47.9993794804437));
#20967=CARTESIAN_POINT('Ctrl Pts',(41.7941388317924,44.0726550104672,49.8315225365139));
#20968=CARTESIAN_POINT('Ctrl Pts',(41.7945517649514,44.0726835015639,49.8316591333403));
#20969=CARTESIAN_POINT('Ctrl Pts',(41.7949647447895,44.0727119845503,49.8317955906776));
#20970=CARTESIAN_POINT('Ctrl Pts',(41.802644360629,44.073241433279,49.8343302189699));
#20971=CARTESIAN_POINT('Ctrl Pts',(41.8099253057731,44.0737399005649,49.8366853220383));
#20972=CARTESIAN_POINT('Ctrl Pts',(41.8372994073923,44.0756015690712,49.8453601986768));
#20973=CARTESIAN_POINT('Ctrl Pts',(41.857482462897,44.0769491718269,49.8513943474694));
#20974=CARTESIAN_POINT('Ctrl Pts',(42.0156298450244,44.0873438253,49.8958673529716));
#20975=CARTESIAN_POINT('Ctrl Pts',(42.1574054013445,44.0957159842479,49.9191697108434));
#20976=CARTESIAN_POINT('Ctrl Pts',(42.4114178390357,44.1109409903733,49.9322925708581));
#20977=CARTESIAN_POINT('Ctrl Pts',(42.5226388205094,44.117681368905,49.9284293729212));
#20978=CARTESIAN_POINT('Ctrl Pts',(42.6498408732625,44.1258206152839,49.9129593041016));
#20979=CARTESIAN_POINT('Ctrl Pts',(42.6667522275056,44.1269112056682,49.9106744831074));
#20980=CARTESIAN_POINT('Ctrl Pts',(42.6945261795634,44.1287173643948,49.9065461500971));
#20981=CARTESIAN_POINT('Ctrl Pts',(42.705407473475,44.1294287994772,49.9048333679679));
#20982=CARTESIAN_POINT('Ctrl Pts',(42.7250226997228,44.1307184363763,49.9015734189465));
#20983=CARTESIAN_POINT('Ctrl Pts',(42.7337618230621,44.1312955816007,49.9000590159322));
#20984=CARTESIAN_POINT('Ctrl Pts',(42.7524718432505,44.132536891767,49.896683693981));
#20985=CARTESIAN_POINT('Ctrl Pts',(42.7624390922706,44.133201630543,49.8948042993963));
#20986=CARTESIAN_POINT('Ctrl Pts',(42.7896488916594,44.1350260328383,49.8894511542574));
#20987=CARTESIAN_POINT('Ctrl Pts',(42.8068591359874,44.136190683925,49.885820121738));
#20988=CARTESIAN_POINT('Ctrl Pts',(42.9064655863125,44.1429955197182,49.8633781252769));
#20989=CARTESIAN_POINT('Ctrl Pts',(42.9875927801679,44.1488004029118,49.8394065883173));
#20990=CARTESIAN_POINT('Ctrl Pts',(43.1738108736867,44.162728713393,49.7708037158923));
#20991=CARTESIAN_POINT('Ctrl Pts',(43.2770394165051,44.1709359854015,49.7220128398442));
#20992=CARTESIAN_POINT('Ctrl Pts',(43.4374301565022,44.1841297680354,49.6280229484996));
#20993=CARTESIAN_POINT('Ctrl Pts',(43.497434281177,44.1891738650293,49.5881940683947));
#20994=CARTESIAN_POINT('Ctrl Pts',(43.5634021499765,44.1947343333016,49.5388781643702));
#20995=CARTESIAN_POINT('Ctrl Pts',(43.5716758815666,44.1954319769836,49.5325880749808));
#20996=CARTESIAN_POINT('Ctrl Pts',(43.5849621858427,44.1965521446186,49.5223167011967));
#20997=CARTESIAN_POINT('Ctrl Pts',(43.5900063542189,44.1969773855264,49.5183768967088));
#20998=CARTESIAN_POINT('Ctrl Pts',(43.5989429662581,44.1977305742534,49.5113249665319));
#20999=CARTESIAN_POINT('Ctrl Pts',(43.6028430539011,44.198059202322,49.5082227887224));
#21000=CARTESIAN_POINT('Ctrl Pts',(43.611310724128,44.1987725191218,49.5014337612527));
#21001=CARTESIAN_POINT('Ctrl Pts',(43.6158735218903,44.1991567896593,49.4977411628335));
#21002=CARTESIAN_POINT('Ctrl Pts',(43.6287960694453,44.2002450515145,49.4871851816739));
#21003=CARTESIAN_POINT('Ctrl Pts',(43.6371152099097,44.2009455793342,49.4802721085683));
#21004=CARTESIAN_POINT('Ctrl Pts',(43.6941082232893,44.2057478818581,49.432095736227));
#21005=CARTESIAN_POINT('Ctrl Pts',(43.7407722777431,44.2096961072876,49.3885048882845));
#21006=CARTESIAN_POINT('Ctrl Pts',(43.8751461366115,44.2214273440893,49.2498758732937));
#21007=CARTESIAN_POINT('Ctrl Pts',(43.9555462062299,44.2289822161182,49.1482700154086));
#21008=CARTESIAN_POINT('Ctrl Pts',(44.0452292177111,44.2390689315626,49.0080414560762));
#21009=CARTESIAN_POINT('Ctrl Pts',(44.0643628533311,44.2413423243037,48.9761264469234));
#21010=CARTESIAN_POINT('Ctrl Pts',(44.1050799187064,44.2464903734566,48.9035287460759));
#21011=CARTESIAN_POINT('Ctrl Pts',(44.1261528171007,44.2493781097702,48.8625877646023));
#21012=CARTESIAN_POINT('Ctrl Pts',(44.1521891002928,44.253284623858,48.8072208933931));
#21013=CARTESIAN_POINT('Ctrl Pts',(44.1584760468713,44.2542575818108,48.7934319033404));
#21014=CARTESIAN_POINT('Ctrl Pts',(44.1684844117886,44.2558568639184,48.7707774337306));
#21015=CARTESIAN_POINT('Ctrl Pts',(44.1723032397453,44.2564798316299,48.7619555025706));
#21016=CARTESIAN_POINT('Ctrl Pts',(44.1795663281646,44.2576899213225,48.7448268922273));
#21017=CARTESIAN_POINT('Ctrl Pts',(44.1830187624535,44.258276745691,48.736523932966));
#21018=CARTESIAN_POINT('Ctrl Pts',(44.1909499317449,44.2596525986001,48.7170671943265));
#21019=CARTESIAN_POINT('Ctrl Pts',(44.1953826840854,44.2604431577854,48.7058951945795));
#21020=CARTESIAN_POINT('Ctrl Pts',(44.2094832602642,44.2630303332213,48.6693649098499));
#21021=CARTESIAN_POINT('Ctrl Pts',(44.218720071881,44.2648412161951,48.643844875651));
#21022=CARTESIAN_POINT('Ctrl Pts',(44.2393548408045,44.2691802610036,48.5828420036908));
#21023=CARTESIAN_POINT('Ctrl Pts',(44.2502686464073,44.2717231095403,48.5472080555882));
#21024=CARTESIAN_POINT('Ctrl Pts',(44.2890834621037,44.2818317589567,48.405992315646));
#21025=CARTESIAN_POINT('Ctrl Pts',(44.3090289062391,44.289613377377,48.2984457100565));
#21026=CARTESIAN_POINT('Ctrl Pts',(44.3296688283109,44.304599254482,48.0896821927224));
#21027=CARTESIAN_POINT('Ctrl Pts',(44.3317210339586,44.3117745488965,47.9889303963974));
#21028=CARTESIAN_POINT('Ctrl Pts',(44.324952285594,44.3197453285775,47.8720474256524));
#21029=CARTESIAN_POINT('Ctrl Pts',(44.3237911858304,44.3208560714008,47.855636982994));
#21030=CARTESIAN_POINT('Ctrl Pts',(44.3218825318956,44.3223874926704,47.8328122899058));
#21031=CARTESIAN_POINT('Ctrl Pts',(44.3213125314514,44.3228172770178,47.8263844585079));
#21032=CARTESIAN_POINT('Ctrl Pts',(44.3202739063996,44.3235554267425,47.8153041862278));
#21033=CARTESIAN_POINT('Ctrl Pts',(44.3198206050515,44.3238646276584,47.8106504163863));
#21034=CARTESIAN_POINT('Ctrl Pts',(44.3188292537852,44.3245144675831,47.8008425114936));
#21035=CARTESIAN_POINT('Ctrl Pts',(44.3182873484585,44.3248548770546,47.7956888151571));
#21036=CARTESIAN_POINT('Ctrl Pts',(44.3168928297472,44.3256957009547,47.7829213722241));
#21037=CARTESIAN_POINT('Ctrl Pts',(44.3160156040515,44.3261947505044,47.7753103000479));
#21038=CARTESIAN_POINT('Ctrl Pts',(44.3125488483363,44.3280611945961,47.7467296357037));
#21039=CARTESIAN_POINT('Ctrl Pts',(44.3096601119123,44.329412887069,47.7257969355128));
#21040=CARTESIAN_POINT('Ctrl Pts',(44.2843377234375,44.3398865984824,47.5621990192405));
#21041=CARTESIAN_POINT('Ctrl Pts',(44.2462890266302,44.3483231044245,47.4223959231744));
#21042=CARTESIAN_POINT('Ctrl Pts',(44.1524526307382,44.3635493628966,47.1860485052103));
#21043=CARTESIAN_POINT('Ctrl Pts',(44.1032821457636,44.3702176376007,47.0876226233518));
#21044=CARTESIAN_POINT('Ctrl Pts',(44.0371176264346,44.3782763389708,46.9793731511841));
#21045=CARTESIAN_POINT('Ctrl Pts',(44.0280330427057,44.379366057995,46.9649436394998));
#21046=CARTESIAN_POINT('Ctrl Pts',(44.0127690762492,44.3811710698602,46.9413972856629));
#21047=CARTESIAN_POINT('Ctrl Pts',(44.0067006515745,44.381882238631,46.9322093800622));
#21048=CARTESIAN_POINT('Ctrl Pts',(43.9956028970884,44.3831715900713,46.9157156221107));
#21049=CARTESIAN_POINT('Ctrl Pts',(43.9906011726788,44.383748718273,46.9083914976581));
#21050=CARTESIAN_POINT('Ctrl Pts',(43.979769747539,44.3849902108442,46.8927633311796));
#21051=CARTESIAN_POINT('Ctrl Pts',(43.9739247048349,44.3856551506623,46.8844702994348));
#21052=CARTESIAN_POINT('Ctrl Pts',(43.9577605398998,44.3874806757288,46.861916299017));
#21053=CARTESIAN_POINT('Ctrl Pts',(43.9473114243264,44.3886462588372,46.8477501437749));
#21054=CARTESIAN_POINT('Ctrl Pts',(43.8854058013768,44.3954708708344,46.7661837195868));
#21055=CARTESIAN_POINT('Ctrl Pts',(43.8297510505488,44.4012957498589,46.7021011777299));
#21056=CARTESIAN_POINT('Ctrl Pts',(43.6887826724702,44.415351384451,46.5598910765366));
#21057=CARTESIAN_POINT('Ctrl Pts',(43.6003000883232,44.423670631537,46.4853543489963));
#21058=CARTESIAN_POINT('Ctrl Pts',(43.4763390821255,44.4344002144715,46.3986505827933));
#21059=CARTESIAN_POINT('Ctrl Pts',(43.446417292435,44.4369248192642,46.378939588558));
#21060=CARTESIAN_POINT('Ctrl Pts',(43.3841735015363,44.442022002074,46.3403785128319));
#21061=CARTESIAN_POINT('Ctrl Pts',(43.351815786948,44.444590828384,46.3216114542265));
#21062=CARTESIAN_POINT('Ctrl Pts',(43.3103530828235,44.4477634934056,46.2991487463523));
#21063=CARTESIAN_POINT('Ctrl Pts',(43.3017403166854,44.448416204538,46.2945668780081));
#21064=CARTESIAN_POINT('Ctrl Pts',(43.288093890278,44.4494400083192,46.2874394589912));
#21065=CARTESIAN_POINT('Ctrl Pts',(43.2830833315075,44.4498137290852,46.2848503866386));
#21066=CARTESIAN_POINT('Ctrl Pts',(43.2735875603142,44.4505177538206,46.2799963439574));
#21067=CARTESIAN_POINT('Ctrl Pts',(43.2691048910654,44.4508483172728,46.2777269405711));
#21068=CARTESIAN_POINT('Ctrl Pts',(43.2585588003516,44.4516219113889,46.2724395194864));
#21069=CARTESIAN_POINT('Ctrl Pts',(43.2524882877063,44.45206404655,46.2694358867045));
#21070=CARTESIAN_POINT('Ctrl Pts',(43.2325139868229,44.4535089116539,46.259683398226));
#21071=CARTESIAN_POINT('Ctrl Pts',(43.2185444873535,44.4545037020621,46.2530694428768));
#21072=CARTESIAN_POINT('Ctrl Pts',(43.1403384798965,44.459994223197,46.2171864080761));
#21073=CARTESIAN_POINT('Ctrl Pts',(43.0746057385242,44.4643168939365,46.1912892287205));
#21074=CARTESIAN_POINT('Ctrl Pts',(42.9637164660441,44.4713639536715,46.1544909620969));
#21075=CARTESIAN_POINT('Ctrl Pts',(42.919328167095,44.47412240224,46.1415118242177));
#21076=CARTESIAN_POINT('Ctrl Pts',(42.743713150388,44.4849290864673,46.0969458894735));
#21077=CARTESIAN_POINT('Ctrl Pts',(42.6098052784933,44.4929709445296,46.0775718515764));
#21078=CARTESIAN_POINT('Ctrl Pts',(42.44969242427,44.5030745136266,46.0713440982121));
#21079=CARTESIAN_POINT('Ctrl Pts',(42.4243901517884,44.5046843019646,46.0708582348964));
#21080=CARTESIAN_POINT('Ctrl Pts',(42.3875208851583,44.507052428667,46.0708756926531));
#21081=CARTESIAN_POINT('Ctrl Pts',(42.3759557178011,44.5077984699511,46.0709851777651));
#21082=CARTESIAN_POINT('Ctrl Pts',(42.35544004121,44.5091278837904,46.0713639172474));
#21083=CARTESIAN_POINT('Ctrl Pts',(42.3464890329019,44.5097099339637,46.0715915107311));
#21084=CARTESIAN_POINT('Ctrl Pts',(42.3278255715669,44.5109279188057,46.0721960994265));
#21085=CARTESIAN_POINT('Ctrl Pts',(42.3181137561512,44.5115641859912,46.0725842004427));
#21086=CARTESIAN_POINT('Ctrl Pts',(42.2927783195184,44.5132306786596,46.073788478204));
#21087=CARTESIAN_POINT('Ctrl Pts',(42.2771612238085,44.5142645338645,46.0747213381197));
#21088=CARTESIAN_POINT('Ctrl Pts',(42.20587711682,44.5190148876253,46.0798502070654));
#21089=CARTESIAN_POINT('Ctrl Pts',(42.1504021385761,44.522800243875,46.0862709823012));
#21090=CARTESIAN_POINT('Ctrl Pts',(41.9888247749733,44.5340915716555,46.1121170755786));
#21091=CARTESIAN_POINT('Ctrl Pts',(41.8839873006605,44.5417702927968,46.1380405103852));
#21092=CARTESIAN_POINT('Ctrl Pts',(41.6848329192596,44.556789476346,46.2054043888763));
#21093=CARTESIAN_POINT('Ctrl Pts',(41.5905490290221,44.5641011349641,46.2459103208958));
#21094=CARTESIAN_POINT('Ctrl Pts',(41.4853714957469,44.5721968629705,46.3013923774642));
#21095=CARTESIAN_POINT('Ctrl Pts',(41.4709199992101,44.5733075912384,46.3092535516756));
#21096=CARTESIAN_POINT('Ctrl Pts',(41.4509416833998,44.5748389957339,46.3204546722301));
#21097=CARTESIAN_POINT('Ctrl Pts',(41.4453288843561,44.5752687776135,46.3236386844582));
#21098=CARTESIAN_POINT('Ctrl Pts',(41.4356767925214,44.5760069242515,46.3291782947736));
#21099=CARTESIAN_POINT('Ctrl Pts',(41.4316299366663,44.5763161245325,46.3315205003515));
#21100=CARTESIAN_POINT('Ctrl Pts',(41.4232059934553,44.5769590977154,46.3364370133502));
#21101=CARTESIAN_POINT('Ctrl Pts',(41.4188304862275,44.5772926886366,46.3390139290042));
#21102=CARTESIAN_POINT('Ctrl Pts',(41.4080943399973,44.57811041484,46.3453941134969));
#21103=CARTESIAN_POINT('Ctrl Pts',(41.4017452622689,44.5785933003072,46.3492168643332));
#21104=CARTESIAN_POINT('Ctrl Pts',(41.3880624276663,44.5796328068658,46.3575630463935));
#21105=CARTESIAN_POINT('Ctrl Pts',(41.3807365939153,44.5801886375716,46.3620992361198));
#21106=CARTESIAN_POINT('Ctrl Pts',(41.3600242338606,44.5817588096497,46.3751172072606));
#21107=CARTESIAN_POINT('Ctrl Pts',(41.3467111677523,44.5827664619391,46.3837152615999));
#21108=CARTESIAN_POINT('Ctrl Pts',(41.1990018193309,44.5939464344257,46.4817115180934));
#21109=CARTESIAN_POINT('Ctrl Pts',(41.0762131346019,44.6032845415953,46.5874849409357));
#21110=CARTESIAN_POINT('Ctrl Pts',(40.907236097218,44.6184783622448,46.7746720786511));
#21111=CARTESIAN_POINT('Ctrl Pts',(40.8512799600288,44.6240381896742,46.8462081153635));
#21112=CARTESIAN_POINT('Ctrl Pts',(40.7903682408413,44.6309625312971,46.9365335290933));
#21113=CARTESIAN_POINT('Ctrl Pts',(40.7803842250836,44.6321296057193,46.9518015264769));
#21114=CARTESIAN_POINT('Ctrl Pts',(40.7650546850809,44.6339742433446,46.975986143251));
#21115=CARTESIAN_POINT('Ctrl Pts',(40.7595619862318,44.6346463304575,46.9848085512758));
#21116=CARTESIAN_POINT('Ctrl Pts',(40.7499849206053,44.6358383244086,47.0004719768261));
#21117=CARTESIAN_POINT('Ctrl Pts',(40.745871114163,44.6363571323165,47.0072947783096));
#21118=CARTESIAN_POINT('Ctrl Pts',(40.7365191483165,44.6375524082843,47.0230246749955));
#21119=CARTESIAN_POINT('Ctrl Pts',(40.7313100928021,44.6382299178428,47.0319487017033));
#21120=CARTESIAN_POINT('Ctrl Pts',(40.7169888416897,44.6401260153166,47.0569425978092));
#21121=CARTESIAN_POINT('Ctrl Pts',(40.7080356097415,44.6413502667593,47.0731017939553));
#21122=CARTESIAN_POINT('Ctrl Pts',(40.6485241769207,44.6497623631535,47.1842468064908));
#21123=CARTESIAN_POINT('Ctrl Pts',(40.6057664372364,44.657224115982,47.2831738533788));
#21124=CARTESIAN_POINT('Ctrl Pts',(40.5280735476161,44.6744967608975,47.5142206047727));
#21125=CARTESIAN_POINT('Ctrl Pts',(40.4984575253915,44.6843669344272,47.6475406060921));
#21126=CARTESIAN_POINT('Ctrl Pts',(40.4797929190569,44.6958314494759,47.8123153779151));
#21127=CARTESIAN_POINT('Ctrl Pts',(40.4771361854944,44.6978557787251,47.8418363665111));
#21128=CARTESIAN_POINT('Ctrl Pts',(40.4745608733765,44.7004508831506,47.8803853438536));
#21129=CARTESIAN_POINT('Ctrl Pts',(40.4740239663874,44.7010520645172,47.8893662706633));
#21130=CARTESIAN_POINT('Ctrl Pts',(40.4732615496555,44.7020134619446,47.9038155566487));
#21131=CARTESIAN_POINT('Ctrl Pts',(40.4729964530498,44.7023758062247,47.9092815615021));
#21132=CARTESIAN_POINT('Ctrl Pts',(40.472544355564,44.7030507216995,47.9195019668547));
#21133=CARTESIAN_POINT('Ctrl Pts',(40.4723516813883,44.7033635983286,47.9242559915644));
#21134=CARTESIAN_POINT('Ctrl Pts',(40.4719917587624,44.7040047678499,47.9340302465868));
#21135=CARTESIAN_POINT('Ctrl Pts',(40.471826524601,44.7043329499244,47.9390505388711));
#21136=CARTESIAN_POINT('Ctrl Pts',(40.4714351338557,44.7052121787776,47.9525450201787));
#21137=CARTESIAN_POINT('Ctrl Pts',(40.4712452191392,44.7057612865506,47.9610202659963));
#21138=CARTESIAN_POINT('Ctrl Pts',(40.4709536582931,44.706949616164,47.9794572211443));
#21139=CARTESIAN_POINT('Ctrl Pts',(40.4708732945297,44.7075877611935,47.9894190445852));
#21140=CARTESIAN_POINT('Ctrl Pts',(40.4708700992302,44.7082223988407,47.9993812464564));
#21141=CARTESIAN_POINT('Ctrl Pts',(40.4708700998153,44.7082222827967,47.9993794248603));
#21142=CARTESIAN_POINT('Ctrl Pts',(40.470843159349,44.7135573880865,48.0831269933827));
#21143=CARTESIAN_POINT('Ctrl Pts',(40.476269768031,44.7186402214411,48.1668007065684));
#21144=CARTESIAN_POINT('Ctrl Pts',(40.4953914375786,44.7274943353322,48.3131877603739));
#21145=CARTESIAN_POINT('Ctrl Pts',(40.5068014281716,44.7312842329043,48.376058029797));
#21146=CARTESIAN_POINT('Ctrl Pts',(40.5434819363403,44.7409453478977,48.5333012428052));
#21147=CARTESIAN_POINT('Ctrl Pts',(40.5728348466523,44.7468497865584,48.6265253016374));
#21148=CARTESIAN_POINT('Ctrl Pts',(40.6197968579192,44.7547875813334,48.7438047007647));
#21149=CARTESIAN_POINT('Ctrl Pts',(40.6310757220145,44.7566114082301,48.7702437413479));
#21150=CARTESIAN_POINT('Ctrl Pts',(40.6480159447999,44.7592438900717,48.8076172154725));
#21151=CARTESIAN_POINT('Ctrl Pts',(40.6531981583057,44.76003617279,48.8187655407772));
#21152=CARTESIAN_POINT('Ctrl Pts',(40.662373983148,44.7614172562074,48.8380215095631));
#21153=CARTESIAN_POINT('Ctrl Pts',(40.666318710524,44.7620043475128,48.8461521179976));
#21154=CARTESIAN_POINT('Ctrl Pts',(40.6745331466187,44.7632136095346,48.8627845633017));
#21155=CARTESIAN_POINT('Ctrl Pts',(40.6788089047951,44.7638359798315,48.8712831187825));
#21156=CARTESIAN_POINT('Ctrl Pts',(40.6898478927262,44.7654252497102,48.8928259725496));
#21157=CARTESIAN_POINT('Ctrl Pts',(40.6966975125556,44.7663951765853,48.9058250731414));
#21158=CARTESIAN_POINT('Ctrl Pts',(40.7238531785901,44.7701798115556,48.9559633918994));
#21159=CARTESIAN_POINT('Ctrl Pts',(40.7452295745284,44.7730323046731,48.9925061891765));
#21160=CARTESIAN_POINT('Ctrl Pts',(40.8646202275298,44.7883415948761,49.1820112465663));
#21161=CARTESIAN_POINT('Ctrl Pts',(40.982670866585,44.8015449302295,49.3212488597038));
#21162=CARTESIAN_POINT('Ctrl Pts',(41.1456183604631,44.8168885332624,49.4660815434753));
#21163=CARTESIAN_POINT('Ctrl Pts',(41.1735149550632,44.8194267695809,49.4894976162129));
#21164=CARTESIAN_POINT('Ctrl Pts',(41.2140892001972,44.8229772335842,49.5216417714577));
#21165=CARTESIAN_POINT('Ctrl Pts',(41.2262328547696,44.8240225963962,49.5310286828503));
#21166=CARTESIAN_POINT('Ctrl Pts',(41.2452161736383,44.8256286127212,49.5453439387762));
#21167=CARTESIAN_POINT('Ctrl Pts',(41.2519780084274,44.8261952492517,49.5503738541882));
#21168=CARTESIAN_POINT('Ctrl Pts',(41.2645224556339,44.8272361706353,49.5595781996076));
#21169=CARTESIAN_POINT('Ctrl Pts',(41.2702956417047,44.8277112486902,49.5637651618043));
#21170=CARTESIAN_POINT('Ctrl Pts',(41.2802024523039,44.8285195347021,49.5708665080266));
#21171=CARTESIAN_POINT('Ctrl Pts',(41.2843245262642,44.8288538133343,49.5737968017262));
#21172=CARTESIAN_POINT('Ctrl Pts',(41.292279506086,44.8294949373911,49.579404863982));
#21173=CARTESIAN_POINT('Ctrl Pts',(41.2961106872475,44.8298019477392,49.5820849545345));
#21174=CARTESIAN_POINT('Ctrl Pts',(41.3052518239312,44.8305303895725,49.5884302363828));
#21175=CARTESIAN_POINT('Ctrl Pts',(41.3105705392294,44.8309509729924,49.5920827986583));
#21176=CARTESIAN_POINT('Ctrl Pts',(41.3295105755805,44.8324375477525,49.6049502790138));
#21177=CARTESIAN_POINT('Ctrl Pts',(41.343231743482,44.8334941975171,49.6140179371061));
#21178=CARTESIAN_POINT('Ctrl Pts',(41.4428992067248,44.841037386174,49.6780673625323));
#21179=CARTESIAN_POINT('Ctrl Pts',(41.5329829214778,44.8471604959084,49.7263368111641));
#21180=CARTESIAN_POINT('Ctrl Pts',(41.6813591843261,44.8568322662279,49.7912809908678));
#21181=CARTESIAN_POINT('Ctrl Pts',(41.7373092069277,44.8603918488044,49.812723502758));
#21182=CARTESIAN_POINT('Ctrl Pts',(41.7941389732838,44.8639880114013,49.8315225833187));
#21183=CARTESIAN_POINT('',(40.4708703960799,44.8789297818532,47.9987638045903));
#21184=CARTESIAN_POINT('Ctrl Pts',(41.7941386463292,45.0367815693785,49.8315224751633));
#21185=CARTESIAN_POINT('Ctrl Pts',(41.7423736161058,45.0334404792981,49.8143987806909));
#21186=CARTESIAN_POINT('Ctrl Pts',(41.6913362171882,45.0300469117126,49.7950810982887));
#21187=CARTESIAN_POINT('Ctrl Pts',(41.6255247393307,45.0254997752931,49.7669238847977));
#21188=CARTESIAN_POINT('Ctrl Pts',(41.6099743193676,45.0244125305486,49.7600259482308));
#21189=CARTESIAN_POINT('Ctrl Pts',(41.584524662545,45.0226108849182,49.7483316256625));
#21190=CARTESIAN_POINT('Ctrl Pts',(41.5745714042614,45.021900582945,49.7436545312493));
#21191=CARTESIAN_POINT('Ctrl Pts',(41.5566674567981,45.0206123168968,49.7350537105253));
#21192=CARTESIAN_POINT('Ctrl Pts',(41.5487027395109,45.0200354014174,49.7311597634824));
#21193=CARTESIAN_POINT('Ctrl Pts',(41.5406123916929,45.0194454123174,49.72713506268));
#21194=CARTESIAN_POINT('Ctrl Pts',(41.5404595371123,45.0194342639373,49.7270589968815));
#21195=CARTESIAN_POINT('Ctrl Pts',(41.5401928483905,45.0194148105832,49.7269262390483));
#21196=CARTESIAN_POINT('Ctrl Pts',(41.5400790096714,45.0194065059214,49.7268695560072));
#21197=CARTESIAN_POINT('Ctrl Pts',(41.5397866977003,45.0193851793683,49.7267239707617));
#21198=CARTESIAN_POINT('Ctrl Pts',(41.5396082326431,45.0193721569003,49.7266350521522));
#21199=CARTESIAN_POINT('Ctrl Pts',(41.5392621224038,45.0193468976411,49.7264625388534));
#21200=CARTESIAN_POINT('Ctrl Pts',(41.5390944755497,45.0193346609603,49.7263789473821));
#21201=CARTESIAN_POINT('Ctrl Pts',(41.5298426356076,45.0186592650582,49.721764145441));
#21202=CARTESIAN_POINT('Ctrl Pts',(41.5207944894213,45.0179936003734,49.7171614003344));
#21203=CARTESIAN_POINT('Ctrl Pts',(41.5021393074035,45.0166103008725,49.7074855077566));
#21204=CARTESIAN_POINT('Ctrl Pts',(41.4925379759166,45.0158923237027,49.7024021995704));
#21205=CARTESIAN_POINT('Ctrl Pts',(41.4682097558261,45.0140574616954,49.689257634042));
#21206=CARTESIAN_POINT('Ctrl Pts',(41.453544473358,45.0129366572529,49.6810848637387));
#21207=CARTESIAN_POINT('Ctrl Pts',(41.4113018213129,45.0096645778771,49.6568156234321));
#21208=CARTESIAN_POINT('Ctrl Pts',(41.3840161638718,45.0074961329812,49.6402252111127));
#21209=CARTESIAN_POINT('Ctrl Pts',(41.2869797716641,44.9995823233978,49.577874055057));
#21210=CARTESIAN_POINT('Ctrl Pts',(41.2198093055301,44.9937112261261,49.5282826336761));
#21211=CARTESIAN_POINT('Ctrl Pts',(41.0543020183072,44.9782968045226,49.3886559448686));
#21212=CARTESIAN_POINT('Ctrl Pts',(40.961695074283,44.968675125656,49.2924981652693));
#21213=CARTESIAN_POINT('Ctrl Pts',(40.8681808394641,44.9583011375594,49.17278486676));
#21214=CARTESIAN_POINT('Ctrl Pts',(40.8568513114721,44.9570319208137,49.1578369806458));
#21215=CARTESIAN_POINT('Ctrl Pts',(40.8412830214561,44.9552728724764,49.1366620335644));
#21216=CARTESIAN_POINT('Ctrl Pts',(40.8368603963706,44.954771410025,49.1305723249656));
#21217=CARTESIAN_POINT('Ctrl Pts',(40.8294993284876,44.9539340182063,49.1203107748375));
#21218=CARTESIAN_POINT('Ctrl Pts',(40.8265416266556,44.9535967919329,49.1161529200378));
#21219=CARTESIAN_POINT('Ctrl Pts',(40.8205269280826,44.9529095357372,49.1076262015717));
#21220=CARTESIAN_POINT('Ctrl Pts',(40.8174714929276,44.9525596108576,49.1032563225958));
#21221=CARTESIAN_POINT('Ctrl Pts',(40.8096688190126,44.951663775415,49.0919978381912));
#21222=CARTESIAN_POINT('Ctrl Pts',(40.8049481398534,44.9511196372045,49.0850908319305));
#21223=CARTESIAN_POINT('Ctrl Pts',(40.78530927915,44.9488458096467,49.0559513484828));
#21224=CARTESIAN_POINT('Ctrl Pts',(40.7708090234979,44.9471420299663,49.0334390691465));
#21225=CARTESIAN_POINT('Ctrl Pts',(40.7325473109733,44.9425550373151,48.9712280651652));
#21226=CARTESIAN_POINT('Ctrl Pts',(40.7097367402525,44.9397170417819,48.9309635449529));
#21227=CARTESIAN_POINT('Ctrl Pts',(40.6236849915747,44.9284124548377,48.7654571738873));
#21228=CARTESIAN_POINT('Ctrl Pts',(40.572743179318,44.9202308619044,48.6343137386726));
#21229=CARTESIAN_POINT('Ctrl Pts',(40.520525839078,44.9078969428999,48.4392296233924));
#21230=CARTESIAN_POINT('Ctrl Pts',(40.5074473200863,44.9040687749348,48.3789313774694));
#21231=CARTESIAN_POINT('Ctrl Pts',(40.494301056645,44.8990005486979,48.3003003637516));
#21232=CARTESIAN_POINT('Ctrl Pts',(40.4915731296504,44.8978448374018,48.2824457756304));
#21233=CARTESIAN_POINT('Ctrl Pts',(40.4876769970517,44.8960143892589,48.2543037785179));
#21234=CARTESIAN_POINT('Ctrl Pts',(40.4863401773526,44.8953449909518,48.2440404794934));
#21235=CARTESIAN_POINT('Ctrl Pts',(40.4841150665476,44.8941527027561,48.2258133805476));
#21236=CARTESIAN_POINT('Ctrl Pts',(40.4831936780118,44.8936308726527,48.217853808289));
#21237=CARTESIAN_POINT('Ctrl Pts',(40.4814094996555,44.8925596589843,48.2015524177631));
#21238=CARTESIAN_POINT('Ctrl Pts',(40.4805514656363,44.8920101369802,48.1932102618167));
#21239=CARTESIAN_POINT('Ctrl Pts',(40.4787714133191,44.890789076234,48.1747200752781));
#21240=CARTESIAN_POINT('Ctrl Pts',(40.4778753571803,44.8901167350987,48.1645698564228));
#21241=CARTESIAN_POINT('Ctrl Pts',(40.4753866197878,44.8880573703142,48.1335770792281));
#21242=CARTESIAN_POINT('Ctrl Pts',(40.4740522934086,44.8866623321658,48.1127158922622));
#21243=CARTESIAN_POINT('Ctrl Pts',(40.4715795845198,44.883169774431,48.0608334712548));
#21244=CARTESIAN_POINT('Ctrl Pts',(40.4708505080496,44.8810601831904,48.0297998266257));
#21245=CARTESIAN_POINT('Ctrl Pts',(40.4708703960799,44.8789297818532,47.9987638045903));
#21246=CARTESIAN_POINT('Ctrl Pts',(40.4708703945825,44.8789299424055,47.9987661435421));
#21247=CARTESIAN_POINT('Ctrl Pts',(40.4709724326017,44.867978938071,47.8392301113058));
#21248=CARTESIAN_POINT('Ctrl Pts',(40.49086526861,44.8564531196928,47.6803279747953));
#21249=CARTESIAN_POINT('Ctrl Pts',(40.5414990586299,44.8418592094896,47.4806989108018));
#21250=CARTESIAN_POINT('Ctrl Pts',(40.5545395419476,44.8385973656448,47.4361067117574));
#21251=CARTESIAN_POINT('Ctrl Pts',(40.5776381127016,44.8335470830323,47.3665488398514));
#21252=CARTESIAN_POINT('Ctrl Pts',(40.5866299052588,44.8317183841791,47.3412494416397));
#21253=CARTESIAN_POINT('Ctrl Pts',(40.5991158523297,44.8293558957583,47.3083144027753));
#21254=CARTESIAN_POINT('Ctrl Pts',(40.6021353196467,44.8287969673646,47.3005035552415));
#21255=CARTESIAN_POINT('Ctrl Pts',(40.6071611758204,44.8278868696172,47.287750074268));
#21256=CARTESIAN_POINT('Ctrl Pts',(40.6091373336753,44.8275339513328,47.2827957625002));
#21257=CARTESIAN_POINT('Ctrl Pts',(40.6130436461375,44.8268459665086,47.2731192882896));
#21258=CARTESIAN_POINT('Ctrl Pts',(40.6149720185738,44.8265108037601,47.2683964966507));
#21259=CARTESIAN_POINT('Ctrl Pts',(40.6193293622951,44.8257632488342,47.2578446840405));
#21260=CARTESIAN_POINT('Ctrl Pts',(40.6217682892586,44.8253514512753,47.2520197738926));
#21261=CARTESIAN_POINT('Ctrl Pts',(40.6303464607727,44.8239255053821,47.2318115647412));
#21262=CARTESIAN_POINT('Ctrl Pts',(40.6366321584293,44.8229197364394,47.2174905662762));
#21263=CARTESIAN_POINT('Ctrl Pts',(40.6948957382308,44.813926014354,47.0890143868371));
#21264=CARTESIAN_POINT('Ctrl Pts',(40.7577251613764,44.8064976170915,46.9800893579967));
#21265=CARTESIAN_POINT('Ctrl Pts',(40.8747699017995,44.7944934605443,46.8163790832072));
#21266=CARTESIAN_POINT('Ctrl Pts',(40.922436338929,44.7899663925866,46.7573857842215));
#21267=CARTESIAN_POINT('Ctrl Pts',(41.0022410071904,44.7827240258423,46.6697211024814));
#21268=CARTESIAN_POINT('Ctrl Pts',(41.0320777430282,44.7800811408751,46.6390589734195));
#21269=CARTESIAN_POINT('Ctrl Pts',(41.0777320774882,44.7761069848767,46.5951608436356));
#21270=CARTESIAN_POINT('Ctrl Pts',(41.09278325985,44.7748074163053,46.5811448773585));
#21271=CARTESIAN_POINT('Ctrl Pts',(41.1172707599401,44.7727077256139,46.559062025718));
#21272=CARTESIAN_POINT('Ctrl Pts',(41.1265661011602,44.7719139744075,46.5508407117222));
#21273=CARTESIAN_POINT('Ctrl Pts',(41.1444160274693,44.7703954528834,46.5353576055527));
#21274=CARTESIAN_POINT('Ctrl Pts',(41.1529559442039,44.7696713870429,46.5280796319701));
#21275=CARTESIAN_POINT('Ctrl Pts',(41.1617175441333,44.7689308296643,46.5207437141244));
#21276=CARTESIAN_POINT('Ctrl Pts',(41.1618763910715,44.7689174041986,46.5206107581764));
#21277=CARTESIAN_POINT('Ctrl Pts',(41.162106970917,44.7688979171034,46.5204178244549));
#21278=CARTESIAN_POINT('Ctrl Pts',(41.1621786868627,44.7688918562982,46.5203578262343));
#21279=CARTESIAN_POINT('Ctrl Pts',(41.162329086151,44.768879146191,46.5202320193915));
#21280=CARTESIAN_POINT('Ctrl Pts',(41.1624077703205,44.7688724968508,46.520166211881));
#21281=CARTESIAN_POINT('Ctrl Pts',(41.1625729614176,44.7688585374881,46.5200280766852));
#21282=CARTESIAN_POINT('Ctrl Pts',(41.1626594695308,44.7688512274045,46.5199557502314));
#21283=CARTESIAN_POINT('Ctrl Pts',(41.1628413039679,44.7688358625589,46.5198037518062));
#21284=CARTESIAN_POINT('Ctrl Pts',(41.1629366316815,44.7688278077278,46.5197240814297));
#21285=CARTESIAN_POINT('Ctrl Pts',(41.1631372704251,44.7688108550905,46.5195564300118));
#21286=CARTESIAN_POINT('Ctrl Pts',(41.1632425832294,44.7688019571948,46.5194684509292));
#21287=CARTESIAN_POINT('Ctrl Pts',(41.1698795621611,44.7682412188554,46.513925072767));
#21288=CARTESIAN_POINT('Ctrl Pts',(41.1764471568338,44.767687627967,46.5085130181536));
#21289=CARTESIAN_POINT('Ctrl Pts',(41.1907538015829,44.7664843441529,46.4968816552194));
#21290=CARTESIAN_POINT('Ctrl Pts',(41.1985054530697,44.7658340288824,46.4906783065771));
#21291=CARTESIAN_POINT('Ctrl Pts',(41.2193524546871,44.7640892629676,46.4742576209772));
#21292=CARTESIAN_POINT('Ctrl Pts',(41.232532213674,44.7629905295507,46.4641493002873));
#21293=CARTESIAN_POINT('Ctrl Pts',(41.2937017116993,44.7579095101366,46.4184771977336));
#21294=CARTESIAN_POINT('Ctrl Pts',(41.3431918427926,44.7538484104954,46.384987464447));
#21295=CARTESIAN_POINT('Ctrl Pts',(41.5173078070522,44.7397210808718,46.2785972171422));
#21296=CARTESIAN_POINT('Ctrl Pts',(41.6485130949886,44.7293007448234,46.2174086845285));
#21297=CARTESIAN_POINT('Ctrl Pts',(41.829756994872,44.7157477688924,46.156479905103));
#21298=CARTESIAN_POINT('Ctrl Pts',(41.8747585697353,44.7124517287111,46.1431571282205));
#21299=CARTESIAN_POINT('Ctrl Pts',(41.9463844072569,44.7073552214268,46.1247650644032));
#21300=CARTESIAN_POINT('Ctrl Pts',(41.972704982429,44.705513672462,46.1185929948208));
#21301=CARTESIAN_POINT('Ctrl Pts',(42.0073594651518,44.7031372922652,46.1112315029435));
#21302=CARTESIAN_POINT('Ctrl Pts',(42.0155822616169,44.7025769631413,46.1095407875614));
#21303=CARTESIAN_POINT('Ctrl Pts',(42.0290518657282,44.7016651673307,46.1068627793161));
#21304=CARTESIAN_POINT('Ctrl Pts',(42.034292092779,44.7013119395573,46.1058435167623));
#21305=CARTESIAN_POINT('Ctrl Pts',(42.0445449277631,44.7006238436473,46.1038933997009));
#21306=CARTESIAN_POINT('Ctrl Pts',(42.0495570874368,44.7002888760953,46.1029606451076));
#21307=CARTESIAN_POINT('Ctrl Pts',(42.0607741642925,44.699542267448,46.1009191385484));
#21308=CARTESIAN_POINT('Ctrl Pts',(42.0669809948305,44.699131216029,46.0998208950556));
#21309=CARTESIAN_POINT('Ctrl Pts',(42.0885391201781,44.6977103589045,46.0961152523012));
#21310=CARTESIAN_POINT('Ctrl Pts',(42.1039170009502,44.6967088542671,46.0936632230954));
#21311=CARTESIAN_POINT('Ctrl Pts',(42.245132941704,44.6876079878924,46.0728961948677));
#21312=CARTESIAN_POINT('Ctrl Pts',(42.3724823942881,44.6800844028492,46.0668768769691));
#21313=CARTESIAN_POINT('Ctrl Pts',(42.590101708618,44.6670852938379,46.0781175326622));
#21314=CARTESIAN_POINT('Ctrl Pts',(42.6802434599076,44.6616600025727,46.0891800762485));
#21315=CARTESIAN_POINT('Ctrl Pts',(42.8022201465067,44.6539949589518,46.1129682779991));
#21316=CARTESIAN_POINT('Ctrl Pts',(42.834998342928,44.6519032179486,46.1202537368055));
#21317=CARTESIAN_POINT('Ctrl Pts',(42.8918753760804,44.6482056126073,46.1344628457622));
#21318=CARTESIAN_POINT('Ctrl Pts',(42.9160607879954,44.6466115165172,46.1410079531934));
#21319=CARTESIAN_POINT('Ctrl Pts',(42.9512885878612,44.6442543345026,46.1512817915509));
#21320=CARTESIAN_POINT('Ctrl Pts',(42.9624362058356,44.6435031972122,46.1546426833999));
#21321=CARTESIAN_POINT('Ctrl Pts',(42.9820834559204,44.6421697809823,46.1607606895917));
#21322=CARTESIAN_POINT('Ctrl Pts',(42.9905957108091,44.6415888768626,46.1634763566809));
#21323=CARTESIAN_POINT('Ctrl Pts',(43.0083767254189,44.6403685924171,46.1692854421108));
#21324=CARTESIAN_POINT('Ctrl Pts',(43.0176414395447,44.6397288468269,46.1723903374381));
#21325=CARTESIAN_POINT('Ctrl Pts',(43.0419094953359,44.6380425636779,46.1807289252985));
#21326=CARTESIAN_POINT('Ctrl Pts',(43.0568721994432,44.6369922338485,46.1860777493972));
#21327=CARTESIAN_POINT('Ctrl Pts',(43.1210795103002,44.632437955839,46.2099289940278));
#21328=CARTESIAN_POINT('Ctrl Pts',(43.1696179032668,44.6288737845812,46.2302550332506));
#21329=CARTESIAN_POINT('Ctrl Pts',(43.340194777772,44.6159006237209,46.3100312165716));
#21330=CARTESIAN_POINT('Ctrl Pts',(43.456705972987,44.6061575130016,46.3803319823137));
#21331=CARTESIAN_POINT('Ctrl Pts',(43.6330693481546,44.5903969107667,46.5139297301077));
#21332=CARTESIAN_POINT('Ctrl Pts',(43.6977740300256,44.5843595749388,46.570087095085));
#21333=CARTESIAN_POINT('Ctrl Pts',(43.7666334402729,44.5778133642753,46.6383886392784));
#21334=CARTESIAN_POINT('Ctrl Pts',(43.774654288143,44.5770489016747,46.6464867709188));
#21335=CARTESIAN_POINT('Ctrl Pts',(43.7867813649554,44.5758907456385,46.6589497032574));
#21336=CARTESIAN_POINT('Ctrl Pts',(43.7909396458804,44.5754931970663,46.6632631685653));
#21337=CARTESIAN_POINT('Ctrl Pts',(43.7985124028554,44.5747685462889,46.6711921341488));
#21338=CARTESIAN_POINT('Ctrl Pts',(43.8019330077403,44.5744409830497,46.6748014759003));
#21339=CARTESIAN_POINT('Ctrl Pts',(43.8096167161664,44.573704605809,46.6829721917727));
#21340=CARTESIAN_POINT('Ctrl Pts',(43.813871656335,44.5732964123506,46.6875410573083));
#21341=CARTESIAN_POINT('Ctrl Pts',(43.8247971803144,44.572246948537,46.6993874492504));
#21342=CARTESIAN_POINT('Ctrl Pts',(43.8314343143005,44.5716081115383,46.706695772081));
#21343=CARTESIAN_POINT('Ctrl Pts',(43.8749240403026,44.5674109059882,46.7553283990281));
#21344=CARTESIAN_POINT('Ctrl Pts',(43.9100426959746,44.5639674134161,46.7981761250351));
#21345=CARTESIAN_POINT('Ctrl Pts',(44.0208473927045,44.5526879625133,46.9459072870236));
#21346=CARTESIAN_POINT('Ctrl Pts',(44.0878315025941,44.545132787662,47.0568744611161));
#21347=CARTESIAN_POINT('Ctrl Pts',(44.1802984631841,44.5320972491625,47.25195153617));
#21348=CARTESIAN_POINT('Ctrl Pts',(44.2120701610644,44.5267761860267,47.3325885493896));
#21349=CARTESIAN_POINT('Ctrl Pts',(44.2436797458177,44.5201433879846,47.431932817233));
#21350=CARTESIAN_POINT('Ctrl Pts',(44.2488098709077,44.5190109955122,47.4488581334481));
#21351=CARTESIAN_POINT('Ctrl Pts',(44.2565201293395,44.5172159666035,47.4756157603817));
#21352=CARTESIAN_POINT('Ctrl Pts',(44.2592565759015,44.5165584388225,47.4854022932371));
#21353=CARTESIAN_POINT('Ctrl Pts',(44.264235076308,44.5153225945993,47.5037654625107));
#21354=CARTESIAN_POINT('Ctrl Pts',(44.2664955895562,44.5147448961752,47.5123368522467));
#21355=CARTESIAN_POINT('Ctrl Pts',(44.2714239707434,44.5134472182802,47.5315606062156));
#21356=CARTESIAN_POINT('Ctrl Pts',(44.2740601004344,44.5127262323699,47.5422207132381));
#21357=CARTESIAN_POINT('Ctrl Pts',(44.2805352691786,44.5108842733074,47.5693989816944));
#21358=CARTESIAN_POINT('Ctrl Pts',(44.2842477076333,44.5097592803214,47.5859460415572));
#21359=CARTESIAN_POINT('Ctrl Pts',(44.3087666296874,44.5018152040406,47.7023988192331));
#21360=CARTESIAN_POINT('Ctrl Pts',(44.3218317882982,44.4947504316987,47.8037525765928));
#21361=CARTESIAN_POINT('Ctrl Pts',(44.3346266640926,44.47624343602,48.0650494290505));
#21362=CARTESIAN_POINT('Ctrl Pts',(44.3226228709961,44.4646164912893,48.2248010721459));
#21363=CARTESIAN_POINT('Ctrl Pts',(44.2879385884095,44.4526840284092,48.396841743561));
#21364=CARTESIAN_POINT('Ctrl Pts',(44.2846027761546,44.4516114426936,48.4123928946114));
#21365=CARTESIAN_POINT('Ctrl Pts',(44.279555525584,44.4500914339533,48.4345808366251));
#21366=CARTESIAN_POINT('Ctrl Pts',(44.2780005638145,44.4496357588842,48.4412520404267));
#21367=CARTESIAN_POINT('Ctrl Pts',(44.2752412150599,44.4488486907401,48.4528115336905));
#21368=CARTESIAN_POINT('Ctrl Pts',(44.2740531782585,44.4485163808613,48.4577036018745));
#21369=CARTESIAN_POINT('Ctrl Pts',(44.2715035002255,44.4478168916883,48.4680262258863));
#21370=CARTESIAN_POINT('Ctrl Pts',(44.270137360466,44.4474499721514,48.4734555464257));
#21371=CARTESIAN_POINT('Ctrl Pts',(44.2663715167304,44.4464593097702,48.4881511426683));
#21372=CARTESIAN_POINT('Ctrl Pts',(44.263926414207,44.4458381152197,48.4974057782156));
#21373=CARTESIAN_POINT('Ctrl Pts',(44.252132506195,44.4429405619229,48.540736818069));
#21374=CARTESIAN_POINT('Ctrl Pts',(44.2419168429715,44.4407097468855,48.5745727475855));
#21375=CARTESIAN_POINT('Ctrl Pts',(44.193164862755,44.4310957552315,48.7213451880885));
#21376=CARTESIAN_POINT('Ctrl Pts',(44.1451256246305,44.4240747086526,48.830855492058));
#21377=CARTESIAN_POINT('Ctrl Pts',(44.0323095037777,44.4101622090856,49.0343892116458));
#21378=CARTESIAN_POINT('Ctrl Pts',(43.9687221775344,44.4033061481595,49.1284951405384));
#21379=CARTESIAN_POINT('Ctrl Pts',(43.8840127041285,44.3947944864602,49.2327567923794));
#21380=CARTESIAN_POINT('Ctrl Pts',(43.8705141988492,44.393454759686,49.2488278307978));
#21381=CARTESIAN_POINT('Ctrl Pts',(43.8496400426422,44.3914058476817,49.2728724001446));
#21382=CARTESIAN_POINT('Ctrl Pts',(43.8424545416399,44.3907045097692,49.281009479908));
#21383=CARTESIAN_POINT('Ctrl Pts',(43.8292827701946,44.3894257482372,49.2956742481131));
#21384=CARTESIAN_POINT('Ctrl Pts',(43.8233194548827,44.388849301627,49.3022222234888));
#21385=CARTESIAN_POINT('Ctrl Pts',(43.8103529791841,44.3876010879183,49.3162645009454));
#21386=CARTESIAN_POINT('Ctrl Pts',(43.8033347412038,44.3869286848072,49.3237444464706));
#21387=CARTESIAN_POINT('Ctrl Pts',(43.784078419096,44.3850921848582,49.3439423338812));
#21388=CARTESIAN_POINT('Ctrl Pts',(43.7717251609623,44.38392310633,49.3565486037799));
#21389=CARTESIAN_POINT('Ctrl Pts',(43.7038721156012,44.3775483195533,49.4239167968687));
#21390=CARTESIAN_POINT('Ctrl Pts',(43.6452711664185,44.3722041151454,49.4754383911357));
#21391=CARTESIAN_POINT('Ctrl Pts',(43.4816054935064,44.3576977433641,49.6026217872984));
#21392=CARTESIAN_POINT('Ctrl Pts',(43.3717717206397,44.3483569994922,49.6715031069482));
#21393=CARTESIAN_POINT('Ctrl Pts',(43.1986480350866,44.3346946891759,49.7572089242787));
#21394=CARTESIAN_POINT('Ctrl Pts',(43.1400299648216,44.3302390817495,49.7826887915561));
#21395=CARTESIAN_POINT('Ctrl Pts',(43.0701284780476,44.3252027094052,49.8090293991536));
#21396=CARTESIAN_POINT('Ctrl Pts',(43.0599749813627,44.3244778422603,49.8127582799106));
#21397=CARTESIAN_POINT('Ctrl Pts',(43.0442646965057,44.3233671372757,49.8183783979983));
#21398=CARTESIAN_POINT('Ctrl Pts',(43.0387299356031,44.3229779013409,49.8203299341357));
#21399=CARTESIAN_POINT('Ctrl Pts',(43.0284804045336,44.322261025031,49.8238913774928));
#21400=CARTESIAN_POINT('Ctrl Pts',(43.0237683138959,44.3219329918874,49.8255082764228));
#21401=CARTESIAN_POINT('Ctrl Pts',(43.0129909110555,44.3211861907937,49.829159813866));
#21402=CARTESIAN_POINT('Ctrl Pts',(43.0069217026778,44.3207681239778,49.8311825499965));
#21403=CARTESIAN_POINT('Ctrl Pts',(42.9909732043189,44.3196757787265,49.8364098382488));
#21404=CARTESIAN_POINT('Ctrl Pts',(42.9810777472447,44.3190042761616,49.8395649174088));
#21405=CARTESIAN_POINT('Ctrl Pts',(42.9009088509373,44.3136108155313,49.8644146051119));
#21406=CARTESIAN_POINT('Ctrl Pts',(42.8294640369798,44.3090928128288,49.8821569444686));
#21407=CARTESIAN_POINT('Ctrl Pts',(42.6464502019643,44.2978433315819,49.9166375385295));
#21408=CARTESIAN_POINT('Ctrl Pts',(42.5341129617762,44.2912241062349,49.9277582219177));
#21409=CARTESIAN_POINT('Ctrl Pts',(42.3372064641162,44.2793209738718,49.9299473170228));
#21410=CARTESIAN_POINT('Ctrl Pts',(42.2530061754285,44.2741375029644,49.9253648643706));
#21411=CARTESIAN_POINT('Ctrl Pts',(42.1519353140055,44.2676596671101,49.9131950365065));
#21412=CARTESIAN_POINT('Ctrl Pts',(42.134519211903,44.2665343998929,49.9108561574548));
#21413=CARTESIAN_POINT('Ctrl Pts',(42.1071100756304,44.2647481254039,49.9067933334878));
#21414=CARTESIAN_POINT('Ctrl Pts',(42.0970942450684,44.2640921420708,49.9052279185289));
#21415=CARTESIAN_POINT('Ctrl Pts',(42.0783417785628,44.2628576602189,49.9021454122809));
#21416=CARTESIAN_POINT('Ctrl Pts',(42.0696023287689,44.2622797664983,49.9006468781169));
#21417=CARTESIAN_POINT('Ctrl Pts',(42.050029776578,44.2609796181628,49.8971517437394));
#21418=CARTESIAN_POINT('Ctrl Pts',(42.0392028921651,44.2602563399303,49.8951225117285));
#21419=CARTESIAN_POINT('Ctrl Pts',(42.0116430755937,44.2584045554499,49.8897123771522));
#21420=CARTESIAN_POINT('Ctrl Pts',(41.9949368460913,44.2572719552437,49.8862019452984));
#21421=CARTESIAN_POINT('Ctrl Pts',(41.9160554454613,44.2518749764341,49.8685305509943));
#21422=CARTESIAN_POINT('Ctrl Pts',(41.8546007877818,44.2475229709969,49.8515231493321));
#21423=CARTESIAN_POINT('Ctrl Pts',(41.7941385063105,44.2430936274184,49.8315224288456));
#21424=CARTESIAN_POINT('Origin',(42.4,48.4493818343519,48.));
#21425=CARTESIAN_POINT('',(41.7941388354972,43.276409063163,49.8315225377394));
#21426=CARTESIAN_POINT('',(41.7941388168303,43.4464579097838,49.8315225315644));
#21427=CARTESIAN_POINT('',(41.7941388317924,48.4493818343519,49.8315225365138));
#21428=CARTESIAN_POINT('Ctrl Pts',(41.7941388354972,43.2764090631631,49.8315225377394));
#21429=CARTESIAN_POINT('Ctrl Pts',(41.7975715031584,43.276665280169,49.8326580520362));
#21430=CARTESIAN_POINT('Ctrl Pts',(41.8010075428829,43.2769216588947,49.8337839754625));
#21431=CARTESIAN_POINT('Ctrl Pts',(41.9411257165846,43.2873726318826,49.8792620926758));
#21432=CARTESIAN_POINT('Ctrl Pts',(42.0823349862631,43.2977977663472,49.9082147047067));
#21433=CARTESIAN_POINT('Ctrl Pts',(42.2464553596324,43.3090798354582,49.9231254082622));
#21434=CARTESIAN_POINT('Ctrl Pts',(42.2674885771241,43.3105094144422,49.9246890932136));
#21435=CARTESIAN_POINT('Ctrl Pts',(42.2961871406248,43.3124340705385,49.9263499310011));
#21436=CARTESIAN_POINT('Ctrl Pts',(42.3038327654162,43.3129443168211,49.9267467488836));
#21437=CARTESIAN_POINT('Ctrl Pts',(42.316656105874,43.3137956853094,49.9273357760045));
#21438=CARTESIAN_POINT('Ctrl Pts',(42.3218325387782,43.3141381515784,49.9275526577141));
#21439=CARTESIAN_POINT('Ctrl Pts',(42.3316832862201,43.3147874879727,49.9279256353647));
#21440=CARTESIAN_POINT('Ctrl Pts',(42.3363573765215,43.3150945785567,49.9280855910779));
#21441=CARTESIAN_POINT('Ctrl Pts',(42.3474859909983,43.3158234209757,49.9284259197283));
#21442=CARTESIAN_POINT('Ctrl Pts',(42.3539409808172,43.3162443225578,49.9285908894053));
#21443=CARTESIAN_POINT('Ctrl Pts',(42.3768669786843,43.3177330343508,49.9290616376128));
#21444=CARTESIAN_POINT('Ctrl Pts',(42.393341487202,43.3187914684695,49.9291888570559));
#21445=CARTESIAN_POINT('Ctrl Pts',(42.5076464392224,43.3260690142513,49.9286072159227));
#21446=CARTESIAN_POINT('Ctrl Pts',(42.6053101363888,43.3319548300672,49.9206681557122));
#21447=CARTESIAN_POINT('Ctrl Pts',(42.8081114099056,43.3442245502955,49.8885281861765));
#21448=CARTESIAN_POINT('Ctrl Pts',(42.9126655714818,43.3505844924173,49.8628650763818));
#21449=CARTESIAN_POINT('Ctrl Pts',(43.0714281067766,43.3608467820581,49.8095107231967));
#21450=CARTESIAN_POINT('Ctrl Pts',(43.1273914950086,43.3645857997682,49.7877486620164));
#21451=CARTESIAN_POINT('Ctrl Pts',(43.1968771704807,43.369433303414,49.7569250218533));
#21452=CARTESIAN_POINT('Ctrl Pts',(43.2114267590251,43.3704599693332,49.7502529380138));
#21453=CARTESIAN_POINT('Ctrl Pts',(43.2347463648457,43.3721251730052,49.7392058740867));
#21454=CARTESIAN_POINT('Ctrl Pts',(43.2435692097062,43.3727597976222,49.7349436730388));
#21455=CARTESIAN_POINT('Ctrl Pts',(43.2603710078212,43.3739773655123,49.7266684823949));
#21456=CARTESIAN_POINT('Ctrl Pts',(43.2683553322433,43.3745598966194,49.7226669241696));
#21457=CARTESIAN_POINT('Ctrl Pts',(43.2864710827563,43.3758907466995,49.7134297855369));
#21458=CARTESIAN_POINT('Ctrl Pts',(43.2965843682175,43.3766402732126,49.708159556855));
#21459=CARTESIAN_POINT('Ctrl Pts',(43.3282057995978,43.3790049089169,49.6913228324035));
#21460=CARTESIAN_POINT('Ctrl Pts',(43.3495406807893,43.3806312659304,49.6794378023391));
#21461=CARTESIAN_POINT('Ctrl Pts',(43.5010307337941,43.3924088401268,49.591237764396));
#21462=CARTESIAN_POINT('Ctrl Pts',(43.6220386995323,43.4031117889145,49.5003035490512));
#21463=CARTESIAN_POINT('Ctrl Pts',(43.7510454448362,43.4158447357743,49.3773056551403));
#21464=CARTESIAN_POINT('Ctrl Pts',(43.7704886522386,43.4178028154307,49.3579600671733));
#21465=CARTESIAN_POINT('Ctrl Pts',(43.8459060223926,43.4255393036476,49.2796512083813));
#21466=CARTESIAN_POINT('Ctrl Pts',(43.8985483732908,43.4312627900929,49.2175825798966));
#21467=CARTESIAN_POINT('Ctrl Pts',(43.9538804706296,43.4375138174259,49.1432961389503));
#21468=CARTESIAN_POINT('Ctrl Pts',(43.9605595460669,43.4382726417457,49.1341624648564));
#21469=CARTESIAN_POINT('Ctrl Pts',(43.9706424125512,43.4394241240661,49.1201163645016));
#21470=CARTESIAN_POINT('Ctrl Pts',(43.9741042464648,43.4398205700947,49.1152461978355));
#21471=CARTESIAN_POINT('Ctrl Pts',(43.9804070353457,43.4405442674723,49.1062915130103));
#21472=CARTESIAN_POINT('Ctrl Pts',(43.9832548257231,43.4408719701686,49.1022120790014));
#21473=CARTESIAN_POINT('Ctrl Pts',(43.9896539119269,43.4416099848318,49.0929694708962));
#21474=CARTESIAN_POINT('Ctrl Pts',(43.9931958522108,43.4420196646912,49.0877999831043));
#21475=CARTESIAN_POINT('Ctrl Pts',(44.0022939659063,43.4430753428977,49.0743814581237));
#21476=CARTESIAN_POINT('Ctrl Pts',(44.0078117318297,43.4437188605155,49.0661064280149));
#21477=CARTESIAN_POINT('Ctrl Pts',(44.0445890219552,43.4480331072836,49.0100162853374));
#21478=CARTESIAN_POINT('Ctrl Pts',(44.073778560978,43.4515814793416,48.9608707693914));
#21479=CARTESIAN_POINT('Ctrl Pts',(44.1227695663135,43.4579136050964,48.8693589383856));
#21480=CARTESIAN_POINT('Ctrl Pts',(44.1432939914581,43.460716116266,48.8274335797468));
#21481=CARTESIAN_POINT('Ctrl Pts',(44.1944880052587,43.4682400723816,48.7124773144469));
#21482=CARTESIAN_POINT('Ctrl Pts',(44.2222138335924,43.4729334213454,48.6382379025086));
#21483=CARTESIAN_POINT('Ctrl Pts',(44.2694315330769,43.4827055493593,48.4833402694934));
#21484=CARTESIAN_POINT('Ctrl Pts',(44.2884417178294,43.4877827075432,48.4027127371394));
#21485=CARTESIAN_POINT('Ctrl Pts',(44.3056706737414,43.4943425595646,48.3006536923249));
#21486=CARTESIAN_POINT('Ctrl Pts',(44.3087950133277,43.4956677845776,48.2801337236734));
#21487=CARTESIAN_POINT('Ctrl Pts',(44.3130421231307,43.4976991307694,48.2488558941182));
#21488=CARTESIAN_POINT('Ctrl Pts',(44.3144065851741,43.4983976145959,48.2381319795386));
#21489=CARTESIAN_POINT('Ctrl Pts',(44.3167248023132,43.4996735525186,48.2186024455147));
#21490=CARTESIAN_POINT('Ctrl Pts',(44.3177081907035,43.5002500535302,48.2098005907817));
#21491=CARTESIAN_POINT('Ctrl Pts',(44.3197039522671,43.5015011173647,48.190749473044));
#21492=CARTESIAN_POINT('Ctrl Pts',(44.3206949225203,43.5021763371244,48.1804982920261));
#21493=CARTESIAN_POINT('Ctrl Pts',(44.3231769383866,43.504027484259,48.1524822227429));
#21494=CARTESIAN_POINT('Ctrl Pts',(44.3245038607183,43.5052085244415,48.1347041878618));
#21495=CARTESIAN_POINT('Ctrl Pts',(44.3305079942351,43.5118153346209,48.0358128695151));
#21496=CARTESIAN_POINT('Ctrl Pts',(44.3303030574671,43.5173921330822,47.9544959544679));
#21497=CARTESIAN_POINT('Ctrl Pts',(44.3166421118602,43.531990720408,47.7467081781516));
#21498=CARTESIAN_POINT('Ctrl Pts',(44.2958141403414,43.5411643913227,47.6211082510863));
#21499=CARTESIAN_POINT('Ctrl Pts',(44.246511159677,43.554569705622,47.4379818211263));
#21500=CARTESIAN_POINT('Ctrl Pts',(44.2272838235973,43.558937474795,47.3783059990936));
#21501=CARTESIAN_POINT('Ctrl Pts',(44.2013845006594,43.5638884526781,47.3095852724974));
#21502=CARTESIAN_POINT('Ctrl Pts',(44.1975007585216,43.5646103904829,47.2995361169574));
#21503=CARTESIAN_POINT('Ctrl Pts',(44.1913745711189,43.5657176461611,47.2840711990845));
#21504=CARTESIAN_POINT('Ctrl Pts',(44.1891913623335,43.5661063288004,47.2786324284739));
#21505=CARTESIAN_POINT('Ctrl Pts',(44.1851054964215,43.5668228148672,47.2685864590024));
#21506=CARTESIAN_POINT('Ctrl Pts',(44.1832097740388,43.5671510057109,47.2639766960238));
#21507=CARTESIAN_POINT('Ctrl Pts',(44.1788341179247,43.567898976042,47.2534527054526));
#21508=CARTESIAN_POINT('Ctrl Pts',(44.1763425445749,43.5683180468312,47.2475434568451));
#21509=CARTESIAN_POINT('Ctrl Pts',(44.1697193537832,43.5694145677293,47.2320515254324));
#21510=CARTESIAN_POINT('Ctrl Pts',(44.165539305244,43.5700892085273,47.2224895987797));
#21511=CARTESIAN_POINT('Ctrl Pts',(44.1301719690914,43.5756592964805,47.1433424305889));
#21512=CARTESIAN_POINT('Ctrl Pts',(44.0949576401499,43.5803353358937,47.0756198223535));
#21513=CARTESIAN_POINT('Ctrl Pts',(43.9875507532231,43.5929630077305,46.8959490133234));
#21514=CARTESIAN_POINT('Ctrl Pts',(43.9076500297772,43.6007492419639,46.7891169228497));
#21515=CARTESIAN_POINT('Ctrl Pts',(43.7743141058009,43.612765729854,46.6447009128769));
#21516=CARTESIAN_POINT('Ctrl Pts',(43.728964592965,43.6167144621358,46.6002047598228));
#21517=CARTESIAN_POINT('Ctrl Pts',(43.6693359420291,43.6217996257477,46.5472116584798));
#21518=CARTESIAN_POINT('Ctrl Pts',(43.6570285595474,43.6228437416178,46.5365496683462));
#21519=CARTESIAN_POINT('Ctrl Pts',(43.6370552901654,43.624530388685,46.5196845054426));
#21520=CARTESIAN_POINT('Ctrl Pts',(43.6294740703362,43.6251688187024,46.5133819391931));
#21521=CARTESIAN_POINT('Ctrl Pts',(43.6149453274925,43.6263891603908,46.5014907731391));
#21522=CARTESIAN_POINT('Ctrl Pts',(43.6080066993058,43.6269706243822,46.4958916722165));
#21523=CARTESIAN_POINT('Ctrl Pts',(43.5920470790329,43.6283051425013,46.4831947812085));
#21524=CARTESIAN_POINT('Ctrl Pts',(43.5830011229461,43.6290594519708,46.476129059341));
#21525=CARTESIAN_POINT('Ctrl Pts',(43.5547221313414,43.6314114199397,46.4544441207616));
#21526=CARTESIAN_POINT('Ctrl Pts',(43.5352777860506,43.6330199771991,46.4401056335424));
#21527=CARTESIAN_POINT('Ctrl Pts',(43.3901208153211,43.6449707105291,46.3372169280715));
#21528=CARTESIAN_POINT('Ctrl Pts',(43.2545127101431,43.6558890937721,46.2636311230716));
#21529=CARTESIAN_POINT('Ctrl Pts',(43.0430540585999,43.6721392356012,46.1797061094291));
#21530=CARTESIAN_POINT('Ctrl Pts',(42.9729532240893,43.6773992446181,46.1564397796033));
#21531=CARTESIAN_POINT('Ctrl Pts',(42.8783742674408,43.6842070487545,46.1309672092805));
#21532=CARTESIAN_POINT('Ctrl Pts',(42.8549435506806,43.6858704171769,46.1251261397517));
#21533=CARTESIAN_POINT('Ctrl Pts',(42.8150663185979,43.6886555811409,46.1159767449595));
#21534=CARTESIAN_POINT('Ctrl Pts',(42.7986755027144,43.6897874034543,46.1124403148853));
#21535=CARTESIAN_POINT('Ctrl Pts',(42.7753813670654,43.6913756209772,46.1077314278336));
#21536=CARTESIAN_POINT('Ctrl Pts',(42.7685151143263,43.6918412816118,46.1063822629051));
#21537=CARTESIAN_POINT('Ctrl Pts',(42.75667298781,43.6926399413582,46.1041222290622));
#21538=CARTESIAN_POINT('Ctrl Pts',(42.751700636494,43.6929739341083,46.1031935240198));
#21539=CARTESIAN_POINT('Ctrl Pts',(42.7412807160417,43.6936709459347,46.1012897392622));
#21540=CARTESIAN_POINT('Ctrl Pts',(42.735832553949,43.6940337471013,46.1003185322283));
#21541=CARTESIAN_POINT('Ctrl Pts',(42.7212422164955,43.6950011411089,46.097782341282));
#21542=CARTESIAN_POINT('Ctrl Pts',(42.7120926693597,43.6956033871048,46.0962597979347));
#21543=CARTESIAN_POINT('Ctrl Pts',(42.6712269806596,43.698275088917,46.0897620248764));
#21544=CARTESIAN_POINT('Ctrl Pts',(42.6393985648793,43.7003072126593,46.0855126511284));
#21545=CARTESIAN_POINT('Ctrl Pts',(42.4666167549632,43.7111477721222,46.0668216580508));
#21546=CARTESIAN_POINT('Ctrl Pts',(42.32449354293,43.7194068259032,46.0671463247065));
#21547=CARTESIAN_POINT('Ctrl Pts',(42.0934278812835,43.7333759436952,46.0932214078828));
#21548=CARTESIAN_POINT('Ctrl Pts',(42.0040214398104,43.7389123784923,46.1097647864302));
#21549=CARTESIAN_POINT('Ctrl Pts',(41.8933814627704,43.7461334256677,46.1384329404577));
#21550=CARTESIAN_POINT('Ctrl Pts',(41.8707543316497,43.7476297257804,46.1447390465631));
#21551=CARTESIAN_POINT('Ctrl Pts',(41.8373717383794,43.7498689715142,46.1547030468463));
#21552=CARTESIAN_POINT('Ctrl Pts',(41.8265238041166,43.7506016445557,46.1580454810828));
#21553=CARTESIAN_POINT('Ctrl Pts',(41.8072231524517,43.7519144733605,46.1641793671379));
#21554=CARTESIAN_POINT('Ctrl Pts',(41.7987590002781,43.7524934031783,46.1669339775062));
#21555=CARTESIAN_POINT('Ctrl Pts',(41.7808943672514,43.7537222309119,46.1728849639977));
#21556=CARTESIAN_POINT('Ctrl Pts',(41.7714989212474,43.7543725844009,46.1760955268901));
#21557=CARTESIAN_POINT('Ctrl Pts',(41.7464588137315,43.7561170165039,46.1848685542025));
#21558=CARTESIAN_POINT('Ctrl Pts',(41.7308607701812,43.7572153730897,46.1905606091011));
#21559=CARTESIAN_POINT('Ctrl Pts',(41.6600562232286,43.7622561306587,46.2174393917042));
#21560=CARTESIAN_POINT('Ctrl Pts',(41.605773630995,43.7662756351905,46.2409541444119));
#21561=CARTESIAN_POINT('Ctrl Pts',(41.4063900519842,43.7816363555379,46.3384370620226));
#21562=CARTESIAN_POINT('Ctrl Pts',(41.2697669650518,43.7934630219118,46.4281812999105));
#21563=CARTESIAN_POINT('Ctrl Pts',(41.119281008156,43.8073865329362,46.5568979715536));
#21564=CARTESIAN_POINT('Ctrl Pts',(41.0931300570314,43.8098408413477,46.5805367731922));
#21565=CARTESIAN_POINT('Ctrl Pts',(41.0516260388392,43.8137748127579,46.620173721828));
#21566=CARTESIAN_POINT('Ctrl Pts',(41.0358757247195,43.8152773185176,46.6357427067194));
#21567=CARTESIAN_POINT('Ctrl Pts',(41.0149444024027,43.8172830071215,46.6571580946363));
#21568=CARTESIAN_POINT('Ctrl Pts',(41.0095263875965,43.8178030069971,46.6627690814153));
#21569=CARTESIAN_POINT('Ctrl Pts',(41.0005457322842,43.8186660962003,46.6721831975122));
#21570=CARTESIAN_POINT('Ctrl Pts',(40.9969642539146,43.8190106079839,46.6759681251936));
#21571=CARTESIAN_POINT('Ctrl Pts',(40.9902148208032,43.8196603669834,46.6831591056424));
#21572=CARTESIAN_POINT('Ctrl Pts',(40.9870437832673,43.8199658576736,46.6865621738041));
#21573=CARTESIAN_POINT('Ctrl Pts',(40.9795686500598,43.8206866123096,46.6946426775067));
#21574=CARTESIAN_POINT('Ctrl Pts',(40.9752752694262,43.8211010701009,46.6993300171964));
#21575=CARTESIAN_POINT('Ctrl Pts',(40.9603405142738,43.8225448662081,46.7157978603576));
#21576=CARTESIAN_POINT('Ctrl Pts',(40.9498211094351,43.8235655489159,46.7276887979375));
#21577=CARTESIAN_POINT('Ctrl Pts',(40.8599396168127,43.8323334603467,46.8318523969784));
#21578=CARTESIAN_POINT('Ctrl Pts',(40.7893164547205,43.8395559995996,46.9313271379131));
#21579=CARTESIAN_POINT('Ctrl Pts',(40.6814586929775,43.8524401583583,47.1184969720259));
#21580=CARTESIAN_POINT('Ctrl Pts',(40.6404386083731,43.8580679703413,47.2035241520015));
#21581=CARTESIAN_POINT('Ctrl Pts',(40.5868032419785,43.8670638828887,47.3392931371805));
#21582=CARTESIAN_POINT('Ctrl Pts',(40.5697481469518,43.8702994585477,47.3881229960178));
#21583=CARTESIAN_POINT('Ctrl Pts',(40.5502276297423,43.8745739027082,47.452170175346));
#21584=CARTESIAN_POINT('Ctrl Pts',(40.5459529064536,43.8755533413091,47.4668164558257));
#21585=CARTESIAN_POINT('Ctrl Pts',(40.5392627949576,43.8771605686069,47.4907923315399));
#21586=CARTESIAN_POINT('Ctrl Pts',(40.5367427427505,43.8777849354326,47.5000922249669));
#21587=CARTESIAN_POINT('Ctrl Pts',(40.5320079699338,43.8789958283477,47.5180985226308));
#21588=CARTESIAN_POINT('Ctrl Pts',(40.5297841856181,43.8795820425237,47.5268023020959));
#21589=CARTESIAN_POINT('Ctrl Pts',(40.5247905371157,43.8809400616988,47.5469323931288));
#21590=CARTESIAN_POINT('Ctrl Pts',(40.5220642015217,43.881713249832,47.5583690313814));
#21591=CARTESIAN_POINT('Ctrl Pts',(40.5137854507118,43.8841656192465,47.5945608943863));
#21592=CARTESIAN_POINT('Ctrl Pts',(40.5086169290759,43.8858569821936,47.6194002513415));
#21593=CARTESIAN_POINT('Ctrl Pts',(40.48182717801,43.8956329924862,47.7622164937813));
#21594=CARTESIAN_POINT('Ctrl Pts',(40.4707597676826,43.904048456566,47.8818850716964));
#21595=CARTESIAN_POINT('Ctrl Pts',(40.4709920943087,43.9219279601681,48.1327081996855));
#21596=CARTESIAN_POINT('Ctrl Pts',(40.4844403931585,43.9313714468035,48.2632860319756));
#21597=CARTESIAN_POINT('Ctrl Pts',(40.5142033584017,43.9413399992729,48.4068913570787));
#21598=CARTESIAN_POINT('Ctrl Pts',(40.5175808668798,43.9423997147379,48.4222413956722));
#21599=CARTESIAN_POINT('Ctrl Pts',(40.5225389177756,43.9438597933432,48.443531478295));
#21600=CARTESIAN_POINT('Ctrl Pts',(40.5239607021994,43.9442685483249,48.4495073338339));
#21601=CARTESIAN_POINT('Ctrl Pts',(40.5266052257117,43.9450109428346,48.4603913107921));
#21602=CARTESIAN_POINT('Ctrl Pts',(40.5278187706747,43.94534509744,48.4653016078481));
#21603=CARTESIAN_POINT('Ctrl Pts',(40.5303699830078,43.9460342273896,48.475452848679));
#21604=CARTESIAN_POINT('Ctrl Pts',(40.5317103964827,43.9463890431988,48.4806930111191));
#21605=CARTESIAN_POINT('Ctrl Pts',(40.5352666837976,43.9473119554533,48.4943562195065));
#21606=CARTESIAN_POINT('Ctrl Pts',(40.5375176211088,43.9478780697811,48.5027701340294));
#21607=CARTESIAN_POINT('Ctrl Pts',(40.5477724777889,43.9503802395638,48.5400881904193));
#21608=CARTESIAN_POINT('Ctrl Pts',(40.5563932912281,43.9522834667221,48.5688203482902));
#21609=CARTESIAN_POINT('Ctrl Pts',(40.5826649485588,43.9575918865548,48.6494954479266));
#21610=CARTESIAN_POINT('Ctrl Pts',(40.6018665558886,43.9609326955394,48.7009051404092));
#21611=CARTESIAN_POINT('Ctrl Pts',(40.6396821521477,43.9667802799114,48.7903205942545));
#21612=CARTESIAN_POINT('Ctrl Pts',(40.6574025647953,43.969300264196,48.8286614973622));
#21613=CARTESIAN_POINT('Ctrl Pts',(40.7373939556336,43.9799241627006,48.9877996358042));
#21614=CARTESIAN_POINT('Ctrl Pts',(40.811069001086,43.9880180878657,49.1024063658033));
#21615=CARTESIAN_POINT('Ctrl Pts',(40.9119972172458,43.9981789058822,49.2280183104509));
#21616=CARTESIAN_POINT('Ctrl Pts',(40.9282116708058,43.9997866312463,49.2474054158674));
#21617=CARTESIAN_POINT('Ctrl Pts',(40.9523906063301,44.0021522802368,49.2751875261074));
#21618=CARTESIAN_POINT('Ctrl Pts',(40.9600575903462,44.0028979438915,49.2838387868735));
#21619=CARTESIAN_POINT('Ctrl Pts',(40.9737998162352,44.0042269242847,49.2990672614106));
#21620=CARTESIAN_POINT('Ctrl Pts',(40.9798440171197,44.004808921621,49.3056721233109));
#21621=CARTESIAN_POINT('Ctrl Pts',(40.9925472469137,44.0060270394181,49.3193611443136));
#21622=CARTESIAN_POINT('Ctrl Pts',(40.9992142781201,44.0066634940976,49.3264374982621));
#21623=CARTESIAN_POINT('Ctrl Pts',(41.0167572925841,44.0083310244023,49.3447777986177));
#21624=CARTESIAN_POINT('Ctrl Pts',(41.0277172412236,44.0093657381083,49.3559600733581));
#21625=CARTESIAN_POINT('Ctrl Pts',(41.0784704061255,44.0141264708654,49.4064971859246));
#21626=CARTESIAN_POINT('Ctrl Pts',(41.1198248272775,44.017921718802,49.4442386385832));
#21627=CARTESIAN_POINT('Ctrl Pts',(41.2458654885061,44.0292586188345,49.5495964244485));
#21628=CARTESIAN_POINT('Ctrl Pts',(41.3346683030235,44.0369748263556,49.6119364515818));
#21629=CARTESIAN_POINT('Ctrl Pts',(41.5160905809453,44.0519778066981,49.7177290844786));
#21630=CARTESIAN_POINT('Ctrl Pts',(41.6078838972144,44.059235648291,49.7619435905247));
#21631=CARTESIAN_POINT('Ctrl Pts',(41.7181180814542,44.0672850269316,49.8046748981993));
#21632=CARTESIAN_POINT('Ctrl Pts',(41.7335686520541,44.0683984323564,49.8104374449469));
#21633=CARTESIAN_POINT('Ctrl Pts',(41.7551725661135,44.0699329204703,49.8181809214312));
#21634=CARTESIAN_POINT('Ctrl Pts',(41.761264320146,44.0703631547713,49.8203299197638));
#21635=CARTESIAN_POINT('Ctrl Pts',(41.7717856096138,44.0711018678385,49.8239822133983));
#21636=CARTESIAN_POINT('Ctrl Pts',(41.7762099821123,44.0714111850153,49.825500054735));
#21637=CARTESIAN_POINT('Ctrl Pts',(41.7851339228988,44.0720323508474,49.8285253023926));
#21638=CARTESIAN_POINT('Ctrl Pts',(41.7896335991051,44.0723441634992,49.8300322214975));
#21639=CARTESIAN_POINT('Ctrl Pts',(41.7941388317924,44.0726550104672,49.8315225365139));
#21640=CARTESIAN_POINT('Ctrl Pts',(41.7941385063105,44.2430936274184,49.8315224288456));
#21641=CARTESIAN_POINT('Ctrl Pts',(41.7396043809166,44.2390985684784,49.8134827225619));
#21642=CARTESIAN_POINT('Ctrl Pts',(41.6858775400372,44.2350409321712,49.7930079174364));
#21643=CARTESIAN_POINT('Ctrl Pts',(41.5524897688099,44.2246986259723,49.7352205757266));
#21644=CARTESIAN_POINT('Ctrl Pts',(41.4743401861913,44.2183834409544,49.6948209815617));
#21645=CARTESIAN_POINT('Ctrl Pts',(41.3476670832953,44.2079215730936,49.6179535927229));
#21646=CARTESIAN_POINT('Ctrl Pts',(41.29760689443,44.2037234975787,49.5842693549995));
#21647=CARTESIAN_POINT('Ctrl Pts',(41.2406316978823,44.1989385276753,49.5419214419756));
#21648=CARTESIAN_POINT('Ctrl Pts',(41.2321138654314,44.1982230057054,49.53547991934));
#21649=CARTESIAN_POINT('Ctrl Pts',(41.2190217033042,44.1971235299003,49.5254071314635));
#21650=CARTESIAN_POINT('Ctrl Pts',(41.2144097947295,44.1967362822372,49.5218253912312));
#21651=CARTESIAN_POINT('Ctrl Pts',(41.2058908338311,44.1960211926425,49.5151470911945));
#21652=CARTESIAN_POINT('Ctrl Pts',(41.2019795332078,44.1956929745052,49.5120563384701));
#21653=CARTESIAN_POINT('Ctrl Pts',(41.1930443539432,44.1949433550565,49.5049392257877));
#21654=CARTESIAN_POINT('Ctrl Pts',(41.1880286149247,44.1945226760866,49.5009028514761));
#21655=CARTESIAN_POINT('Ctrl Pts',(41.1748679765853,44.1934188970424,49.490202945857));
#21656=CARTESIAN_POINT('Ctrl Pts',(41.1667571001944,44.1927386677006,49.4834976429441));
#21657=CARTESIAN_POINT('Ctrl Pts',(41.0955846346437,44.1867657717694,49.4236718643789));
#21658=CARTESIAN_POINT('Ctrl Pts',(41.0359257461182,44.1817300279545,49.3666184424669));
#21659=CARTESIAN_POINT('Ctrl Pts',(40.9649099835989,44.175418843928,49.2894038944256));
#21660=CARTESIAN_POINT('Ctrl Pts',(40.9500136096402,44.1740754465618,49.272629266521));
#21661=CARTESIAN_POINT('Ctrl Pts',(40.8821675541652,44.167845645648,49.1934905513447));
#21662=CARTESIAN_POINT('Ctrl Pts',(40.8329271506569,44.1629955559193,49.1280591072135));
#21663=CARTESIAN_POINT('Ctrl Pts',(40.742098263753,44.1529974307122,48.9898908856949));
#21664=CARTESIAN_POINT('Ctrl Pts',(40.7007948009494,44.1478552448536,48.9171811423939));
#21665=CARTESIAN_POINT('Ctrl Pts',(40.6566815879319,44.1414239047763,48.8262511841174));
#21666=CARTESIAN_POINT('Ctrl Pts',(40.6492427093973,44.140300843664,48.8103696575544));
#21667=CARTESIAN_POINT('Ctrl Pts',(40.637850242419,44.1385172799369,48.7851582022315));
#21668=CARTESIAN_POINT('Ctrl Pts',(40.633751751813,44.1378617751561,48.7758945095482));
#21669=CARTESIAN_POINT('Ctrl Pts',(40.6262025635197,44.1366277126542,48.7584615019133));
#21670=CARTESIAN_POINT('Ctrl Pts',(40.6227348563843,44.1360497556231,48.750299807015));
#21671=CARTESIAN_POINT('Ctrl Pts',(40.6150819524767,44.1347488282835,48.7319369486293));
#21672=CARTESIAN_POINT('Ctrl Pts',(40.6109277242812,44.1340248289547,48.7217232965608));
#21673=CARTESIAN_POINT('Ctrl Pts',(40.6005524540698,44.1321699507473,48.6955743749994));
#21674=CARTESIAN_POINT('Ctrl Pts',(40.5944555058039,44.131034954445,48.6795912219813));
#21675=CARTESIAN_POINT('Ctrl Pts',(40.5482043034027,44.122056771913,48.553325976131));
#21676=CARTESIAN_POINT('Ctrl Pts',(40.5179846001232,44.1138830551309,48.4396885679311));
#21677=CARTESIAN_POINT('Ctrl Pts',(40.4799840558294,44.0978022847672,48.2166639866494));
#21678=CARTESIAN_POINT('Ctrl Pts',(40.4708152443879,44.0899511801632,48.107941920363));
#21679=CARTESIAN_POINT('Ctrl Pts',(40.470892390324,44.0792642431648,47.955174391841));
#21680=CARTESIAN_POINT('Ctrl Pts',(40.4724097294795,44.0762390376702,47.9113324877965));
#21681=CARTESIAN_POINT('Ctrl Pts',(40.4761166126907,44.072602088951,47.8574582923058));
#21682=CARTESIAN_POINT('Ctrl Pts',(40.4768926373583,44.0719228833635,47.8473451304902));
#21683=CARTESIAN_POINT('Ctrl Pts',(40.4782363620645,44.0708630782726,47.8314754460039));
#21684=CARTESIAN_POINT('Ctrl Pts',(40.4787502369596,44.070479613273,47.825714729279));
#21685=CARTESIAN_POINT('Ctrl Pts',(40.4797092734487,44.0698008980635,47.8154837068449));
#21686=CARTESIAN_POINT('Ctrl Pts',(40.4801441411887,44.0695050894838,47.8110126486227));
#21687=CARTESIAN_POINT('Ctrl Pts',(40.4812210748171,44.0688000360116,47.8003277305434));
#21688=CARTESIAN_POINT('Ctrl Pts',(40.4818777082651,44.0683916128377,47.7941154314454));
#21689=CARTESIAN_POINT('Ctrl Pts',(40.4839554061722,44.0671609518959,47.7753319779812));
#21690=CARTESIAN_POINT('Ctrl Pts',(40.4854699979236,44.0663437474693,47.7627712129868));
#21691=CARTESIAN_POINT('Ctrl Pts',(40.5001076258453,44.0590945534547,47.6506691373463));
#21692=CARTESIAN_POINT('Ctrl Pts',(40.5208614714453,44.0530386114581,47.552264448604));
#21693=CARTESIAN_POINT('Ctrl Pts',(40.593792426295,44.0375753268503,47.3041768244243));
#21694=CARTESIAN_POINT('Ctrl Pts',(40.6568812889464,44.0282546936184,47.1585207093695));
#21695=CARTESIAN_POINT('Ctrl Pts',(40.7490479257255,44.0167688779226,47.0017708137638));
#21696=CARTESIAN_POINT('Ctrl Pts',(40.7614356743688,44.0152593297112,46.9815643702612));
#21697=CARTESIAN_POINT('Ctrl Pts',(40.7803229166398,44.013004184184,46.9519931169555));
#21698=CARTESIAN_POINT('Ctrl Pts',(40.7865384954973,44.0122690801958,46.942448939493));
#21699=CARTESIAN_POINT('Ctrl Pts',(40.7977626646186,44.0109536966941,46.9255432323975));
#21700=CARTESIAN_POINT('Ctrl Pts',(40.8027384309435,44.0103746635257,46.9181602244851));
#21701=CARTESIAN_POINT('Ctrl Pts',(40.8133558779722,44.0091475041356,46.9026390558817));
#21702=CARTESIAN_POINT('Ctrl Pts',(40.8190094541697,44.0084989360779,46.894509385194));
#21703=CARTESIAN_POINT('Ctrl Pts',(40.8342442795958,44.0067638449538,46.8729580681041));
#21704=CARTESIAN_POINT('Ctrl Pts',(40.843935284495,44.0056731218927,46.8596153874515));
#21705=CARTESIAN_POINT('Ctrl Pts',(40.8934581210256,44.0001619490616,46.7932385307542));
#21706=CARTESIAN_POINT('Ctrl Pts',(40.9358309704575,43.9956424667775,46.7421649727376));
#21707=CARTESIAN_POINT('Ctrl Pts',(41.0867129800117,43.980164491468,46.5782765625424));
#21708=CARTESIAN_POINT('Ctrl Pts',(41.2062731361509,43.968806573042,46.476508076267));
#21709=CARTESIAN_POINT('Ctrl Pts',(41.3795019024677,43.9542145375196,46.3620911372923));
#21710=CARTESIAN_POINT('Ctrl Pts',(41.4233161831185,43.9506679324602,46.335592734507));
#21711=CARTESIAN_POINT('Ctrl Pts',(41.4774028104587,43.9465040608731,46.3057541561646));
#21712=CARTESIAN_POINT('Ctrl Pts',(41.4867112498932,43.9457948849207,46.3007183209059));
#21713=CARTESIAN_POINT('Ctrl Pts',(41.501258237666,43.9446986714798,46.2930025152234));
#21714=CARTESIAN_POINT('Ctrl Pts',(41.5064682295816,43.9443084499135,46.2902695692181));
#21715=CARTESIAN_POINT('Ctrl Pts',(41.516111693892,43.9435906767285,46.2852671276505));
#21716=CARTESIAN_POINT('Ctrl Pts',(41.5205414455149,43.9432627241665,46.2829909688371));
#21717=CARTESIAN_POINT('Ctrl Pts',(41.5306639730694,43.9425172703144,46.2778391179925));
#21718=CARTESIAN_POINT('Ctrl Pts',(41.5363622301048,43.9421004599446,46.2749744823581));
#21719=CARTESIAN_POINT('Ctrl Pts',(41.5540043644087,43.940818375033,46.266214735048));
#21720=CARTESIAN_POINT('Ctrl Pts',(41.5659954668941,43.9399587707146,46.2604148704296));
#21721=CARTESIAN_POINT('Ctrl Pts',(41.5942106864125,43.9379613872016,46.2471265332531));
#21722=CARTESIAN_POINT('Ctrl Pts',(41.6104809093452,43.936828929371,46.239738240181));
#21723=CARTESIAN_POINT('Ctrl Pts',(41.6687133144725,43.9328359275574,46.2142648480355));
#21724=CARTESIAN_POINT('Ctrl Pts',(41.7112148782668,43.9300313216531,46.1974446269455));
#21725=CARTESIAN_POINT('Ctrl Pts',(41.8827669088913,43.9189934961097,46.1365071921942));
#21726=CARTESIAN_POINT('Ctrl Pts',(42.0157339164397,43.9110340671312,46.104616951551));
#21727=CARTESIAN_POINT('Ctrl Pts',(42.2186752124673,43.8985663858154,46.078196792599));
#21728=CARTESIAN_POINT('Ctrl Pts',(42.286808694316,43.8943336019554,46.072983538407));
#21729=CARTESIAN_POINT('Ctrl Pts',(42.3721104073123,43.8889018105405,46.070996305141));
#21730=CARTESIAN_POINT('Ctrl Pts',(42.3891546993872,43.8878100300894,46.0708251936027));
#21731=CARTESIAN_POINT('Ctrl Pts',(42.4163180270974,43.8860588096875,46.0709124740152));
#21732=CARTESIAN_POINT('Ctrl Pts',(42.4264368854148,43.8854039583007,46.0710246125147));
#21733=CARTESIAN_POINT('Ctrl Pts',(42.4453371591557,43.8841759556817,46.0713828097941));
#21734=CARTESIAN_POINT('Ctrl Pts',(42.4541187185341,43.8836034356067,46.0716092500855));
#21735=CARTESIAN_POINT('Ctrl Pts',(42.4738922441569,43.8823097353178,46.0722542987999));
#21736=CARTESIAN_POINT('Ctrl Pts',(42.4848827167647,43.8815875040528,46.0727069584259));
#21737=CARTESIAN_POINT('Ctrl Pts',(42.5175444788061,43.8794314257994,46.0743320996273));
#21738=CARTESIAN_POINT('Ctrl Pts',(42.5391998942937,43.877989130819,46.0757762887909));
#21739=CARTESIAN_POINT('Ctrl Pts',(42.5886386083864,43.8746659511311,46.0799122391407));
#21740=CARTESIAN_POINT('Ctrl Pts',(42.6163965576802,43.872778013412,46.0828422265461));
#21741=CARTESIAN_POINT('Ctrl Pts',(42.7108900058775,43.8662743529486,46.0948947136178));
#21742=CARTESIAN_POINT('Ctrl Pts',(42.7772015130253,43.8615769427655,46.1069082975719));
#21743=CARTESIAN_POINT('Ctrl Pts',(42.9234178890359,43.850956840166,46.1413858726562));
#21744=CARTESIAN_POINT('Ctrl Pts',(43.0027805898271,43.8450107319942,46.1655879590356));
#21745=CARTESIAN_POINT('Ctrl Pts',(43.1598118098149,43.8330571387581,46.2247699007983));
#21746=CARTESIAN_POINT('Ctrl Pts',(43.2372314064008,43.8270649837217,46.2599417066109));
#21747=CARTESIAN_POINT('Ctrl Pts',(43.3213789463785,43.82061606856,46.3050915762605));
#21748=CARTESIAN_POINT('Ctrl Pts',(43.3306290300838,43.8199081243847,46.3101528624677));
#21749=CARTESIAN_POINT('Ctrl Pts',(43.345465030567,43.8187747914756,46.3184293178073));
#21750=CARTESIAN_POINT('Ctrl Pts',(43.3510769955171,43.8183465838505,46.3215969986883));
#21751=CARTESIAN_POINT('Ctrl Pts',(43.3610024518412,43.8175902679387,46.3272652031216));
#21752=CARTESIAN_POINT('Ctrl Pts',(43.3653222372219,43.8172614556712,46.329754391276));
#21753=CARTESIAN_POINT('Ctrl Pts',(43.3746768542666,43.8165501944101,46.3351932142708));
#21754=CARTESIAN_POINT('Ctrl Pts',(43.3797079769292,43.8161681448506,46.3381489578728));
#21755=CARTESIAN_POINT('Ctrl Pts',(43.3938912827197,43.8150922444615,46.3465683306048));
#21756=CARTESIAN_POINT('Ctrl Pts',(43.4030118766294,43.8144017353067,46.3520851493039));
#21757=CARTESIAN_POINT('Ctrl Pts',(43.4630022523947,43.8098656645753,46.3890544099371));
#21758=CARTESIAN_POINT('Ctrl Pts',(43.5124369929753,43.8061548070958,46.4227856938001));
#21759=CARTESIAN_POINT('Ctrl Pts',(43.6300530378476,43.7971859385698,46.5113259929496));
#21760=CARTESIAN_POINT('Ctrl Pts',(43.6962272156501,43.7920109907518,46.5685751417703));
#21761=CARTESIAN_POINT('Ctrl Pts',(43.8452587444114,43.779475606459,46.7163457783542));
#21762=CARTESIAN_POINT('Ctrl Pts',(43.92380328119,43.7720859501231,46.8106477428373));
#21763=CARTESIAN_POINT('Ctrl Pts',(44.0024487612938,43.7632293631749,46.9257614385125));
#21764=CARTESIAN_POINT('Ctrl Pts',(44.0118359322739,43.7621447488908,46.9398983927712));
#21765=CARTESIAN_POINT('Ctrl Pts',(44.0269902834931,43.7603465658684,46.9633873254915));
#21766=CARTESIAN_POINT('Ctrl Pts',(44.032866364946,43.7596370684299,46.9726681911334));
#21767=CARTESIAN_POINT('Ctrl Pts',(44.0433406826263,43.7583496625795,46.9895285549876));
#21768=CARTESIAN_POINT('Ctrl Pts',(44.0479665739168,43.7577727963455,46.9970905787663));
#21769=CARTESIAN_POINT('Ctrl Pts',(44.0577817747028,43.7565306615202,47.0133869257393));
#21770=CARTESIAN_POINT('Ctrl Pts',(44.0629545151425,43.7558648089082,47.0221308652526));
#21771=CARTESIAN_POINT('Ctrl Pts',(44.0769362061054,43.7540336284165,47.0461971466891));
#21772=CARTESIAN_POINT('Ctrl Pts',(44.0856038540458,43.7528632486421,47.0616000138322));
#21773=CARTESIAN_POINT('Ctrl Pts',(44.1353635423867,43.7459302643111,47.1529399073332));
#21774=CARTESIAN_POINT('Ctrl Pts',(44.1715260081066,43.7399953975201,47.2314368932607));
#21775=CARTESIAN_POINT('Ctrl Pts',(44.2476315743987,43.7250031603343,47.4308292315819));
#21776=CARTESIAN_POINT('Ctrl Pts',(44.2811064191148,43.715817018117,47.5537562068724));
#21777=CARTESIAN_POINT('Ctrl Pts',(44.3118394863456,43.7027851189303,47.7359243846737));
#21778=CARTESIAN_POINT('Ctrl Pts',(44.3188779749747,43.6987748366,47.7931792030661));
#21779=CARTESIAN_POINT('Ctrl Pts',(44.3241129056797,43.6942132499683,47.8606035209589));
#21780=CARTESIAN_POINT('Ctrl Pts',(44.3248072924222,43.6935448041562,47.8705444108917));
#21781=CARTESIAN_POINT('Ctrl Pts',(44.3258131360316,43.6924622958709,47.8867496155983));
#21782=CARTESIAN_POINT('Ctrl Pts',(44.3261711187319,43.6920457949093,47.8930107080291));
#21783=CARTESIAN_POINT('Ctrl Pts',(44.3267582758952,43.6913020052596,47.9042407013748));
#21784=CARTESIAN_POINT('Ctrl Pts',(44.3269987707252,43.6909741042078,47.9092088310919));
#21785=CARTESIAN_POINT('Ctrl Pts',(44.3274855348091,43.6902551967842,47.9201396151387));
#21786=CARTESIAN_POINT('Ctrl Pts',(44.3277233543404,43.6898646634689,47.9261025070023));
#21787=CARTESIAN_POINT('Ctrl Pts',(44.3283308542687,43.688739996444,47.943343184428));
#21788=CARTESIAN_POINT('Ctrl Pts',(44.3286292704426,43.6880097017303,47.9546234610542));
#21789=CARTESIAN_POINT('Ctrl Pts',(44.3302423000544,43.682141972275,48.0458788371182));
#21790=CARTESIAN_POINT('Ctrl Pts',(44.3266809532286,43.6772467427395,48.1258728991357));
#21791=CARTESIAN_POINT('Ctrl Pts',(44.3134586082108,43.6697669502737,48.2493376308208));
#21792=CARTESIAN_POINT('Ctrl Pts',(44.3072489656745,43.6671322529295,48.2930778549741));
#21793=CARTESIAN_POINT('Ctrl Pts',(44.2761556763671,43.6565024838846,48.4685645688254));
#21794=CARTESIAN_POINT('Ctrl Pts',(44.2390770143016,43.6485104838561,48.5977484454606));
#21795=CARTESIAN_POINT('Ctrl Pts',(44.1794290439232,43.6384619120511,48.7455310813909));
#21796=CARTESIAN_POINT('Ctrl Pts',(44.1694859274379,43.636850407855,48.768832733965));
#21797=CARTESIAN_POINT('Ctrl Pts',(44.1543381675142,43.6344803498472,48.8024798959907));
#21798=CARTESIAN_POINT('Ctrl Pts',(44.1494944116956,43.6337341251294,48.8129856599655));
#21799=CARTESIAN_POINT('Ctrl Pts',(44.1407353023115,43.6324046412208,48.8315427266547));
#21800=CARTESIAN_POINT('Ctrl Pts',(44.1368578101212,43.6318227067984,48.8396116017844));
#21801=CARTESIAN_POINT('Ctrl Pts',(44.1286561801086,43.6306052267388,48.8563788437636));
#21802=CARTESIAN_POINT('Ctrl Pts',(44.1243222328192,43.6299693506033,48.8650721037106));
#21803=CARTESIAN_POINT('Ctrl Pts',(44.1128454799523,43.6283044754593,48.8876638446211));
#21804=CARTESIAN_POINT('Ctrl Pts',(44.1055992480987,43.6272718578881,48.9015086907929));
#21805=CARTESIAN_POINT('Ctrl Pts',(44.0717820977166,43.6225343157168,48.9642532402107));
#21806=CARTESIAN_POINT('Ctrl Pts',(44.0432734267204,43.6187609802245,49.0120726617762));
#21807=CARTESIAN_POINT('Ctrl Pts',(43.9539045223643,43.6075241113913,49.1482244551945));
#21808=CARTESIAN_POINT('Ctrl Pts',(43.8877043217979,43.5998899468667,49.2327894441272));
#21809=CARTESIAN_POINT('Ctrl Pts',(43.7446787911724,43.5848593983462,49.3870945477004));
#21810=CARTESIAN_POINT('Ctrl Pts',(43.6685586271243,43.5774915480332,49.4570365471399));
#21811=CARTESIAN_POINT('Ctrl Pts',(43.5742072607798,43.5693416658177,49.5307029889878));
#21812=CARTESIAN_POINT('Ctrl Pts',(43.561083112113,43.5682284851432,49.5406817916319));
#21813=CARTESIAN_POINT('Ctrl Pts',(43.5426417328059,43.5666943274142,49.5543339834343));
#21814=CARTESIAN_POINT('Ctrl Pts',(43.5374319833061,43.5662642019595,49.5581504253169));
#21815=CARTESIAN_POINT('Ctrl Pts',(43.5284170179191,43.5655256839152,49.5646850981975));
#21816=CARTESIAN_POINT('Ctrl Pts',(43.5246209434617,43.5652164532757,49.5674157577201));
#21817=CARTESIAN_POINT('Ctrl Pts',(43.5166001163627,43.5645668129532,49.573141301285));
#21818=CARTESIAN_POINT('Ctrl Pts',(43.5123731681496,43.5642266311973,49.5761330240599));
#21819=CARTESIAN_POINT('Ctrl Pts',(43.5018729310297,43.5633868186809,49.5835015344439));
#21820=CARTESIAN_POINT('Ctrl Pts',(43.4955854759229,43.562888546501,49.587858159757));
#21821=CARTESIAN_POINT('Ctrl Pts',(43.4718977907813,43.5610278414858,49.6040638515419));
#21822=CARTESIAN_POINT('Ctrl Pts',(43.4543291698906,43.5596809891024,49.6156657461265));
#21823=CARTESIAN_POINT('Ctrl Pts',(43.3159409335616,43.5492983452555,49.7038350541132));
#21824=CARTESIAN_POINT('Ctrl Pts',(43.187118939986,43.5409358818335,49.7670473995798));
#21825=CARTESIAN_POINT('Ctrl Pts',(42.9477406500279,43.5257104959986,49.8530810500426));
#21826=CARTESIAN_POINT('Ctrl Pts',(42.8399578479711,43.5189586897117,49.881584824778));
#21827=CARTESIAN_POINT('Ctrl Pts',(42.7135155694936,43.5108068347728,49.9035602775646));
#21828=CARTESIAN_POINT('Ctrl Pts',(42.6966658470497,43.509716278299,49.9062589247028));
#21829=CARTESIAN_POINT('Ctrl Pts',(42.668886008522,43.5079102735847,49.9103309049066));
#21830=CARTESIAN_POINT('Ctrl Pts',(42.6579757671994,43.5071989591367,49.9118348116516));
#21831=CARTESIAN_POINT('Ctrl Pts',(42.6382595782198,43.505909608294,49.9143807227299));
#21832=CARTESIAN_POINT('Ctrl Pts',(42.6294581275232,43.5053326285677,49.9154555963193));
#21833=CARTESIAN_POINT('Ctrl Pts',(42.610577385004,43.5040917509735,49.9176294006394));
#21834=CARTESIAN_POINT('Ctrl Pts',(42.6004962501935,43.5034272801634,49.9187096185345));
#21835=CARTESIAN_POINT('Ctrl Pts',(42.5729143611864,43.5016038194823,49.9214453391665));
#21836=CARTESIAN_POINT('Ctrl Pts',(42.5553991093112,43.5004398486277,49.9229411456379));
#21837=CARTESIAN_POINT('Ctrl Pts',(42.453703013485,43.4936448672338,49.9302275443369));
#21838=CARTESIAN_POINT('Ctrl Pts',(42.3692466707364,43.4878497115731,49.9307286396926));
#21839=CARTESIAN_POINT('Ctrl Pts',(42.1721038684476,43.4739896791129,49.9189595077675));
#21840=CARTESIAN_POINT('Ctrl Pts',(42.0599847530573,43.465843539056,49.9022957655123));
#21841=CARTESIAN_POINT('Ctrl Pts',(41.8974319923271,43.453975712517,49.8633003986517));
#21842=CARTESIAN_POINT('Ctrl Pts',(41.8454383540773,43.4501740579362,49.8484922372584));
#21843=CARTESIAN_POINT('Ctrl Pts',(41.7941388168303,43.4464579097838,49.8315225315644));
#21844=CARTESIAN_POINT('Origin',(42.4,48.4493818343519,48.));
#21845=CARTESIAN_POINT('',(41.7941388473837,42.4816651137235,49.8315225416714));
#21846=CARTESIAN_POINT('',(41.7941387803776,42.6541583936299,49.831522519506));
#21847=CARTESIAN_POINT('',(41.7941388317924,48.4493818343519,49.8315225365138));
#21848=CARTESIAN_POINT('',(40.4708700154104,43.1171846258035,47.9997561613629));
#21849=CARTESIAN_POINT('Ctrl Pts',(41.7941388473837,42.4816651137235,49.8315225416714));
#21850=CARTESIAN_POINT('Ctrl Pts',(41.8064630223161,42.482483011755,49.835599334973));
#21851=CARTESIAN_POINT('Ctrl Pts',(41.818829501791,42.4833047422321,49.8395521181629));
#21852=CARTESIAN_POINT('Ctrl Pts',(41.8482097833632,42.4852602051173,49.8486172222061));
#21853=CARTESIAN_POINT('Ctrl Pts',(41.8652541673143,42.4863971510643,49.8536194156301));
#21854=CARTESIAN_POINT('Ctrl Pts',(41.8922720476968,42.4882044730286,49.8611449844618));
#21855=CARTESIAN_POINT('Ctrl Pts',(41.9022010913276,42.4888697366671,49.8638252510529));
#21856=CARTESIAN_POINT('Ctrl Pts',(41.9207205486733,42.4901127853861,49.8686658931034));
#21857=CARTESIAN_POINT('Ctrl Pts',(41.9293053652268,42.4906898883104,49.8708467518466));
#21858=CARTESIAN_POINT('Ctrl Pts',(41.9484177902461,42.4919767901498,49.8755621332616));
#21859=CARTESIAN_POINT('Ctrl Pts',(41.9589522682066,42.4926875174423,49.8780672772906));
#21860=CARTESIAN_POINT('Ctrl Pts',(41.9898249471174,42.4947747934622,49.8851348578991));
#21861=CARTESIAN_POINT('Ctrl Pts',(42.0102161316325,42.496158999751,49.8894563991354));
#21862=CARTESIAN_POINT('Ctrl Pts',(42.1556092623919,42.506071652407,49.9178161415338));
#21863=CARTESIAN_POINT('Ctrl Pts',(42.2826279827468,42.5149879083897,49.9297560378969));
#21864=CARTESIAN_POINT('Ctrl Pts',(42.5410790763416,42.533410577361,49.9284331585886));
#21865=CARTESIAN_POINT('Ctrl Pts',(42.6718821183329,42.5428755706923,49.914377978479));
#21866=CARTESIAN_POINT('Ctrl Pts',(42.8156057942993,42.5528617198913,49.8838950852006));
#21867=CARTESIAN_POINT('Ctrl Pts',(42.8309188965244,42.5539199469981,49.8804514914747));
#21868=CARTESIAN_POINT('Ctrl Pts',(42.8521615097783,42.5553783311235,49.8754013476342));
#21869=CARTESIAN_POINT('Ctrl Pts',(42.8581274511205,42.5557868551339,49.8739529040816));
#21870=CARTESIAN_POINT('Ctrl Pts',(42.8689950331896,42.5565289618442,49.8712594127245));
#21871=CARTESIAN_POINT('Ctrl Pts',(42.8738988856499,42.55686305821,49.8700235237476));
#21872=CARTESIAN_POINT('Ctrl Pts',(42.8840389987243,42.5575522307446,49.8674255209777));
#21873=CARTESIAN_POINT('Ctrl Pts',(42.8892744601708,42.5579071462862,49.866060645613));
#21874=CARTESIAN_POINT('Ctrl Pts',(42.9029295318001,42.5588306151888,49.8624393739717));
#21875=CARTESIAN_POINT('Ctrl Pts',(42.9113398282644,42.5593971820126,49.8601478765829));
#21876=CARTESIAN_POINT('Ctrl Pts',(42.9486849695732,42.5619043257611,49.8497002694421));
#21877=CARTESIAN_POINT('Ctrl Pts',(42.9774441082996,42.5638119138052,49.840924991343));
#21878=CARTESIAN_POINT('Ctrl Pts',(43.0582494066556,42.5691367100614,49.8141886655199));
#21879=CARTESIAN_POINT('Ctrl Pts',(43.1097504510469,42.5724890569018,49.7946665351987));
#21880=CARTESIAN_POINT('Ctrl Pts',(43.1964598878373,42.5781711377423,49.7574805842364));
#21881=CARTESIAN_POINT('Ctrl Pts',(43.23208958716,42.5805173647586,49.7408944211078));
#21882=CARTESIAN_POINT('Ctrl Pts',(43.3910934682799,42.5911362585437,49.6608782824261));
#21883=CARTESIAN_POINT('Ctrl Pts',(43.507897169724,42.599387191362,49.5853520924081));
#21884=CARTESIAN_POINT('Ctrl Pts',(43.6351270256294,42.6097204451805,49.4821055622656));
#21885=CARTESIAN_POINT('Ctrl Pts',(43.6543521249132,42.6113212602249,49.4658704991461));
#21886=CARTESIAN_POINT('Ctrl Pts',(43.6819227125147,42.613678607839,49.4416483203481));
#21887=CARTESIAN_POINT('Ctrl Pts',(43.6905232361527,42.6144230043342,49.4339544929466));
#21888=CARTESIAN_POINT('Ctrl Pts',(43.7056707729474,42.6157505314537,49.42015720745));
#21889=CARTESIAN_POINT('Ctrl Pts',(43.7122453637348,42.6163323526687,49.4140844253525));
#21890=CARTESIAN_POINT('Ctrl Pts',(43.725880055521,42.6175509224679,49.4013134348597));
#21891=CARTESIAN_POINT('Ctrl Pts',(43.7329321885743,42.6181880110101,49.3946071271564));
#21892=CARTESIAN_POINT('Ctrl Pts',(43.7512285187791,42.6198590490037,49.3769424676549));
#21893=CARTESIAN_POINT('Ctrl Pts',(43.7623900170183,42.6208966648458,49.3658998813309));
#21894=CARTESIAN_POINT('Ctrl Pts',(43.8130568548912,42.6256926970787,49.3145339353961));
#21895=CARTESIAN_POINT('Ctrl Pts',(43.8509115752256,42.629521613006,49.2726286309728));
#21896=CARTESIAN_POINT('Ctrl Pts',(43.9569880798478,42.6410150481259,49.1443082197007));
#21897=CARTESIAN_POINT('Ctrl Pts',(44.0197109432773,42.6488604211206,49.0536530190111));
#21898=CARTESIAN_POINT('Ctrl Pts',(44.1237531765662,42.6638239032473,48.8718416577719));
#21899=CARTESIAN_POINT('Ctrl Pts',(44.1664044254,42.6709132787453,48.7818262140145));
#21900=CARTESIAN_POINT('Ctrl Pts',(44.2078072408997,42.6788065946554,48.6735330225806));
#21901=CARTESIAN_POINT('Ctrl Pts',(44.2134912060516,42.6799185687593,48.6580755600456));
#21902=CARTESIAN_POINT('Ctrl Pts',(44.2211270870521,42.6814514089007,48.6364592440801));
#21903=CARTESIAN_POINT('Ctrl Pts',(44.2232468848637,42.6818814019582,48.6303610365154));
#21904=CARTESIAN_POINT('Ctrl Pts',(44.2268493476047,42.6826198129632,48.6198273047643));
#21905=CARTESIAN_POINT('Ctrl Pts',(44.2283465546226,42.6829290677816,48.6153968670267));
#21906=CARTESIAN_POINT('Ctrl Pts',(44.2314685482322,42.6835789063445,48.6060464984561));
#21907=CARTESIAN_POINT('Ctrl Pts',(44.2330896510122,42.6839192611931,48.601125389497));
#21908=CARTESIAN_POINT('Ctrl Pts',(44.2370573240605,42.6847597576228,48.5889155922338));
#21909=CARTESIAN_POINT('Ctrl Pts',(44.2393803946537,42.685258536684,48.5816192528417));
#21910=CARTESIAN_POINT('Ctrl Pts',(44.247941034534,42.6871227609294,48.5541675070197));
#21911=CARTESIAN_POINT('Ctrl Pts',(44.2538915288623,42.688472552249,48.533923197382));
#21912=CARTESIAN_POINT('Ctrl Pts',(44.2978072444465,42.6989094084934,48.3749197776708));
#21913=CARTESIAN_POINT('Ctrl Pts',(44.320480197986,42.7073159210129,48.232387985803));
#21914=CARTESIAN_POINT('Ctrl Pts',(44.3321664322069,42.722541611044,47.978335406385));
#21915=CARTESIAN_POINT('Ctrl Pts',(44.3277596444973,42.7292435571353,47.8678089781625));
#21916=CARTESIAN_POINT('Ctrl Pts',(44.3117883733165,42.7373398321595,47.7413521500286));
#21917=CARTESIAN_POINT('Ctrl Pts',(44.3094268111809,42.7384299325873,47.72445922697));
#21918=CARTESIAN_POINT('Ctrl Pts',(44.3051723834534,42.7402354464551,47.6967146062724));
#21919=CARTESIAN_POINT('Ctrl Pts',(44.3034099956255,42.7409467318035,47.6858436361289));
#21920=CARTESIAN_POINT('Ctrl Pts',(44.3000604084328,42.7422362081907,47.6662461024846));
#21921=CARTESIAN_POINT('Ctrl Pts',(44.2985059111952,42.7428133438314,47.6575142038897));
#21922=CARTESIAN_POINT('Ctrl Pts',(44.2950444127382,42.7440547564853,47.638818406935));
#21923=CARTESIAN_POINT('Ctrl Pts',(44.2931189243271,42.74471960824,47.6288582466368));
#21924=CARTESIAN_POINT('Ctrl Pts',(44.2876389165738,42.7465446414545,47.6016640647011));
#21925=CARTESIAN_POINT('Ctrl Pts',(44.2839270831589,42.7477098162639,47.58446310994));
#21926=CARTESIAN_POINT('Ctrl Pts',(44.2609892347393,42.7545257504976,47.484799866778));
#21927=CARTESIAN_POINT('Ctrl Pts',(44.2365886640935,42.7603418541486,47.4036355026783));
#21928=CARTESIAN_POINT('Ctrl Pts',(44.1667398428654,42.7743399988669,47.2168350097494));
#21929=CARTESIAN_POINT('Ctrl Pts',(44.117025452517,42.7826083957699,47.1131302550583));
#21930=CARTESIAN_POINT('Ctrl Pts',(44.0401625750332,42.7932829239806,46.9837899621869));
#21931=CARTESIAN_POINT('Ctrl Pts',(44.0210826420139,42.7957991132616,46.9536217668829));
#21932=CARTESIAN_POINT('Ctrl Pts',(43.9798584843873,42.8009476791142,46.892276905242));
#21933=CARTESIAN_POINT('Ctrl Pts',(43.9576012310408,42.8035745978824,46.8611926597074));
#21934=CARTESIAN_POINT('Ctrl Pts',(43.9284785441651,42.8068078953192,46.8229730549326));
#21935=CARTESIAN_POINT('Ctrl Pts',(43.9224639535176,42.8074653514169,46.815203557688));
#21936=CARTESIAN_POINT('Ctrl Pts',(43.9128942978015,42.8084948916057,46.8030349289609));
#21937=CARTESIAN_POINT('Ctrl Pts',(43.9093788994098,42.8088696519123,46.7986050284478));
#21938=CARTESIAN_POINT('Ctrl Pts',(43.9027059310309,42.8095744652772,46.7902716638738));
#21939=CARTESIAN_POINT('Ctrl Pts',(43.8995526296431,42.8099047869644,46.7863650985981));
#21940=CARTESIAN_POINT('Ctrl Pts',(43.8921279384753,42.8106762528692,46.7772399057708));
#21941=CARTESIAN_POINT('Ctrl Pts',(43.8878443922079,42.8111165167494,46.7720313111644));
#21942=CARTESIAN_POINT('Ctrl Pts',(43.8737599049004,42.8125488809768,46.7550871212149));
#21943=CARTESIAN_POINT('Ctrl Pts',(43.8638464552114,42.8135332301481,46.7434452164594));
#21944=CARTESIAN_POINT('Ctrl Pts',(43.808414130964,42.8189157287396,46.6798945131296));
#21945=CARTESIAN_POINT('Ctrl Pts',(43.760267661785,42.823148195664,46.6303347779063));
#21946=CARTESIAN_POINT('Ctrl Pts',(43.6210540467661,42.8345930374396,46.5016347278824));
#21947=CARTESIAN_POINT('Ctrl Pts',(43.525072526141,42.8416630246131,46.4282862707686));
#21948=CARTESIAN_POINT('Ctrl Pts',(43.3594117468947,42.8535227856353,46.3246869083624));
#21949=CARTESIAN_POINT('Ctrl Pts',(43.2937017392239,42.8581464911346,46.2887314308566));
#21950=CARTESIAN_POINT('Ctrl Pts',(43.2102812569007,42.8640196517993,46.2492023898993));
#21951=CARTESIAN_POINT('Ctrl Pts',(43.1943875344759,42.8651385908506,46.241933903511));
#21952=CARTESIAN_POINT('Ctrl Pts',(43.1690469699447,42.8669235979914,46.2307589892593));
#21953=CARTESIAN_POINT('Ctrl Pts',(43.1596638104627,42.8675847658357,46.2267098701942));
#21954=CARTESIAN_POINT('Ctrl Pts',(43.1420845385212,42.8688240642544,46.2192890091701));
#21955=CARTESIAN_POINT('Ctrl Pts',(43.1338964723469,42.8694015471476,46.2158988093074));
#21956=CARTESIAN_POINT('Ctrl Pts',(43.1155758638925,42.870694335968,46.2084607763376));
#21957=CARTESIAN_POINT('Ctrl Pts',(43.1054318185329,42.8714106119728,46.2044422738388));
#21958=CARTESIAN_POINT('Ctrl Pts',(43.0754312418341,42.8735306290427,46.1928511928368));
#21959=CARTESIAN_POINT('Ctrl Pts',(43.0554835867018,42.8749423978768,46.1855206312639));
#21960=CARTESIAN_POINT('Ctrl Pts',(42.9002203639791,42.8859514841693,46.1313573344985));
#21961=CARTESIAN_POINT('Ctrl Pts',(42.7602161300534,42.8960487230764,46.0994014203309));
#21962=CARTESIAN_POINT('Ctrl Pts',(42.5053847581452,42.9143663694379,46.0704192086731));
#21963=CARTESIAN_POINT('Ctrl Pts',(42.3918532351142,42.9224898657566,46.0675594961786));
#21964=CARTESIAN_POINT('Ctrl Pts',(42.2625137749523,42.9313100999593,46.0757069478478));
#21965=CARTESIAN_POINT('Ctrl Pts',(42.2463212854115,42.9324062335398,46.0769323704122));
#21966=CARTESIAN_POINT('Ctrl Pts',(42.2237530503901,42.9339208920289,46.078927186937));
#21967=CARTESIAN_POINT('Ctrl Pts',(42.2173632876267,42.9343482729947,46.0795241281049));
#21968=CARTESIAN_POINT('Ctrl Pts',(42.2063322541284,42.9350834170212,46.0806102169387));
#21969=CARTESIAN_POINT('Ctrl Pts',(42.2016896094386,42.9353920003094,46.0810843360712));
#21970=CARTESIAN_POINT('Ctrl Pts',(42.191885273169,42.9360418733012,46.082121542847));
#21971=CARTESIAN_POINT('Ctrl Pts',(42.18672404891,42.9363829260291,46.0826886309725));
#21972=CARTESIAN_POINT('Ctrl Pts',(42.1739040138135,42.937227587697,46.084149636133));
#21973=CARTESIAN_POINT('Ctrl Pts',(42.1662480526417,42.937729804059,46.0850686582135));
#21974=CARTESIAN_POINT('Ctrl Pts',(42.1372798205406,42.9396224125798,46.0887223269825));
#21975=CARTESIAN_POINT('Ctrl Pts',(42.1160073187364,42.9409965285494,46.0917671823678));
#21976=CARTESIAN_POINT('Ctrl Pts',(42.0614196160911,42.9444924872656,46.1005137564378));
#21977=CARTESIAN_POINT('Ctrl Pts',(42.0281944181947,42.9465912712206,46.1067368003444));
#21978=CARTESIAN_POINT('Ctrl Pts',(41.9019273335135,42.9545142015236,46.1338390643839));
#21979=CARTESIAN_POINT('Ctrl Pts',(41.810312831732,42.9601567612324,46.1607326924264));
#21980=CARTESIAN_POINT('Ctrl Pts',(41.6044397705594,42.9732894552609,46.2381404684115));
#21981=CARTESIAN_POINT('Ctrl Pts',(41.4923596724948,42.9807983524011,46.2931759880739));
#21982=CARTESIAN_POINT('Ctrl Pts',(41.3705879936912,42.9898893550905,46.3683757352764));
#21983=CARTESIAN_POINT('Ctrl Pts',(41.3549432338029,42.9910758019406,46.3783517221726));
#21984=CARTESIAN_POINT('Ctrl Pts',(41.330639386907,42.9929494413156,46.3943469969767));
#21985=CARTESIAN_POINT('Ctrl Pts',(41.3218813497263,42.9936309571743,46.400214434503));
#21986=CARTESIAN_POINT('Ctrl Pts',(41.3060331481791,42.9948760279561,46.4110211633118));
#21987=CARTESIAN_POINT('Ctrl Pts',(41.2989271978326,42.9954386782114,46.4159369025948));
#21988=CARTESIAN_POINT('Ctrl Pts',(41.2915315015136,42.9960289460104,46.421126889021));
#21989=CARTESIAN_POINT('Ctrl Pts',(41.2912084655882,42.9960547376362,46.4213537299554));
#21990=CARTESIAN_POINT('Ctrl Pts',(41.2905851640724,42.9961045209791,46.4217917078338));
#21991=CARTESIAN_POINT('Ctrl Pts',(41.2902848890574,42.9961285121799,46.4220028313765));
#21992=CARTESIAN_POINT('Ctrl Pts',(41.2897027831224,42.9961750366911,46.4224123587304));
#21993=CARTESIAN_POINT('Ctrl Pts',(41.2894209450126,42.9961975696148,46.4226107524406));
#21994=CARTESIAN_POINT('Ctrl Pts',(41.2888723150507,42.9962414464674,46.4229971683064));
#21995=CARTESIAN_POINT('Ctrl Pts',(41.2886055177166,42.9962627900947,46.4231851826609));
#21996=CARTESIAN_POINT('Ctrl Pts',(41.2880842408237,42.9963045045029,46.4235527289544));
#21997=CARTESIAN_POINT('Ctrl Pts',(41.2878297569839,42.9963248750503,46.4237322548371));
#21998=CARTESIAN_POINT('Ctrl Pts',(41.287330871325,42.9963648206045,46.4240843751918));
#21999=CARTESIAN_POINT('Ctrl Pts',(41.2870864661852,42.9963843954257,46.4242569648979));
#22000=CARTESIAN_POINT('Ctrl Pts',(41.2866058715751,42.9964228977067,46.4245965103033));
#22001=CARTESIAN_POINT('Ctrl Pts',(41.2863696794509,42.9964418250248,46.4247634622974));
#22002=CARTESIAN_POINT('Ctrl Pts',(41.2859039247204,42.9964791583864,46.4250928373308));
#22003=CARTESIAN_POINT('Ctrl Pts',(41.2856743600918,42.996497564315,46.4252552574391));
#22004=CARTESIAN_POINT('Ctrl Pts',(41.2852204896007,42.9965339640057,46.42557652595));
#22005=CARTESIAN_POINT('Ctrl Pts',(41.2849961820487,42.9965519576894,46.4257353721817));
#22006=CARTESIAN_POINT('Ctrl Pts',(41.2845516204484,42.9965876289632,46.4260503367831));
#22007=CARTESIAN_POINT('Ctrl Pts',(41.2843313652555,42.9966053064839,46.4262064534278));
#22008=CARTESIAN_POINT('Ctrl Pts',(41.2838938314484,42.9966404314073,46.426516714931));
#22009=CARTESIAN_POINT('Ctrl Pts',(41.2836765520593,42.9966578787562,46.4266708585142));
#22010=CARTESIAN_POINT('Ctrl Pts',(41.2742044384064,42.9974186691157,46.4333935693888));
#22011=CARTESIAN_POINT('Ctrl Pts',(41.2650078885551,42.9981651442654,46.4400435094194));
#22012=CARTESIAN_POINT('Ctrl Pts',(41.2453618047822,42.9997769446754,46.4545151066457));
#22013=CARTESIAN_POINT('Ctrl Pts',(41.2349319553795,43.0006432467611,46.462362411183));
#22014=CARTESIAN_POINT('Ctrl Pts',(41.1483491824757,43.0079253367884,46.5288930173265));
#22015=CARTESIAN_POINT('Ctrl Pts',(41.0766131644606,43.0145608886104,46.593078650251));
#22016=CARTESIAN_POINT('Ctrl Pts',(40.9286095496375,43.0296205056926,46.7468761745433));
#22017=CARTESIAN_POINT('Ctrl Pts',(40.8551378749106,43.0380906247425,46.8386608009726));
#22018=CARTESIAN_POINT('Ctrl Pts',(40.7590899929671,43.0503765464944,46.9840297805876));
#22019=CARTESIAN_POINT('Ctrl Pts',(40.7298316237233,43.0543335495474,47.0328805340369));
#22020=CARTESIAN_POINT('Ctrl Pts',(40.6980501352524,43.0588429169013,47.0917005152954));
#22021=CARTESIAN_POINT('Ctrl Pts',(40.6933940371286,43.0595094574922,47.1004793533341));
#22022=CARTESIAN_POINT('Ctrl Pts',(40.6859138250224,43.0605895713322,47.1148500830018));
#22023=CARTESIAN_POINT('Ctrl Pts',(40.6830488155163,43.0610055648211,47.1204203142092));
#22024=CARTESIAN_POINT('Ctrl Pts',(40.6779570038355,43.0617489135434,47.1304396358338));
#22025=CARTESIAN_POINT('Ctrl Pts',(40.675720241656,43.0620768765117,47.1348834620457));
#22026=CARTESIAN_POINT('Ctrl Pts',(40.6708338981159,43.0627964791208,47.1446855098964));
#22027=CARTESIAN_POINT('Ctrl Pts',(40.6681920168422,43.0631876410548,47.1500474150047));
#22028=CARTESIAN_POINT('Ctrl Pts',(40.6606167884098,43.0643156220048,47.1656038928636));
#22029=CARTESIAN_POINT('Ctrl Pts',(40.6557481378535,43.065048568306,47.1758299467089));
#22030=CARTESIAN_POINT('Ctrl Pts',(40.6164593051054,43.0710349805492,47.260259532205));
#22031=CARTESIAN_POINT('Ctrl Pts',(40.5866959650059,43.076035075355,47.3365504427054));
#22032=CARTESIAN_POINT('Ctrl Pts',(40.5105069092393,43.0911449539596,47.5757446024541));
#22033=CARTESIAN_POINT('Ctrl Pts',(40.4805893457751,43.1010078668195,47.7430221298709));
#22034=CARTESIAN_POINT('Ctrl Pts',(40.4720391729479,43.1127741992305,47.9303851764094));
#22035=CARTESIAN_POINT('Ctrl Pts',(40.4714643159154,43.1139324325308,47.9487237418962));
#22036=CARTESIAN_POINT('Ctrl Pts',(40.470965094922,43.1157911205326,47.9779627812974));
#22037=CARTESIAN_POINT('Ctrl Pts',(40.4708713927328,43.1164864610854,47.9888594717965));
#22038=CARTESIAN_POINT('Ctrl Pts',(40.4708700154104,43.1171846258035,47.9997561613629));
#22039=CARTESIAN_POINT('Ctrl Pts',(40.4708700152961,43.1171846838461,47.9997570672691));
#22040=CARTESIAN_POINT('Ctrl Pts',(40.4708691867194,43.1176062557005,48.0063367990707));
#22041=CARTESIAN_POINT('Ctrl Pts',(40.4709020206306,43.1180288511859,48.0129164416807));
#22042=CARTESIAN_POINT('Ctrl Pts',(40.4710492573248,43.1189669100671,48.0274849697494));
#22043=CARTESIAN_POINT('Ctrl Pts',(40.4711796306079,43.1194828568839,48.0354735207403));
#22044=CARTESIAN_POINT('Ctrl Pts',(40.471550273897,43.1205484984144,48.0519213408788));
#22045=CARTESIAN_POINT('Ctrl Pts',(40.4717965903867,43.1210983704599,48.0603802871184));
#22046=CARTESIAN_POINT('Ctrl Pts',(40.4724376332605,43.1222694301181,48.0783337627932));
#22047=CARTESIAN_POINT('Ctrl Pts',(40.4728468721927,43.1228910588557,48.0878275159865));
#22048=CARTESIAN_POINT('Ctrl Pts',(40.4740376087615,43.1244407069268,48.1114014448298));
#22049=CARTESIAN_POINT('Ctrl Pts',(40.4749033753785,43.1253713453995,48.1254766201613));
#22050=CARTESIAN_POINT('Ctrl Pts',(40.4788213904405,43.1289648396312,48.1795007139328));
#22051=CARTESIAN_POINT('Ctrl Pts',(40.48296337304,43.1316614393306,48.2193579752236));
#22052=CARTESIAN_POINT('Ctrl Pts',(40.5089853044917,43.1448817626614,48.411382869605));
#22053=CARTESIAN_POINT('Ctrl Pts',(40.547758894432,43.155920687225,48.5606788678566));
#22054=CARTESIAN_POINT('Ctrl Pts',(40.6315878158932,43.172280749307,48.7746319405569));
#22055=CARTESIAN_POINT('Ctrl Pts',(40.6635289140438,43.1776496924322,48.8438049889268));
#22056=CARTESIAN_POINT('Ctrl Pts',(40.7070441711018,43.1839165395718,48.9250404774965));
#22057=CARTESIAN_POINT('Ctrl Pts',(40.714786517364,43.1849973794551,48.9390712873937));
#22058=CARTESIAN_POINT('Ctrl Pts',(40.7260978020611,43.186526987497,48.958979254092));
#22059=CARTESIAN_POINT('Ctrl Pts',(40.7295244689828,43.1869841450365,48.9649358952295));
#22060=CARTESIAN_POINT('Ctrl Pts',(40.7355187414656,43.1877729916333,48.9752282217527));
#22061=CARTESIAN_POINT('Ctrl Pts',(40.7380716139452,43.1881056084452,48.9795723488135));
#22062=CARTESIAN_POINT('Ctrl Pts',(40.7434929548609,43.1888049052147,48.988715440387));
#22063=CARTESIAN_POINT('Ctrl Pts',(40.7463652855857,43.1891713311604,48.9935119757252));
#22064=CARTESIAN_POINT('Ctrl Pts',(40.7541911191952,43.1901589284921,49.0064524544127));
#22065=CARTESIAN_POINT('Ctrl Pts',(40.7591842738233,43.1907775794305,49.0145724109104));
#22066=CARTESIAN_POINT('Ctrl Pts',(40.7827271010708,43.1936433646494,49.0522297485454));
#22067=CARTESIAN_POINT('Ctrl Pts',(40.8020167110844,43.1958461637218,49.0812996071235));
#22068=CARTESIAN_POINT('Ctrl Pts',(40.8909163817015,43.2054566028717,49.2076935405672));
#22069=CARTESIAN_POINT('Ctrl Pts',(40.9687081603729,43.2124968292755,49.2989480374893));
#22070=CARTESIAN_POINT('Ctrl Pts',(41.1109009360525,43.224359327367,49.4373481161009));
#22071=CARTESIAN_POINT('Ctrl Pts',(41.1706495506119,43.229102887719,49.4887719939867));
#22072=CARTESIAN_POINT('Ctrl Pts',(41.2702041073036,43.2368377477768,49.5643665915635));
#22073=CARTESIAN_POINT('Ctrl Pts',(41.3080296069225,43.2397407203512,49.5910002257988));
#22074=CARTESIAN_POINT('Ctrl Pts',(41.3559653126048,43.2433964880269,49.6222374983448));
#22075=CARTESIAN_POINT('Ctrl Pts',(41.3652080920163,43.2441003231359,49.6281488349178));
#22076=CARTESIAN_POINT('Ctrl Pts',(41.3831864221297,43.245467650845,49.6394321772678));
#22077=CARTESIAN_POINT('Ctrl Pts',(41.3919153895778,43.2461307540997,49.6448140100018));
#22078=CARTESIAN_POINT('Ctrl Pts',(41.4081058405409,43.2473594724225,49.654618918038));
#22079=CARTESIAN_POINT('Ctrl Pts',(41.4155550812215,43.2479243426073,49.6590617786114));
#22080=CARTESIAN_POINT('Ctrl Pts',(41.4321154461181,43.2491792140088,49.6687878742903));
#22081=CARTESIAN_POINT('Ctrl Pts',(41.4412403328401,43.2498700689745,49.6740470041675));
#22082=CARTESIAN_POINT('Ctrl Pts',(41.4665210914475,43.2517827426571,49.688343079832));
#22083=CARTESIAN_POINT('Ctrl Pts',(41.4827643282326,43.2530101556091,49.6972224101654));
#22084=CARTESIAN_POINT('Ctrl Pts',(41.5938307375592,43.2613951900539,49.7558765560863));
#22085=CARTESIAN_POINT('Ctrl Pts',(41.6925074132272,43.2688232141108,49.7979032234379));
#22086=CARTESIAN_POINT('Ctrl Pts',(41.7941388354972,43.276409063163,49.8315225377394));
#22087=CARTESIAN_POINT('',(40.470870769445,43.2895297265089,48.001722996834));
#22088=CARTESIAN_POINT('Ctrl Pts',(41.7941388168303,43.4464579097838,49.8315225315644));
#22089=CARTESIAN_POINT('Ctrl Pts',(41.7761768129493,43.4451567388353,49.8255807641355));
#22090=CARTESIAN_POINT('Ctrl Pts',(41.7582998990573,43.4438661233107,49.81937399617));
#22091=CARTESIAN_POINT('Ctrl Pts',(41.7307636638786,43.4418880138451,49.8093570494479));
#22092=CARTESIAN_POINT('Ctrl Pts',(41.7210418610757,43.4411915573444,49.805731448244));
#22093=CARTESIAN_POINT('Ctrl Pts',(41.7053766573696,43.4400729799323,49.7997449413589));
#22094=CARTESIAN_POINT('Ctrl Pts',(41.6994150688083,43.4396481531526,49.7974326688846));
#22095=CARTESIAN_POINT('Ctrl Pts',(41.6888295573247,43.4388954987841,49.7932662864778));
#22096=CARTESIAN_POINT('Ctrl Pts',(41.6842012080984,43.4385669935767,49.7914238650287));
#22097=CARTESIAN_POINT('Ctrl Pts',(41.6741337302187,43.4378537215749,49.7873710254473));
#22098=CARTESIAN_POINT('Ctrl Pts',(41.6686975308336,43.4374693744035,49.7851536978842));
#22099=CARTESIAN_POINT('Ctrl Pts',(41.6536181768234,43.4364052498043,49.7789226593268));
#22100=CARTESIAN_POINT('Ctrl Pts',(41.6439971969751,43.4357286040933,49.7748553257913));
#22101=CARTESIAN_POINT('Ctrl Pts',(41.6221561935667,43.4341967064757,49.7654120708336));
#22102=CARTESIAN_POINT('Ctrl Pts',(41.6099578614026,43.4333441432331,49.7599869909483));
#22103=CARTESIAN_POINT('Ctrl Pts',(41.5707951915101,43.4306136532361,49.7420805769805));
#22104=CARTESIAN_POINT('Ctrl Pts',(41.5440614684296,43.4287599847571,49.729102302794));
#22105=CARTESIAN_POINT('Ctrl Pts',(41.4215373756617,43.420264083815,49.6660827417399));
#22106=CARTESIAN_POINT('Ctrl Pts',(41.3297544440341,43.413890009113,49.6086636124085));
#22107=CARTESIAN_POINT('Ctrl Pts',(41.1485050237377,43.4003540529157,49.4728615919337));
#22108=CARTESIAN_POINT('Ctrl Pts',(41.0605016272557,43.3931965071083,49.3933052886631));
#22109=CARTESIAN_POINT('Ctrl Pts',(40.9687728368603,43.3845917004353,49.29360880437));
#22110=CARTESIAN_POINT('Ctrl Pts',(40.9573634452525,43.3834989610702,49.2808726213637));
#22111=CARTESIAN_POINT('Ctrl Pts',(40.9388792798639,43.3816900835254,49.2596786596117));
#22112=CARTESIAN_POINT('Ctrl Pts',(40.9317048888039,43.3809781021997,49.2513087318448));
#22113=CARTESIAN_POINT('Ctrl Pts',(40.9188895869558,43.379688035779,49.2360959254372));
#22114=CARTESIAN_POINT('Ctrl Pts',(40.9132233362289,43.3791110126694,49.2292747211909));
#22115=CARTESIAN_POINT('Ctrl Pts',(40.9011845171979,43.3778705881727,49.2145770254516));
#22116=CARTESIAN_POINT('Ctrl Pts',(40.8948265896499,43.3772066178663,49.2066889410113));
#22117=CARTESIAN_POINT('Ctrl Pts',(40.8776292788225,43.3753859514126,49.1850053777982));
#22118=CARTESIAN_POINT('Ctrl Pts',(40.8669157078838,43.3742242998406,49.1711118121825));
#22119=CARTESIAN_POINT('Ctrl Pts',(40.8103085637684,43.3679346890437,49.095594492469));
#22120=CARTESIAN_POINT('Ctrl Pts',(40.7679438016097,43.3626723101874,49.0314242661745));
#22121=CARTESIAN_POINT('Ctrl Pts',(40.6756291536202,43.3497659340359,48.8716060407526));
#22122=CARTESIAN_POINT('Ctrl Pts',(40.6296510097581,43.3420310535434,48.7739594924638));
#22123=CARTESIAN_POINT('Ctrl Pts',(40.562192431016,43.3282549881674,48.5927389771338));
#22124=CARTESIAN_POINT('Ctrl Pts',(40.5376908329482,43.3222110482301,48.5105724067162));
#22125=CARTESIAN_POINT('Ctrl Pts',(40.5163946678963,43.3157142083722,48.416755034115));
#22126=CARTESIAN_POINT('Ctrl Pts',(40.5141441680002,43.3150060121356,48.4064499953036));
#22127=CARTESIAN_POINT('Ctrl Pts',(40.5106547889467,43.3138723557064,48.3898188948568));
#22128=CARTESIAN_POINT('Ctrl Pts',(40.5093629332993,43.3134440741202,48.3835043445843));
#22129=CARTESIAN_POINT('Ctrl Pts',(40.5071279229701,43.3126876777404,48.3722938544672));
#22130=CARTESIAN_POINT('Ctrl Pts',(40.5061720742926,43.3123588583899,48.3674006040953));
#22131=CARTESIAN_POINT('Ctrl Pts',(40.5041388603734,43.3116476394694,48.3567732254181));
#22132=CARTESIAN_POINT('Ctrl Pts',(40.5030685311495,43.3112656389007,48.3510378894507));
#22133=CARTESIAN_POINT('Ctrl Pts',(40.5009102771965,43.3104791041233,48.3391747527503));
#22134=CARTESIAN_POINT('Ctrl Pts',(40.4998259514978,43.3100747707399,48.3330463573078));
#22135=CARTESIAN_POINT('Ctrl Pts',(40.4971135140632,43.3090388467933,48.3172716149712));
#22136=CARTESIAN_POINT('Ctrl Pts',(40.4955290628552,43.3084095354203,48.3076178063816));
#22137=CARTESIAN_POINT('Ctrl Pts',(40.4786997314613,43.3014391903391,48.1999615826876));
#22138=CARTESIAN_POINT('Ctrl Pts',(40.4709593710398,43.29546088323,48.100924529371));
#22139=CARTESIAN_POINT('Ctrl Pts',(40.470870769445,43.2895297265089,48.001722996834));
#22140=CARTESIAN_POINT('Ctrl Pts',(40.470870770631,43.2895298058776,48.0017243243157));
#22141=CARTESIAN_POINT('Ctrl Pts',(40.4707541166506,43.2817267810287,47.871214882825));
#22142=CARTESIAN_POINT('Ctrl Pts',(40.4838808354969,43.2740228213524,47.7410348150679));
#22143=CARTESIAN_POINT('Ctrl Pts',(40.5174173845313,43.2636492378451,47.5771820820791));
#22144=CARTESIAN_POINT('Ctrl Pts',(40.5258104418137,43.2613439678219,47.5414091936409));
#22145=CARTESIAN_POINT('Ctrl Pts',(40.539745682672,43.257882335434,47.4888163225953));
#22146=CARTESIAN_POINT('Ctrl Pts',(40.54450649835,43.2567507473241,47.4717967160789));
#22147=CARTESIAN_POINT('Ctrl Pts',(40.5523712283617,43.2549567065817,47.4451002905912));
#22148=CARTESIAN_POINT('Ctrl Pts',(40.5553190002772,43.2542993530091,47.4353782080099));
#22149=CARTESIAN_POINT('Ctrl Pts',(40.5609824999741,43.2530636630526,47.4172172141841));
#22150=CARTESIAN_POINT('Ctrl Pts',(40.5636798844698,43.2524859431979,47.408772827317));
#22151=CARTESIAN_POINT('Ctrl Pts',(40.5698499344321,43.2511879896419,47.3899065929289));
#22152=CARTESIAN_POINT('Ctrl Pts',(40.57335358815,43.2504667475821,47.3794952817078));
#22153=CARTESIAN_POINT('Ctrl Pts',(40.5824958604471,43.248623691456,47.3530770795669));
#22154=CARTESIAN_POINT('Ctrl Pts',(40.588257039099,43.2474978493109,47.3371139053633));
#22155=CARTESIAN_POINT('Ctrl Pts',(40.6373551515685,43.238182795715,47.2064954311846));
#22156=CARTESIAN_POINT('Ctrl Pts',(40.6913106955539,43.2296306559741,47.0961542600228));
#22157=CARTESIAN_POINT('Ctrl Pts',(40.8092856755564,43.2135679449637,46.9037256890813));
#22158=CARTESIAN_POINT('Ctrl Pts',(40.8701884658898,43.2061387072989,46.8202258639562));
#22159=CARTESIAN_POINT('Ctrl Pts',(40.9572393556313,43.1967956922784,46.7190228101481));
#22160=CARTESIAN_POINT('Ctrl Pts',(40.9775400292117,43.1946947414766,46.6965167149004));
#22161=CARTESIAN_POINT('Ctrl Pts',(41.0118382876095,43.1912826196213,46.660248453157));
#22162=CARTESIAN_POINT('Ctrl Pts',(41.0255301015716,43.1899545898043,46.6462054371001));
#22163=CARTESIAN_POINT('Ctrl Pts',(41.0446247040912,43.1881516244909,46.6272094235261));
#22164=CARTESIAN_POINT('Ctrl Pts',(41.0498445463117,43.1876636600574,46.6220753232572));
#22165=CARTESIAN_POINT('Ctrl Pts',(41.0588279843742,43.1868324188253,46.6133395100025));
#22166=CARTESIAN_POINT('Ctrl Pts',(41.0625771321628,43.1864880244398,46.6097231338673));
#22167=CARTESIAN_POINT('Ctrl Pts',(41.0697008787049,43.1858384654623,46.6029071510149));
#22168=CARTESIAN_POINT('Ctrl Pts',(41.0730724669884,43.1855330576821,46.5997044940125));
#22169=CARTESIAN_POINT('Ctrl Pts',(41.0810789557544,43.1848124783659,46.5921540495342));
#22170=CARTESIAN_POINT('Ctrl Pts',(41.0857238593242,43.1843981127126,46.5878168780077));
#22171=CARTESIAN_POINT('Ctrl Pts',(41.1020451130176,43.1829545401866,46.5727272104199));
#22172=CARTESIAN_POINT('Ctrl Pts',(41.1138330371377,43.1819339870904,46.5620955917117));
#22173=CARTESIAN_POINT('Ctrl Pts',(41.2169495263108,43.1731812997313,46.4713768782964));
#22174=CARTESIAN_POINT('Ctrl Pts',(41.3155352466535,43.1659718170732,46.3999245034361));
#22175=CARTESIAN_POINT('Ctrl Pts',(41.5015704577851,43.1530912092974,46.2902368834838));
#22176=CARTESIAN_POINT('Ctrl Pts',(41.5863513956463,43.1474532602462,46.2483037481745));
#22177=CARTESIAN_POINT('Ctrl Pts',(41.7057053763789,43.1395145355678,46.1998113215623));
#22178=CARTESIAN_POINT('Ctrl Pts',(41.7378922896855,43.1373744343821,46.1877258828294));
#22179=CARTESIAN_POINT('Ctrl Pts',(41.7945001357346,43.133599070185,46.168180298256));
#22180=CARTESIAN_POINT('Ctrl Pts',(41.8187785817019,43.1319762905807,46.1603328913135));
#22181=CARTESIAN_POINT('Ctrl Pts',(41.8544329281658,43.1295845879111,46.1495847334892));
#22182=CARTESIAN_POINT('Ctrl Pts',(41.8656916408498,43.1288281282393,46.1463024368184));
#22183=CARTESIAN_POINT('Ctrl Pts',(41.8855908458022,43.1274886557041,46.1406974910744));
#22184=CARTESIAN_POINT('Ctrl Pts',(41.8942189570669,43.1269070605278,46.1383318959328));
#22185=CARTESIAN_POINT('Ctrl Pts',(41.9122661716195,43.1256887140195,46.1335185570328));
#22186=CARTESIAN_POINT('Ctrl Pts',(41.9216879455063,43.1250516211692,46.1310819073807));
#22187=CARTESIAN_POINT('Ctrl Pts',(41.9463657675858,43.1233800128109,46.1248985842091));
#22188=CARTESIAN_POINT('Ctrl Pts',(41.9616495967122,43.1223418244375,46.1212668536184));
#22189=CARTESIAN_POINT('Ctrl Pts',(42.0266915923158,43.1179103568648,46.1066484971889));
#22190=CARTESIAN_POINT('Ctrl Pts',(42.0768263219138,43.1144607999057,46.0974498608068));
#22191=CARTESIAN_POINT('Ctrl Pts',(42.1522507269199,43.1092182382893,46.0866782822063));
#22192=CARTESIAN_POINT('Ctrl Pts',(42.1773055905031,43.1074682575869,46.0836005604724));
#22193=CARTESIAN_POINT('Ctrl Pts',(42.3370708368975,43.0962598243401,46.0671504191077));
#22194=CARTESIAN_POINT('Ctrl Pts',(42.4728099022343,43.0864769656933,46.0674987858754));
#22195=CARTESIAN_POINT('Ctrl Pts',(42.6706589276612,43.0724040328661,46.0888909297531));
#22196=CARTESIAN_POINT('Ctrl Pts',(42.7335719570051,43.0679641415169,46.0988620099974));
#22197=CARTESIAN_POINT('Ctrl Pts',(42.8064609701078,43.0629430612375,46.1141450608485));
#22198=CARTESIAN_POINT('Ctrl Pts',(42.8170205135377,43.0622187366912,46.1164519447807));
#22199=CARTESIAN_POINT('Ctrl Pts',(42.8332814056699,43.0611086834193,46.1201478246893));
#22200=CARTESIAN_POINT('Ctrl Pts',(42.8389965376927,43.0607195626893,46.1214742430067));
#22201=CARTESIAN_POINT('Ctrl Pts',(42.8495534762029,43.0600027907616,46.1239752001683));
#22202=CARTESIAN_POINT('Ctrl Pts',(42.8543967739232,43.0596747477524,46.1251424186548));
#22203=CARTESIAN_POINT('Ctrl Pts',(42.8654512653732,43.0589277871756,46.1278518672668));
#22204=CARTESIAN_POINT('Ctrl Pts',(42.8716593472753,43.0585095719483,46.12940625085));
#22205=CARTESIAN_POINT('Ctrl Pts',(42.887929383402,43.0574165781021,46.1335661005816));
#22206=CARTESIAN_POINT('Ctrl Pts',(42.8979783751301,43.0567445806947,46.1362220804298));
#22207=CARTESIAN_POINT('Ctrl Pts',(42.9772609843494,43.0514635730865,46.1578637423645));
#22208=CARTESIAN_POINT('Ctrl Pts',(43.0454156983398,43.0470486348728,46.1806217332715));
#22209=CARTESIAN_POINT('Ctrl Pts',(43.2181792678902,43.0358099784963,46.2492455385647));
#22210=CARTESIAN_POINT('Ctrl Pts',(43.320263931079,43.0291105944545,46.3006843022093));
#22211=CARTESIAN_POINT('Ctrl Pts',(43.4890424145211,43.0171053161274,46.4054226642243));
#22212=CARTESIAN_POINT('Ctrl Pts',(43.5578619437439,43.0119041918912,46.4546704792855));
#22213=CARTESIAN_POINT('Ctrl Pts',(43.6368243346242,43.0054064745744,46.5194199031533));
#22214=CARTESIAN_POINT('Ctrl Pts',(43.6502702307908,43.0042802737057,46.5307565977705));
#22215=CARTESIAN_POINT('Ctrl Pts',(43.6712215619849,43.0024928520106,46.5489172560233));
#22216=CARTESIAN_POINT('Ctrl Pts',(43.6788316058072,43.0018366661885,46.5556194729273));
#22217=CARTESIAN_POINT('Ctrl Pts',(43.6929959229987,43.0006020064794,46.5682937738862));
#22218=CARTESIAN_POINT('Ctrl Pts',(43.6995625741055,43.0000241391273,46.5742516749651));
#22219=CARTESIAN_POINT('Ctrl Pts',(43.7141912966492,42.9987243184008,46.5877092961627));
#22220=CARTESIAN_POINT('Ctrl Pts',(43.722230645678,42.9980013436831,46.5952331483834));
#22221=CARTESIAN_POINT('Ctrl Pts',(43.7425577409355,42.9961508609826,46.6145859204196));
#22222=CARTESIAN_POINT('Ctrl Pts',(43.754753613385,42.9950192688974,46.6265095286991));
#22223=CARTESIAN_POINT('Ctrl Pts',(43.844868604185,42.9864940747393,46.7169807953295));
#22224=CARTESIAN_POINT('Ctrl Pts',(43.9160460750823,42.9788089208104,46.8019264271976));
#22225=CARTESIAN_POINT('Ctrl Pts',(44.0620329650053,42.9607686655669,47.0101343461055));
#22226=CARTESIAN_POINT('Ctrl Pts',(44.1311215009206,42.9503446010809,47.1366294302752));
#22227=CARTESIAN_POINT('Ctrl Pts',(44.1935074225809,42.9390637437029,47.2891425625455));
#22228=CARTESIAN_POINT('Ctrl Pts',(44.2011704915683,42.9376343655986,47.3087893796055));
#22229=CARTESIAN_POINT('Ctrl Pts',(44.2111742375575,42.9357100251437,47.3357342243179));
#22230=CARTESIAN_POINT('Ctrl Pts',(44.2137955466328,42.9351998969627,47.3429255297551));
#22231=CARTESIAN_POINT('Ctrl Pts',(44.218118838154,42.9343487403253,47.3550090901977));
#22232=CARTESIAN_POINT('Ctrl Pts',(44.219844022777,42.9340063683103,47.3598928853407));
#22233=CARTESIAN_POINT('Ctrl Pts',(44.2230889836003,42.9333572270065,47.369198151321));
#22234=CARTESIAN_POINT('Ctrl Pts',(44.2246123838327,42.9330502372792,47.3736182758472));
#22235=CARTESIAN_POINT('Ctrl Pts',(44.2282006310545,42.932321660967,47.3841536972047));
#22236=CARTESIAN_POINT('Ctrl Pts',(44.2302509025028,42.931900923855,47.3902739526123));
#22237=CARTESIAN_POINT('Ctrl Pts',(44.2374220894991,42.9304129336969,47.4120427594252));
#22238=CARTESIAN_POINT('Ctrl Pts',(44.2423735143219,42.92935504673,47.4277469711916));
#22239=CARTESIAN_POINT('Ctrl Pts',(44.2758104687147,42.9219750827021,47.5387328765873));
#22240=CARTESIAN_POINT('Ctrl Pts',(44.2970954680145,42.9159977488544,47.636041036543));
#22241=CARTESIAN_POINT('Ctrl Pts',(44.3259242975384,42.903481070421,47.8435725494755));
#22242=CARTESIAN_POINT('Ctrl Pts',(44.3317105371758,42.8969663731238,47.953667049074));
#22243=CARTESIAN_POINT('Ctrl Pts',(44.3262170847473,42.8867405391596,48.1200699951871));
#22244=CARTESIAN_POINT('Ctrl Pts',(44.3218793116618,42.8832171891892,48.1763747317665));
#22245=CARTESIAN_POINT('Ctrl Pts',(44.3131886726569,42.8786148635724,48.2479880662432));
#22246=CARTESIAN_POINT('Ctrl Pts',(44.3111074462546,42.8776076409016,48.2635474975751));
#22247=CARTESIAN_POINT('Ctrl Pts',(44.3074291192456,42.8759664392421,48.2887063750635));
#22248=CARTESIAN_POINT('Ctrl Pts',(44.3059488364976,42.8753361689039,48.2983223806951));
#22249=CARTESIAN_POINT('Ctrl Pts',(44.3029677354521,42.8741218269356,48.3167592289698));
#22250=CARTESIAN_POINT('Ctrl Pts',(44.3014781600874,42.8735381273917,48.3255816540619));
#22251=CARTESIAN_POINT('Ctrl Pts',(44.2979277685529,42.8721973773524,48.3457539669727));
#22252=CARTESIAN_POINT('Ctrl Pts',(44.2958264309725,42.8714390533499,48.357096281264));
#22253=CARTESIAN_POINT('Ctrl Pts',(44.288820679913,42.8690170229253,48.3931049021154));
#22254=CARTESIAN_POINT('Ctrl Pts',(44.2835357626495,42.8673412732813,48.4176936123286));
#22255=CARTESIAN_POINT('Ctrl Pts',(44.2459200630748,42.856306514292,48.5774365601054));
#22256=CARTESIAN_POINT('Ctrl Pts',(44.1995515044912,42.8464892464088,48.7088404387417));
#22257=CARTESIAN_POINT('Ctrl Pts',(44.1226160467818,42.8337793922827,48.8692866059474));
#22258=CARTESIAN_POINT('Ctrl Pts',(44.1046803404323,42.8309898770007,48.9039525649023));
#22259=CARTESIAN_POINT('Ctrl Pts',(44.058920322573,42.8242946922188,48.9861846784148));
#22260=CARTESIAN_POINT('Ctrl Pts',(44.0300839366676,42.8204047383894,49.0331524742518));
#22261=CARTESIAN_POINT('Ctrl Pts',(43.9824571725836,42.8145173885406,49.103755521919));
#22262=CARTESIAN_POINT('Ctrl Pts',(43.9650575277466,42.8124636692133,49.1282916885228));
#22263=CARTESIAN_POINT('Ctrl Pts',(43.9418833676139,42.8098595726407,49.1594025219305));
#22264=CARTESIAN_POINT('Ctrl Pts',(43.9366291621493,42.8092774301099,49.1663573004659));
#22265=CARTESIAN_POINT('Ctrl Pts',(43.9280380549988,42.8083391875214,49.1775701757878));
#22266=CARTESIAN_POINT('Ctrl Pts',(43.924730136477,42.8079811332171,49.1818501720399));
#22267=CARTESIAN_POINT('Ctrl Pts',(43.9182959514685,42.8072909492012,49.190103154022));
#22268=CARTESIAN_POINT('Ctrl Pts',(43.9151720233292,42.8069586716358,49.1940778257007));
#22269=CARTESIAN_POINT('Ctrl Pts',(43.9082218307476,42.806225519278,49.2028495821503));
#22270=CARTESIAN_POINT('Ctrl Pts',(43.9043881942443,42.8058251638368,49.2076408288754));
#22271=CARTESIAN_POINT('Ctrl Pts',(43.8906761565823,42.8044071382266,49.2246113940858));
#22272=CARTESIAN_POINT('Ctrl Pts',(43.8806718698636,42.8033980268368,49.2366888542377));
#22273=CARTESIAN_POINT('Ctrl Pts',(43.7855089102804,42.7940198729723,49.3487617884767));
#22274=CARTESIAN_POINT('Ctrl Pts',(43.6904814708786,42.7862670300302,49.4399517428875));
#22275=CARTESIAN_POINT('Ctrl Pts',(43.4869373108206,42.770860259021,49.5988096809996));
#22276=CARTESIAN_POINT('Ctrl Pts',(43.3795280964244,42.7632423367256,49.6667765490118));
#22277=CARTESIAN_POINT('Ctrl Pts',(43.2474268579138,42.7538754904716,49.733162822768));
#22278=CARTESIAN_POINT('Ctrl Pts',(43.2284657035034,42.7525318353256,49.742305992699));
#22279=CARTESIAN_POINT('Ctrl Pts',(43.1994937941521,42.7504781336782,49.755696542629));
#22280=CARTESIAN_POINT('Ctrl Pts',(43.1895900903884,42.749775991563,49.7601727636372));
#22281=CARTESIAN_POINT('Ctrl Pts',(43.1715476200334,42.7484963849554,49.7681445859927));
#22282=CARTESIAN_POINT('Ctrl Pts',(43.1634215425631,42.7479199039048,49.7716682959576));
#22283=CARTESIAN_POINT('Ctrl Pts',(43.1458426097537,42.7466723225122,49.7791476494624));
#22284=CARTESIAN_POINT('Ctrl Pts',(43.1363819634245,42.7460005914546,49.7830841691193));
#22285=CARTESIAN_POINT('Ctrl Pts',(43.110582672471,42.7441677067713,49.7935787620019));
#22286=CARTESIAN_POINT('Ctrl Pts',(43.0941852223347,42.74300160408,49.7999887088273));
#22287=CARTESIAN_POINT('Ctrl Pts',(43.0054542591068,42.7366835283692,49.8332818741423));
#22288=CARTESIAN_POINT('Ctrl Pts',(42.931653717996,42.731396034906,49.856027715763));
#22289=CARTESIAN_POINT('Ctrl Pts',(42.7306077192985,42.716919944404,49.9050154024218));
#22290=CARTESIAN_POINT('Ctrl Pts',(42.6017426471223,42.7075466553483,49.9229354592763));
#22291=CARTESIAN_POINT('Ctrl Pts',(42.4078443894754,42.6938213012057,49.9301843965695));
#22292=CARTESIAN_POINT('Ctrl Pts',(42.3435307826269,42.6893366913106,49.9293746093143));
#22293=CARTESIAN_POINT('Ctrl Pts',(42.2685618543556,42.6842721158948,49.924677602452));
#22294=CARTESIAN_POINT('Ctrl Pts',(42.257758000344,42.6835462567445,49.9239093238542));
#22295=CARTESIAN_POINT('Ctrl Pts',(42.2411076775928,42.6824343604537,49.9225842670244));
#22296=CARTESIAN_POINT('Ctrl Pts',(42.2352565287868,42.6820449140683,49.9220917316563));
#22297=CARTESIAN_POINT('Ctrl Pts',(42.2244456072618,42.6813278468881,49.9211319652107));
#22298=CARTESIAN_POINT('Ctrl Pts',(42.2194854049952,42.6809998315774,49.9206722402568));
#22299=CARTESIAN_POINT('Ctrl Pts',(42.2081634422171,42.6802533209486,49.9195786420002));
#22300=CARTESIAN_POINT('Ctrl Pts',(42.2018030108196,42.6798355245672,49.9189323552678));
#22301=CARTESIAN_POINT('Ctrl Pts',(42.1851326314525,42.678744360844,49.9171546994656));
#22302=CARTESIAN_POINT('Ctrl Pts',(42.1748282278167,42.6780737596555,49.9159717670626));
#22303=CARTESIAN_POINT('Ctrl Pts',(42.0928645744725,42.6727669345001,49.9058920528224));
#22304=CARTESIAN_POINT('Ctrl Pts',(42.021737952952,42.6683272009993,49.8930602248049));
#22305=CARTESIAN_POINT('Ctrl Pts',(41.8984164307745,42.6606629043884,49.8635810507729));
#22306=CARTESIAN_POINT('Ctrl Pts',(41.845918938182,42.6574112284475,49.8486512139258));
#22307=CARTESIAN_POINT('Ctrl Pts',(41.7941387803776,42.6541583936299,49.831522519506));
#22308=CARTESIAN_POINT('Origin',(42.4,48.4493818343519,48.));
#22309=CARTESIAN_POINT('',(41.7941388322699,41.6906508784004,49.8315225366718));
#22310=CARTESIAN_POINT('',(41.7941388317731,41.8624153300426,49.8315225365075));
#22311=CARTESIAN_POINT('',(41.7941388317924,48.4493818343519,49.8315225365138));
#22312=CARTESIAN_POINT('Ctrl Pts',(41.7941388322699,41.6906508784004,49.8315225366718));
#22313=CARTESIAN_POINT('Ctrl Pts',(41.902301765201,41.6975401149299,49.8673024517636));
#22314=CARTESIAN_POINT('Ctrl Pts',(42.0134254443717,41.704230344215,49.8934319960916));
#22315=CARTESIAN_POINT('Ctrl Pts',(42.2104237760017,41.7162554282414,49.9216766110695));
#22316=CARTESIAN_POINT('Ctrl Pts',(42.2953332145075,41.7214877326998,49.9281655307091));
#22317=CARTESIAN_POINT('Ctrl Pts',(42.3980024058597,41.7280207752068,49.9292093980171));
#22318=CARTESIAN_POINT('Ctrl Pts',(42.4156189574747,41.7291488241351,49.9291471967907));
#22319=CARTESIAN_POINT('Ctrl Pts',(42.4433790754323,41.7309386364785,49.9286689223164));
#22320=CARTESIAN_POINT('Ctrl Pts',(42.4535247188529,41.7315953438571,49.928414025573));
#22321=CARTESIAN_POINT('Ctrl Pts',(42.4725316487446,41.7328306580704,49.9277863916251));
#22322=CARTESIAN_POINT('Ctrl Pts',(42.4813933261753,41.733408655195,49.927432575689));
#22323=CARTESIAN_POINT('Ctrl Pts',(42.5012469691224,41.7347083389644,49.9265027277153));
#22324=CARTESIAN_POINT('Ctrl Pts',(42.5122370050278,41.73543104391,49.9258937028818));
#22325=CARTESIAN_POINT('Ctrl Pts',(42.5402233859625,41.7372800051956,49.9241024460917));
#22326=CARTESIAN_POINT('Ctrl Pts',(42.5572100891708,41.7384103323653,49.9227890620355));
#22327=CARTESIAN_POINT('Ctrl Pts',(42.6982288167364,41.7478634839723,49.9100045898656));
#22328=CARTESIAN_POINT('Ctrl Pts',(42.8208768570923,41.7565618355221,49.8867723954869));
#22329=CARTESIAN_POINT('Ctrl Pts',(43.0318271865955,41.7722073235644,49.8252138952612));
#22330=CARTESIAN_POINT('Ctrl Pts',(43.1211447864983,41.7790559776539,49.7918041813452));
#22331=CARTESIAN_POINT('Ctrl Pts',(43.2384227365765,41.7881254672382,49.7377397642685));
#22332=CARTESIAN_POINT('Ctrl Pts',(43.26883669027,41.7904839659775,49.7227348174888));
#22333=CARTESIAN_POINT('Ctrl Pts',(43.3178977911307,41.7942820013022,49.6969001338608));
#22334=CARTESIAN_POINT('Ctrl Pts',(43.3367862114319,41.7957425890707,49.6865462072277));
#22335=CARTESIAN_POINT('Ctrl Pts',(43.3622027011903,41.7977017609218,49.6720550471824));
#22336=CARTESIAN_POINT('Ctrl Pts',(43.3688843342456,41.7982162052556,49.6681922163997));
#22337=CARTESIAN_POINT('Ctrl Pts',(43.3800233476619,41.7990726124423,49.6616629527363));
#22338=CARTESIAN_POINT('Ctrl Pts',(43.384493408753,41.7994159530059,49.6590184630073));
#22339=CARTESIAN_POINT('Ctrl Pts',(43.3929586098621,41.8000654414189,49.6539641842161));
#22340=CARTESIAN_POINT('Ctrl Pts',(43.3969557634222,41.8003718197589,49.6515579101284));
#22341=CARTESIAN_POINT('Ctrl Pts',(43.4064260216254,41.8010970873829,49.6458099344876));
#22342=CARTESIAN_POINT('Ctrl Pts',(43.4118913137847,41.8015151459244,49.6424553721232));
#22343=CARTESIAN_POINT('Ctrl Pts',(43.4311110535656,41.8029839575296,49.6305260676264));
#22344=CARTESIAN_POINT('Ctrl Pts',(43.4447745136464,41.8040256573163,49.6218050188767));
#22345=CARTESIAN_POINT('Ctrl Pts',(43.5537248026694,41.8123256765482,49.5503163099166));
#22346=CARTESIAN_POINT('Ctrl Pts',(43.6433946923034,41.8191258503394,49.4793709252952));
#22347=CARTESIAN_POINT('Ctrl Pts',(43.7984877666602,41.8318650744642,49.3325400174104));
#22348=CARTESIAN_POINT('Ctrl Pts',(43.8653027277568,41.8377842371834,49.2586965798393));
#22349=CARTESIAN_POINT('Ctrl Pts',(43.94777852791,41.8460834114385,49.1520318462068));
#22350=CARTESIAN_POINT('Ctrl Pts',(43.9686567313663,41.8482851215911,49.1234373955597));
#22351=CARTESIAN_POINT('Ctrl Pts',(44.0035385508157,41.8521593703719,49.072794337793));
#22352=CARTESIAN_POINT('Ctrl Pts',(44.0179032991913,41.853818482534,49.0510054165264));
#22353=CARTESIAN_POINT('Ctrl Pts',(44.0381333772114,41.8562539744058,49.0189218106444));
#22354=CARTESIAN_POINT('Ctrl Pts',(44.0443532482775,41.8570172244743,49.0088533106183));
#22355=CARTESIAN_POINT('Ctrl Pts',(44.0551207776517,41.8583646086331,48.9910590919031));
#22356=CARTESIAN_POINT('Ctrl Pts',(44.0597080036014,41.8589472710854,48.9833576411897));
#22357=CARTESIAN_POINT('Ctrl Pts',(44.06914117163,41.8601638001704,48.9672663413911));
#22358=CARTESIAN_POINT('Ctrl Pts',(44.0739779064899,41.8607979802326,48.9588714141048));
#22359=CARTESIAN_POINT('Ctrl Pts',(44.086388876947,41.8624529177927,48.9369500736254));
#22360=CARTESIAN_POINT('Ctrl Pts',(44.0938635393647,41.8634772124119,48.9233683830394));
#22361=CARTESIAN_POINT('Ctrl Pts',(44.124291827974,41.8677653012249,48.8664662294501));
#22362=CARTESIAN_POINT('Ctrl Pts',(44.1457518011165,41.8710809133144,48.8223721477913));
#22363=CARTESIAN_POINT('Ctrl Pts',(44.2214613400341,41.8839880979541,48.6504573694087));
#22364=CARTESIAN_POINT('Ctrl Pts',(44.2635300692004,41.8939493544161,48.5177471345995));
#22365=CARTESIAN_POINT('Ctrl Pts',(44.3066737159292,41.9094860842328,48.3040060300991));
#22366=CARTESIAN_POINT('Ctrl Pts',(44.3175545189683,41.9150857403102,48.2254142597761));
#22367=CARTESIAN_POINT('Ctrl Pts',(44.3248085884504,41.9215902287793,48.1300817375579));
#22368=CARTESIAN_POINT('Ctrl Pts',(44.3258410521265,41.9226923571831,48.1137789354332));
#22369=CARTESIAN_POINT('Ctrl Pts',(44.3270162125813,41.9242464773297,48.0905484675476));
#22370=CARTESIAN_POINT('Ctrl Pts',(44.3273288327098,41.9247072194103,48.0836306331353));
#22371=CARTESIAN_POINT('Ctrl Pts',(44.3278048813653,41.925500190321,48.0716684401934));
#22372=CARTESIAN_POINT('Ctrl Pts',(44.3279857758168,41.9258333746621,48.0666248949335));
#22373=CARTESIAN_POINT('Ctrl Pts',(44.3283245566772,41.9265316489924,48.0560173350611));
#22374=CARTESIAN_POINT('Ctrl Pts',(44.3284781575461,41.9268965004976,48.0504533004413));
#22375=CARTESIAN_POINT('Ctrl Pts',(44.3288268755569,41.9278753175095,48.0354708693569));
#22376=CARTESIAN_POINT('Ctrl Pts',(44.3289770942293,41.9284868386388,48.0260514337042));
#22377=CARTESIAN_POINT('Ctrl Pts',(44.3293485383783,41.9312678215677,47.9829670987715));
#22378=CARTESIAN_POINT('Ctrl Pts',(44.3287575336453,41.9333960796806,47.94929887603));
#22379=CARTESIAN_POINT('Ctrl Pts',(44.3220159834673,41.9429986843331,47.7952432363451));
#22380=CARTESIAN_POINT('Ctrl Pts',(44.3054719796454,41.950091208388,47.6755730656905));
#22381=CARTESIAN_POINT('Ctrl Pts',(44.2518821165112,41.9640796624603,47.4477794411589));
#22382=CARTESIAN_POINT('Ctrl Pts',(44.2162117644928,41.9709379025354,47.3398598828189));
#22383=CARTESIAN_POINT('Ctrl Pts',(44.1627972412724,41.9794763321761,47.2160702639712));
#22384=CARTESIAN_POINT('Ctrl Pts',(44.1539984997376,41.9808410967088,47.196576606338));
#22385=CARTESIAN_POINT('Ctrl Pts',(44.1402126263616,41.9829206450285,47.1673402744874));
#22386=CARTESIAN_POINT('Ctrl Pts',(44.1354635030115,41.9836272154368,47.1574867211703));
#22387=CARTESIAN_POINT('Ctrl Pts',(44.1267146682417,41.984911661889,47.1397223816314));
#22388=CARTESIAN_POINT('Ctrl Pts',(44.1227437142393,41.9854885201635,47.1317977097342));
#22389=CARTESIAN_POINT('Ctrl Pts',(44.1140865718742,41.9867332776627,47.1148142570634));
#22390=CARTESIAN_POINT('Ctrl Pts',(44.1093828934035,41.98740178081,47.1057647444193));
#22391=CARTESIAN_POINT('Ctrl Pts',(44.0964674395091,41.989216803376,47.0813906968972));
#22392=CARTESIAN_POINT('Ctrl Pts',(44.0881200586082,41.9903681100572,47.0661394863386));
#22393=CARTESIAN_POINT('Ctrl Pts',(44.0434765814393,41.9964164352621,46.9871278573033));
#22394=CARTESIAN_POINT('Ctrl Pts',(44.0037753157641,42.0014353123003,46.925370936773));
#22395=CARTESIAN_POINT('Ctrl Pts',(43.8830809660258,42.0157696292457,46.7592618070071));
#22396=CARTESIAN_POINT('Ctrl Pts',(43.7947538136503,42.0252994238503,46.6607400523754));
#22397=CARTESIAN_POINT('Ctrl Pts',(43.6639137946898,42.03781294897,46.5418945402952));
#22398=CARTESIAN_POINT('Ctrl Pts',(43.6297102446273,42.0409559573606,46.5129348183442));
#22399=CARTESIAN_POINT('Ctrl Pts',(43.5806774401909,42.0452557661766,46.4742692132599));
#22400=CARTESIAN_POINT('Ctrl Pts',(43.566677986607,42.0464611168152,46.4635377727867));
#22401=CARTESIAN_POINT('Ctrl Pts',(43.541957788275,42.0485482202678,46.4451209475018));
#22402=CARTESIAN_POINT('Ctrl Pts',(43.5313019226346,42.0494348106958,46.4373508258329));
#22403=CARTESIAN_POINT('Ctrl Pts',(43.5153953911154,42.050738032053,46.4259999869463));
#22404=CARTESIAN_POINT('Ctrl Pts',(43.5102056308366,42.0511600826889,46.4223351497442));
#22405=CARTESIAN_POINT('Ctrl Pts',(43.5013050926794,42.0518784170553,46.4161155521731));
#22406=CARTESIAN_POINT('Ctrl Pts',(43.4976033671385,42.0521755570466,46.4135480778687));
#22407=CARTESIAN_POINT('Ctrl Pts',(43.489187168632,42.0528474549226,46.4077542582658));
#22408=CARTESIAN_POINT('Ctrl Pts',(43.4844673352797,42.0532216732456,46.4045358696638));
#22409=CARTESIAN_POINT('Ctrl Pts',(43.4715888172863,42.0542359597282,46.3958377412963));
#22410=CARTESIAN_POINT('Ctrl Pts',(43.4634023091277,42.0548733326904,46.3903992158092));
#22411=CARTESIAN_POINT('Ctrl Pts',(43.4221460119354,42.0580505112439,46.3634436631518));
#22412=CARTESIAN_POINT('Ctrl Pts',(43.3884606940368,42.0605331228437,46.3428804893813));
#22413=CARTESIAN_POINT('Ctrl Pts',(43.3264174110082,42.0649523196356,46.3075719577956));
#22414=CARTESIAN_POINT('Ctrl Pts',(43.2982801390761,42.0669019562324,46.2924711253116));
#22415=CARTESIAN_POINT('Ctrl Pts',(43.1758613114292,42.0752072330507,46.2306348422674));
#22416=CARTESIAN_POINT('Ctrl Pts',(43.0782173102583,42.0813988720314,46.1909570717585));
#22417=CARTESIAN_POINT('Ctrl Pts',(42.9171319641701,42.0915557019867,46.1403862080576));
#22418=CARTESIAN_POINT('Ctrl Pts',(42.8555404200791,42.0954243164026,46.1243478742562));
#22419=CARTESIAN_POINT('Ctrl Pts',(42.7669448977293,42.1010518617757,46.1058993696022));
#22420=CARTESIAN_POINT('Ctrl Pts',(42.7405065386958,42.1027387539933,46.1009684183926));
#22421=CARTESIAN_POINT('Ctrl Pts',(42.6931748613807,42.1057779222193,46.0931608716059));
#22422=CARTESIAN_POINT('Ctrl Pts',(42.6723208948376,42.1071235273944,46.0900711439292));
#22423=CARTESIAN_POINT('Ctrl Pts',(42.6406373600095,42.1091797298192,46.0859063458874));
#22424=CARTESIAN_POINT('Ctrl Pts',(42.6298419925145,42.1098823952755,46.0845800705307));
#22425=CARTESIAN_POINT('Ctrl Pts',(42.6102333432009,42.111162713484,46.0823391853539));
#22426=CARTESIAN_POINT('Ctrl Pts',(42.6014238196071,42.1117393796737,46.0813938655603));
#22427=CARTESIAN_POINT('Ctrl Pts',(42.5824132868096,42.1129870884406,46.0794862841292));
#22428=CARTESIAN_POINT('Ctrl Pts',(42.5722105379181,42.113658760048,46.0785445454569));
#22429=CARTESIAN_POINT('Ctrl Pts',(42.5444693575738,42.1154908022985,46.0762066897057));
#22430=CARTESIAN_POINT('Ctrl Pts',(42.5269189042309,42.1166561124127,46.0749691813575));
#22431=CARTESIAN_POINT('Ctrl Pts',(42.4325784839858,42.1229554852961,46.0696127972839));
#22432=CARTESIAN_POINT('Ctrl Pts',(42.3556205371879,42.1282240791879,46.0698487447964));
#22433=CARTESIAN_POINT('Ctrl Pts',(42.1492547754344,42.1426873278712,46.0828298934952));
#22434=CARTESIAN_POINT('Ctrl Pts',(42.0207780564953,42.152068522268,46.1040567560623));
#22435=CARTESIAN_POINT('Ctrl Pts',(41.8332331090855,42.1658143695247,46.1548795119261));
#22436=CARTESIAN_POINT('Ctrl Pts',(41.7719181695772,42.1703107709796,46.1748399067633));
#22437=CARTESIAN_POINT('Ctrl Pts',(41.7015860372479,42.1753869644381,46.2017013676445));
#22438=CARTESIAN_POINT('Ctrl Pts',(41.6914931497129,42.1761133732053,46.2056538541874));
#22439=CARTESIAN_POINT('Ctrl Pts',(41.6759820780979,42.1772259990183,46.2118794461265));
#22440=CARTESIAN_POINT('Ctrl Pts',(41.6705402614033,42.177615630992,46.2140925112233));
#22441=CARTESIAN_POINT('Ctrl Pts',(41.6605013426352,42.1783329759775,46.2182286560142));
#22442=CARTESIAN_POINT('Ctrl Pts',(41.6559015905259,42.1786610842978,46.2201446844045));
#22443=CARTESIAN_POINT('Ctrl Pts',(41.6454165529065,42.1794077349973,46.2245599817978));
#22444=CARTESIAN_POINT('Ctrl Pts',(41.6395362303249,42.1798255786509,46.2270707022663));
#22445=CARTESIAN_POINT('Ctrl Pts',(41.6241509696908,42.1809167353337,46.2337303737719));
#22446=CARTESIAN_POINT('Ctrl Pts',(41.6146666665027,42.1815872832902,46.2379268808921));
#22447=CARTESIAN_POINT('Ctrl Pts',(41.5391454724107,42.1869134609174,46.2720735401987));
#22448=CARTESIAN_POINT('Ctrl Pts',(41.474803088873,42.1913709102639,46.3056524631706));
#22449=CARTESIAN_POINT('Ctrl Pts',(41.3149749064669,42.2026153057761,46.4008906360139));
#22450=CARTESIAN_POINT('Ctrl Pts',(41.2227715628433,42.2092828097478,46.4674973401075));
#22451=CARTESIAN_POINT('Ctrl Pts',(41.0731394476817,42.2212478096591,46.5971057254677));
#22452=CARTESIAN_POINT('Ctrl Pts',(41.0130251898619,42.2264422950811,46.6565084654121));
#22453=CARTESIAN_POINT('Ctrl Pts',(40.945328082262,42.2329327445638,46.7328057006051));
#22454=CARTESIAN_POINT('Ctrl Pts',(40.9338379386411,42.2340588076252,46.7461178055265));
#22455=CARTESIAN_POINT('Ctrl Pts',(40.9160104377474,42.2358461799329,46.7673522819909));
#22456=CARTESIAN_POINT('Ctrl Pts',(40.9095506574443,42.23650245671,46.7751709636296));
#22457=CARTESIAN_POINT('Ctrl Pts',(40.8975577628057,42.2377373921983,46.7899220898925));
#22458=CARTESIAN_POINT('Ctrl Pts',(40.8920102037896,42.2383154448917,46.7968424896431));
#22459=CARTESIAN_POINT('Ctrl Pts',(40.879679624264,42.2396158228637,46.8124437381098));
#22460=CARTESIAN_POINT('Ctrl Pts',(40.8729228903293,42.2403391712661,46.8211448720999));
#22461=CARTESIAN_POINT('Ctrl Pts',(40.8558882521919,42.2421908917947,46.8434738176695));
#22462=CARTESIAN_POINT('Ctrl Pts',(40.8457161927574,42.2433233556235,46.8571808040224));
#22463=CARTESIAN_POINT('Ctrl Pts',(40.76444525678,42.2525949042985,46.9697868261324));
#22464=CARTESIAN_POINT('Ctrl Pts',(40.702689985873,42.2610918800934,47.0750636232511));
#22465=CARTESIAN_POINT('Ctrl Pts',(40.6140074355371,42.27603628677,47.2654498846551));
#22466=CARTESIAN_POINT('Ctrl Pts',(40.5822731484203,42.2823799074249,47.3479243482902));
#22467=CARTESIAN_POINT('Ctrl Pts',(40.5388034807396,42.292804990859,47.4890951116254));
#22468=CARTESIAN_POINT('Ctrl Pts',(40.5239429427125,42.2969417156182,47.5466924834733));
#22469=CARTESIAN_POINT('Ctrl Pts',(40.5095847950574,42.3016666833414,47.6153101928554));
#22470=CARTESIAN_POINT('Ctrl Pts',(40.5074905880706,42.3023799760855,47.6257487030368));
#22471=CARTESIAN_POINT('Ctrl Pts',(40.5043828017806,42.3034768408688,47.6419329363921));
#22472=CARTESIAN_POINT('Ctrl Pts',(40.5033087288179,42.3038636815727,47.6476666233743));
#22473=CARTESIAN_POINT('Ctrl Pts',(40.5013645695192,42.3045785211562,47.6583116401143));
#22474=CARTESIAN_POINT('Ctrl Pts',(40.5004875242647,42.3049068920747,47.6632214547396));
#22475=CARTESIAN_POINT('Ctrl Pts',(40.4985197223067,42.3056575123142,47.6744897430042));
#22476=CARTESIAN_POINT('Ctrl Pts',(40.497441810224,42.30607903305,47.6808503308051));
#22477=CARTESIAN_POINT('Ctrl Pts',(40.4946829493129,42.3071862889506,47.6976407822273));
#22478=CARTESIAN_POINT('Ctrl Pts',(40.4930557040947,42.3078691252827,47.7080794207947));
#22479=CARTESIAN_POINT('Ctrl Pts',(40.4778536262782,42.3145619144477,47.8111563757288));
#22480=CARTESIAN_POINT('Ctrl Pts',(40.4709523081264,42.320239481112,47.9046666910671));
#22481=CARTESIAN_POINT('Ctrl Pts',(40.4707326658507,42.3353503593733,48.1568250863074));
#22482=CARTESIAN_POINT('Ctrl Pts',(40.4901284879639,42.3446521508147,48.3147276882422));
#22483=CARTESIAN_POINT('Ctrl Pts',(40.5355259498835,42.3563944593319,48.4960729318445));
#22484=CARTESIAN_POINT('Ctrl Pts',(40.5430435955585,42.3581988458114,48.5235118108636));
#22485=CARTESIAN_POINT('Ctrl Pts',(40.5544009834311,42.3607495104922,48.5616362721644));
#22486=CARTESIAN_POINT('Ctrl Pts',(40.5577326953223,42.3614793147686,48.5724702623754));
#22487=CARTESIAN_POINT('Ctrl Pts',(40.5636815291388,42.3627516018686,48.5912246631112));
#22488=CARTESIAN_POINT('Ctrl Pts',(40.5662549323146,42.3632926400475,48.599158703337));
#22489=CARTESIAN_POINT('Ctrl Pts',(40.5717318621456,42.3644251476594,48.6156787477004));
#22490=CARTESIAN_POINT('Ctrl Pts',(40.5746446015717,42.3650169101352,48.6242614588041));
#22491=CARTESIAN_POINT('Ctrl Pts',(40.581700850075,42.3664261751426,48.6445817986773));
#22492=CARTESIAN_POINT('Ctrl Pts',(40.5858976539058,42.3672454311106,48.6563003575406));
#22493=CARTESIAN_POINT('Ctrl Pts',(40.6004800506452,42.3700302379984,48.6958093563631));
#22494=CARTESIAN_POINT('Ctrl Pts',(40.6113927561166,42.3720132518584,48.7233993840596));
#22495=CARTESIAN_POINT('Ctrl Pts',(40.6579607594428,42.3800963704878,48.8336317904666));
#22496=CARTESIAN_POINT('Ctrl Pts',(40.6987387612596,42.3863641146625,48.9139742710991));
#22497=CARTESIAN_POINT('Ctrl Pts',(40.7891386014527,42.3988307694079,49.0649218736079));
#22498=CARTESIAN_POINT('Ctrl Pts',(40.8381884884264,42.4050056605702,49.135639605686));
#22499=CARTESIAN_POINT('Ctrl Pts',(40.9388159901847,42.4164724175829,49.2618130969654));
#22500=CARTESIAN_POINT('Ctrl Pts',(40.9892661233009,42.421768686245,49.3179770682951));
#22501=CARTESIAN_POINT('Ctrl Pts',(41.050287381502,42.4275654919543,49.3783783933363));
#22502=CARTESIAN_POINT('Ctrl Pts',(41.0577529283942,42.4282650383196,49.3856492912272));
#22503=CARTESIAN_POINT('Ctrl Pts',(41.0699043113111,42.429387651067,49.3972934858881));
#22504=CARTESIAN_POINT('Ctrl Pts',(41.0745535453387,42.4298134530209,49.4017044358679));
#22505=CARTESIAN_POINT('Ctrl Pts',(41.0828574677388,42.4305672475333,49.4095045040463));
#22506=CARTESIAN_POINT('Ctrl Pts',(41.0865033973776,42.4308959247206,49.4129027121736));
#22507=CARTESIAN_POINT('Ctrl Pts',(41.0944674049044,42.4316088995569,49.4202681373253));
#22508=CARTESIAN_POINT('Ctrl Pts',(41.0987904189152,42.4319927824082,49.4242298154117));
#22509=CARTESIAN_POINT('Ctrl Pts',(41.1111178473789,42.4330788263269,49.4354238845152));
#22510=CARTESIAN_POINT('Ctrl Pts',(41.1191651087773,42.4337775461156,49.442609069024));
#22511=CARTESIAN_POINT('Ctrl Pts',(41.1746484356022,42.4385289027755,49.4913183638746));
#22512=CARTESIAN_POINT('Ctrl Pts',(41.2240402379247,42.4424317002741,49.5305676509149));
#22513=CARTESIAN_POINT('Ctrl Pts',(41.3792013342771,42.4540417539977,49.641912464604));
#22514=CARTESIAN_POINT('Ctrl Pts',(41.4902937618086,42.4615218099984,49.7059728287113));
#22515=CARTESIAN_POINT('Ctrl Pts',(41.6680250795623,42.4733250684864,49.7861269607951));
#22516=CARTESIAN_POINT('Ctrl Pts',(41.7305183552398,42.4774429182762,49.8104771088016));
#22517=CARTESIAN_POINT('Ctrl Pts',(41.7941388473837,42.4816651137235,49.8315225416714));
#22518=CARTESIAN_POINT('Ctrl Pts',(41.7941387803776,42.6541583936299,49.831522519506));
#22519=CARTESIAN_POINT('Ctrl Pts',(41.7609009518026,42.652070389834,49.8205275624997));
#22520=CARTESIAN_POINT('Ctrl Pts',(41.7279586839609,42.6499820599924,49.8086265893831));
#22521=CARTESIAN_POINT('Ctrl Pts',(41.5956548730879,42.6414642847965,49.756713017299));
#22522=CARTESIAN_POINT('Ctrl Pts',(41.4994045378027,42.6349506160875,49.7093668430316));
#22523=CARTESIAN_POINT('Ctrl Pts',(41.3917602407269,42.6269721619504,49.6447904877291));
#22524=CARTESIAN_POINT('Ctrl Pts',(41.3760716721312,42.6257913447037,49.6350699991745));
#22525=CARTESIAN_POINT('Ctrl Pts',(41.3518254647877,42.6239368557057,49.6195614701564));
#22526=CARTESIAN_POINT('Ctrl Pts',(41.3431704957749,42.6232688847087,49.6139270751799));
#22527=CARTESIAN_POINT('Ctrl Pts',(41.3279215831576,42.6220811364806,49.6038247599118));
#22528=CARTESIAN_POINT('Ctrl Pts',(41.3213092349631,42.6215624262371,49.5993849513433));
#22529=CARTESIAN_POINT('Ctrl Pts',(41.3061330323522,42.6203633166099,49.589058088627));
#22530=CARTESIAN_POINT('Ctrl Pts',(41.2975889392358,42.6196818450353,49.5831425702874));
#22531=CARTESIAN_POINT('Ctrl Pts',(41.2741742783418,42.6177963749581,49.566649930126));
#22532=CARTESIAN_POINT('Ctrl Pts',(41.2594056709308,42.6165869435133,49.5559306207276));
#22533=CARTESIAN_POINT('Ctrl Pts',(41.1719468499182,42.6093006096093,49.4905371539673));
#22534=CARTESIAN_POINT('Ctrl Pts',(41.1030560339781,42.6030321492513,49.4309952944857));
#22535=CARTESIAN_POINT('Ctrl Pts',(40.9243428172365,42.5852678196432,49.2529952347166));
#22536=CARTESIAN_POINT('Ctrl Pts',(40.8247891827718,42.5735042162092,49.125287031941));
#22537=CARTESIAN_POINT('Ctrl Pts',(40.7342135112047,42.5613480654729,48.9731121728331));
#22538=CARTESIAN_POINT('Ctrl Pts',(40.7263033633215,42.5602717528433,48.9594433445829));
#22539=CARTESIAN_POINT('Ctrl Pts',(40.7126304185622,42.5583868133458,48.9351325300023));
#22540=CARTESIAN_POINT('Ctrl Pts',(40.7067983192092,42.5575744873042,48.9245307131735));
#22541=CARTESIAN_POINT('Ctrl Pts',(40.698159436616,42.5563592574608,48.9084706398389));
#22542=CARTESIAN_POINT('Ctrl Pts',(40.6952784460699,42.5559519130763,48.9030529512611));
#22543=CARTESIAN_POINT('Ctrl Pts',(40.6903375899028,42.5552498188499,48.8936537883733));
#22544=CARTESIAN_POINT('Ctrl Pts',(40.6882657150764,42.5549543223757,48.8896788123023));
#22545=CARTESIAN_POINT('Ctrl Pts',(40.6835125403024,42.5542738955873,48.8804815822695));
#22546=CARTESIAN_POINT('Ctrl Pts',(40.6808412092165,42.5538895931239,48.8752542889642));
#22547=CARTESIAN_POINT('Ctrl Pts',(40.6734469733955,42.5528202735524,48.8606206970058));
#22548=CARTESIAN_POINT('Ctrl Pts',(40.6687770405337,42.5521384591879,48.8511876494182));
#22549=CARTESIAN_POINT('Ctrl Pts',(40.6423176908154,42.5482347511193,48.7966223103786));
#22550=CARTESIAN_POINT('Ctrl Pts',(40.6222143640819,42.5451061107667,48.7506886160387));
#22551=CARTESIAN_POINT('Ctrl Pts',(40.5464705896604,42.5323775971079,48.5574529036845));
#22552=CARTESIAN_POINT('Ctrl Pts',(40.5071739215705,42.523264081888,48.4044011422224));
#22553=CARTESIAN_POINT('Ctrl Pts',(40.4783569354245,42.5095998207401,48.1823444814838));
#22554=CARTESIAN_POINT('Ctrl Pts',(40.4732158323177,42.5054724483302,48.1160297848249));
#22555=CARTESIAN_POINT('Ctrl Pts',(40.4710832469472,42.5001853991219,48.0330909520352));
#22556=CARTESIAN_POINT('Ctrl Pts',(40.4708707736736,42.4991275403952,48.0165907249398));
#22557=CARTESIAN_POINT('Ctrl Pts',(40.4708695389681,42.4974241211575,47.9901855699998));
#22558=CARTESIAN_POINT('Ctrl Pts',(40.470945355125,42.4967828133157,47.9802812344377));
#22559=CARTESIAN_POINT('Ctrl Pts',(40.4712341389415,42.4955605003437,47.9614763859268));
#22560=CARTESIAN_POINT('Ctrl Pts',(40.4714324580168,42.4949799707037,47.952575880103));
#22561=CARTESIAN_POINT('Ctrl Pts',(40.4720247824293,42.4936525711461,47.9322966418178));
#22562=CARTESIAN_POINT('Ctrl Pts',(40.472457926531,42.4929044917547,47.9209194726211));
#22563=CARTESIAN_POINT('Ctrl Pts',(40.4741019567423,42.4905908045723,47.8858950943901));
#22564=CARTESIAN_POINT('Ctrl Pts',(40.4756474802739,42.4890147993743,47.8622665721702));
#22565=CARTESIAN_POINT('Ctrl Pts',(40.4853499042818,42.481226002824,47.7466522358662));
#22566=CARTESIAN_POINT('Ctrl Pts',(40.4996684931085,42.4748238418407,47.6553177569385));
#22567=CARTESIAN_POINT('Ctrl Pts',(40.539991294348,42.4621705760943,47.4809439606581));
#22568=CARTESIAN_POINT('Ctrl Pts',(40.5651804567917,42.4559496928389,47.3979302582343));
#22569=CARTESIAN_POINT('Ctrl Pts',(40.624566617186,42.4440144985864,47.2410865388286));
#22570=CARTESIAN_POINT('Ctrl Pts',(40.6580232508475,42.4383062136994,47.1671534229146));
#22571=CARTESIAN_POINT('Ctrl Pts',(40.7009628580811,42.432121744993,47.0862572916244));
#22572=CARTESIAN_POINT('Ctrl Pts',(40.7059647171079,42.4314163326977,47.0770171079096));
#22573=CARTESIAN_POINT('Ctrl Pts',(40.7141505213841,42.4302862500226,47.0621857981093));
#22574=CARTESIAN_POINT('Ctrl Pts',(40.7172872978379,42.4298587858299,47.0565690768457));
#22575=CARTESIAN_POINT('Ctrl Pts',(40.7229043664715,42.4291032778905,47.04662827826));
#22576=CARTESIAN_POINT('Ctrl Pts',(40.7253733834617,42.4287745359542,47.0422980103479));
#22577=CARTESIAN_POINT('Ctrl Pts',(40.7307729155486,42.4280628452155,47.032912809011));
#22578=CARTESIAN_POINT('Ctrl Pts',(40.7337096233356,42.4276803002181,47.0278615955998));
#22579=CARTESIAN_POINT('Ctrl Pts',(40.7420866743934,42.4266015744032,47.013602339998));
#22580=CARTESIAN_POINT('Ctrl Pts',(40.7475808068098,42.4259087631971,47.0044259135753));
#22581=CARTESIAN_POINT('Ctrl Pts',(40.7847641284604,42.4213132502957,46.9434773406724));
#22582=CARTESIAN_POINT('Ctrl Pts',(40.8188087867542,42.4175493506,46.8931743555525));
#22583=CARTESIAN_POINT('Ctrl Pts',(40.9076216851214,42.4085210498048,46.7744316383732));
#22584=CARTESIAN_POINT('Ctrl Pts',(40.9647865687304,42.4033371474799,46.7079572147242));
#22585=CARTESIAN_POINT('Ctrl Pts',(41.1112991766687,42.3908706054489,46.5593544237548));
#22586=CARTESIAN_POINT('Ctrl Pts',(41.2042457298506,42.3835591401598,46.4813244026563));
#22587=CARTESIAN_POINT('Ctrl Pts',(41.3179479988541,42.3747828562728,46.4028155797908));
#22588=CARTESIAN_POINT('Ctrl Pts',(41.3321388572537,42.3736907149887,46.3932930711532));
#22589=CARTESIAN_POINT('Ctrl Pts',(41.3556863785254,42.371882624531,46.3779417147987));
#22590=CARTESIAN_POINT('Ctrl Pts',(41.3649700052253,42.3711708258873,46.3720021737815));
#22591=CARTESIAN_POINT('Ctrl Pts',(41.3818140566204,42.3698809555803,46.3614278858521));
#22592=CARTESIAN_POINT('Ctrl Pts',(41.3893565649688,42.369303944446,46.3567650711569));
#22593=CARTESIAN_POINT('Ctrl Pts',(41.4055867408465,42.3680633962687,46.3468855110679));
#22594=CARTESIAN_POINT('Ctrl Pts',(41.4142838715086,42.3673992892066,46.3416849060366));
#22595=CARTESIAN_POINT('Ctrl Pts',(41.4381575830003,42.3655778593715,46.3276633553057));
#22596=CARTESIAN_POINT('Ctrl Pts',(41.4534139192642,42.3644155741969,46.3189808313745));
#22597=CARTESIAN_POINT('Ctrl Pts',(41.5422434497142,42.3576559827849,46.2700197931112));
#22598=CARTESIAN_POINT('Ctrl Pts',(41.618252644225,42.3518965769761,46.2343711012668));
#22599=CARTESIAN_POINT('Ctrl Pts',(41.7998688851173,42.3382110845038,46.1632227855643));
#22600=CARTESIAN_POINT('Ctrl Pts',(41.9067166666116,42.3302089967473,46.1316914650072));
#22601=CARTESIAN_POINT('Ctrl Pts',(42.0895314665905,42.3169542758542,46.0945257791644));
#22602=CARTESIAN_POINT('Ctrl Pts',(42.1642129545515,42.3116620256094,46.0838502661021));
#22603=CARTESIAN_POINT('Ctrl Pts',(42.2497168103004,42.3058691639686,46.0767043780905));
#22604=CARTESIAN_POINT('Ctrl Pts',(42.2601055067152,42.3051698186053,46.0759208361231));
#22605=CARTESIAN_POINT('Ctrl Pts',(42.276892604627,42.3040475285068,46.0747913950961));
#22606=CARTESIAN_POINT('Ctrl Pts',(42.2832871085363,42.3036218496646,46.0743931587452));
#22607=CARTESIAN_POINT('Ctrl Pts',(42.2946579611768,42.3028682756267,46.0737418560076));
#22608=CARTESIAN_POINT('Ctrl Pts',(42.299633428302,42.3025396961623,46.0734762042283));
#22609=CARTESIAN_POINT('Ctrl Pts',(42.3104645530616,42.301826945031,46.0729399802209));
#22610=CARTESIAN_POINT('Ctrl Pts',(42.3163204405345,42.3014431878226,46.072676817534));
#22611=CARTESIAN_POINT('Ctrl Pts',(42.3329522985102,42.300357537789,46.0720053300256));
#22612=CARTESIAN_POINT('Ctrl Pts',(42.3437308243798,42.2996590834918,46.0716606536693));
#22613=CARTESIAN_POINT('Ctrl Pts',(42.4174842130787,42.294911352532,46.0699210979319));
#22614=CARTESIAN_POINT('Ctrl Pts',(42.4804987093173,42.2910116680776,46.0715208071771));
#22615=CARTESIAN_POINT('Ctrl Pts',(42.6708075327619,42.2794098195746,46.0856993526566));
#22616=CARTESIAN_POINT('Ctrl Pts',(42.7970290810384,42.2719348092528,46.1078441193079));
#22617=CARTESIAN_POINT('Ctrl Pts',(42.9526399110486,42.2621526387475,46.1514137792241));
#22618=CARTESIAN_POINT('Ctrl Pts',(42.9848982487448,42.2600942526379,46.1613657852326));
#22619=CARTESIAN_POINT('Ctrl Pts',(43.0649236823023,42.2548889816222,46.1883735540481));
#22620=CARTESIAN_POINT('Ctrl Pts',(43.1123078643337,42.2517164381873,46.2064753408143));
#22621=CARTESIAN_POINT('Ctrl Pts',(43.1733387324515,42.2474811853246,46.2325906841536));
#22622=CARTESIAN_POINT('Ctrl Pts',(43.1876802100688,42.2464749537834,46.2389354503562));
#22623=CARTESIAN_POINT('Ctrl Pts',(43.210788087629,42.2448349691112,46.2494972647144));
#22624=CARTESIAN_POINT('Ctrl Pts',(43.2196029295151,42.2442049142801,46.2536070941962));
#22625=CARTESIAN_POINT('Ctrl Pts',(43.236467552388,42.2429907151324,46.2616258561156));
#22626=CARTESIAN_POINT('Ctrl Pts',(43.2445219692226,42.2424069408119,46.2655244973582));
#22627=CARTESIAN_POINT('Ctrl Pts',(43.2630805255329,42.2410526852155,46.2746674524518));
#22628=CARTESIAN_POINT('Ctrl Pts',(43.2735644059398,42.2402808149916,46.2799518578051));
#22629=CARTESIAN_POINT('Ctrl Pts',(43.3067400483057,42.23781604646,46.2970555964997));
#22630=CARTESIAN_POINT('Ctrl Pts',(43.3292444192832,42.236110689375,46.3092303946116));
#22631=CARTESIAN_POINT('Ctrl Pts',(43.3815124347247,42.2320687610992,46.3388659641628));
#22632=CARTESIAN_POINT('Ctrl Pts',(43.4110621232873,42.2297200597884,46.3566844255384));
#22633=CARTESIAN_POINT('Ctrl Pts',(43.5201796878129,42.2208042032081,46.4265397405072));
#22634=CARTESIAN_POINT('Ctrl Pts',(43.5963361383991,42.2140736291461,46.4836372669162));
#22635=CARTESIAN_POINT('Ctrl Pts',(43.6770591482021,42.206428225723,46.5540373328247));
#22636=CARTESIAN_POINT('Ctrl Pts',(43.6860767837742,42.2055665345662,46.5620519453292));
#22637=CARTESIAN_POINT('Ctrl Pts',(43.7749316780139,42.197002525794,46.6425280732277));
#22638=CARTESIAN_POINT('Ctrl Pts',(43.8486441076355,42.189290989514,46.7214845249482));
#22639=CARTESIAN_POINT('Ctrl Pts',(43.9255149602306,42.1808349223287,46.8190618069945));
#22640=CARTESIAN_POINT('Ctrl Pts',(43.9354884323182,42.1797288973699,46.8320589794255));
#22641=CARTESIAN_POINT('Ctrl Pts',(43.9491508338691,42.1782029655587,46.8503410381966));
#22642=CARTESIAN_POINT('Ctrl Pts',(43.9529803510777,42.1777740331066,46.85551930264));
#22643=CARTESIAN_POINT('Ctrl Pts',(43.959542839346,42.1770370083119,46.8644866741722));
#22644=CARTESIAN_POINT('Ctrl Pts',(43.9622880816329,42.1767280855286,46.8682666692001));
#22645=CARTESIAN_POINT('Ctrl Pts',(43.9680503139702,42.1760784359588,46.8762617573903));
#22646=CARTESIAN_POINT('Ctrl Pts',(43.971064095289,42.1757379407688,46.8804791048579));
#22647=CARTESIAN_POINT('Ctrl Pts',(43.9784970661807,42.1748962507885,46.8909695906641));
#22648=CARTESIAN_POINT('Ctrl Pts',(43.9828959545468,42.1743964281027,46.8972571293659));
#22649=CARTESIAN_POINT('Ctrl Pts',(43.9993208984981,42.1725229850714,46.9210348744693));
#22650=CARTESIAN_POINT('Ctrl Pts',(44.0110960566988,42.1711652221737,46.9386976563516));
#22651=CARTESIAN_POINT('Ctrl Pts',(44.1016882124214,42.1605701136352,47.0795698752269));
#22652=CARTESIAN_POINT('Ctrl Pts',(44.166562512146,42.1520347784681,47.2112016237231));
#22653=CARTESIAN_POINT('Ctrl Pts',(44.2523591620418,42.1368059234787,47.4504973330234));
#22654=CARTESIAN_POINT('Ctrl Pts',(44.2801876586331,42.1302484117127,47.5549410539981));
#22655=CARTESIAN_POINT('Ctrl Pts',(44.3021296292297,42.1223131890977,47.6779201244869));
#22656=CARTESIAN_POINT('Ctrl Pts',(44.3048986555747,42.1212247858372,47.6947236416833));
#22657=CARTESIAN_POINT('Ctrl Pts',(44.3090899262524,42.119421615162,47.7224404999025));
#22658=CARTESIAN_POINT('Ctrl Pts',(44.3106419301598,42.1187109588467,47.7333334872246));
#22659=CARTESIAN_POINT('Ctrl Pts',(44.3132760897926,42.1174223132936,47.7530267858801));
#22660=CARTESIAN_POINT('Ctrl Pts',(44.3143909280882,42.1168453754762,47.7618224731361));
#22661=CARTESIAN_POINT('Ctrl Pts',(44.3166514757714,42.1156040463651,47.7806996946924));
#22662=CARTESIAN_POINT('Ctrl Pts',(44.3177783541332,42.1149390781362,47.7907831717692));
#22663=CARTESIAN_POINT('Ctrl Pts',(44.3206436294494,42.1131128394222,47.8183937738161));
#22664=CARTESIAN_POINT('Ctrl Pts',(44.3222215811193,42.1119465624861,47.8359361994197));
#22665=CARTESIAN_POINT('Ctrl Pts',(44.3300199215587,42.1051025662833,47.9383272623535));
#22666=CARTESIAN_POINT('Ctrl Pts',(44.3308613389443,42.099257844589,48.0234795864345));
#22667=CARTESIAN_POINT('Ctrl Pts',(44.319499291407,42.0850623748474,48.225364491383));
#22668=CARTESIAN_POINT('Ctrl Pts',(44.3022756720269,42.0766177001956,48.3414837930243));
#22669=CARTESIAN_POINT('Ctrl Pts',(44.2585218460129,42.0634782662563,48.52162854368));
#22670=CARTESIAN_POINT('Ctrl Pts',(44.2389054284624,42.0587033003943,48.5870508387798));
#22671=CARTESIAN_POINT('Ctrl Pts',(44.2123661714189,42.0533968537077,48.6610435092885));
#22672=CARTESIAN_POINT('Ctrl Pts',(44.2087937437583,42.0527021929845,48.6707569340298));
#22673=CARTESIAN_POINT('Ctrl Pts',(44.202890647127,42.0515859241476,48.6864172611924));
#22674=CARTESIAN_POINT('Ctrl Pts',(44.2006083686509,42.0511616276561,48.6923820098819));
#22675=CARTESIAN_POINT('Ctrl Pts',(44.1964933872782,42.0504095445521,48.7029785746101));
#22676=CARTESIAN_POINT('Ctrl Pts',(44.1946723249955,42.0500810844624,48.7076147360727));
#22677=CARTESIAN_POINT('Ctrl Pts',(44.1906635597271,42.0493674833538,48.7177054466541));
#22678=CARTESIAN_POINT('Ctrl Pts',(44.1884688806253,42.0489827651985,48.7231570767106));
#22679=CARTESIAN_POINT('Ctrl Pts',(44.1821499386006,42.0478916147088,48.7386487403222));
#22680=CARTESIAN_POINT('Ctrl Pts',(44.1779657295315,42.0471886761076,48.7486643060134));
#22681=CARTESIAN_POINT('Ctrl Pts',(44.1481655485945,42.0423126859851,48.8183366071522));
#22682=CARTESIAN_POINT('Ctrl Pts',(44.119633903019,42.0382986502641,48.8767090431292));
#22683=CARTESIAN_POINT('Ctrl Pts',(44.0251891504439,42.0264479031388,49.0475029895595));
#22684=CARTESIAN_POINT('Ctrl Pts',(43.950790536409,42.0188365505356,49.154795686159));
#22685=CARTESIAN_POINT('Ctrl Pts',(43.8166746619035,42.0063192085236,49.31162868257));
#22686=CARTESIAN_POINT('Ctrl Pts',(43.7638271258525,42.00161991698,49.3664956801145));
#22687=CARTESIAN_POINT('Ctrl Pts',(43.6949825788593,41.9956619456997,49.4299897075119));
#22688=CARTESIAN_POINT('Ctrl Pts',(43.6819227517177,41.9945385959975,49.4417088711395));
#22689=CARTESIAN_POINT('Ctrl Pts',(43.6609960437561,41.9927482405143,49.4599781716692));
#22690=CARTESIAN_POINT('Ctrl Pts',(43.6532335616526,41.9920861874737,49.4666468277555));
#22691=CARTESIAN_POINT('Ctrl Pts',(43.6386536138436,41.9908462753185,49.4789720245611));
#22692=CARTESIAN_POINT('Ctrl Pts',(43.6318495055318,41.9902690726206,49.4846440030623));
#22693=CARTESIAN_POINT('Ctrl Pts',(43.6165975935941,41.9889782647441,49.4971811328279));
#22694=CARTESIAN_POINT('Ctrl Pts',(43.6081303136521,41.9882637013066,49.5040220032294));
#22695=CARTESIAN_POINT('Ctrl Pts',(43.5830545021161,41.9861531993344,49.5239328266083));
#22696=CARTESIAN_POINT('Ctrl Pts',(43.5662890096734,41.9847493390159,49.5368015812861));
#22697=CARTESIAN_POINT('Ctrl Pts',(43.5276460181946,41.9815285913494,49.5654663822261));
#22698=CARTESIAN_POINT('Ctrl Pts',(43.505642122205,41.9797052513742,49.5810837773764));
#22699=CARTESIAN_POINT('Ctrl Pts',(43.4304131414429,41.9735054225005,49.6321395592134));
#22700=CARTESIAN_POINT('Ctrl Pts',(43.3757599899359,41.9690554288254,49.6653893990819));
#22701=CARTESIAN_POINT('Ctrl Pts',(43.2164183584837,41.9562666784319,49.7517905489689));
#22702=CARTESIAN_POINT('Ctrl Pts',(43.1083929651652,41.9477965963403,49.7981899265001));
#22703=CARTESIAN_POINT('Ctrl Pts',(42.942703813865,41.935510412296,49.8520945381106));
#22704=CARTESIAN_POINT('Ctrl Pts',(42.8878247836764,41.9315531232386,49.867300167906));
#22705=CARTESIAN_POINT('Ctrl Pts',(42.8226661425047,41.9270436084813,49.8822844083522));
#22706=CARTESIAN_POINT('Ctrl Pts',(42.8129665139945,41.9263771847094,49.8844362367873));
#22707=CARTESIAN_POINT('Ctrl Pts',(42.7971265585748,41.9252972850791,49.8878220967214));
#22708=CARTESIAN_POINT('Ctrl Pts',(42.790996226322,41.9248813895836,49.8891013011853));
#22709=CARTESIAN_POINT('Ctrl Pts',(42.779986111754,41.9241382353002,49.8913428689186));
#22710=CARTESIAN_POINT('Ctrl Pts',(42.775108752777,41.9238103689161,49.8923162310336));
#22711=CARTESIAN_POINT('Ctrl Pts',(42.7643635393785,41.9230910101079,49.8944174484557));
#22712=CARTESIAN_POINT('Ctrl Pts',(42.7584941849696,41.9226999948541,49.8955369106312));
#22713=CARTESIAN_POINT('Ctrl Pts',(42.7414907469936,41.9215725314157,49.8986981749699));
#22714=CARTESIAN_POINT('Ctrl Pts',(42.7303435468655,41.920839951727,49.9006693152455));
#22715=CARTESIAN_POINT('Ctrl Pts',(42.6386687406261,41.9148642360215,49.91604910605));
#22716=CARTESIAN_POINT('Ctrl Pts',(42.5573710276034,41.9098734741224,49.924433619399));
#22717=CARTESIAN_POINT('Ctrl Pts',(42.3504074242769,41.8974057694764,49.9325695346165));
#22718=CARTESIAN_POINT('Ctrl Pts',(42.2248590663551,41.8900454592222,49.925255854848));
#22719=CARTESIAN_POINT('Ctrl Pts',(42.0369512034123,41.8784335553712,49.8957662132446));
#22720=CARTESIAN_POINT('Ctrl Pts',(41.9735447531489,41.8744135933015,49.8825165486961));
#22721=CARTESIAN_POINT('Ctrl Pts',(41.894473350856,41.8692082285989,49.8617934204995));
#22722=CARTESIAN_POINT('Ctrl Pts',(41.8780762246925,41.86811827093,49.8572634375709));
#22723=CARTESIAN_POINT('Ctrl Pts',(41.8521236157303,41.8663753929775,49.8497227735046));
#22724=CARTESIAN_POINT('Ctrl Pts',(41.8425277329969,41.8657270858545,49.846853414999));
#22725=CARTESIAN_POINT('Ctrl Pts',(41.8253134753806,41.8645568828941,49.841559628887));
#22726=CARTESIAN_POINT('Ctrl Pts',(41.8176869532196,41.8640358880018,49.8391623040474));
#22727=CARTESIAN_POINT('Ctrl Pts',(41.8047558058709,41.8631480883241,49.83500902626));
#22728=CARTESIAN_POINT('Ctrl Pts',(41.7994434842431,41.8627820907004,49.8332772967566));
#22729=CARTESIAN_POINT('Ctrl Pts',(41.7941388317731,41.8624153300426,49.8315225365075));
#22730=CARTESIAN_POINT('Origin',(42.4,48.4493818343519,48.));
#22731=CARTESIAN_POINT('',(41.7941391176755,40.8966643233312,49.8315226310829));
#22732=CARTESIAN_POINT('',(41.7941388317924,41.0669118624314,49.8315225365138));
#22733=CARTESIAN_POINT('',(41.7941388317924,48.4493818343519,49.8315225365138));
#22734=CARTESIAN_POINT('',(40.4708703149926,41.5327745867846,48.0011024170354));
#22735=CARTESIAN_POINT('Ctrl Pts',(41.7941391176755,40.8966643233312,49.831522631083));
#22736=CARTESIAN_POINT('Ctrl Pts',(41.8581185305211,40.9014506186217,49.8526867831712));
#22737=CARTESIAN_POINT('Ctrl Pts',(41.923203389598,40.9061877965546,49.8704973808751));
#22738=CARTESIAN_POINT('Ctrl Pts',(42.0043953511471,40.9118383466694,49.88819586063));
#22739=CARTESIAN_POINT('Ctrl Pts',(42.0197007163529,40.912892311347,49.8913379230974));
#22740=CARTESIAN_POINT('Ctrl Pts',(42.0412423446147,40.9143584412164,49.8954881582493));
#22741=CARTESIAN_POINT('Ctrl Pts',(42.0474474720219,40.9147787593746,49.8966520848971));
#22742=CARTESIAN_POINT('Ctrl Pts',(42.0586772025161,40.9155356720216,49.8987014860313));
#22743=CARTESIAN_POINT('Ctrl Pts',(42.0636998085074,40.9158728519888,49.8995975280238));
#22744=CARTESIAN_POINT('Ctrl Pts',(42.0739835353635,40.9165603709582,49.9013900975472));
#22745=CARTESIAN_POINT('Ctrl Pts',(42.079244913191,40.9169106024865,49.9022847353325));
#22746=CARTESIAN_POINT('Ctrl Pts',(42.092780018769,40.9178078452656,49.9045284750944));
#22747=CARTESIAN_POINT('Ctrl Pts',(42.1010590553984,40.9183530743935,49.9058455203013));
#22748=CARTESIAN_POINT('Ctrl Pts',(42.1359511288381,40.9206368578791,49.9111632562143));
#22749=CARTESIAN_POINT('Ctrl Pts',(42.1626392193267,40.9223492231011,49.9146610232021));
#22750=CARTESIAN_POINT('Ctrl Pts',(42.2357217950739,40.9269659906813,49.9226875573822));
#22751=CARTESIAN_POINT('Ctrl Pts',(42.2822227046178,40.9298244628309,49.9260955001744));
#22752=CARTESIAN_POINT('Ctrl Pts',(42.4700533778608,40.9412117768441,49.9330322234343));
#22753=CARTESIAN_POINT('Ctrl Pts',(42.6114463742316,40.9494544976037,49.9227098379474));
#22754=CARTESIAN_POINT('Ctrl Pts',(42.8121119432309,40.9619279698461,49.8856401608799));
#22755=CARTESIAN_POINT('Ctrl Pts',(42.8731805425021,40.9658259841865,49.8712493211526));
#22756=CARTESIAN_POINT('Ctrl Pts',(42.9496175863159,40.9708922245715,49.8492556864682));
#22757=CARTESIAN_POINT('Ctrl Pts',(42.9657372610522,40.9719713043977,49.8443880848739));
#22758=CARTESIAN_POINT('Ctrl Pts',(42.9913060365639,40.9737009302023,49.8363004458457));
#22759=CARTESIAN_POINT('Ctrl Pts',(43.0007976710782,40.9743469874377,49.8332169289235));
#22760=CARTESIAN_POINT('Ctrl Pts',(43.0178563342052,40.9755154899954,49.8275284257964));
#22761=CARTESIAN_POINT('Ctrl Pts',(43.0254319380804,40.9760370549094,49.8249497210565));
#22762=CARTESIAN_POINT('Ctrl Pts',(43.0432203348745,40.9772680932921,49.8187708536315));
#22763=CARTESIAN_POINT('Ctrl Pts',(43.0534192064458,40.9779788494558,49.8151317169069));
#22764=CARTESIAN_POINT('Ctrl Pts',(43.0831602139729,40.9800662951778,49.804236463598));
#22765=CARTESIAN_POINT('Ctrl Pts',(43.1026155065284,40.9814506441943,49.7967494222345));
#22766=CARTESIAN_POINT('Ctrl Pts',(43.1465294381284,40.9846195150195,49.7790275937559));
#22767=CARTESIAN_POINT('Ctrl Pts',(43.1709056482116,40.986410195073,49.7686010704173));
#22768=CARTESIAN_POINT('Ctrl Pts',(43.2517696803878,40.9924585867652,49.7320234417323));
#22769=CARTESIAN_POINT('Ctrl Pts',(43.3072011634058,40.9967858856148,49.7036436128271));
#22770=CARTESIAN_POINT('Ctrl Pts',(43.4803451615369,41.0108606910713,49.6041485848714));
#22771=CARTESIAN_POINT('Ctrl Pts',(43.5918630127751,41.0208274688692,49.5231215463907));
#22772=CARTESIAN_POINT('Ctrl Pts',(43.7243233454903,41.0332954200884,49.4033535762986));
#22773=CARTESIAN_POINT('Ctrl Pts',(43.7539386987984,41.0361273786897,49.3748033143166));
#22774=CARTESIAN_POINT('Ctrl Pts',(43.7895630905453,41.0395664894806,49.3381913420326));
#22775=CARTESIAN_POINT('Ctrl Pts',(43.7964500152556,41.0402329148829,49.3310030112076));
#22776=CARTESIAN_POINT('Ctrl Pts',(43.8072210245297,41.0412772305618,49.3195849767576));
#22777=CARTESIAN_POINT('Ctrl Pts',(43.8111422805214,41.0416578542565,49.3153908122778));
#22778=CARTESIAN_POINT('Ctrl Pts',(43.8181033689359,41.0423342202955,49.307878297928));
#22779=CARTESIAN_POINT('Ctrl Pts',(43.8211503087269,41.0426304968696,49.3045668276438));
#22780=CARTESIAN_POINT('Ctrl Pts',(43.8284420233011,41.04334010751,49.2965861945416));
#22781=CARTESIAN_POINT('Ctrl Pts',(43.832675505979,41.0437525886897,49.2919068353246));
#22782=CARTESIAN_POINT('Ctrl Pts',(43.845537737919,41.0450076103139,49.2775489538392));
#22783=CARTESIAN_POINT('Ctrl Pts',(43.8540921455035,41.0458448219212,49.2678039026912));
#22784=CARTESIAN_POINT('Ctrl Pts',(43.873801695274,41.0477817810324,49.2448891337871));
#22785=CARTESIAN_POINT('Ctrl Pts',(43.884879813597,41.0488766397435,49.2316543250378));
#22786=CARTESIAN_POINT('Ctrl Pts',(43.9231571179139,41.0526888437998,49.1846579313957));
#22787=CARTESIAN_POINT('Ctrl Pts',(43.9493959824538,41.0553555861517,49.1501280838907));
#22788=CARTESIAN_POINT('Ctrl Pts',(44.0493472765207,41.0658638629027,49.0089577657068));
#22789=CARTESIAN_POINT('Ctrl Pts',(44.1133935866279,41.0734399193963,48.8958944141878));
#22790=CARTESIAN_POINT('Ctrl Pts',(44.1968236310758,41.0859918736241,48.7063750272404));
#22791=CARTESIAN_POINT('Ctrl Pts',(44.223727933227,41.0907699387044,48.6336837932964));
#22792=CARTESIAN_POINT('Ctrl Pts',(44.2513015484851,41.0968166850214,48.5427114806805));
#22793=CARTESIAN_POINT('Ctrl Pts',(44.256182282602,41.0979449192005,48.5257760696058));
#22794=CARTESIAN_POINT('Ctrl Pts',(44.2635342521272,41.0997414462192,48.498886533775));
#22795=CARTESIAN_POINT('Ctrl Pts',(44.2661593994532,41.100404729799,48.4889752258828));
#22796=CARTESIAN_POINT('Ctrl Pts',(44.2709054014978,41.1016459550314,48.4704615056965));
#22797=CARTESIAN_POINT('Ctrl Pts',(44.2730462525148,41.1022232311508,48.4618644619581));
#22798=CARTESIAN_POINT('Ctrl Pts',(44.2776811569261,41.1035129284537,48.4426896607373));
#22799=CARTESIAN_POINT('Ctrl Pts',(44.2801451807345,41.1042262978829,48.4321050265027));
#22800=CARTESIAN_POINT('Ctrl Pts',(44.2871160620178,41.1063291323712,48.4009714305734));
#22801=CARTESIAN_POINT('Ctrl Pts',(44.2913762546677,41.1077264298493,48.3803694560659));
#22802=CARTESIAN_POINT('Ctrl Pts',(44.3183048644127,41.1173929101452,48.2384807024407));
#22803=CARTESIAN_POINT('Ctrl Pts',(44.3296243489846,41.1260242166596,48.1153532461277));
#22804=CARTESIAN_POINT('Ctrl Pts',(44.3285528170195,41.144451865538,47.8566579616313));
#22805=CARTESIAN_POINT('Ctrl Pts',(44.3137490867992,41.154229566161,47.7217329695923));
#22806=CARTESIAN_POINT('Ctrl Pts',(44.2816824002445,41.1644655577599,47.5745022806212));
#22807=CARTESIAN_POINT('Ctrl Pts',(44.2782460980373,41.1654974604114,47.5595813400823));
#22808=CARTESIAN_POINT('Ctrl Pts',(44.2730570298807,41.1669656742092,47.5382159876295));
#22809=CARTESIAN_POINT('Ctrl Pts',(44.2714479892359,41.1674096107121,47.5317377464024));
#22810=CARTESIAN_POINT('Ctrl Pts',(44.2685682076344,41.1681845382193,47.5203952847873));
#22811=CARTESIAN_POINT('Ctrl Pts',(44.2673120298438,41.1685163476397,47.5155274878681));
#22812=CARTESIAN_POINT('Ctrl Pts',(44.2646088509248,41.1692173385357,47.5052191589439));
#22813=CARTESIAN_POINT('Ctrl Pts',(44.2631570554076,41.1695862419943,47.4997800118772));
#22814=CARTESIAN_POINT('Ctrl Pts',(44.2591368284411,41.170587677254,47.4849785865974));
#22815=CARTESIAN_POINT('Ctrl Pts',(44.2565214607171,41.1712175667514,47.4756290638882));
#22816=CARTESIAN_POINT('Ctrl Pts',(44.2422174246752,41.1745526281412,47.4259432795249));
#22817=CARTESIAN_POINT('Ctrl Pts',(44.2292836060134,41.177192140311,47.3859737400662));
#22818=CARTESIAN_POINT('Ctrl Pts',(44.1822462704462,41.1857721797249,47.2553395510333));
#22819=CARTESIAN_POINT('Ctrl Pts',(44.1426215129348,41.1915154249538,47.1668169402818));
#22820=CARTESIAN_POINT('Ctrl Pts',(44.0385611170396,41.2045567738288,46.974583264883));
#22821=CARTESIAN_POINT('Ctrl Pts',(43.9706136600271,41.2118576649052,46.8732658295929));
#22822=CARTESIAN_POINT('Ctrl Pts',(43.8773850802449,41.2211429881538,46.7592218104055));
#22823=CARTESIAN_POINT('Ctrl Pts',(43.8607996737614,41.2227702652929,46.7397375646306));
#22824=CARTESIAN_POINT('Ctrl Pts',(43.836128408382,41.2251593869539,46.7118957008343));
#22825=CARTESIAN_POINT('Ctrl Pts',(43.82834631145,41.2259086175819,46.7032716954816));
#22826=CARTESIAN_POINT('Ctrl Pts',(43.8144234679185,41.2272416987186,46.6881200062042));
#22827=CARTESIAN_POINT('Ctrl Pts',(43.8083141753005,41.2278242016569,46.6815637884909));
#22828=CARTESIAN_POINT('Ctrl Pts',(43.7954998634203,41.2290410956961,46.6680027366848));
#22829=CARTESIAN_POINT('Ctrl Pts',(43.7887872809272,41.2296758050924,46.6610054291406));
#22830=CARTESIAN_POINT('Ctrl Pts',(43.7711811586311,41.2313336740226,46.6429273286832));
#22831=CARTESIAN_POINT('Ctrl Pts',(43.7602061638159,41.2323603940855,46.6319272048614));
#22832=CARTESIAN_POINT('Ctrl Pts',(43.7100289143523,41.2370255737875,46.5828357503763));
#22833=CARTESIAN_POINT('Ctrl Pts',(43.669354814801,41.2407298862756,46.5462917728606));
#22834=CARTESIAN_POINT('Ctrl Pts',(43.4900258917407,41.2567547848277,46.3984421606042));
#22835=CARTESIAN_POINT('Ctrl Pts',(43.3379206332399,41.2697118963725,46.3048796378381));
#22836=CARTESIAN_POINT('Ctrl Pts',(43.1346935751145,41.2852412093358,46.2157011588096));
#22837=CARTESIAN_POINT('Ctrl Pts',(43.0936081709804,41.2882917906962,46.1993319572692));
#22838=CARTESIAN_POINT('Ctrl Pts',(43.0424234990391,41.2919547427511,46.1809513497059));
#22839=CARTESIAN_POINT('Ctrl Pts',(43.0328265866957,41.2926356826593,46.1775904778178));
#22840=CARTESIAN_POINT('Ctrl Pts',(43.0177234653792,41.2936976652191,46.1724350067101));
#22841=CARTESIAN_POINT('Ctrl Pts',(43.012235152103,41.294081590945,46.1705891098231));
#22842=CARTESIAN_POINT('Ctrl Pts',(43.0020434660126,41.2947907449261,46.1672123185203));
#22843=CARTESIAN_POINT('Ctrl Pts',(42.9973425390369,41.2951163419757,46.1656748074063));
#22844=CARTESIAN_POINT('Ctrl Pts',(42.9864618227649,41.295866556083,46.1621623644641));
#22845=CARTESIAN_POINT('Ctrl Pts',(42.9802779385651,41.2962904062305,46.1602005106044));
#22846=CARTESIAN_POINT('Ctrl Pts',(42.9608242969471,41.297616217463,46.1541366322295));
#22847=CARTESIAN_POINT('Ctrl Pts',(42.9475197156489,41.2985119382389,46.1501465862393));
#22848=CARTESIAN_POINT('Ctrl Pts',(42.8440925020433,41.3053983926774,46.1203424046129));
#22849=CARTESIAN_POINT('Ctrl Pts',(42.7522273592976,41.31106873742,46.1009814748822));
#22850=CARTESIAN_POINT('Ctrl Pts',(42.4968217993807,41.3264991902148,46.0663362243753));
#22851=CARTESIAN_POINT('Ctrl Pts',(42.332207857763,41.3361364094624,46.065102306466));
#22852=CARTESIAN_POINT('Ctrl Pts',(42.1465764946837,41.3479554843129,46.0874496862799));
#22853=CARTESIAN_POINT('Ctrl Pts',(42.1237798941795,41.3494220885553,46.0906088518849));
#22854=CARTESIAN_POINT('Ctrl Pts',(42.0899223361059,41.3516253703375,46.0959198598464));
#22855=CARTESIAN_POINT('Ctrl Pts',(42.0788143478763,41.3523522595083,46.0977620796102));
#22856=CARTESIAN_POINT('Ctrl Pts',(42.0589648606536,41.3536586949761,46.1012328614315));
#22857=CARTESIAN_POINT('Ctrl Pts',(42.0502172252744,41.3542370614802,46.1028248318007));
#22858=CARTESIAN_POINT('Ctrl Pts',(42.0316722542319,41.3554689142301,46.1063324255448));
#22859=CARTESIAN_POINT('Ctrl Pts',(42.0218781878226,41.3561228863688,46.1082637341229));
#22860=CARTESIAN_POINT('Ctrl Pts',(41.9955930169642,41.3578873778243,46.113659230078));
#22861=CARTESIAN_POINT('Ctrl Pts',(41.9791318959196,41.359002348794,46.117263556315));
#22862=CARTESIAN_POINT('Ctrl Pts',(41.8930448450856,41.3648872532325,46.137298554385));
#22863=CARTESIAN_POINT('Ctrl Pts',(41.8243335716497,41.3697732701749,46.1573751978238));
#22864=CARTESIAN_POINT('Ctrl Pts',(41.6699137041991,41.3811890255286,46.2119760490236));
#22865=CARTESIAN_POINT('Ctrl Pts',(41.5852498792528,41.387773256894,46.2489330625927));
#22866=CARTESIAN_POINT('Ctrl Pts',(41.415093985788,41.4015002727654,46.3382284333001));
#22867=CARTESIAN_POINT('Ctrl Pts',(41.3303572477324,41.4086237939684,46.3914624840049));
#22868=CARTESIAN_POINT('Ctrl Pts',(41.2368948554861,41.4165486229286,46.4608443045582));
#22869=CARTESIAN_POINT('Ctrl Pts',(41.2237958301023,41.4176607624129,46.4708310665137));
#22870=CARTESIAN_POINT('Ctrl Pts',(41.2057419707601,41.419193793046,46.4849646863879));
#22871=CARTESIAN_POINT('Ctrl Pts',(41.2006780681594,41.4196238140539,46.4889701695022));
#22872=CARTESIAN_POINT('Ctrl Pts',(41.1919810062191,41.4203622600533,46.495920700819));
#22873=CARTESIAN_POINT('Ctrl Pts',(41.1883383106288,41.4206715220936,46.4988536449626));
#22874=CARTESIAN_POINT('Ctrl Pts',(41.1807632224527,41.4213145134435,46.50499832273));
#22875=CARTESIAN_POINT('Ctrl Pts',(41.1768327823442,41.4216480613642,46.5082123832679));
#22876=CARTESIAN_POINT('Ctrl Pts',(41.1674556438012,41.4224437706635,46.51594237792));
#22877=CARTESIAN_POINT('Ctrl Pts',(41.1620209467042,41.4229048903603,46.5204728853126));
#22878=CARTESIAN_POINT('Ctrl Pts',(41.1501883291649,41.423909063726,46.5304477165828));
#22879=CARTESIAN_POINT('Ctrl Pts',(41.1438007628363,41.4244512776692,46.5359041668028));
#22880=CARTESIAN_POINT('Ctrl Pts',(41.1258977195987,41.4259720489525,46.551400904881));
#22881=CARTESIAN_POINT('Ctrl Pts',(41.1144653142055,41.426944420053,46.5615367356305));
#22882=CARTESIAN_POINT('Ctrl Pts',(41.0763782681241,41.4301929581844,46.5961210324591));
#22883=CARTESIAN_POINT('Ctrl Pts',(41.0502897676578,41.4324334434746,46.6211841124654));
#22884=CARTESIAN_POINT('Ctrl Pts',(40.9006183386253,41.4454902951244,46.7732944147));
#22885=CARTESIAN_POINT('Ctrl Pts',(40.7943164375551,41.4556954805726,46.9161463978581));
#22886=CARTESIAN_POINT('Ctrl Pts',(40.6868109816384,41.4695093578633,47.1119386162762));
#22887=CARTESIAN_POINT('Ctrl Pts',(40.666071766935,41.4724023354703,47.1531458276636));
#22888=CARTESIAN_POINT('Ctrl Pts',(40.6405024762728,41.4763149254304,47.2088356744813));
#22889=CARTESIAN_POINT('Ctrl Pts',(40.6343377382921,41.4772885326166,47.2226909995008));
#22890=CARTESIAN_POINT('Ctrl Pts',(40.6245322428981,41.4788886105219,47.2454476469767));
#22891=CARTESIAN_POINT('Ctrl Pts',(40.6207934893816,41.4795117182643,47.254306231116));
#22892=CARTESIAN_POINT('Ctrl Pts',(40.6136870707343,41.4807218870179,47.2715018748569));
#22893=CARTESIAN_POINT('Ctrl Pts',(40.6103111556473,41.4813086489769,47.2798352720588));
#22894=CARTESIAN_POINT('Ctrl Pts',(40.6025609293593,41.4826840591227,47.2993576739203));
#22895=CARTESIAN_POINT('Ctrl Pts',(40.5982326778415,41.4834742350113,47.3105644428771));
#22896=CARTESIAN_POINT('Ctrl Pts',(40.5844803926511,41.4860588425968,47.3471862190126));
#22897=CARTESIAN_POINT('Ctrl Pts',(40.5754876363461,41.4878675017102,47.3727585913714));
#22898=CARTESIAN_POINT('Ctrl Pts',(40.5554372704731,41.4922002267333,47.4338595767914));
#22899=CARTESIAN_POINT('Ctrl Pts',(40.5448632185349,41.4947389220043,47.4695343048505));
#22900=CARTESIAN_POINT('Ctrl Pts',(40.4924363865387,41.5088548081407,47.667222849361));
#22901=CARTESIAN_POINT('Ctrl Pts',(40.4707747286394,41.5210116021514,47.8338349804454));
#22902=CARTESIAN_POINT('Ctrl Pts',(40.4708703149926,41.5327745867846,48.0011024170354));
#22903=CARTESIAN_POINT('Ctrl Pts',(40.4708703166185,41.5327747866074,48.0011052584796));
#22904=CARTESIAN_POINT('Ctrl Pts',(40.4708910356162,41.5353179380368,48.0372684133744));
#22905=CARTESIAN_POINT('Ctrl Pts',(40.4719286180371,41.5378363427205,48.0734265716021));
#22906=CARTESIAN_POINT('Ctrl Pts',(40.4750553011039,41.5416089606166,48.1284040113603));
#22907=CARTESIAN_POINT('Ctrl Pts',(40.476405553459,41.5428923869818,48.1472554005316));
#22908=CARTESIAN_POINT('Ctrl Pts',(40.478611137742,41.5446135884969,48.1727788857062));
#22909=CARTESIAN_POINT('Ctrl Pts',(40.4792245864809,41.5450632790307,48.1794701016799));
#22910=CARTESIAN_POINT('Ctrl Pts',(40.4803556963078,41.5458445185021,48.1911369299981));
#22911=CARTESIAN_POINT('Ctrl Pts',(40.480857768946,41.5461768877265,48.1961139390409));
#22912=CARTESIAN_POINT('Ctrl Pts',(40.4818771242539,41.5468245464197,48.2058397630237));
#22913=CARTESIAN_POINT('Ctrl Pts',(40.4823926986165,41.5471399266619,48.2105887324994));
#22914=CARTESIAN_POINT('Ctrl Pts',(40.4835409100536,41.5478168761997,48.2208109325732));
#22915=CARTESIAN_POINT('Ctrl Pts',(40.4841793590307,41.5481781164396,48.2262834172197));
#22916=CARTESIAN_POINT('Ctrl Pts',(40.4859422200879,41.5491368194173,48.2408513244274));
#22917=CARTESIAN_POINT('Ctrl Pts',(40.4871080312627,41.5497320084403,48.2499417320189));
#22918=CARTESIAN_POINT('Ctrl Pts',(40.4925113790291,41.5523309932763,48.2898198245944));
#22919=CARTESIAN_POINT('Ctrl Pts',(40.4974279965344,41.5542998855106,48.3205127176437));
#22920=CARTESIAN_POINT('Ctrl Pts',(40.5108502723839,41.558905790742,48.3930353809672));
#22921=CARTESIAN_POINT('Ctrl Pts',(40.520006677116,41.5615169095456,48.4347286998954));
#22922=CARTESIAN_POINT('Ctrl Pts',(40.5590234336272,41.5710860523173,48.5879368617066));
#22923=CARTESIAN_POINT('Ctrl Pts',(40.5974884784632,41.5778605429286,48.6970064100749));
#22924=CARTESIAN_POINT('Ctrl Pts',(40.6809573254201,41.5899908299084,48.8796135899817));
#22925=CARTESIAN_POINT('Ctrl Pts',(40.7215493280278,41.5952395868679,48.9547923400153));
#22926=CARTESIAN_POINT('Ctrl Pts',(40.7763672505195,41.6017911588872,49.041954925123));
#22927=CARTESIAN_POINT('Ctrl Pts',(40.7859569548367,41.6029200635117,49.056748970379));
#22928=CARTESIAN_POINT('Ctrl Pts',(40.8013859716145,41.604710927223,49.0798512879276));
#22929=CARTESIAN_POINT('Ctrl Pts',(40.8070905800947,41.6053678201035,49.0882486798621));
#22930=CARTESIAN_POINT('Ctrl Pts',(40.8179023232201,41.6066032978008,49.1038968011063));
#22931=CARTESIAN_POINT('Ctrl Pts',(40.8229937142394,41.6071812713189,49.1111581240335));
#22932=CARTESIAN_POINT('Ctrl Pts',(40.8345136167881,41.608480657631,49.127349103891));
#22933=CARTESIAN_POINT('Ctrl Pts',(40.8409687788145,41.6092030866577,49.1362593281865));
#22934=CARTESIAN_POINT('Ctrl Pts',(40.8576047341472,41.6110508650984,49.1588137050245));
#22935=CARTESIAN_POINT('Ctrl Pts',(40.8678903846456,41.6121802764086,49.1723789719563));
#22936=CARTESIAN_POINT('Ctrl Pts',(40.9525487989169,41.6213748629403,49.2810140649258));
#22937=CARTESIAN_POINT('Ctrl Pts',(41.035501606412,41.6297911433942,49.3690312177839));
#22938=CARTESIAN_POINT('Ctrl Pts',(41.1910658328288,41.6445268695145,49.5058223536642));
#22939=CARTESIAN_POINT('Ctrl Pts',(41.2597825688829,41.6507416859,49.5585015669848));
#22940=CARTESIAN_POINT('Ctrl Pts',(41.3667885169207,41.65982324221,49.6296569783237));
#22941=CARTESIAN_POINT('Ctrl Pts',(41.4025277725476,41.662764962641,49.6517740303494));
#22942=CARTESIAN_POINT('Ctrl Pts',(41.4536177261703,41.6668173151942,49.6811272415018));
#22943=CARTESIAN_POINT('Ctrl Pts',(41.4683830515961,41.6679711354929,49.6893543485922));
#22944=CARTESIAN_POINT('Ctrl Pts',(41.4943892194213,41.669970843268,49.7034000704587));
#22945=CARTESIAN_POINT('Ctrl Pts',(41.5055825652418,41.6708211911854,49.7093039984893));
#22946=CARTESIAN_POINT('Ctrl Pts',(41.5223645603684,41.6720798508136,49.717945661478));
#22947=CARTESIAN_POINT('Ctrl Pts',(41.5279094069499,41.6724930975791,49.7207670559632));
#22948=CARTESIAN_POINT('Ctrl Pts',(41.5334875835222,41.6729061325938,49.7235715214273));
#22949=CARTESIAN_POINT('Ctrl Pts',(41.5335072653789,41.6729075898995,49.7235814161896));
#22950=CARTESIAN_POINT('Ctrl Pts',(41.5335468125291,41.6729105180257,49.7236012970858));
#22951=CARTESIAN_POINT('Ctrl Pts',(41.5335666780665,41.6729119888635,49.7236112833344));
#22952=CARTESIAN_POINT('Ctrl Pts',(41.5336065939171,41.6729149441512,49.7236313478524));
#22953=CARTESIAN_POINT('Ctrl Pts',(41.5336266451778,41.6729164286705,49.7236414265902));
#22954=CARTESIAN_POINT('Ctrl Pts',(41.5336669357823,41.672919411564,49.7236616777246));
#22955=CARTESIAN_POINT('Ctrl Pts',(41.5336871741521,41.6729209098655,49.7236718496235));
#22956=CARTESIAN_POINT('Ctrl Pts',(41.5337278412036,41.6729239204862,49.7236922881759));
#22957=CARTESIAN_POINT('Ctrl Pts',(41.533748269972,41.6729254328113,49.7237025548645));
#22958=CARTESIAN_POINT('Ctrl Pts',(41.5337893193495,41.6729284715906,49.7237231837391));
#22959=CARTESIAN_POINT('Ctrl Pts',(41.533809940713,41.6729299980999,49.7237335462957));
#22960=CARTESIAN_POINT('Ctrl Pts',(41.5338513778411,41.6729330654351,49.723754368167));
#22961=CARTESIAN_POINT('Ctrl Pts',(41.5338721937306,41.6729346062695,49.7237648275358));
#22962=CARTESIAN_POINT('Ctrl Pts',(41.5339140228206,41.6729377024681,49.7237858444674));
#22963=CARTESIAN_POINT('Ctrl Pts',(41.5339350356898,41.6729392578071,49.7237964018547));
#22964=CARTESIAN_POINT('Ctrl Pts',(41.5339772614457,41.672942383213,49.7238176161562));
#22965=CARTESIAN_POINT('Ctrl Pts',(41.5339984738186,41.6729439532413,49.723828272803));
#22966=CARTESIAN_POINT('Ctrl Pts',(41.5340411007461,41.6729471081837,49.7238496866831));
#22967=CARTESIAN_POINT('Ctrl Pts',(41.5340625153346,41.6729486930996,49.723860443924));
#22968=CARTESIAN_POINT('Ctrl Pts',(41.5341055489994,41.6729518779859,49.7238820601223));
#22969=CARTESIAN_POINT('Ctrl Pts',(41.5341271681326,41.6729534779596,49.7238929190989));
#22970=CARTESIAN_POINT('Ctrl Pts',(41.5341706132983,41.6729566931377,49.723914739951));
#22971=CARTESIAN_POINT('Ctrl Pts',(41.5341924395709,41.6729583083591,49.7239257019374));
#22972=CARTESIAN_POINT('Ctrl Pts',(41.5342363020941,41.6729615542578,49.7239477303261));
#22973=CARTESIAN_POINT('Ctrl Pts',(41.5342583377425,41.6729631848898,49.7239587964159));
#22974=CARTESIAN_POINT('Ctrl Pts',(41.5343026215585,41.6729664617954,49.7239810342574));
#22975=CARTESIAN_POINT('Ctrl Pts',(41.5343248696589,41.6729681080633,49.7239922059652));
#22976=CARTESIAN_POINT('Ctrl Pts',(41.5343695800479,41.6729714163618,49.7240146558499));
#22977=CARTESIAN_POINT('Ctrl Pts',(41.5343920434813,41.6729730784763,49.7240259345913));
#22978=CARTESIAN_POINT('Ctrl Pts',(41.5344371881827,41.6729764187352,49.7240486003426));
#22979=CARTESIAN_POINT('Ctrl Pts',(41.5344598685596,41.6729780968129,49.7240599868944));
#22980=CARTESIAN_POINT('Ctrl Pts',(41.5345054497366,41.6729814691872,49.7240828695341));
#22981=CARTESIAN_POINT('Ctrl Pts',(41.5345283508829,41.6729831635086,49.7240943657849));
#22982=CARTESIAN_POINT('Ctrl Pts',(41.5345743761216,41.6729865685544,49.724117469056));
#22983=CARTESIAN_POINT('Ctrl Pts',(41.5345975003172,41.6729882792855,49.724129076117));
#22984=CARTESIAN_POINT('Ctrl Pts',(41.5346439747086,41.672991717374,49.7241524025081));
#22985=CARTESIAN_POINT('Ctrl Pts',(41.5346673247705,41.6729934447205,49.7241641217595));
#22986=CARTESIAN_POINT('Ctrl Pts',(41.5347142538249,41.6729969162538,49.7241876739677));
#22987=CARTESIAN_POINT('Ctrl Pts',(41.5347378326906,41.6729986604303,49.7241995068492));
#22988=CARTESIAN_POINT('Ctrl Pts',(41.5347852222905,41.6730021658381,49.7242232877568));
#22989=CARTESIAN_POINT('Ctrl Pts',(41.5348090328349,41.6730039270543,49.7242352356757));
#22990=CARTESIAN_POINT('Ctrl Pts',(41.5348568884404,41.6730074667347,49.724259247951));
#22991=CARTESIAN_POINT('Ctrl Pts',(41.5348809337817,41.6730092452185,49.7242713124359));
#22992=CARTESIAN_POINT('Ctrl Pts',(41.5349292620101,41.673012819655,49.7242955593261));
#22993=CARTESIAN_POINT('Ctrl Pts',(41.5349535448745,41.673014615605,49.7243077417076));
#22994=CARTESIAN_POINT('Ctrl Pts',(41.5350023515116,41.6730182252196,49.7243322260406));
#22995=CARTESIAN_POINT('Ctrl Pts',(41.53502687491,41.6730200388554,49.7243445277916));
#22996=CARTESIAN_POINT('Ctrl Pts',(41.5350761650012,41.6730236840151,49.7243692520219));
#22997=CARTESIAN_POINT('Ctrl Pts',(41.5351009325253,41.6730255155994,49.7243816749053));
#22998=CARTESIAN_POINT('Ctrl Pts',(41.5351507143927,41.6730291969133,49.7244066431291));
#22999=CARTESIAN_POINT('Ctrl Pts',(41.5351757283507,41.6730310466135,49.7244191882629));
#23000=CARTESIAN_POINT('Ctrl Pts',(41.5352260064123,41.6730347644021,49.7244444026158));
#23001=CARTESIAN_POINT('Ctrl Pts',(41.5352512704939,41.6730366324878,49.7244570718102));
#23002=CARTESIAN_POINT('Ctrl Pts',(41.5353020520409,41.6730403872835,49.724482535867));
#23003=CARTESIAN_POINT('Ctrl Pts',(41.5353275692568,41.6730422739739,49.7244953305902));
#23004=CARTESIAN_POINT('Ctrl Pts',(41.5353788602599,41.6730460662116,49.7245210472609));
#23005=CARTESIAN_POINT('Ctrl Pts',(41.5354046340135,41.6730479717551,49.7245339691771));
#23006=CARTESIAN_POINT('Ctrl Pts',(41.535456440713,41.6730518018892,49.7245599415049));
#23007=CARTESIAN_POINT('Ctrl Pts',(41.5354824745391,41.6730537265436,49.7245729923431));
#23008=CARTESIAN_POINT('Ctrl Pts',(41.5355348054584,41.6730575951972,49.7245992245132));
#23009=CARTESIAN_POINT('Ctrl Pts',(41.5355611018867,41.6730595391461,49.7246124054969));
#23010=CARTESIAN_POINT('Ctrl Pts',(41.5356139616158,41.6730634466514,49.7246388997205));
#23011=CARTESIAN_POINT('Ctrl Pts',(41.5356405247149,41.6730654101917,49.724652212844));
#23012=CARTESIAN_POINT('Ctrl Pts',(41.5356939207531,41.6730693570957,49.7246789727882));
#23013=CARTESIAN_POINT('Ctrl Pts',(41.5357207539793,41.6730713404794,49.7246924197372));
#23014=CARTESIAN_POINT('Ctrl Pts',(41.5357746940368,41.6730753273444,49.724719449172));
#23015=CARTESIAN_POINT('Ctrl Pts',(41.5358018005083,41.673077330798,49.7247330314615));
#23016=CARTESIAN_POINT('Ctrl Pts',(41.5358562899825,41.6730813580154,49.7247603329956));
#23017=CARTESIAN_POINT('Ctrl Pts',(41.5358836738819,41.6730833818442,49.7247740526731));
#23018=CARTESIAN_POINT('Ctrl Pts',(41.5359387223972,41.6730874501173,49.7248016310303));
#23019=CARTESIAN_POINT('Ctrl Pts',(41.5359663863995,41.673089494515,49.724815489386));
#23020=CARTESIAN_POINT('Ctrl Pts',(41.5360219987301,41.6730936041886,49.7248433468575));
#23021=CARTESIAN_POINT('Ctrl Pts',(41.5360499472611,41.6730956694782,49.7248573460578));
#23022=CARTESIAN_POINT('Ctrl Pts',(41.5405326392237,41.6734269123859,49.7271025550605));
#23023=CARTESIAN_POINT('Ctrl Pts',(41.5449959295021,41.6737549844919,49.7293164604325));
#23024=CARTESIAN_POINT('Ctrl Pts',(41.5551987785285,41.6745010294112,49.7343281755207));
#23025=CARTESIAN_POINT('Ctrl Pts',(41.5609436864827,41.6749183080931,49.7371148004176));
#23026=CARTESIAN_POINT('Ctrl Pts',(41.5760290881034,41.6760069979231,49.7443398273652));
#23027=CARTESIAN_POINT('Ctrl Pts',(41.5853917653395,41.6766756642317,49.7487318068621));
#23028=CARTESIAN_POINT('Ctrl Pts',(41.6582624608841,41.6818291769998,49.7822027853363));
#23029=CARTESIAN_POINT('Ctrl Pts',(41.7232797262281,41.6861303680353,49.8078919529853));
#23030=CARTESIAN_POINT('Ctrl Pts',(41.7910819634347,41.690456096612,49.8305092118532));
#23031=CARTESIAN_POINT('Ctrl Pts',(41.7926101020481,41.6905535087766,49.8310168381293));
#23032=CARTESIAN_POINT('Ctrl Pts',(41.7941388322699,41.6906508784004,49.8315225366718));
#23033=CARTESIAN_POINT('',(40.4708708172652,41.7025068343519,47.9982242689299));
#23034=CARTESIAN_POINT('Ctrl Pts',(41.7941388317731,41.8624153300426,49.8315225365075));
#23035=CARTESIAN_POINT('Ctrl Pts',(41.7892186830212,41.8620751537533,49.8298949687264));
#23036=CARTESIAN_POINT('Ctrl Pts',(41.7843051319335,41.8617343210511,49.8282475879286));
#23037=CARTESIAN_POINT('Ctrl Pts',(41.7599237344004,41.8600374975222,49.8199637278008));
#23038=CARTESIAN_POINT('Ctrl Pts',(41.7405569098558,41.8586719070556,49.8130362244661));
#23039=CARTESIAN_POINT('Ctrl Pts',(41.6969070890574,41.855552516025,49.7966308099455));
#23040=CARTESIAN_POINT('Ctrl Pts',(41.6726984071991,41.8537928278026,49.786967876266));
#23041=CARTESIAN_POINT('Ctrl Pts',(41.5928156839767,41.8478857162481,49.7531904243072));
#23042=CARTESIAN_POINT('Ctrl Pts',(41.5380881659186,41.8436722457972,49.7269423780626));
#23043=CARTESIAN_POINT('Ctrl Pts',(41.3555549628571,41.8290720271415,49.6285571541991));
#23044=CARTESIAN_POINT('Ctrl Pts',(41.2347856430922,41.818412713764,49.5444537451597));
#23045=CARTESIAN_POINT('Ctrl Pts',(41.0982253084333,41.8057648919477,49.4241389510254));
#23046=CARTESIAN_POINT('Ctrl Pts',(41.072377611227,41.8033430665789,49.4000743799898));
#23047=CARTESIAN_POINT('Ctrl Pts',(41.0403811485847,41.8003246672332,49.3686017337567));
#23048=CARTESIAN_POINT('Ctrl Pts',(41.0336089283717,41.7996845996916,49.3618405102973));
#23049=CARTESIAN_POINT('Ctrl Pts',(41.0229551610083,41.7986761590713,49.3510445605028));
#23050=CARTESIAN_POINT('Ctrl Pts',(41.019040491923,41.7983052838696,49.3470429585196));
#23051=CARTESIAN_POINT('Ctrl Pts',(41.0116383365694,41.797603477322,49.3394102411973));
#23052=CARTESIAN_POINT('Ctrl Pts',(41.008147674562,41.7972723109,49.3357825449606));
#23053=CARTESIAN_POINT('Ctrl Pts',(40.9999402297618,41.7964930593378,49.3271857945718));
#23054=CARTESIAN_POINT('Ctrl Pts',(40.9952356605449,41.7960459109071,49.3222052214658));
#23055=CARTESIAN_POINT('Ctrl Pts',(40.9801341754675,41.794608617292,49.3060461876689));
#23056=CARTESIAN_POINT('Ctrl Pts',(40.9698430787115,41.7936261167636,49.2947690217377));
#23057=CARTESIAN_POINT('Ctrl Pts',(40.9055841622379,41.7874626740857,49.2226519016328));
#23058=CARTESIAN_POINT('Ctrl Pts',(40.8553686886246,41.7825146099197,49.1585653325076));
#23059=CARTESIAN_POINT('Ctrl Pts',(40.7633702271068,41.7727499424644,49.0244940229064));
#23060=CARTESIAN_POINT('Ctrl Pts',(40.7216750842606,41.767941930125,48.9546573638967));
#23061=CARTESIAN_POINT('Ctrl Pts',(40.6389408014605,41.7570796979552,48.7938117786158));
#23062=CARTESIAN_POINT('Ctrl Pts',(40.6003099179131,41.7510014937008,48.7018393035765));
#23063=CARTESIAN_POINT('Ctrl Pts',(40.5636316196754,41.7435992833381,48.5912526374627));
#23064=CARTESIAN_POINT('Ctrl Pts',(40.5585196052753,41.7425183919732,48.5751334074503));
#23065=CARTESIAN_POINT('Ctrl Pts',(40.5504427930779,41.7407251104298,48.5484532451553));
#23066=CARTESIAN_POINT('Ctrl Pts',(40.5473549196674,41.7400167526098,48.5379303132434));
#23067=CARTESIAN_POINT('Ctrl Pts',(40.5419339151009,41.7387305630651,48.5188559932604));
#23068=CARTESIAN_POINT('Ctrl Pts',(40.5395696648142,41.7381537644266,48.5103137085197));
#23069=CARTESIAN_POINT('Ctrl Pts',(40.5346185808692,41.7369108238037,48.4919331240307));
#23070=CARTESIAN_POINT('Ctrl Pts',(40.5320505412383,41.7362440907617,48.4820900850759));
#23071=CARTESIAN_POINT('Ctrl Pts',(40.526958307188,41.7348753964956,48.4619203181699));
#23072=CARTESIAN_POINT('Ctrl Pts',(40.5244413888776,41.734173225229,48.4515921299839));
#23073=CARTESIAN_POINT('Ctrl Pts',(40.5182996512163,41.7323925617641,48.4254521121162));
#23074=CARTESIAN_POINT('Ctrl Pts',(40.5147887323197,41.7313104746275,48.4096146373933));
#23075=CARTESIAN_POINT('Ctrl Pts',(40.4843509256643,41.7213041594941,48.2636219241579));
#23076=CARTESIAN_POINT('Ctrl Pts',(40.4707487026118,41.7119532339184,48.1310819386935));
#23077=CARTESIAN_POINT('Ctrl Pts',(40.4708708148797,41.7024705085611,47.9982268623347));
#23078=CARTESIAN_POINT('Ctrl Pts',(40.4708708172652,41.7025068343519,47.9982242689299));
#23079=CARTESIAN_POINT('Ctrl Pts',(40.4709547042422,41.6965367373028,47.9070906405182));
#23080=CARTESIAN_POINT('Ctrl Pts',(40.4775000933314,41.6905666402537,47.8162440648578));
#23081=CARTESIAN_POINT('Ctrl Pts',(40.4903640311629,41.6845965432046,47.7264437472407));
#23082=CARTESIAN_POINT('Ctrl Pts',(40.4984641755126,41.6808373017878,47.6698984230275));
#23083=CARTESIAN_POINT('Ctrl Pts',(40.5090686524231,41.677078060371,47.6137673003875));
#23084=CARTESIAN_POINT('Ctrl Pts',(40.5221325309265,41.6733188189542,47.5582349883756));
#23085=CARTESIAN_POINT('Ctrl Pts',(40.5376179791024,41.6688627504042,47.4924089980676));
#23086=CARTESIAN_POINT('Ctrl Pts',(40.5565997538975,41.6644066818542,47.4272665547092));
#23087=CARTESIAN_POINT('Ctrl Pts',(40.5790011947558,41.6599506133042,47.3632065419625));
#23088=CARTESIAN_POINT('Ctrl Pts',(40.6013686812249,41.6555012989218,47.2992436264797));
#23089=CARTESIAN_POINT('Ctrl Pts',(40.6271453858133,41.6510519845394,47.2363603479597));
#23090=CARTESIAN_POINT('Ctrl Pts',(40.6562040755905,41.646602670157,47.1749434377494));
#23091=CARTESIAN_POINT('Ctrl Pts',(40.6852283916312,41.6421586189011,47.113599178051));
#23092=CARTESIAN_POINT('Ctrl Pts',(40.7175267728883,41.6377145676452,47.0537182861443));
#23093=CARTESIAN_POINT('Ctrl Pts',(40.7529234645091,41.6332705163893,46.9956686586911));
#23094=CARTESIAN_POINT('Ctrl Pts',(40.7882978569756,41.6288292647901,46.9376556012545));
#23095=CARTESIAN_POINT('Ctrl Pts',(40.826766431711,41.6243880131909,46.8814719405339));
#23096=CARTESIAN_POINT('Ctrl Pts',(40.8681077126806,41.6199467615917,46.8274606288268));
#23097=CARTESIAN_POINT('Ctrl Pts',(40.9094372396547,41.6155067727123,46.7734646734101));
#23098=CARTESIAN_POINT('Ctrl Pts',(40.9536375515899,41.6110667838328,46.7216402328485));
#23099=CARTESIAN_POINT('Ctrl Pts',(41.0004451721161,41.6066267949533,46.6722994160403));
#23100=CARTESIAN_POINT('Ctrl Pts',(41.0472556636165,41.6021865337444,46.6229555728828));
#23101=CARTESIAN_POINT('Ctrl Pts',(41.0966734394862,41.5977462725355,46.5760960122977));
#23102=CARTESIAN_POINT('Ctrl Pts',(41.1483975187492,41.5933060113266,46.5319966669565));
#23103=CARTESIAN_POINT('Ctrl Pts',(41.2001770856412,41.588860986774,46.4878500135114));
#23104=CARTESIAN_POINT('Ctrl Pts',(41.25426751686,41.5844159622214,46.4464698053674));
#23105=CARTESIAN_POINT('Ctrl Pts',(41.3103348355896,41.5799709376688,46.4080915898299));
#23106=CARTESIAN_POINT('Ctrl Pts',(41.3664360672225,41.5755232244967,46.3696901608278));
#23107=CARTESIAN_POINT('Ctrl Pts',(41.4245161442928,41.5710755113246,46.3342945948905));
#23108=CARTESIAN_POINT('Ctrl Pts',(41.4842146373594,41.5666277981524,46.3020954895893));
#23109=CARTESIAN_POINT('Ctrl Pts',(41.5440166770513,41.5621723704524,46.2698405351615));
#23110=CARTESIAN_POINT('Ctrl Pts',(41.605442288967,41.5577169427524,46.2407933171338));
#23111=CARTESIAN_POINT('Ctrl Pts',(41.6681099803568,41.5532615150524,46.215096765635));
#23112=CARTESIAN_POINT('Ctrl Pts',(41.697030645708,41.5512053688844,46.2032380015718));
#23113=CARTESIAN_POINT('Ctrl Pts',(41.7262156185646,41.5491492227164,46.1920921510697));
#23114=CARTESIAN_POINT('Ctrl Pts',(41.7556264548729,41.5470930765484,46.1816696418856));
#23115=CARTESIAN_POINT('Ctrl Pts',(41.8193654558946,41.5426370079984,46.1590820378961));
#23116=CARTESIAN_POINT('Ctrl Pts',(41.8844210576915,41.5381809394484,46.139804735805));
#23117=CARTESIAN_POINT('Ctrl Pts',(41.9504163152003,41.5337248708983,46.1239890545997));
#23118=CARTESIAN_POINT('Ctrl Pts',(42.0163115421492,41.5292755565159,46.1081973455933));
#23119=CARTESIAN_POINT('Ctrl Pts',(42.0831431220984,41.5248262421335,46.0958569591184));
#23120=CARTESIAN_POINT('Ctrl Pts',(42.1505169711984,41.5203769277512,46.0870701070766));
#23121=CARTESIAN_POINT('Ctrl Pts',(42.2178111232798,41.5159328764953,46.0782936490663));
#23122=CARTESIAN_POINT('Ctrl Pts',(42.2856457833941,41.5114888252394,46.0730624413153));
#23123=CARTESIAN_POINT('Ctrl Pts',(42.3536164582438,41.5070447739835,46.0714276980227));
#23124=CARTESIAN_POINT('Ctrl Pts',(42.4215443130304,41.5026035223843,46.0697939845831));
#23125=CARTESIAN_POINT('Ctrl Pts',(42.4896075201079,41.4981622707851,46.0717522533283));
#23126=CARTESIAN_POINT('Ctrl Pts',(42.5573978303185,41.4937210191859,46.0773017709711));
#23127=CARTESIAN_POINT('Ctrl Pts',(42.6251688666464,41.4892810303064,46.0828497107962));
#23128=CARTESIAN_POINT('Ctrl Pts',(42.692666668266,41.484841041427,46.0919868324016));
#23129=CARTESIAN_POINT('Ctrl Pts',(42.7594862043598,41.4804010525475,46.1046603930232));
#23130=CARTESIAN_POINT('Ctrl Pts',(42.826309838871,41.4759607913386,46.1173347309854));
#23131=CARTESIAN_POINT('Ctrl Pts',(42.8924546406677,41.4715205301297,46.1335458440079));
#23132=CARTESIAN_POINT('Ctrl Pts',(42.9575257144821,41.4670802689208,46.1531898758694));
#23133=CARTESIAN_POINT('Ctrl Pts',(43.0226665940747,41.4626352443682,46.1728549811027));
#23134=CARTESIAN_POINT('Ctrl Pts',(43.0867309734581,41.4581902198155,46.1959602114558));
#23135=CARTESIAN_POINT('Ctrl Pts',(43.1493400721229,41.4537451952629,46.2223521121407));
#23136=CARTESIAN_POINT('Ctrl Pts',(43.2119870405549,41.4492974820908,46.2487599762423));
#23137=CARTESIAN_POINT('Ctrl Pts',(43.2731765323258,41.4448497689187,46.2784582512317));
#23138=CARTESIAN_POINT('Ctrl Pts',(43.3325532602683,41.4404020557466,46.3112469174971));
#23139=CARTESIAN_POINT('Ctrl Pts',(43.3920329767367,41.4359466280465,46.3440924554785));
#23140=CARTESIAN_POINT('Ctrl Pts',(43.4496932356182,41.4314912003465,46.3800388213601));
#23141=CARTESIAN_POINT('Ctrl Pts',(43.5052074443319,41.4270357726465,46.4188424930155));
#23142=CARTESIAN_POINT('Ctrl Pts',(43.5308268315607,41.4249796264785,46.4367500938456));
#23143=CARTESIAN_POINT('Ctrl Pts',(43.5559896265865,41.4229234803105,46.4552656648749));
#23144=CARTESIAN_POINT('Ctrl Pts',(43.5806662614674,41.4208673341425,46.4743625149032));
#23145=CARTESIAN_POINT('Ctrl Pts',(43.6341453274618,41.4164112655925,46.5157491021699));
#23146=CARTESIAN_POINT('Ctrl Pts',(43.6855526064654,41.4119551970425,46.5600338327948));
#23147=CARTESIAN_POINT('Ctrl Pts',(43.7345569108915,41.4074991284925,46.6069815476844));
#23148=CARTESIAN_POINT('Ctrl Pts',(43.7834869383439,41.4030498141101,46.6538581028213));
#23149=CARTESIAN_POINT('Ctrl Pts',(43.8300208656851,41.3986004997277,46.7033892932277));
#23150=CARTESIAN_POINT('Ctrl Pts',(43.8738595338283,41.3941511853453,46.7552989790944));
#23151=CARTESIAN_POINT('Ctrl Pts',(43.9176463448905,41.3897071340894,46.8071472606143));
#23152=CARTESIAN_POINT('Ctrl Pts',(43.9587439112277,41.3852630828335,46.8613680747775));
#23153=CARTESIAN_POINT('Ctrl Pts',(43.9968903328296,41.3808190315776,46.9176489378139));
#23154=CARTESIAN_POINT('Ctrl Pts',(44.0350127230065,41.3763777799784,46.9738943451172));
#23155=CARTESIAN_POINT('Ctrl Pts',(44.0701873797892,41.3719365283792,47.0321968192874));
#23156=CARTESIAN_POINT('Ctrl Pts',(44.102194060573,41.36749527678,47.0922126146227));
#23157=CARTESIAN_POINT('Ctrl Pts',(44.1341916413392,41.3630552879006,47.1522113464958));
#23158=CARTESIAN_POINT('Ctrl Pts',(44.1630228018407,41.3586152990211,47.2139219971069));
#23159=CARTESIAN_POINT('Ctrl Pts',(44.1885127819975,41.3541753101416,47.2769753907842));
#23160=CARTESIAN_POINT('Ctrl Pts',(44.2140043255979,41.3497350489327,47.3400326518802));
#23161=CARTESIAN_POINT('Ctrl Pts',(44.2361540993866,41.3452947877238,47.4044323608179));
#23162=CARTESIAN_POINT('Ctrl Pts',(44.2548358143818,41.3408545265149,47.4697862142619));
#23163=CARTESIAN_POINT('Ctrl Pts',(44.2735375704117,41.3364095019623,47.5352101768392));
#23164=CARTESIAN_POINT('Ctrl Pts',(44.2887637072124,41.3319644774097,47.601589850939));
#23165=CARTESIAN_POINT('Ctrl Pts',(44.3004383675356,41.3275194528571,47.6685236537871));
#23166=CARTESIAN_POINT('Ctrl Pts',(44.3121200893991,41.323071739685,47.735497942245));
#23167=CARTESIAN_POINT('Ctrl Pts',(44.3202460008862,41.3186240265128,47.8030265362109));
#23168=CARTESIAN_POINT('Ctrl Pts',(44.3247921167709,41.3141763133407,47.8707024202982));
#23169=CARTESIAN_POINT('Ctrl Pts',(44.3293461178622,41.3097208856407,47.9384956877405));
#23170=CARTESIAN_POINT('Ctrl Pts',(44.3303079245906,41.3052654579407,48.0064362617902));
#23171=CARTESIAN_POINT('Ctrl Pts',(44.3277056620925,41.3008100302407,48.0741177255224));
#23172=CARTESIAN_POINT('Ctrl Pts',(44.3265047376417,41.2987538840727,48.105352208869));
#23173=CARTESIAN_POINT('Ctrl Pts',(44.3245454806939,41.2966977379047,48.1365315920614));
#23174=CARTESIAN_POINT('Ctrl Pts',(44.3218343432927,41.2946415917367,48.1676165679185));
#23175=CARTESIAN_POINT('Ctrl Pts',(44.3159587813817,41.2901855231867,48.2349837548678));
#23176=CARTESIAN_POINT('Ctrl Pts',(44.3065249804363,41.2857294546367,48.3021763817014));
#23177=CARTESIAN_POINT('Ctrl Pts',(44.2935515461884,41.2812733860866,48.3687886912954));
#23178=CARTESIAN_POINT('Ctrl Pts',(44.2805977760792,41.2768240717042,48.4353000350494));
#23179=CARTESIAN_POINT('Ctrl Pts',(44.2641151134346,41.2723747573218,48.5012323264475));
#23180=CARTESIAN_POINT('Ctrl Pts',(44.2441739570645,41.2679254429394,48.566184575015));
#23181=CARTESIAN_POINT('Ctrl Pts',(44.2242563892341,41.2634813916835,48.631059991093));
#23182=CARTESIAN_POINT('Ctrl Pts',(44.2008885963532,41.2590373404276,48.6949571968475));
#23183=CARTESIAN_POINT('Ctrl Pts',(44.1741917003665,41.2545932891718,48.7574868759593));
#23184=CARTESIAN_POINT('Ctrl Pts',(44.14751162285,41.2501520375726,48.8199771627184));
#23185=CARTESIAN_POINT('Ctrl Pts',(44.1175067956851,41.2457107859734,48.8811011786283));
#23186=CARTESIAN_POINT('Ctrl Pts',(44.0843471692799,41.2412695343742,48.9404877299778));
#23187=CARTESIAN_POINT('Ctrl Pts',(44.0511969706933,41.2368295454947,48.9998573967694));
#23188=CARTESIAN_POINT('Ctrl Pts',(44.014893993986,41.2323895566152,49.0574901487156));
#23189=CARTESIAN_POINT('Ctrl Pts',(43.9756541825435,41.2279495677358,49.1130392867879));
#23190=CARTESIAN_POINT('Ctrl Pts',(43.9364119643029,41.2235093065269,49.1685918320008));
#23191=CARTESIAN_POINT('Ctrl Pts',(43.8942328407227,41.2190690453179,49.2220601078674));
#23192=CARTESIAN_POINT('Ctrl Pts',(43.8493750645417,41.214628784109,49.27312783301));
#23193=CARTESIAN_POINT('Ctrl Pts',(43.8044691666411,41.2101837595564,49.3242503416698));
#23194=CARTESIAN_POINT('Ctrl Pts',(43.7568792081038,41.2057387350038,49.3729667888091));
#23195=CARTESIAN_POINT('Ctrl Pts',(43.7069018931882,41.2012937104512,49.4189961234905));
#23196=CARTESIAN_POINT('Ctrl Pts',(43.6568943489718,41.1968459972791,49.4650532994956));
#23197=CARTESIAN_POINT('Ctrl Pts',(43.6044969551146,41.192398284107,49.5084198137376));
#23198=CARTESIAN_POINT('Ctrl Pts',(43.5500390471774,41.1879505709348,49.5488553021077));
#23199=CARTESIAN_POINT('Ctrl Pts',(43.4954866823738,41.1834951432348,49.5893609255541));
#23200=CARTESIAN_POINT('Ctrl Pts',(43.438867082001,41.1790397155348,49.6269251043419));
#23201=CARTESIAN_POINT('Ctrl Pts',(43.3805372695588,41.1745842878348,49.6613516244029));
#23202=CARTESIAN_POINT('Ctrl Pts',(43.3536185025159,41.1725281416668,49.6772392028953));
#23203=CARTESIAN_POINT('Ctrl Pts',(43.3263358248222,41.1704719954988,49.6924591937595));
#23204=CARTESIAN_POINT('Ctrl Pts',(43.2987257854211,41.1684158493308,49.7069957584948));
#23205=CARTESIAN_POINT('Ctrl Pts',(43.2389078604469,41.1639611509718,49.7384896338235));
#23206=CARTESIAN_POINT('Ctrl Pts',(43.1773128632059,41.1595064526128,49.7668983951178));
#23207=CARTESIAN_POINT('Ctrl Pts',(43.1142917840521,41.1550517542537,49.7920183604349));
#23208=CARTESIAN_POINT('Ctrl Pts',(43.0513574843709,41.1506031899752,49.8171037357803));
#23209=CARTESIAN_POINT('Ctrl Pts',(42.9870014511529,41.1461546256967,49.8389091144193));
#23210=CARTESIAN_POINT('Ctrl Pts',(42.9215988152741,41.1417060614182,49.8572768325709));
#23211=CARTESIAN_POINT('Ctrl Pts',(42.8562636241999,41.1372620846084,49.8756256094804));
#23212=CARTESIAN_POINT('Ctrl Pts',(42.7898844443704,41.1328181077987,49.8905436256558));
#23213=CARTESIAN_POINT('Ctrl Pts',(42.7228542004076,41.1283741309889,49.9019221125428));
#23214=CARTESIAN_POINT('Ctrl Pts',(42.6558699067754,41.1239332005981,49.9132927992906));
#23215=CARTESIAN_POINT('Ctrl Pts',(42.5882359204943,41.1194922702072,49.921128690664));
#23216=CARTESIAN_POINT('Ctrl Pts',(42.5203562755619,41.1150513398164,49.9253718923452));
#23217=CARTESIAN_POINT('Ctrl Pts',(42.4524776557753,41.1106104764943,49.9296150299438));
#23218=CARTESIAN_POINT('Ctrl Pts',(42.3843538763555,41.1061696131721,49.9302655382472));
#23219=CARTESIAN_POINT('Ctrl Pts',(42.3163935852902,41.10172874985,49.9273174425401));
#23220=CARTESIAN_POINT('Ctrl Pts',(42.248435826869,41.0972880520235,49.9243694566983));
#23221=CARTESIAN_POINT('Ctrl Pts',(42.1806420378965,41.0928473541969,49.9178231631969));
#23222=CARTESIAN_POINT('Ctrl Pts',(42.1134180541516,41.0884066563703,49.9077246513095));
#23223=CARTESIAN_POINT('Ctrl Pts',(42.0461359862326,41.0839621216057,49.8976174139093));
#23224=CARTESIAN_POINT('Ctrl Pts',(41.9794251940253,41.079517586841,49.8839519130002));
#23225=CARTESIAN_POINT('Ctrl Pts',(41.9136824370759,41.0750730520763,49.8668255903784));
#23226=CARTESIAN_POINT('Ctrl Pts',(41.8734428217844,41.072352655528,49.8563429658941));
#23227=CARTESIAN_POINT('Ctrl Pts',(41.8335656395969,41.0696322589797,49.844564784894));
#23228=CARTESIAN_POINT('Ctrl Pts',(41.7941388317924,41.0669118624314,49.8315225365138));
#23229=CARTESIAN_POINT('Origin',(42.4,48.4493818343519,48.));
#23230=CARTESIAN_POINT('',(41.7941388318207,40.1003056653051,49.8315225365232));
#23231=CARTESIAN_POINT('',(41.7933319732428,40.273017144546,49.8339081536803));
#23232=CARTESIAN_POINT('',(41.7941388317924,48.4493818343519,49.8315225365138));
#23233=CARTESIAN_POINT('Ctrl Pts',(41.7941388318207,40.1003056653051,49.8315225365232));
#23234=CARTESIAN_POINT('Ctrl Pts',(41.9417997033319,40.110751722448,49.8803682298326));
#23235=CARTESIAN_POINT('Ctrl Pts',(42.094800152278,40.1218028811348,49.9111691005024));
#23236=CARTESIAN_POINT('Ctrl Pts',(42.3518158958192,40.1402150999778,49.9312408979334));
#23237=CARTESIAN_POINT('Ctrl Pts',(42.454315125457,40.1474984258421,49.9310794105004));
#23238=CARTESIAN_POINT('Ctrl Pts',(42.5689914074891,40.1552819395496,49.9217559422526));
#23239=CARTESIAN_POINT('Ctrl Pts',(42.581645482915,40.1561356585347,49.920601191584));
#23240=CARTESIAN_POINT('Ctrl Pts',(42.6005145546417,40.1574000601793,49.9186911273435));
#23241=CARTESIAN_POINT('Ctrl Pts',(42.60673848085,40.1578157182278,49.9180304825638));
#23242=CARTESIAN_POINT('Ctrl Pts',(42.6174262346275,40.1585269504496,49.9168433921574));
#23243=CARTESIAN_POINT('Ctrl Pts',(42.6218915433195,40.1588233331116,49.9163316263134));
#23244=CARTESIAN_POINT('Ctrl Pts',(42.6320931728744,40.1594986906424,49.9151262883405));
#23245=CARTESIAN_POINT('Ctrl Pts',(42.6378281930103,40.1598770891584,49.9144225484361));
#23246=CARTESIAN_POINT('Ctrl Pts',(42.6535927438972,40.1609139722711,49.9124161582588));
#23247=CARTESIAN_POINT('Ctrl Pts',(42.6636154988476,40.1615695584285,49.9110603657899));
#23248=CARTESIAN_POINT('Ctrl Pts',(42.7165797682563,40.1650168705974,49.9034711956959));
#23249=CARTESIAN_POINT('Ctrl Pts',(42.7593160644031,40.1677390954992,49.8958686556973));
#23250=CARTESIAN_POINT('Ctrl Pts',(42.8190628227866,40.1715067945335,49.8831467703358));
#23251=CARTESIAN_POINT('Ctrl Pts',(42.8363115276671,40.1725899837901,49.8792252894721));
#23252=CARTESIAN_POINT('Ctrl Pts',(42.8655653586619,40.1744229785679,49.8721499494924));
#23253=CARTESIAN_POINT('Ctrl Pts',(42.8775981932023,40.175175745795,49.8691165053104));
#23254=CARTESIAN_POINT('Ctrl Pts',(43.0003577371279,40.1828506939619,49.8369062892878));
#23255=CARTESIAN_POINT('Ctrl Pts',(43.108307736997,40.1895737292688,49.7980420934161));
#23256=CARTESIAN_POINT('Ctrl Pts',(43.2889365399485,40.2016087955895,49.7142041968312));
#23257=CARTESIAN_POINT('Ctrl Pts',(43.3632612226724,40.20681475279,49.673567853177));
#23258=CARTESIAN_POINT('Ctrl Pts',(43.4495224805585,40.2133181221175,49.6187509635083));
#23259=CARTESIAN_POINT('Ctrl Pts',(43.4642419484988,40.2144447903505,49.6091119169191));
#23260=CARTESIAN_POINT('Ctrl Pts',(43.4872367266874,40.2162329062418,49.5936002509831));
#23261=CARTESIAN_POINT('Ctrl Pts',(43.4956013061423,40.2168893142542,49.5878612128394));
#23262=CARTESIAN_POINT('Ctrl Pts',(43.5111936786003,40.2181243650534,49.5769812393727));
#23263=CARTESIAN_POINT('Ctrl Pts',(43.5184320621103,40.2187024006963,49.5718558899296));
#23264=CARTESIAN_POINT('Ctrl Pts',(43.5345790544161,40.2200025665416,49.5602545384407));
#23265=CARTESIAN_POINT('Ctrl Pts',(43.5434680056432,40.2207257183945,49.5537518357014));
#23266=CARTESIAN_POINT('Ctrl Pts',(43.5659821423875,40.2225765959712,49.536983804038));
#23267=CARTESIAN_POINT('Ctrl Pts',(43.579527499039,40.2237084070158,49.5266133817451));
#23268=CARTESIAN_POINT('Ctrl Pts',(43.6798932593009,40.2322347925752,49.4476394271683));
#23269=CARTESIAN_POINT('Ctrl Pts',(43.7607898711524,40.2399209921067,49.3718709906854));
#23270=CARTESIAN_POINT('Ctrl Pts',(43.9307729139648,40.257960721092,49.1827574868696));
#23271=CARTESIAN_POINT('Ctrl Pts',(44.0145749331128,40.2683830478816,49.0655193927069));
#23272=CARTESIAN_POINT('Ctrl Pts',(44.0948608350144,40.2796624190017,48.9216474148817));
#23273=CARTESIAN_POINT('Ctrl Pts',(44.1048342876457,40.2810918586419,48.9030655287994));
#23274=CARTESIAN_POINT('Ctrl Pts',(44.1180108119841,40.2830163594297,48.8775192374203));
#23275=CARTESIAN_POINT('Ctrl Pts',(44.1214796324773,40.2835265866745,48.8706945744657));
#23276=CARTESIAN_POINT('Ctrl Pts',(44.1272277269227,40.2843779323347,48.8592169556688));
#23277=CARTESIAN_POINT('Ctrl Pts',(44.129529021435,40.2847203946612,48.8545751948618));
#23278=CARTESIAN_POINT('Ctrl Pts',(44.1338721102007,40.2853697304738,48.8457256853358));
#23279=CARTESIAN_POINT('Ctrl Pts',(44.1359173394209,40.2856768243729,48.8415197093557));
#23280=CARTESIAN_POINT('Ctrl Pts',(44.1407498964978,40.2864056833402,48.8314890555598));
#23281=CARTESIAN_POINT('Ctrl Pts',(44.1435233374075,40.2868265980652,48.8256576933044));
#23282=CARTESIAN_POINT('Ctrl Pts',(44.1532687309632,40.2883154000398,48.8048992079333));
#23283=CARTESIAN_POINT('Ctrl Pts',(44.160078922686,40.2893739097298,48.7898963270121));
#23284=CARTESIAN_POINT('Ctrl Pts',(44.2078613594484,40.2969483306882,48.6809440230193));
#23285=CARTESIAN_POINT('Ctrl Pts',(44.2414861357994,40.3030975850257,48.5839364046351));
#23286=CARTESIAN_POINT('Ctrl Pts',(44.2943161442119,40.3156524624026,48.3804177004246));
#23287=CARTESIAN_POINT('Ctrl Pts',(44.3126016608496,40.322038007028,48.2740520015252));
#23288=CARTESIAN_POINT('Ctrl Pts',(44.326735158817,40.332086908909,48.111123124695));
#23289=CARTESIAN_POINT('Ctrl Pts',(44.3291429028897,40.3355712281245,48.0553487415454));
#23290=CARTESIAN_POINT('Ctrl Pts',(44.3291263159966,40.3401293230084,47.9839090586368));
#23291=CARTESIAN_POINT('Ctrl Pts',(44.3289324137831,40.3411330932029,47.968267033101));
#23292=CARTESIAN_POINT('Ctrl Pts',(44.3283096522953,40.3427701760943,47.9429131821155));
#23293=CARTESIAN_POINT('Ctrl Pts',(44.3279975726937,40.3433998170171,47.9331989982244));
#23294=CARTESIAN_POINT('Ctrl Pts',(44.3272569746067,40.3446139818703,47.9145407372712));
#23295=CARTESIAN_POINT('Ctrl Pts',(44.3268395619174,40.3451981414213,47.9055964523037));
#23296=CARTESIAN_POINT('Ctrl Pts',(44.3257402812549,40.3465414232836,47.8851056602076));
#23297=CARTESIAN_POINT('Ctrl Pts',(44.3250168097472,40.3473018336337,47.8735618237272));
#23298=CARTESIAN_POINT('Ctrl Pts',(44.3223793737449,40.3497367056006,47.83678022075));
#23299=CARTESIAN_POINT('Ctrl Pts',(44.3200725934344,40.3514233884554,47.8115741924639));
#23300=CARTESIAN_POINT('Ctrl Pts',(44.3023435777907,40.3621926561487,47.6524225257492));
#23301=CARTESIAN_POINT('Ctrl Pts',(44.2734124885541,40.3717035878287,47.5203809366346));
#23302=CARTESIAN_POINT('Ctrl Pts',(44.2075958273054,40.3866276316793,47.3220277889969));
#23303=CARTESIAN_POINT('Ctrl Pts',(44.1801813062461,40.3919405292553,47.2530031806838));
#23304=CARTESIAN_POINT('Ctrl Pts',(44.134411331972,40.3995581310088,47.1547004869882));
#23305=CARTESIAN_POINT('Ctrl Pts',(44.1191409972667,40.4019395121946,47.124061391812));
#23306=CARTESIAN_POINT('Ctrl Pts',(44.0928774960435,40.4057700870818,47.074700856978));
#23307=CARTESIAN_POINT('Ctrl Pts',(44.0823698162676,40.4072407541839,47.0557306424382));
#23308=CARTESIAN_POINT('Ctrl Pts',(44.0676812519924,40.4092111259118,47.0302362822469));
#23309=CARTESIAN_POINT('Ctrl Pts',(44.0637781350985,40.409726918484,47.0235550457194));
#23310=CARTESIAN_POINT('Ctrl Pts',(44.0571860286228,40.4105849458717,47.0124251725123));
#23311=CARTESIAN_POINT('Ctrl Pts',(44.0545191026196,40.410928569234,47.007963652678));
#23312=CARTESIAN_POINT('Ctrl Pts',(44.0494259954213,40.4115781162381,46.9995210264337));
#23313=CARTESIAN_POINT('Ctrl Pts',(44.0470033694404,40.4118842735511,46.9955378587875));
#23314=CARTESIAN_POINT('Ctrl Pts',(44.0412214686857,40.4126084237112,46.9861086892509));
#23315=CARTESIAN_POINT('Ctrl Pts',(44.0378494652773,40.4130255919084,46.9806704991874));
#23316=CARTESIAN_POINT('Ctrl Pts',(44.0258847013086,40.4144881840771,46.9615870192747));
#23317=CARTESIAN_POINT('Ctrl Pts',(44.0171476943862,40.4155246545485,46.9480323407776));
#23318=CARTESIAN_POINT('Ctrl Pts',(43.9442392261779,40.4239343505241,46.8379768422594));
#23319=CARTESIAN_POINT('Ctrl Pts',(43.8716523813066,40.4308341587448,46.7473151739668));
#23320=CARTESIAN_POINT('Ctrl Pts',(43.6932765016396,40.4461933452028,46.5615888541548));
#23321=CARTESIAN_POINT('Ctrl Pts',(43.5842669151826,40.4546360512688,46.470589617404));
#23322=CARTESIAN_POINT('Ctrl Pts',(43.4489899111222,40.4649240456652,46.3808663920005));
#23323=CARTESIAN_POINT('Ctrl Pts',(43.4315070608787,40.4662494439422,46.3696728536568));
#23324=CARTESIAN_POINT('Ctrl Pts',(43.4046499532447,40.4682810015496,46.3530823018262));
#23325=CARTESIAN_POINT('Ctrl Pts',(43.3954049545883,40.4689795210464,46.3474781690943));
#23326=CARTESIAN_POINT('Ctrl Pts',(43.3785013684331,40.4702554961488,46.3374248680319));
#23327=CARTESIAN_POINT('Ctrl Pts',(43.3708582654323,40.4708319983841,46.3329501442662));
#23328=CARTESIAN_POINT('Ctrl Pts',(43.3542617006342,40.4720830327096,46.3233863823124));
#23329=CARTESIAN_POINT('Ctrl Pts',(43.3452977942177,40.4727582214937,46.3183161148528));
#23330=CARTESIAN_POINT('Ctrl Pts',(43.3207089595532,40.4746092016209,46.3046666098901));
#23331=CARTESIAN_POINT('Ctrl Pts',(43.3050053596735,40.4757901042452,46.2962319540647));
#23332=CARTESIAN_POINT('Ctrl Pts',(43.2172125876069,40.4823872207518,46.2506332463756));
#23333=CARTESIAN_POINT('Ctrl Pts',(43.1429616252921,40.4879538976458,46.2178312858369));
#23334=CARTESIAN_POINT('Ctrl Pts',(42.947601533405,40.5025486194758,46.1458607881171));
#23335=CARTESIAN_POINT('Ctrl Pts',(42.8242785740639,40.5117296819375,46.1138176641386));
#23336=CARTESIAN_POINT('Ctrl Pts',(42.6367763687192,40.5251454393547,46.0844295552565));
#23337=CARTESIAN_POINT('Ctrl Pts',(42.574394352051,40.5295162481237,46.0777457252237));
#23338=CARTESIAN_POINT('Ctrl Pts',(42.5010349178353,40.5344701898344,46.073487452713));
#23339=CARTESIAN_POINT('Ctrl Pts',(42.4902730477458,40.5351922360268,46.0729531818098));
#23340=CARTESIAN_POINT('Ctrl Pts',(42.4736511330289,40.5362996219209,46.0722675453735));
#23341=CARTESIAN_POINT('Ctrl Pts',(42.4677941333653,40.5366883276011,46.0720526812786));
#23342=CARTESIAN_POINT('Ctrl Pts',(42.4569543397704,40.5374048344325,46.071704482161));
#23343=CARTESIAN_POINT('Ctrl Pts',(42.4519720205151,40.537733023192,46.0715637653955));
#23344=CARTESIAN_POINT('Ctrl Pts',(42.440578507512,40.5384809611306,46.0712861640979));
#23345=CARTESIAN_POINT('Ctrl Pts',(42.434167134293,40.5389000018557,46.0711619337227));
#23346=CARTESIAN_POINT('Ctrl Pts',(42.4173225860087,40.539996391233,46.0709195595341));
#23347=CARTESIAN_POINT('Ctrl Pts',(42.4068886996906,40.5406709316627,46.0708540814113));
#23348=CARTESIAN_POINT('Ctrl Pts',(42.3202927448594,40.5462350177639,46.0710132333689));
#23349=CARTESIAN_POINT('Ctrl Pts',(42.2441962217715,40.5509056905943,46.0756634267802));
#23350=CARTESIAN_POINT('Ctrl Pts',(42.0778108905353,40.5610163586496,46.0957695946922));
#23351=CARTESIAN_POINT('Ctrl Pts',(41.9879493351605,40.5664135498373,46.1131735276365));
#23352=CARTESIAN_POINT('Ctrl Pts',(41.8102644416101,40.5774586906191,46.1608908987508));
#23353=CARTESIAN_POINT('Ctrl Pts',(41.7227235722522,40.5830956859637,46.1912977144555));
#23354=CARTESIAN_POINT('Ctrl Pts',(41.6159302159832,40.5904388173201,46.237235347621));
#23355=CARTESIAN_POINT('Ctrl Pts',(41.5943266028937,40.5919488731925,46.2470040090321));
#23356=CARTESIAN_POINT('Ctrl Pts',(41.5626162810388,40.5942047603212,46.2620526851427));
#23357=CARTESIAN_POINT('Ctrl Pts',(41.552366991471,40.5949400908624,46.2670283800173));
#23358=CARTESIAN_POINT('Ctrl Pts',(41.5341856274308,40.5962558744529,46.2760547154927));
#23359=CARTESIAN_POINT('Ctrl Pts',(41.5262363335693,40.5968350803296,46.2800700821029));
#23360=CARTESIAN_POINT('Ctrl Pts',(41.5095051351027,40.5980626020129,46.2886673133666));
#23361=CARTESIAN_POINT('Ctrl Pts',(41.5007301711631,40.5987113598786,46.2932620478017));
#23362=CARTESIAN_POINT('Ctrl Pts',(41.4774373787271,40.6004469554241,46.305688087215));
#23363=CARTESIAN_POINT('Ctrl Pts',(41.4629842193625,40.6015379954668,46.3136382221086));
#23364=CARTESIAN_POINT('Ctrl Pts',(41.3982778658854,40.6064878547876,46.3503193932303));
#23365=CARTESIAN_POINT('Ctrl Pts',(41.3492359528753,40.6104203718835,46.3811154877808));
#23366=CARTESIAN_POINT('Ctrl Pts',(41.1930143323616,40.6235615783891,46.4893073054275));
#23367=CARTESIAN_POINT('Ctrl Pts',(41.0924001713771,40.6330590924896,46.575506361972));
#23368=CARTESIAN_POINT('Ctrl Pts',(40.9623256012841,40.6465029188335,46.712423562647));
#23369=CARTESIAN_POINT('Ctrl Pts',(40.925083313537,40.6505128018396,46.7552581015143));
#23370=CARTESIAN_POINT('Ctrl Pts',(40.8707076216271,40.65655740037,46.823672212863));
#23371=CARTESIAN_POINT('Ctrl Pts',(40.8522075615836,40.6586517173107,46.8481228075257));
#23372=CARTESIAN_POINT('Ctrl Pts',(40.8291703805095,40.6612991634921,46.8801277436908));
#23373=CARTESIAN_POINT('Ctrl Pts',(40.8240923622885,40.661885327244,46.8872849921935));
#23374=CARTESIAN_POINT('Ctrl Pts',(40.8159552978936,40.6628285141119,46.8989212783622));
#23375=CARTESIAN_POINT('Ctrl Pts',(40.8128660616002,40.6631875274136,46.9033789018485));
#23376=CARTESIAN_POINT('Ctrl Pts',(40.8069364447978,40.6638783520808,46.9120126049537));
#23377=CARTESIAN_POINT('Ctrl Pts',(40.8040936222508,40.6642103196321,46.9161868718386));
#23378=CARTESIAN_POINT('Ctrl Pts',(40.7978470774428,40.6649415632018,46.9254368716389));
#23379=CARTESIAN_POINT('Ctrl Pts',(40.7944509842546,40.6653403307043,46.9305177586199));
#23380=CARTESIAN_POINT('Ctrl Pts',(40.7825172907873,40.6667462130417,46.9485566878378));
#23381=CARTESIAN_POINT('Ctrl Pts',(40.7741116813166,40.6677449623632,46.9616019234378));
#23382=CARTESIAN_POINT('Ctrl Pts',(40.6950451642346,40.6772371371896,47.0876249820522));
#23383=CARTESIAN_POINT('Ctrl Pts',(40.6361014036552,40.6850947264693,47.2075535069091));
#23384=CARTESIAN_POINT('Ctrl Pts',(40.5832793780464,40.6942070585453,47.3508121732161));
#23385=CARTESIAN_POINT('Ctrl Pts',(40.5768450938865,40.6953655303543,47.3691079078347));
#23386=CARTESIAN_POINT('Ctrl Pts',(40.5412818275329,40.7020732158501,47.4753218570515));
#23387=CARTESIAN_POINT('Ctrl Pts',(40.5182414996086,40.7076836396037,47.5651406787126));
#23388=CARTESIAN_POINT('Ctrl Pts',(40.4964455500316,40.7153620873896,47.6855061952501));
#23389=CARTESIAN_POINT('Ctrl Pts',(40.491826549795,40.7172467537808,47.7148687503005));
#23390=CARTESIAN_POINT('Ctrl Pts',(40.4862369811517,40.7199516243615,47.7566713726347));
#23391=CARTESIAN_POINT('Ctrl Pts',(40.4847057662242,40.7207541680439,47.7690331207121));
#23392=CARTESIAN_POINT('Ctrl Pts',(40.4822672299272,40.7221473156802,47.790415279881));
#23393=CARTESIAN_POINT('Ctrl Pts',(40.4813035713438,40.722736124833,47.7994289595217));
#23394=CARTESIAN_POINT('Ctrl Pts',(40.479464053374,40.7239436000353,47.8178633801338));
#23395=CARTESIAN_POINT('Ctrl Pts',(40.4785939011038,40.7245624290778,47.8272844294978));
#23396=CARTESIAN_POINT('Ctrl Pts',(40.476570168006,40.7261318402742,47.851107481023));
#23397=CARTESIAN_POINT('Ctrl Pts',(40.4755090332667,40.7270853008353,47.8655165423795));
#23398=CARTESIAN_POINT('Ctrl Pts',(40.4720939067683,40.7307260192037,47.9202826825161));
#23399=CARTESIAN_POINT('Ctrl Pts',(40.4708469418687,40.7334474714769,47.9606958459015));
#23400=CARTESIAN_POINT('Ctrl Pts',(40.4709085825278,40.740719875977,48.0672588147051));
#23401=CARTESIAN_POINT('Ctrl Pts',(40.4743484768184,40.7453296025145,48.1333497355389));
#23402=CARTESIAN_POINT('Ctrl Pts',(40.4957775446428,40.7599959601246,48.339843184221));
#23403=CARTESIAN_POINT('Ctrl Pts',(40.5258137430645,40.7702637749302,48.4785207838106));
#23404=CARTESIAN_POINT('Ctrl Pts',(40.5810551611003,40.7823215734393,48.6434567674931));
#23405=CARTESIAN_POINT('Ctrl Pts',(40.5921441131223,40.784544458076,48.6739839246788));
#23406=CARTESIAN_POINT('Ctrl Pts',(40.6073981370496,40.7873532077696,48.712886954693));
#23407=CARTESIAN_POINT('Ctrl Pts',(40.6108598177641,40.7879757256517,48.721530779779));
#23408=CARTESIAN_POINT('Ctrl Pts',(40.6164815524939,40.7889629834857,48.7352790059569));
#23409=CARTESIAN_POINT('Ctrl Pts',(40.6186012010772,40.7893300536813,48.7403996152913));
#23410=CARTESIAN_POINT('Ctrl Pts',(40.6226965602814,40.7900293842234,48.7501737110327));
#23411=CARTESIAN_POINT('Ctrl Pts',(40.6246685178124,40.7903618506289,48.7548286179249));
#23412=CARTESIAN_POINT('Ctrl Pts',(40.6294063280299,40.7911506642196,48.7658911882673));
#23413=CARTESIAN_POINT('Ctrl Pts',(40.6321887279894,40.7916060146594,48.7722917672449));
#23414=CARTESIAN_POINT('Ctrl Pts',(40.641729145953,40.7931413835098,48.7939166218842));
#23415=CARTESIAN_POINT('Ctrl Pts',(40.6486498011372,40.7942120281791,48.8090689246679));
#23416=CARTESIAN_POINT('Ctrl Pts',(40.6659910317275,40.7967972211464,48.8457708417275));
#23417=CARTESIAN_POINT('Ctrl Pts',(40.6766182819495,40.7983011482689,48.8672202611373));
#23418=CARTESIAN_POINT('Ctrl Pts',(40.7211294447461,40.8043100800076,48.9530073491391));
#23419=CARTESIAN_POINT('Ctrl Pts',(40.7582411803242,40.808682413978,49.0156076718594));
#23420=CARTESIAN_POINT('Ctrl Pts',(40.8855125480237,40.8223216435242,49.2050063163955));
#23421=CARTESIAN_POINT('Ctrl Pts',(40.9874925675597,40.8314953805544,49.3230758438179));
#23422=CARTESIAN_POINT('Ctrl Pts',(41.120282241947,40.8428259013328,49.4437591321584));
#23423=CARTESIAN_POINT('Ctrl Pts',(41.1383327932775,40.8443534167587,49.4595594369491));
#23424=CARTESIAN_POINT('Ctrl Pts',(41.1654244714394,40.8466304097556,49.4823956413424));
#23425=CARTESIAN_POINT('Ctrl Pts',(41.1742416201356,40.8473690935423,49.4896945855008));
#23426=CARTESIAN_POINT('Ctrl Pts',(41.1900384229289,40.8486886201596,49.5025361774477));
#23427=CARTESIAN_POINT('Ctrl Pts',(41.1969925729493,40.8492681890081,49.5081097799927));
#23428=CARTESIAN_POINT('Ctrl Pts',(41.2117339572474,40.8504941341118,49.5197578442459));
#23429=CARTESIAN_POINT('Ctrl Pts',(41.2195296974178,40.8511409357268,49.5258210747216));
#23430=CARTESIAN_POINT('Ctrl Pts',(41.2403637024477,40.8528657030654,49.5417697386173));
#23431=CARTESIAN_POINT('Ctrl Pts',(41.2534815264133,40.8539477792481,49.5515494291376));
#23432=CARTESIAN_POINT('Ctrl Pts',(41.3189507157316,40.8593305459919,49.5990748360092));
#23433=CARTESIAN_POINT('Ctrl Pts',(41.3730435103735,40.8637247399463,49.6343398102676));
#23434=CARTESIAN_POINT('Ctrl Pts',(41.4940758530742,40.8734467339797,49.7048613272617));
#23435=CARTESIAN_POINT('Ctrl Pts',(41.5615282696256,40.8787984580475,49.7390267930907));
#23436=CARTESIAN_POINT('Ctrl Pts',(41.6843087315625,40.8883492346791,49.792409657613));
#23437=CARTESIAN_POINT('Ctrl Pts',(41.738810557847,40.8925251977351,49.8132201490352));
#23438=CARTESIAN_POINT('Ctrl Pts',(41.7941391176755,40.8966643233312,49.831522631083));
#23439=CARTESIAN_POINT('',(40.4706609686455,40.9087567724484,48.0006653527742));
#23440=CARTESIAN_POINT('Ctrl Pts',(41.7941388317924,41.0669118624314,49.8315225365138));
#23441=CARTESIAN_POINT('Ctrl Pts',(41.7295757742925,41.0624570985652,49.8101653057618));
#23442=CARTESIAN_POINT('Ctrl Pts',(41.6662218155483,41.0580023346989,49.7854160650458));
#23443=CARTESIAN_POINT('Ctrl Pts',(41.604445100534,41.0535475708326,49.7574512678409));
#23444=CARTESIAN_POINT('Ctrl Pts',(41.5519449881319,41.0497617495301,49.7336857601377));
#23445=CARTESIAN_POINT('Ctrl Pts',(41.5005837656602,41.0459759282275,49.7075988058735));
#23446=CARTESIAN_POINT('Ctrl Pts',(41.4505716588481,41.042190106925,49.6793237870993));
#23447=CARTESIAN_POINT('Ctrl Pts',(41.3917053367279,41.037734038375,49.6460429183415));
#23448=CARTESIAN_POINT('Ctrl Pts',(41.3344733071312,41.033277969825,49.6095965126297));
#23449=CARTESIAN_POINT('Ctrl Pts',(41.279237085149,41.0288219012749,49.5701697505667));
#23450=CARTESIAN_POINT('Ctrl Pts',(41.2240845860042,41.0243725868925,49.5308027485718));
#23451=CARTESIAN_POINT('Ctrl Pts',(41.1709222897294,41.0199232725101,49.4884646395959));
#23452=CARTESIAN_POINT('Ctrl Pts',(41.1200858975378,41.0154739581277,49.4433857582845));
#23453=CARTESIAN_POINT('Ctrl Pts',(41.0693096400861,41.0110299068719,49.3983602011112));
#23454=CARTESIAN_POINT('Ctrl Pts',(41.0208541905169,41.006585855616,49.3506006360544));
#23455=CARTESIAN_POINT('Ctrl Pts',(40.9750235941449,41.0021418043601,49.3003787139353));
#23456=CARTESIAN_POINT('Ctrl Pts',(40.9292218700627,40.9977005527609,49.250188430547));
#23457=CARTESIAN_POINT('Ctrl Pts',(40.8860420512438,40.9932593011617,49.1975392309242));
#23458=CARTESIAN_POINT('Ctrl Pts',(40.8457514447914,40.9888180495625,49.1427396840628));
#23459=CARTESIAN_POINT('Ctrl Pts',(40.8054722936107,40.984378060683,49.0879557175998));
#23460=CARTESIAN_POINT('Ctrl Pts',(40.7680810164976,40.9799380718036,49.0310230151296));
#23461=CARTESIAN_POINT('Ctrl Pts',(40.7338035596483,40.9754980829241,48.9722818413708));
#23462=CARTESIAN_POINT('Ctrl Pts',(40.6995240003702,40.9710578217152,48.9135370646859));
#23463=CARTESIAN_POINT('Ctrl Pts',(40.6683588870979,40.9666175605063,48.8529840242597));
#23464=CARTESIAN_POINT('Ctrl Pts',(40.6404889427882,40.9621772992974,48.7909888725194));
#23465=CARTESIAN_POINT('Ctrl Pts',(40.6125891006601,40.9577322747448,48.7289272147334));
#23466=CARTESIAN_POINT('Ctrl Pts',(40.5879916846751,40.9532872501922,48.6654208095263));
#23467=CARTESIAN_POINT('Ctrl Pts',(40.5668294146933,40.9488422256396,48.6008561908363));
#23468=CARTESIAN_POINT('Ctrl Pts',(40.5456543444915,40.9443945124674,48.5362525195623));
#23469=CARTESIAN_POINT('Ctrl Pts',(40.5279186839299,40.9399467992953,48.4705898377334));
#23470=CARTESIAN_POINT('Ctrl Pts',(40.5137045979685,40.9354990861232,48.4042675020018));
#23471=CARTESIAN_POINT('Ctrl Pts',(40.4994658577728,40.9310436584232,48.3378301306353));
#23472=CARTESIAN_POINT('Ctrl Pts',(40.488760960153,40.9265882307232,48.2707313091753));
#23473=CARTESIAN_POINT('Ctrl Pts',(40.4816204135195,40.9221328030231,48.2033772825931));
#23474=CARTESIAN_POINT('Ctrl Pts',(40.4783251052828,40.9200766568551,48.1722939090133));
#23475=CARTESIAN_POINT('Ctrl Pts',(40.4757881850223,40.9180205106871,48.1411562042223));
#23476=CARTESIAN_POINT('Ctrl Pts',(40.4740089101723,40.9159643645191,48.1100039944922));
#23477=CARTESIAN_POINT('Ctrl Pts',(40.4719299112248,40.9135618544634,48.0736041031328));
#23478=CARTESIAN_POINT('Ctrl Pts',(40.4708827128295,40.9111593444076,48.0371447193032));
#23479=CARTESIAN_POINT('Ctrl Pts',(40.4708701150393,40.9087568343519,48.0006662218881));
#23480=CARTESIAN_POINT('Ctrl Pts',(40.4679315868973,40.9087559646023,48.0006540107483));
#23481=CARTESIAN_POINT('Ctrl Pts',(40.4706336067486,40.8690835171059,47.397369030549));
#23482=CARTESIAN_POINT('Ctrl Pts',(41.0996381208906,40.7873358221411,46.1494151750972));
#23483=CARTESIAN_POINT('Ctrl Pts',(43.2260810454985,40.6635128797074,45.8734020167473));
#23484=CARTESIAN_POINT('Ctrl Pts',(44.6354314050272,40.5372871373016,47.5442859344671));
#23485=CARTESIAN_POINT('Ctrl Pts',(43.992617684286,40.4110613948957,49.6335231212952));
#23486=CARTESIAN_POINT('Ctrl Pts',(42.5236823535331,40.3229713973105,50.0450157258572));
#23487=CARTESIAN_POINT('Ctrl Pts',(41.8501070242599,40.2769566471939,49.8531354571792));
#23488=CARTESIAN_POINT('Ctrl Pts',(41.7933319732428,40.273017144546,49.8339081536803));
#23489=CARTESIAN_POINT('Origin',(42.4,48.4493818343519,48.));
#23490=CARTESIAN_POINT('',(41.7943887027378,39.3084106968695,49.8307330830672));
#23491=CARTESIAN_POINT('',(41.7941386883808,39.4806729614233,49.8315224890738));
#23492=CARTESIAN_POINT('',(41.7941388317924,48.4493818343519,49.8315225365138));
#23493=CARTESIAN_POINT('',(40.4723183568643,39.943967372631,47.9983796934389));
#23494=CARTESIAN_POINT('Ctrl Pts',(40.4723183568643,39.943967372631,47.9983796934389));
#23495=CARTESIAN_POINT('Ctrl Pts',(40.4707394637107,39.9308026672141,47.7970115409001));
#23496=CARTESIAN_POINT('Ctrl Pts',(40.5925624326654,39.8755627143287,46.9539226443301));
#23497=CARTESIAN_POINT('Ctrl Pts',(41.8157413936134,39.7782475139746,45.7946723748715));
#23498=CARTESIAN_POINT('Ctrl Pts',(43.9386634949042,39.6520217715687,46.3155586377849));
#23499=CARTESIAN_POINT('Ctrl Pts',(44.6490663174714,39.5257960291628,48.3827907429751));
#23500=CARTESIAN_POINT('Ctrl Pts',(43.4201964457156,39.4112590042631,49.939726251279));
#23501=CARTESIAN_POINT('Ctrl Pts',(42.2366982772441,39.338797226832,49.9723701804534));
#23502=CARTESIAN_POINT('Ctrl Pts',(41.794388702738,39.3084106968696,49.8307330830672));
#23503=CARTESIAN_POINT('Ctrl Pts',(40.4708706300359,39.9431346927996,47.9984408842249));
#23504=CARTESIAN_POINT('Ctrl Pts',(40.4708198929901,39.9469209793088,48.0612189837307));
#23505=CARTESIAN_POINT('Ctrl Pts',(40.4738335460248,39.9507533765101,48.1239587143083));
#23506=CARTESIAN_POINT('Ctrl Pts',(40.4829575575197,39.9566479477974,48.2179258832443));
#23507=CARTESIAN_POINT('Ctrl Pts',(40.486788968357,39.9586440079182,48.2493326845192));
#23508=CARTESIAN_POINT('Ctrl Pts',(40.4930226546594,39.9613803307887,48.2917290150256));
#23509=CARTESIAN_POINT('Ctrl Pts',(40.4947513793214,39.9620996324809,48.3028136368557));
#23510=CARTESIAN_POINT('Ctrl Pts',(40.4979882649397,39.963380594018,48.3224425308214));
#23511=CARTESIAN_POINT('Ctrl Pts',(40.4994575820188,39.963941019675,48.3309929597083));
#23512=CARTESIAN_POINT('Ctrl Pts',(40.5025547379043,39.9650814816492,48.3483154166093));
#23513=CARTESIAN_POINT('Ctrl Pts',(40.5041858524087,39.9656616091957,48.3570866357031));
#23514=CARTESIAN_POINT('Ctrl Pts',(40.5077428997219,39.9668853856204,48.3755028016507));
#23515=CARTESIAN_POINT('Ctrl Pts',(40.5096818636515,39.9675294361126,48.3851449401285));
#23516=CARTESIAN_POINT('Ctrl Pts',(40.5150043720375,39.9692389829103,48.4106040159622));
#23517=CARTESIAN_POINT('Ctrl Pts',(40.518513197882,39.9703084618701,48.426393669733));
#23518=CARTESIAN_POINT('Ctrl Pts',(40.5348792070062,39.9750584023931,48.4959010127887));
#23519=CARTESIAN_POINT('Ctrl Pts',(40.549840314866,39.978805646307,48.5490915100576));
#23520=CARTESIAN_POINT('Ctrl Pts',(40.5873785567798,39.9871146086576,48.663469104035));
#23521=CARTESIAN_POINT('Ctrl Pts',(40.610817533297,39.9916969155441,48.7243014571535));
#23522=CARTESIAN_POINT('Ctrl Pts',(40.6913670948981,40.0057803290618,48.9054456747975));
#23523=CARTESIAN_POINT('Ctrl Pts',(40.7578893999033,40.0154128887556,49.0211432663966));
#23524=CARTESIAN_POINT('Ctrl Pts',(40.8459046548955,40.025761835615,49.1430785446304));
#23525=CARTESIAN_POINT('Ctrl Pts',(40.856201949067,40.0269416262726,49.1569479352129));
#23526=CARTESIAN_POINT('Ctrl Pts',(40.8745582195432,40.0289889028447,49.1809903803335));
#23527=CARTESIAN_POINT('Ctrl Pts',(40.882536022862,40.029860989169,49.1912237424591));
#23528=CARTESIAN_POINT('Ctrl Pts',(40.8945474054465,40.0311471005716,49.2063145860914));
#23529=CARTESIAN_POINT('Ctrl Pts',(40.8985023630385,40.0315663472175,49.2112337693731));
#23530=CARTESIAN_POINT('Ctrl Pts',(40.9053183806479,40.0322815531519,49.2196268548349));
#23531=CARTESIAN_POINT('Ctrl Pts',(40.9081675267248,40.0325783477594,49.2231102491008));
#23532=CARTESIAN_POINT('Ctrl Pts',(40.9146788241066,40.0332516981206,49.2310144247334));
#23533=CARTESIAN_POINT('Ctrl Pts',(40.9183485352365,40.0336276985401,49.2354288520781));
#23534=CARTESIAN_POINT('Ctrl Pts',(40.9284323800113,40.0346516044508,49.2474495138265));
#23535=CARTESIAN_POINT('Ctrl Pts',(40.9348858458118,40.0352967290142,49.2550227389352));
#23536=CARTESIAN_POINT('Ctrl Pts',(40.9682655366456,40.0385840068125,49.2935858449541));
#23537=CARTESIAN_POINT('Ctrl Pts',(40.9961195476466,40.0411641104287,49.3237628743878));
#23538=CARTESIAN_POINT('Ctrl Pts',(41.0402111799009,40.0450498620308,49.3685731225626));
#23539=CARTESIAN_POINT('Ctrl Pts',(41.0557675928957,40.0463854687096,49.3838559603307));
#23540=CARTESIAN_POINT('Ctrl Pts',(41.1468999684066,40.0540324283081,49.4703985701753));
#23541=CARTESIAN_POINT('Ctrl Pts',(41.2278759628396,40.06014924869,49.5357273945426));
#23542=CARTESIAN_POINT('Ctrl Pts',(41.3714815013165,40.0705709040585,49.6335781407554));
#23543=CARTESIAN_POINT('Ctrl Pts',(41.4313346834385,40.0748039198113,49.6697647122206));
#23544=CARTESIAN_POINT('Ctrl Pts',(41.5182463594611,40.0809141772239,49.7160624442938));
#23545=CARTESIAN_POINT('Ctrl Pts',(41.5437717730731,40.0827041644582,49.7289398179383));
#23546=CARTESIAN_POINT('Ctrl Pts',(41.5893784605062,40.0859014441967,49.7506903647484));
#23547=CARTESIAN_POINT('Ctrl Pts',(41.6093429998216,40.0873007461735,49.7597969993163));
#23548=CARTESIAN_POINT('Ctrl Pts',(41.6392824052511,40.0894008182492,49.7728412622097));
#23549=CARTESIAN_POINT('Ctrl Pts',(41.6491422435325,40.0900926830378,49.7770396793133));
#23550=CARTESIAN_POINT('Ctrl Pts',(41.6590906632278,40.0907911564754,49.7811782378637));
#23551=CARTESIAN_POINT('Ctrl Pts',(41.6591449388137,40.0907949671481,49.7812008136845));
#23552=CARTESIAN_POINT('Ctrl Pts',(41.6592566585854,40.090802810984,49.7812472773089));
#23553=CARTESIAN_POINT('Ctrl Pts',(41.659314102755,40.0908068441474,49.7812711647565));
#23554=CARTESIAN_POINT('Ctrl Pts',(41.6594323553904,40.0908151467091,49.7813203319432));
#23555=CARTESIAN_POINT('Ctrl Pts',(41.659493163925,40.0908194161136,49.7813456113183));
#23556=CARTESIAN_POINT('Ctrl Pts',(41.6596183543239,40.0908282058388,49.7813976480581));
#23557=CARTESIAN_POINT('Ctrl Pts',(41.6596827363164,40.0908327261702,49.7814244050346));
#23558=CARTESIAN_POINT('Ctrl Pts',(41.6598152965887,40.0908420334086,49.7814794882868));
#23559=CARTESIAN_POINT('Ctrl Pts',(41.6598834752016,40.0908468203409,49.7815078142043));
#23560=CARTESIAN_POINT('Ctrl Pts',(41.6600238676881,40.0908566775662,49.781566133104));
#23561=CARTESIAN_POINT('Ctrl Pts',(41.6600960816602,40.0908617478683,49.7815961255683));
#23562=CARTESIAN_POINT('Ctrl Pts',(41.6602448002229,40.0908721897694,49.7816578819079));
#23563=CARTESIAN_POINT('Ctrl Pts',(41.6603213048771,40.0908775613753,49.7816896451804));
#23564=CARTESIAN_POINT('Ctrl Pts',(41.6604788776197,40.0908886250471,49.7817550544779));
#23565=CARTESIAN_POINT('Ctrl Pts',(41.6605599460215,40.0908943171379,49.7817886999239));
#23566=CARTESIAN_POINT('Ctrl Pts',(41.6607269381773,40.0909060422848,49.7818579925507));
#23567=CARTESIAN_POINT('Ctrl Pts',(41.6608128624655,40.0909120753818,49.7818936391539));
#23568=CARTESIAN_POINT('Ctrl Pts',(41.660989880056,40.0909245045748,49.7819670617734));
#23569=CARTESIAN_POINT('Ctrl Pts',(41.6610809735456,40.0909309006878,49.7820048369655));
#23570=CARTESIAN_POINT('Ctrl Pts',(41.6612686646559,40.0909440794544,49.7820826529696));
#23571=CARTESIAN_POINT('Ctrl Pts',(41.6613652627393,40.0909508621447,49.7821226929553));
#23572=CARTESIAN_POINT('Ctrl Pts',(41.6615643231018,40.0909648393614,49.7822051846756));
#23573=CARTESIAN_POINT('Ctrl Pts',(41.661666785674,40.090972033913,49.7822476353817));
#23574=CARTESIAN_POINT('Ctrl Pts',(41.6618779607458,40.0909868619517,49.7823351048308));
#23575=CARTESIAN_POINT('Ctrl Pts',(41.6619866737438,40.0909944954791,49.7823801224804));
#23576=CARTESIAN_POINT('Ctrl Pts',(41.6622107635565,40.0910102305483,49.7824728932246));
#23577=CARTESIAN_POINT('Ctrl Pts',(41.6623261410521,40.091018332144,49.7825206451307));
#23578=CARTESIAN_POINT('Ctrl Pts',(41.6625640051157,40.0910350346339,49.7826190641635));
#23579=CARTESIAN_POINT('Ctrl Pts',(41.6626864920904,40.0910436355636,49.7826697297941));
#23580=CARTESIAN_POINT('Ctrl Pts',(41.6629390524401,40.0910613702606,49.7827741686183));
#23581=CARTESIAN_POINT('Ctrl Pts',(41.6630691265414,40.0910705040869,49.7828279402271));
#23582=CARTESIAN_POINT('Ctrl Pts',(41.6633373748465,40.0910893406741,49.7829387975903));
#23583=CARTESIAN_POINT('Ctrl Pts',(41.6634755496589,40.0910990434868,49.7829958814592));
#23584=CARTESIAN_POINT('Ctrl Pts',(41.6637605509215,40.0911190568044,49.7831135846472));
#23585=CARTESIAN_POINT('Ctrl Pts',(41.6639073782758,40.0911293673831,49.7831742019152));
#23586=CARTESIAN_POINT('Ctrl Pts',(41.6642102781484,40.0911506379438,49.7832992095053));
#23587=CARTESIAN_POINT('Ctrl Pts',(41.6643663515719,40.0911615980011,49.7833635974487));
#23588=CARTESIAN_POINT('Ctrl Pts',(41.6646883813852,40.0911842123444,49.7834964010764));
#23589=CARTESIAN_POINT('Ctrl Pts',(41.6648543389566,40.0911958667267,49.7835648141212));
#23590=CARTESIAN_POINT('Ctrl Pts',(41.6651968232844,40.091219917952,49.7837059412464));
#23591=CARTESIAN_POINT('Ctrl Pts',(41.665373351295,40.0912323148981,49.7837786522889));
#23592=CARTESIAN_POINT('Ctrl Pts',(41.6657377140861,40.0912579030969,49.7839286683168));
#23593=CARTESIAN_POINT('Ctrl Pts',(41.665925550341,40.0912710944704,49.7840059698655));
#23594=CARTESIAN_POINT('Ctrl Pts',(41.6662510195833,40.0912939517994,49.7841398523607));
#23595=CARTESIAN_POINT('Ctrl Pts',(41.6663886468353,40.0913036172827,49.7841964470181));
#23596=CARTESIAN_POINT('Ctrl Pts',(41.6667109039363,40.0913262494038,49.7843289210064));
#23597=CARTESIAN_POINT('Ctrl Pts',(41.6668955389595,40.0913392164695,49.7844047875828));
#23598=CARTESIAN_POINT('Ctrl Pts',(41.6673278852495,40.0913695808376,49.7845823603499));
#23599=CARTESIAN_POINT('Ctrl Pts',(41.6675756059249,40.0913869789176,49.7846840436247));
#23600=CARTESIAN_POINT('Ctrl Pts',(41.6681556685602,40.091427718874,49.7849220040277));
#23601=CARTESIAN_POINT('Ctrl Pts',(41.6684880273522,40.091451062144,49.7850582398889));
#23602=CARTESIAN_POINT('Ctrl Pts',(41.6770663736592,40.0920535759897,49.7885717573387));
#23603=CARTESIAN_POINT('Ctrl Pts',(41.6853355055779,40.0926346680125,49.7918919094512));
#23604=CARTESIAN_POINT('Ctrl Pts',(41.7042683260003,40.0939659451399,49.7993417573945));
#23605=CARTESIAN_POINT('Ctrl Pts',(41.7149462439636,40.094717363842,49.803434130722));
#23606=CARTESIAN_POINT('Ctrl Pts',(41.7480799877713,40.0970512031551,49.815796104629));
#23607=CARTESIAN_POINT('Ctrl Pts',(41.7706530473724,40.098644282232,49.8237427234191));
#23608=CARTESIAN_POINT('Ctrl Pts',(41.793624421975,40.1002692745907,49.8313523114559));
#23609=CARTESIAN_POINT('Ctrl Pts',(41.7938816187901,40.1002874691372,49.8314374513637));
#23610=CARTESIAN_POINT('Ctrl Pts',(41.7941388318207,40.1003056653051,49.8315225365232));
#23611=CARTESIAN_POINT('',(40.4728302759175,40.1150077701205,48.0014409743479));
#23612=CARTESIAN_POINT('Ctrl Pts',(41.7933319732428,40.273017144546,49.8339081536803));
#23613=CARTESIAN_POINT('Ctrl Pts',(41.2437298911391,40.2348813997253,49.6477812220981));
#23614=CARTESIAN_POINT('Ctrl Pts',(40.6001596419136,40.1822116082501,49.0283757153127));
#23615=CARTESIAN_POINT('Ctrl Pts',(40.471311607613,40.1295418167751,48.2239035093802));
#23616=CARTESIAN_POINT('Ctrl Pts',(40.4728302759175,40.1150077701205,48.0014409743479));
#23617=CARTESIAN_POINT('Ctrl Pts',(40.4708704789563,40.1161353185692,48.0013593887718));
#23618=CARTESIAN_POINT('Ctrl Pts',(40.4708380686763,40.1133347529338,47.9553654617617));
#23619=CARTESIAN_POINT('Ctrl Pts',(40.4724505230042,40.1105018024918,47.9093871381568));
#23620=CARTESIAN_POINT('Ctrl Pts',(40.4776042865313,40.1059406866609,47.8367260892297));
#23621=CARTESIAN_POINT('Ctrl Pts',(40.480063172739,40.1042439796843,47.8099838988324));
#23622=CARTESIAN_POINT('Ctrl Pts',(40.4843588666476,40.101803077152,47.7719838627056));
#23623=CARTESIAN_POINT('Ctrl Pts',(40.485738604911,40.1010729939168,47.7606767605226));
#23624=CARTESIAN_POINT('Ctrl Pts',(40.4883527066305,40.0997777399369,47.7407251993612));
#23625=CARTESIAN_POINT('Ctrl Pts',(40.4895457866756,40.0992138735614,47.7320755868885));
#23626=CARTESIAN_POINT('Ctrl Pts',(40.4920182108331,40.0980964698556,47.7150078105216));
#23627=CARTESIAN_POINT('Ctrl Pts',(40.4932946517388,40.0975430361036,47.7065894227091));
#23628=CARTESIAN_POINT('Ctrl Pts',(40.4961311359064,40.0963608234212,47.6886828600618));
#23629=CARTESIAN_POINT('Ctrl Pts',(40.4977064673102,40.0957315726104,47.6791973767437));
#23630=CARTESIAN_POINT('Ctrl Pts',(40.5019505023879,40.0941034184224,47.6547741086693));
#23631=CARTESIAN_POINT('Ctrl Pts',(40.5047246192555,40.093101187367,47.6398555566224));
#23632=CARTESIAN_POINT('Ctrl Pts',(40.516659863959,40.0890232439818,47.5796324594816));
#23633=CARTESIAN_POINT('Ctrl Pts',(40.5272711802967,40.0859018538545,47.5346344585295));
#23634=CARTESIAN_POINT('Ctrl Pts',(40.558779960203,40.0777290546985,47.4196739905426));
#23635=CARTESIAN_POINT('Ctrl Pts',(40.5820499012658,40.0726115679466,47.3504424002996));
#23636=CARTESIAN_POINT('Ctrl Pts',(40.662055976507,40.0573393182124,47.1506982591026));
#23637=CARTESIAN_POINT('Ctrl Pts',(40.7293622893511,40.0470279472954,47.0249433346778));
#23638=CARTESIAN_POINT('Ctrl Pts',(40.8217736054067,40.0358554383224,46.8904121543121));
#23639=CARTESIAN_POINT('Ctrl Pts',(40.8339488644304,40.0344316920863,46.8732934410902));
#23640=CARTESIAN_POINT('Ctrl Pts',(40.8509325406227,40.0325136301454,46.8502213378908));
#23641=CARTESIAN_POINT('Ctrl Pts',(40.8554998181267,40.032004272587,46.8440933607709));
#23642=CARTESIAN_POINT('Ctrl Pts',(40.8632219050962,40.0311540398518,46.8338600228404));
#23643=CARTESIAN_POINT('Ctrl Pts',(40.8663570053764,40.0308118272764,46.8297399748523));
#23644=CARTESIAN_POINT('Ctrl Pts',(40.8723560676635,40.0301627088197,46.8219217129795));
#23645=CARTESIAN_POINT('Ctrl Pts',(40.8752169423016,40.0298555843619,46.8182212294692));
#23646=CARTESIAN_POINT('Ctrl Pts',(40.882062693014,40.0291263360085,46.8094326328191));
#23647=CARTESIAN_POINT('Ctrl Pts',(40.8860597656042,40.0287050652564,46.8043540267516));
#23648=CARTESIAN_POINT('Ctrl Pts',(40.900360758893,40.0272133944104,46.7863701494729));
#23649=CARTESIAN_POINT('Ctrl Pts',(40.9108051222076,40.0261524203982,46.7735767747563));
#23650=CARTESIAN_POINT('Ctrl Pts',(40.9846375109812,40.0188343754772,46.6854731063218));
#23651=CARTESIAN_POINT('Ctrl Pts',(41.053552377494,40.0129146061821,46.614967268689));
#23652=CARTESIAN_POINT('Ctrl Pts',(41.1920313682759,40.0019065625327,46.4934434472128));
#23653=CARTESIAN_POINT('Ctrl Pts',(41.2602072208809,39.9968211917294,46.4412271586212));
#23654=CARTESIAN_POINT('Ctrl Pts',(41.3749780756536,39.9884664598837,46.3648905178379));
#23655=CARTESIAN_POINT('Ctrl Pts',(41.4194734034244,39.9852736659388,46.3378267373196));
#23656=CARTESIAN_POINT('Ctrl Pts',(41.4855843287958,39.9805518435421,46.3011945375382));
#23657=CARTESIAN_POINT('Ctrl Pts',(41.5063683849867,39.9790705496073,46.2901700425527));
#23658=CARTESIAN_POINT('Ctrl Pts',(41.5394708728636,39.9767129709179,46.2733799069669));
#23659=CARTESIAN_POINT('Ctrl Pts',(41.5516579478092,39.9758453559421,46.2673595087847));
#23660=CARTESIAN_POINT('Ctrl Pts',(41.5747992725415,39.9741979302012,46.2562304087504));
#23661=CARTESIAN_POINT('Ctrl Pts',(41.5857399356248,39.9734190831801,46.2510948668921));
#23662=CARTESIAN_POINT('Ctrl Pts',(41.6048147607361,39.9720608572839,46.2423589371548));
#23663=CARTESIAN_POINT('Ctrl Pts',(41.6129269920797,39.9714831252402,46.2387113393016));
#23664=CARTESIAN_POINT('Ctrl Pts',(41.6286764237479,39.9703611653448,46.2317602725213));
#23665=CARTESIAN_POINT('Ctrl Pts',(41.6363103561749,39.9698171913481,46.2284498546886));
#23666=CARTESIAN_POINT('Ctrl Pts',(41.6563075030613,39.9683917345989,46.2199314629391));
#23667=CARTESIAN_POINT('Ctrl Pts',(41.6687038713394,39.9675075731117,46.2148029567246));
#23668=CARTESIAN_POINT('Ctrl Pts',(41.7121333162006,39.9644076366284,46.1973639978971));
#23669=CARTESIAN_POINT('Ctrl Pts',(41.7434301193798,39.9621694017786,46.1857307570226));
#23670=CARTESIAN_POINT('Ctrl Pts',(41.9201550575998,39.9494995049822,46.1252124088615));
#23671=CARTESIAN_POINT('Ctrl Pts',(42.0706886883256,39.9385275372414,46.0930081611002));
#23672=CARTESIAN_POINT('Ctrl Pts',(42.2369739080843,39.9266172723342,46.0777225612502));
#23673=CARTESIAN_POINT('Ctrl Pts',(42.2505495367126,39.9256469141815,46.0766194805214));
#23674=CARTESIAN_POINT('Ctrl Pts',(42.3428892935131,39.9190639442161,46.0701000149224));
#23675=CARTESIAN_POINT('Ctrl Pts',(42.4219196440293,39.9135122025576,46.0693788444267));
#23676=CARTESIAN_POINT('Ctrl Pts',(42.5120246297948,39.9074238000866,46.0740924661395));
#23677=CARTESIAN_POINT('Ctrl Pts',(42.5232643190722,39.906668692889,46.0747791635083));
#23678=CARTESIAN_POINT('Ctrl Pts',(42.5404457227236,39.9055217293803,46.075979961664));
#23679=CARTESIAN_POINT('Ctrl Pts',(42.5463919084768,39.9051261281493,46.0764232480964));
#23680=CARTESIAN_POINT('Ctrl Pts',(42.55729477516,39.904403339198,46.0772869028557));
#23681=CARTESIAN_POINT('Ctrl Pts',(42.5622518960863,39.9040757063069,46.0776988728193));
#23682=CARTESIAN_POINT('Ctrl Pts',(42.5734610277722,39.9033370679969,46.0786740956611));
#23683=CARTESIAN_POINT('Ctrl Pts',(42.5797119171643,39.9029267009378,46.0792486916809));
#23684=CARTESIAN_POINT('Ctrl Pts',(42.5958978742643,39.9018678407538,46.0808162496946));
#23685=CARTESIAN_POINT('Ctrl Pts',(42.6058283833303,39.9012218542597,46.081855862707));
#23686=CARTESIAN_POINT('Ctrl Pts',(42.6735305633519,39.8968399712864,46.0894753612223));
#23687=CARTESIAN_POINT('Ctrl Pts',(42.7309932505305,39.8932308825393,46.0985878257651));
#23688=CARTESIAN_POINT('Ctrl Pts',(42.8329844938905,39.886883859484,46.1195268028226));
#23689=CARTESIAN_POINT('Ctrl Pts',(42.8776639593492,39.8841240645453,46.1303763837589));
#23690=CARTESIAN_POINT('Ctrl Pts',(43.0308717896726,39.874609742797,46.1734314810836));
#23691=CARTESIAN_POINT('Ctrl Pts',(43.1369170989435,39.8679205080747,46.2135780262212));
#23692=CARTESIAN_POINT('Ctrl Pts',(43.2904295826289,39.857456421598,46.287702987494));
#23693=CARTESIAN_POINT('Ctrl Pts',(43.3408895045421,39.853881560762,46.3149030070584));
#23694=CARTESIAN_POINT('Ctrl Pts',(43.4035980647876,39.8492206594647,46.3524010616639));
#23695=CARTESIAN_POINT('Ctrl Pts',(43.4170350706918,39.8482087111747,46.360661420472));
#23696=CARTESIAN_POINT('Ctrl Pts',(43.4386080599026,39.8465617064191,46.3742906680056));
#23697=CARTESIAN_POINT('Ctrl Pts',(43.4468074672948,39.8459304081136,46.3795581914682));
#23698=CARTESIAN_POINT('Ctrl Pts',(43.4624532356056,39.8447153774266,46.389777765402));
#23699=CARTESIAN_POINT('Ctrl Pts',(43.4699057826619,39.8441320270595,46.3947199202883));
#23700=CARTESIAN_POINT('Ctrl Pts',(43.4868641682392,39.8427939044853,46.4061364201039));
#23701=CARTESIAN_POINT('Ctrl Pts',(43.4963469330379,39.8420378757616,46.4126442666584));
#23702=CARTESIAN_POINT('Ctrl Pts',(43.5262238119617,39.8396307198262,46.4335436467429));
#23703=CARTESIAN_POINT('Ctrl Pts',(43.5463963894135,39.8379677574257,46.4482458957952));
#23704=CARTESIAN_POINT('Ctrl Pts',(43.6801558865336,39.8266790944768,46.5497648616212));
#23705=CARTESIAN_POINT('Ctrl Pts',(43.7840536772881,39.816565033277,46.6485704291856));
#23706=CARTESIAN_POINT('Ctrl Pts',(43.8985986243681,39.8038559302602,46.7846937843164));
#23707=CARTESIAN_POINT('Ctrl Pts',(43.9203963046694,39.8013554931575,46.8120765354504));
#23708=CARTESIAN_POINT('Ctrl Pts',(43.9900313651473,39.7931155584811,46.9046123326988));
#23709=CARTESIAN_POINT('Ctrl Pts',(44.0345256058119,39.7874271401505,46.9721853214095));
#23710=CARTESIAN_POINT('Ctrl Pts',(44.0802638157801,39.7812094070985,47.052168896266));
#23711=CARTESIAN_POINT('Ctrl Pts',(44.0857880920703,39.7804514458512,47.0620294164645));
#23712=CARTESIAN_POINT('Ctrl Pts',(44.094098229957,39.7793010665626,47.0771731467608));
#23713=CARTESIAN_POINT('Ctrl Pts',(44.0969466365806,39.7789048701243,47.0824214863061));
#23714=CARTESIAN_POINT('Ctrl Pts',(44.1021228515544,39.7781815145435,47.0920654795095));
#23715=CARTESIAN_POINT('Ctrl Pts',(44.1044580368625,39.777853905374,47.0964569202328));
#23716=CARTESIAN_POINT('Ctrl Pts',(44.1096970795922,39.7771159690502,47.1064018111144));
#23717=CARTESIAN_POINT('Ctrl Pts',(44.1125908776776,39.7767062747462,47.1119604087828));
#23718=CARTESIAN_POINT('Ctrl Pts',(44.1200089315979,39.7756503254396,47.1263806175873));
#23719=CARTESIAN_POINT('Ctrl Pts',(44.124491876757,39.7750065542618,47.1352634347741));
#23720=CARTESIAN_POINT('Ctrl Pts',(44.1543135600822,39.770682706301,47.1955085021706));
#23721=CARTESIAN_POINT('Ctrl Pts',(44.1774255081934,39.7671256235491,47.2479477623848));
#23722=CARTESIAN_POINT('Ctrl Pts',(44.2146037969928,39.7608639049724,47.3436355463144));
#23723=CARTESIAN_POINT('Ctrl Pts',(44.2295394843348,39.758137845114,47.386496279672));
#23724=CARTESIAN_POINT('Ctrl Pts',(44.2767446232207,39.7485859166721,47.5390806858801));
#23725=CARTESIAN_POINT('Ctrl Pts',(44.3007586060393,39.7418317044264,47.6510984688772));
#23726=CARTESIAN_POINT('Ctrl Pts',(44.3217420361472,39.7312792228694,47.8217611548666));
#23727=CARTESIAN_POINT('Ctrl Pts',(44.326206988774,39.7276856069946,47.8792225341522));
#23728=CARTESIAN_POINT('Ctrl Pts',(44.3286119373994,39.7230033882651,47.9525849827165));
#23729=CARTESIAN_POINT('Ctrl Pts',(44.3289355724879,39.721989739491,47.9683816175594));
#23730=CARTESIAN_POINT('Ctrl Pts',(44.3291451006418,39.7203406462953,47.993931260495));
#23731=CARTESIAN_POINT('Ctrl Pts',(44.3291511294837,39.7197089779125,48.0036827604339));
#23732=CARTESIAN_POINT('Ctrl Pts',(44.3290209665491,39.7184936963109,48.0223741400859));
#23733=CARTESIAN_POINT('Ctrl Pts',(44.3288965572465,39.7179104686639,48.0313138695423));
#23734=CARTESIAN_POINT('Ctrl Pts',(44.3284702899616,39.7165732777726,48.051738696733));
#23735=CARTESIAN_POINT('Ctrl Pts',(44.3281279665236,39.7158180640398,48.0632225195437));
#23736=CARTESIAN_POINT('Ctrl Pts',(44.3267191239553,39.7134161752024,48.0995774735461));
#23737=CARTESIAN_POINT('Ctrl Pts',(44.3252737995631,39.7117577381274,48.1244305173558));
#23738=CARTESIAN_POINT('Ctrl Pts',(44.3121934537165,39.7003925155832,48.2929963390269));
#23739=CARTESIAN_POINT('Ctrl Pts',(44.2849607637538,39.6901879564356,48.4350156825309));
#23740=CARTESIAN_POINT('Ctrl Pts',(44.2090952952734,39.6719299524125,48.6790706088753));
#23741=CARTESIAN_POINT('Ctrl Pts',(44.1668501527213,39.6639626757688,48.7824374944683));
#23742=CARTESIAN_POINT('Ctrl Pts',(44.1098094001838,39.6555095117496,48.8934610254329));
#23743=CARTESIAN_POINT('Ctrl Pts',(44.1035851536705,39.654611768955,48.9052725763823));
#23744=CARTESIAN_POINT('Ctrl Pts',(44.0942040922014,39.6532954859621,48.9226352484668));
#23745=CARTESIAN_POINT('Ctrl Pts',(44.0911416936151,39.6528713708583,48.9282365446162));
#23746=CARTESIAN_POINT('Ctrl Pts',(44.0856404833439,39.6521194829628,48.9381809664632));
#23747=CARTESIAN_POINT('Ctrl Pts',(44.083212600403,39.6517910381102,48.9425299510779));
#23748=CARTESIAN_POINT('Ctrl Pts',(44.0778823967139,39.6510773235496,48.9519914802742));
#23749=CARTESIAN_POINT('Ctrl Pts',(44.0749735385761,39.6506924778185,48.9571001844423));
#23750=CARTESIAN_POINT('Ctrl Pts',(44.0667728298719,39.6496201861095,48.9713508460675));
#23751=CARTESIAN_POINT('Ctrl Pts',(44.061429084704,39.6489359713391,48.9804629219373));
#23752=CARTESIAN_POINT('Ctrl Pts',(44.0299491234931,39.6449856312155,49.033145612655));
#23753=CARTESIAN_POINT('Ctrl Pts',(44.0021721767424,39.6418153969879,49.0757180458397));
#23754=CARTESIAN_POINT('Ctrl Pts',(43.8735284995272,39.6281992354596,49.2568253026773));
#23755=CARTESIAN_POINT('Ctrl Pts',(43.7561479631914,39.6183225634696,49.3826660682542));
#23756=CARTESIAN_POINT('Ctrl Pts',(43.5960456342671,39.6055800605953,49.5140328656471));
#23757=CARTESIAN_POINT('Ctrl Pts',(43.5677840085502,39.6033572793829,49.5359365082439));
#23758=CARTESIAN_POINT('Ctrl Pts',(43.5177101487212,39.5994493960218,49.5725641084382));
#23759=CARTESIAN_POINT('Ctrl Pts',(43.4961746749687,39.5977780538879,49.5876507258598));
#23760=CARTESIAN_POINT('Ctrl Pts',(43.4644813066983,39.5953280154655,49.6089011618202));
#23761=CARTESIAN_POINT('Ctrl Pts',(43.4545636135286,39.5945626785039,49.615419133067));
#23762=CARTESIAN_POINT('Ctrl Pts',(43.4370480333845,39.5932130366146,49.6267004450533));
#23763=CARTESIAN_POINT('Ctrl Pts',(43.429475823536,39.5926302211794,49.6315031368898));
#23764=CARTESIAN_POINT('Ctrl Pts',(43.4136684988975,39.5914147710388,49.6413751071379));
#23765=CARTESIAN_POINT('Ctrl Pts',(43.4054282165221,39.5907818328079,49.646435593526));
#23766=CARTESIAN_POINT('Ctrl Pts',(43.3839448822949,39.5891332265844,49.6594074208124));
#23767=CARTESIAN_POINT('Ctrl Pts',(43.3706445780308,39.588114069993,49.6672221205236));
#23768=CARTESIAN_POINT('Ctrl Pts',(43.3152532414906,39.5838747655288,49.6988802705821));
#23769=CARTESIAN_POINT('Ctrl Pts',(43.2723696561869,39.5806042569261,49.7212940326191));
#23770=CARTESIAN_POINT('Ctrl Pts',(43.0876736738055,39.5665578581451,49.8091527426551));
#23771=CARTESIAN_POINT('Ctrl Pts',(42.9390435451542,39.5552871755764,49.8588565344614));
#23772=CARTESIAN_POINT('Ctrl Pts',(42.7388802085037,39.540796999496,49.899743108681));
#23773=CARTESIAN_POINT('Ctrl Pts',(42.691329001164,39.5374092627518,49.9076141402746));
#23774=CARTESIAN_POINT('Ctrl Pts',(42.6251777098498,39.5328111103733,49.9160323115752));
#23775=CARTESIAN_POINT('Ctrl Pts',(42.60679195547,39.5315453356662,49.9181037413716));
#23776=CARTESIAN_POINT('Ctrl Pts',(42.5747613362871,39.5293645275621,49.9212465342048));
#23777=CARTESIAN_POINT('Ctrl Pts',(42.5611298369547,39.5284440724283,49.9224377679704));
#23778=CARTESIAN_POINT('Ctrl Pts',(42.5410579681312,39.527101091732,49.923976812116));
#23779=CARTESIAN_POINT('Ctrl Pts',(42.5346270411319,39.526672670391,49.9244374987805));
#23780=CARTESIAN_POINT('Ctrl Pts',(42.5232639473802,39.5259191056261,49.9251942674772));
#23781=CARTESIAN_POINT('Ctrl Pts',(42.5183328193101,39.5255932366131,49.9255036520611));
#23782=CARTESIAN_POINT('Ctrl Pts',(42.507596149151,39.5248862349984,49.9261358808473));
#23783=CARTESIAN_POINT('Ctrl Pts',(42.5017903092753,39.5245055109469,49.926451426312));
#23784=CARTESIAN_POINT('Ctrl Pts',(42.4857177506217,39.5234557047476,49.9272521012426));
#23785=CARTESIAN_POINT('Ctrl Pts',(42.4754482663264,39.5227896413108,49.9276814479935));
#23786=CARTESIAN_POINT('Ctrl Pts',(42.4193470767905,39.519174289965,49.9295779067254));
#23787=CARTESIAN_POINT('Ctrl Pts',(42.3734737023976,39.5163027972602,49.9294927621431));
#23788=CARTESIAN_POINT('Ctrl Pts',(42.2160620065461,39.5066081559006,49.9235844778319));
#23789=CARTESIAN_POINT('Ctrl Pts',(42.1050481183819,39.5000351013078,49.9097165252285));
#23790=CARTESIAN_POINT('Ctrl Pts',(41.9276400629401,39.4891781157111,49.871706447512));
#23791=CARTESIAN_POINT('Ctrl Pts',(41.8603051399067,39.4849734388322,49.8534101226387));
#23792=CARTESIAN_POINT('Ctrl Pts',(41.7941386883808,39.4806729614233,49.8315224890738));
#23793=CARTESIAN_POINT('Origin',(42.4,48.4493818343519,48.));
#23794=CARTESIAN_POINT('',(41.7941388317924,38.5145390814761,49.8315225365138));
#23795=CARTESIAN_POINT('',(41.7941383335288,38.6866921868075,49.8315223716899));
#23796=CARTESIAN_POINT('',(41.7941388317924,48.4493818343519,49.8315225365138));
#23797=CARTESIAN_POINT('',(40.4705489998756,39.1502182104393,47.9997072692622));
#23798=CARTESIAN_POINT('Ctrl Pts',(40.4708700223059,39.1502181656481,47.9997066371674));
#23799=CARTESIAN_POINT('Ctrl Pts',(40.4708724067228,39.1491850444138,47.9840269063358));
#23800=CARTESIAN_POINT('Ctrl Pts',(40.4710659517807,39.1481519231795,47.9683488185713));
#23801=CARTESIAN_POINT('Ctrl Pts',(40.4714505599335,39.1471188019453,47.9526754385228));
#23802=CARTESIAN_POINT('Ctrl Pts',(40.4731094555565,39.1426627333953,47.885072863346));
#23803=CARTESIAN_POINT('Ctrl Pts',(40.4783305474797,39.1382066648452,47.8174223947577));
#23804=CARTESIAN_POINT('Ctrl Pts',(40.4871205945074,39.1337505962952,47.7501301599985));
#23805=CARTESIAN_POINT('Ctrl Pts',(40.4958973182547,39.1293012819128,47.6829399216579));
#23806=CARTESIAN_POINT('Ctrl Pts',(40.5082321983288,39.1248519675304,47.6161073251916));
#23807=CARTESIAN_POINT('Ctrl Pts',(40.5240800039167,39.120402653148,47.5500369735246));
#23808=CARTESIAN_POINT('Ctrl Pts',(40.5399090630196,39.1159586018922,47.4840447769595));
#23809=CARTESIAN_POINT('Ctrl Pts',(40.5592426806972,39.1115145506363,47.4188135124089));
#23810=CARTESIAN_POINT('Ctrl Pts',(40.581984273194,39.1070704993804,47.3547392976586));
#23811=CARTESIAN_POINT('Ctrl Pts',(40.6047115389767,39.1026292477812,47.2907054482854));
#23812=CARTESIAN_POINT('Ctrl Pts',(40.6308423562216,39.098187996182,47.2278276671201));
#23813=CARTESIAN_POINT('Ctrl Pts',(40.6602302766802,39.0937467445828,47.1664870326626));
#23814=CARTESIAN_POINT('Ctrl Pts',(40.6896098416771,39.0893067557033,47.1051638383406));
#23815=CARTESIAN_POINT('Ctrl Pts',(40.7222444583952,39.0848667668239,47.045377368246));
#23816=CARTESIAN_POINT('Ctrl Pts',(40.7579402462904,39.0804267779444,46.9874871249474));
#23817=CARTESIAN_POINT('Ctrl Pts',(40.7936382236088,39.0759865167355,46.9295933309152));
#23818=CARTESIAN_POINT('Ctrl Pts',(40.832397483487,39.0715462555265,46.8735964134657));
#23819=CARTESIAN_POINT('Ctrl Pts',(40.8739800198014,39.0671059943176,46.8198281578793));
#23820=CARTESIAN_POINT('Ctrl Pts',(40.9156071642824,39.062660969765,46.7660022217491));
#23821=CARTESIAN_POINT('Ctrl Pts',(40.9600633266848,39.0582159452124,46.7144101099497));
#23822=CARTESIAN_POINT('Ctrl Pts',(41.0070699251909,39.0537709206598,46.665350846255));
#23823=CARTESIAN_POINT('Ctrl Pts',(41.054104956129,39.0493232074877,46.6162619085522));
#23824=CARTESIAN_POINT('Ctrl Pts',(41.1036931331262,39.0448754943155,46.5697092057024));
#23825=CARTESIAN_POINT('Ctrl Pts',(41.1555207669375,39.0404277811434,46.5259531909141));
#23826=CARTESIAN_POINT('Ctrl Pts',(41.207438295423,39.0359723534434,46.4821212816194));
#23827=CARTESIAN_POINT('Ctrl Pts',(41.2616026394671,39.0315169257434,46.4410960392844));
#23828=CARTESIAN_POINT('Ctrl Pts',(41.3176697199394,39.0270614980434,46.4030955815191));
#23829=CARTESIAN_POINT('Ctrl Pts',(41.3435442533007,39.0250053518754,46.3855586578214));
#23830=CARTESIAN_POINT('Ctrl Pts',(41.3698236599141,39.0229492057074,46.3686653037414));
#23831=CARTESIAN_POINT('Ctrl Pts',(41.3964724507869,39.0208930595394,46.3524336083573));
#23832=CARTESIAN_POINT('Ctrl Pts',(41.4542255622892,39.0164369909894,46.3172563683145));
#23833=CARTESIAN_POINT('Ctrl Pts',(41.5139460713761,39.0119809224394,46.2850491254104));
#23834=CARTESIAN_POINT('Ctrl Pts',(41.5752960700954,39.0075248538894,46.2560372753697));
#23835=CARTESIAN_POINT('Ctrl Pts',(41.6365530791826,39.003075539507,46.2270693992707));
#23836=CARTESIAN_POINT('Ctrl Pts',(41.6994342337059,38.9986262251246,46.2012875137176));
#23837=CARTESIAN_POINT('Ctrl Pts',(41.7635747817648,38.9941769107422,46.1788724650661));
#23838=CARTESIAN_POINT('Ctrl Pts',(41.8276394575007,38.9897328594863,46.1564839313395));
#23839=CARTESIAN_POINT('Ctrl Pts',(41.892960104418,38.9852888082304,46.1374544874787));
#23840=CARTESIAN_POINT('Ctrl Pts',(41.9591513253518,38.9808447569745,46.121917200185));
#23841=CARTESIAN_POINT('Ctrl Pts',(42.0253008472402,38.9764035053753,46.1063897010481));
#23842=CARTESIAN_POINT('Ctrl Pts',(42.0923193756932,38.9719622537761,46.0943501072782));
#23843=CARTESIAN_POINT('Ctrl Pts',(42.1598071857408,38.9675210021769,46.0858814120128));
#23844=CARTESIAN_POINT('Ctrl Pts',(42.2272758079114,38.9630810132975,46.0774151245345));
#23845=CARTESIAN_POINT('Ctrl Pts',(42.2952129571544,38.958641024418,46.0725177816399));
#23846=CARTESIAN_POINT('Ctrl Pts',(42.3632113939956,38.9542010355385,46.0712208121798));
#23847=CARTESIAN_POINT('Ctrl Pts',(42.4312140015627,38.9497607743296,46.0699237631693));
#23848=CARTESIAN_POINT('Ctrl Pts',(42.4992774104961,38.9453205131207,46.0722275327985));
#23849=CARTESIAN_POINT('Ctrl Pts',(42.5669938207757,38.9408802519118,46.07811144425));
#23850=CARTESIAN_POINT('Ctrl Pts',(42.6347828746501,38.9364352273592,46.0840016677385));
#23851=CARTESIAN_POINT('Ctrl Pts',(42.7022236941851,38.9319902028066,46.0934796546508));
#23852=CARTESIAN_POINT('Ctrl Pts',(42.768914081602,38.927545178254,46.1064728791761));
#23853=CARTESIAN_POINT('Ctrl Pts',(42.8356448073962,38.9230974650819,46.1194739627889));
#23854=CARTESIAN_POINT('Ctrl Pts',(42.9016237187846,38.9186497519098,46.1359943953654));
#23855=CARTESIAN_POINT('Ctrl Pts',(42.9664620640971,38.9142020387376,46.1559112584155));
#23856=CARTESIAN_POINT('Ctrl Pts',(43.0314128710733,38.9097466110376,46.1758626671275));
#23857=CARTESIAN_POINT('Ctrl Pts',(43.0952187004583,38.9052911833376,46.1992220937228));
#23858=CARTESIAN_POINT('Ctrl Pts',(43.1575099653391,38.9008357556376,46.2258181577663));
#23859=CARTESIAN_POINT('Ctrl Pts',(43.1862569127051,38.8987796094696,46.238092040062));
#23860=CARTESIAN_POINT('Ctrl Pts',(43.2146816329436,38.8967234633016,46.251054597812));
#23861=CARTESIAN_POINT('Ctrl Pts',(43.2427497133888,38.8946673171336,46.2646857698149));
#23862=CARTESIAN_POINT('Ctrl Pts',(43.3035787013652,38.8902112485836,46.2942271700357));
#23863=CARTESIAN_POINT('Ctrl Pts',(43.3629741837397,38.8857551800335,46.3270299500181));
#23864=CARTESIAN_POINT('Ctrl Pts',(43.4205637910556,38.8812991114835,46.3629318568593));
#23865=CARTESIAN_POINT('Ctrl Pts',(43.4780661084529,38.8768497971011,46.3987793463382));
#23866=CARTESIAN_POINT('Ctrl Pts',(43.5337675672398,38.8724004827187,46.437716381483));
#23867=CARTESIAN_POINT('Ctrl Pts',(43.5873187428817,38.8679511683363,46.4795340320475));
#23868=CARTESIAN_POINT('Ctrl Pts',(43.6408065724465,38.8635071170805,46.5213022162074));
#23869=CARTESIAN_POINT('Ctrl Pts',(43.6921487828764,38.8590630658246,46.5659439464106));
#23870=CARTESIAN_POINT('Ctrl Pts',(43.7410249647544,38.8546190145687,46.6132070807775));
#23871=CARTESIAN_POINT('Ctrl Pts',(43.7898703556891,38.8501777629695,46.6604404403864));
#23872=CARTESIAN_POINT('Ctrl Pts',(43.8362524454727,38.8457365113703,46.7102915860248));
#23873=CARTESIAN_POINT('Ctrl Pts',(43.8798851867402,38.8412952597711,46.7624692363553));
#23874=CARTESIAN_POINT('Ctrl Pts',(43.9235055225129,38.8368552708916,46.814632051735));
#23875=CARTESIAN_POINT('Ctrl Pts',(43.9643777448819,38.8324152820121,46.8691196801779));
#23876=CARTESIAN_POINT('Ctrl Pts',(44.0022551082116,38.8279752931327,46.925606624597));
#23877=CARTESIAN_POINT('Ctrl Pts',(44.0401347947727,38.8235350319238,46.9820970336777));
#23878=CARTESIAN_POINT('Ctrl Pts',(44.0750189848174,38.8190947707148,47.0405865906522));
#23879=CARTESIAN_POINT('Ctrl Pts',(44.106704451789,38.8146545095059,47.1007211382761));
#23880=CARTESIAN_POINT('Ctrl Pts',(44.138423909727,38.8102094849533,47.1609201959602));
#23881=CARTESIAN_POINT('Ctrl Pts',(44.1669375661157,38.8057644604007,47.2227673282688));
#23882=CARTESIAN_POINT('Ctrl Pts',(44.1920888316226,38.8013194358481,47.2858850397355));
#23883=CARTESIAN_POINT('Ctrl Pts',(44.217255310135,38.796871722676,47.349040928609));
#23884=CARTESIAN_POINT('Ctrl Pts',(44.2390551921984,38.7924240095039,47.4134684583036));
#23885=CARTESIAN_POINT('Ctrl Pts',(44.2573815443677,38.7879762963317,47.4787741798967));
#23886=CARTESIAN_POINT('Ctrl Pts',(44.2757396834686,38.7835208686317,47.5441931738144));
#23887=CARTESIAN_POINT('Ctrl Pts',(44.2906121607465,38.7790654409317,47.6104929181125));
#23888=CARTESIAN_POINT('Ctrl Pts',(44.3019431685829,38.7746100132317,47.6772698644672));
#23889=CARTESIAN_POINT('Ctrl Pts',(44.3071723429542,38.7725538670637,47.7080869198887));
#23890=CARTESIAN_POINT('Ctrl Pts',(44.3116479998062,38.7704977208957,47.7390055408118));
#23891=CARTESIAN_POINT('Ctrl Pts',(44.3153683942132,38.7684415747277,47.7699859322796));
#23892=CARTESIAN_POINT('Ctrl Pts',(44.323431212299,38.7639855061777,47.8371264645216));
#23893=CARTESIAN_POINT('Ctrl Pts',(44.3279756041396,38.7595294376277,47.9048257570133));
#23894=CARTESIAN_POINT('Ctrl Pts',(44.3289365802731,38.7550733690777,47.9726828591508));
#23895=CARTESIAN_POINT('Ctrl Pts',(44.3298960998326,38.7506240546953,48.040437108687));
#23896=CARTESIAN_POINT('Ctrl Pts',(44.3272829755928,38.7461747403129,48.108348203499));
#23897=CARTESIAN_POINT('Ctrl Pts',(44.3210838880556,38.7417254259305,48.1760092382609));
#23898=CARTESIAN_POINT('Ctrl Pts',(44.3148921334643,38.7372813746746,48.2435902362903));
#23899=CARTESIAN_POINT('Ctrl Pts',(44.3051228843093,38.7328373234187,48.3109212723607));
#23900=CARTESIAN_POINT('Ctrl Pts',(44.2918148602202,38.7283932721628,48.3775964665486));
#23901=CARTESIAN_POINT('Ctrl Pts',(44.2785152199001,38.7239520205636,48.4442296567984));
#23902=CARTESIAN_POINT('Ctrl Pts',(44.2616813230989,38.7195107689644,48.5102073416065));
#23903=CARTESIAN_POINT('Ctrl Pts',(44.2414033964069,38.7150695173652,48.5751313663862));
#23904=CARTESIAN_POINT('Ctrl Pts',(44.2211312350577,38.7106295284858,48.6400369322145));
#23905=CARTESIAN_POINT('Ctrl Pts',(44.1974171347102,38.7061895396063,48.7038889616217));
#23906=CARTESIAN_POINT('Ctrl Pts',(44.1704013602613,38.7017495507268,48.7663038434492));
#23907=CARTESIAN_POINT('Ctrl Pts',(44.1433839287832,38.6973092895179,48.8287225535319));
#23908=CARTESIAN_POINT('Ctrl Pts',(44.113064619696,38.692869028309,48.8897034889676));
#23909=CARTESIAN_POINT('Ctrl Pts',(44.0796313453446,38.6884287671001,48.9488841344632));
#23910=CARTESIAN_POINT('Ctrl Pts',(44.0461622050455,38.6839837425475,49.0081282667091));
#23911=CARTESIAN_POINT('Ctrl Pts',(44.0095726763772,38.6795387179949,49.0655678242221));
#23912=CARTESIAN_POINT('Ctrl Pts',(43.9700955301258,38.6750936934423,49.1208668891439));
#23913=CARTESIAN_POINT('Ctrl Pts',(43.9305945057102,38.6706459802702,49.1761994022826));
#23914=CARTESIAN_POINT('Ctrl Pts',(43.8882026956471,38.6661982670981,49.2293884601807));
#23915=CARTESIAN_POINT('Ctrl Pts',(43.8431931514392,38.6617505539259,49.2801312762912));
#23916=CARTESIAN_POINT('Ctrl Pts',(43.7981055384867,38.6572951262259,49.330962105467));
#23917=CARTESIAN_POINT('Ctrl Pts',(43.7503914763641,38.6528396985259,49.3793378736793));
#23918=CARTESIAN_POINT('Ctrl Pts',(43.7003601690913,38.6483842708259,49.4249933289461));
#23919=CARTESIAN_POINT('Ctrl Pts',(43.6772710993866,38.6463281246579,49.4460629760634));
#23920=CARTESIAN_POINT('Ctrl Pts',(43.6536889636795,38.6442719784899,49.4665538398702));
#23921=CARTESIAN_POINT('Ctrl Pts',(43.6296462866558,38.6422158323219,49.4864429241022));
#23922=CARTESIAN_POINT('Ctrl Pts',(43.5775411306069,38.6377597637719,49.5295464369329));
#23923=CARTESIAN_POINT('Ctrl Pts',(43.5230626028515,38.6333036952218,49.5699931390812));
#23924=CARTESIAN_POINT('Ctrl Pts',(43.4665127553548,38.6288476266718,49.6075114617214));
#23925=CARTESIAN_POINT('Ctrl Pts',(43.4100486217883,38.6243983122894,49.6449729169599));
#23926=CARTESIAN_POINT('Ctrl Pts',(43.3515198070534,38.619948997907,49.6795145304511));
#23927=CARTESIAN_POINT('Ctrl Pts',(43.2912613242142,38.6154996835246,49.7109049678051));
#23928=CARTESIAN_POINT('Ctrl Pts',(43.2310741215748,38.6110556322688,49.7422582731812));
#23929=CARTESIAN_POINT('Ctrl Pts',(43.1691617498466,38.6066115810129,49.7704675779291));
#23930=CARTESIAN_POINT('Ctrl Pts',(43.1058865124272,38.602167529757,49.7953458687599));
#23931=CARTESIAN_POINT('Ctrl Pts',(43.0426511370463,38.5977262781578,49.8202084868027));
#23932=CARTESIAN_POINT('Ctrl Pts',(42.9780550574625,38.5932850265586,49.8417440730858));
#23933=CARTESIAN_POINT('Ctrl Pts',(42.9124819446754,38.5888437749594,49.859813112461));
#23934=CARTESIAN_POINT('Ctrl Pts',(42.846927475386,38.5844037860799,49.8778770145157));
#23935=CARTESIAN_POINT('Ctrl Pts',(42.7803970000913,38.5799637972005,49.8924761950324));
#23936=CARTESIAN_POINT('Ctrl Pts',(42.7132890286575,38.575523808321,49.9035210903541));
#23937=CARTESIAN_POINT('Ctrl Pts',(42.646176941115,38.5710835471121,49.9145666631213));
#23938=CARTESIAN_POINT('Ctrl Pts',(42.5784877747189,38.5666432859032,49.9220574402996));
#23939=CARTESIAN_POINT('Ctrl Pts',(42.5106280739844,38.5622030246943,49.9259553437571));
#23940=CARTESIAN_POINT('Ctrl Pts',(42.4426955759387,38.5577580001417,49.9298574287375));
#23941=CARTESIAN_POINT('Ctrl Pts',(42.3745926723404,38.553312975589,49.930158919949));
#23942=CARTESIAN_POINT('Ctrl Pts',(42.3067278065509,38.5488679510364,49.9268738554532));
#23943=CARTESIAN_POINT('Ctrl Pts',(42.2388218919885,38.5444202378643,49.9235868039519));
#23944=CARTESIAN_POINT('Ctrl Pts',(42.1711547930101,38.5399725246922,49.9167089295442));
#23945=CARTESIAN_POINT('Ctrl Pts',(42.1041288801391,38.5355248115201,49.9063060712625));
#23946=CARTESIAN_POINT('Ctrl Pts',(42.0369867112835,38.5310693838201,49.8958851692947));
#23947=CARTESIAN_POINT('Ctrl Pts',(41.9704884309552,38.52661395612,49.8819271827729));
#23948=CARTESIAN_POINT('Ctrl Pts',(41.9050244002588,38.52215852842,49.8645486618914));
#23949=CARTESIAN_POINT('Ctrl Pts',(41.8748132454782,38.520102382252,49.8565286060129));
#23950=CARTESIAN_POINT('Ctrl Pts',(41.8448221191952,38.518046236084,49.8477807509429));
#23951=CARTESIAN_POINT('Ctrl Pts',(41.8150879574917,38.515990089916,49.8383200100714));
#23952=CARTESIAN_POINT('Ctrl Pts',(41.8080935585759,38.5155064204361,49.8360945497959));
#23953=CARTESIAN_POINT('Ctrl Pts',(41.8011103478743,38.5150227509561,49.8338286893421));
#23954=CARTESIAN_POINT('Ctrl Pts',(41.7941388317924,38.5145390814761,49.8315225365138));
#23955=CARTESIAN_POINT('Ctrl Pts',(41.794388702738,39.3084106968696,49.8307330830672));
#23956=CARTESIAN_POINT('Ctrl Pts',(41.6242464827134,39.2967219793634,49.7762498623184));
#23957=CARTESIAN_POINT('Ctrl Pts',(40.8927293640396,39.243991282706,49.4267783126541));
#23958=CARTESIAN_POINT('Ctrl Pts',(40.4690312818219,39.1912605860486,48.6236303199305));
#23959=CARTESIAN_POINT('Ctrl Pts',(40.4677075517586,39.1502186068972,47.9997128640878));
#23960=CARTESIAN_POINT('Ctrl Pts',(41.7941386883808,39.4806729614233,49.8315224890738));
#23961=CARTESIAN_POINT('Ctrl Pts',(41.7572007799993,39.4782721882691,49.8193035565988));
#23962=CARTESIAN_POINT('Ctrl Pts',(41.720626997409,39.4758420980136,49.8059653724231));
#23963=CARTESIAN_POINT('Ctrl Pts',(41.6648128553858,39.4720348275255,49.7836732792336));
#23964=CARTESIAN_POINT('Ctrl Pts',(41.6452889524772,39.4706839644207,49.775500403506));
#23965=CARTESIAN_POINT('Ctrl Pts',(41.6159277838943,39.4686214767054,49.7626377800555));
#23966=CARTESIAN_POINT('Ctrl Pts',(41.6059888700241,39.4679178616983,49.7581830112859));
#23967=CARTESIAN_POINT('Ctrl Pts',(41.5880356441581,39.466636703225,49.7499528324736));
#23968=CARTESIAN_POINT('Ctrl Pts',(41.5800085491572,39.4660601549749,49.7462059005683));
#23969=CARTESIAN_POINT('Ctrl Pts',(41.5627688755735,39.4648137120119,49.7380135876415));
#23970=CARTESIAN_POINT('Ctrl Pts',(41.5535653133043,39.4641431961828,49.7335499706784));
#23971=CARTESIAN_POINT('Ctrl Pts',(41.5286901639997,39.4623168446785,49.7212405049893));
#23972=CARTESIAN_POINT('Ctrl Pts',(41.5130896082403,39.4611561186577,49.7132541051122));
#23973=CARTESIAN_POINT('Ctrl Pts',(41.4306461857406,39.4549382696789,49.6696210011786));
#23974=CARTESIAN_POINT('Ctrl Pts',(41.3658458138884,39.4497507967578,49.6302771643636));
#23975=CARTESIAN_POINT('Ctrl Pts',(41.1963341554496,39.4353488207674,49.5131775915762));
#23976=CARTESIAN_POINT('Ctrl Pts',(41.0969173575093,39.4259401962981,49.4284568581312));
#23977=CARTESIAN_POINT('Ctrl Pts',(40.9762616586075,39.413595948292,49.3024830002245));
#23978=CARTESIAN_POINT('Ctrl Pts',(40.9468170149334,39.4104991199501,49.2695481691971));
#23979=CARTESIAN_POINT('Ctrl Pts',(40.9073374957543,39.4062560106887,49.2222137290788));
#23980=CARTESIAN_POINT('Ctrl Pts',(40.896330196568,39.4050624252255,49.2086459038197));
#23981=CARTESIAN_POINT('Ctrl Pts',(40.8774008566907,39.4029936908133,49.1846542640887));
#23982=CARTESIAN_POINT('Ctrl Pts',(40.8693979126598,39.4021138133726,49.1742960231302));
#23983=CARTESIAN_POINT('Ctrl Pts',(40.857680046825,39.400818581186,49.1588062068697));
#23984=CARTESIAN_POINT('Ctrl Pts',(40.8538841673837,39.4003978982557,49.153736754207));
#23985=CARTESIAN_POINT('Ctrl Pts',(40.8474329986074,39.399681165666,49.1450321069591));
#23986=CARTESIAN_POINT('Ctrl Pts',(40.8447653943652,39.3993842695105,49.141406212859));
#23987=CARTESIAN_POINT('Ctrl Pts',(40.838735123276,39.3987119483314,49.1331492812333));
#23988=CARTESIAN_POINT('Ctrl Pts',(40.8353803549895,39.398337069403,49.1285125951464));
#23989=CARTESIAN_POINT('Ctrl Pts',(40.8262918142114,39.3973189247411,49.1158327243912));
#23990=CARTESIAN_POINT('Ctrl Pts',(40.8205990075511,39.3966783895212,49.1077601897435));
#23991=CARTESIAN_POINT('Ctrl Pts',(40.7921010249354,39.3934556013828,49.0666830753785));
#23992=CARTESIAN_POINT('Ctrl Pts',(40.7702655459503,39.3909325345241,49.0330140525441));
#23993=CARTESIAN_POINT('Ctrl Pts',(40.7373861659563,39.3870033112992,48.9786750416741));
#23994=CARTESIAN_POINT('Ctrl Pts',(40.7256425512353,39.3855705623336,48.9584449915192));
#23995=CARTESIAN_POINT('Ctrl Pts',(40.6632895401385,39.3777703119716,48.8463877054721));
#23996=CARTESIAN_POINT('Ctrl Pts',(40.6198618690059,39.3715981013804,48.7507631724698));
#23997=CARTESIAN_POINT('Ctrl Pts',(40.5525759702005,39.359654748008,48.5634196189072));
#23998=CARTESIAN_POINT('Ctrl Pts',(40.5272734114907,39.353922997071,48.4725560589942));
#23999=CARTESIAN_POINT('Ctrl Pts',(40.5039970048509,39.346464967583,48.3567729292254));
#24000=CARTESIAN_POINT('Ctrl Pts',(40.4997208135259,39.3449422661323,48.3332464754407));
#24001=CARTESIAN_POINT('Ctrl Pts',(40.4940485475633,39.3426712186698,48.2983659743585));
#24002=CARTESIAN_POINT('Ctrl Pts',(40.4923142882815,39.3419335863272,48.2870686498577));
#24003=CARTESIAN_POINT('Ctrl Pts',(40.4894072254195,39.3406153820887,48.2669403625762));
#24004=CARTESIAN_POINT('Ctrl Pts',(40.488194998409,39.3400360767431,48.2581153596175));
#24005=CARTESIAN_POINT('Ctrl Pts',(40.4857672255838,39.3388101134469,48.2394849921932));
#24006=CARTESIAN_POINT('Ctrl Pts',(40.4845658063796,39.338163026284,48.2296780787845));
#24007=CARTESIAN_POINT('Ctrl Pts',(40.4815718759133,39.3364361325577,48.2035797335713));
#24008=CARTESIAN_POINT('Ctrl Pts',(40.4799115898022,39.3353521956303,48.1872742478333));
#24009=CARTESIAN_POINT('Ctrl Pts',(40.4733613752745,39.3304338430108,48.11364743718));
#24010=CARTESIAN_POINT('Ctrl Pts',(40.4708297108102,39.3265266190048,48.056151172904));
#24011=CARTESIAN_POINT('Ctrl Pts',(40.4709432424599,39.315454698046,47.895994494694));
#24012=CARTESIAN_POINT('Ctrl Pts',(40.4792070365146,39.308147369249,47.7935357747464));
#24013=CARTESIAN_POINT('Ctrl Pts',(40.5122448140058,39.2933532485622,47.5891031991035));
#24014=CARTESIAN_POINT('Ctrl Pts',(40.5372622012714,39.2858911459844,47.4874885874659));
#24015=CARTESIAN_POINT('Ctrl Pts',(40.5756031817763,39.277657876097,47.3727924232959));
#24016=CARTESIAN_POINT('Ctrl Pts',(40.5810173459183,39.2765472774639,47.3572595834893));
#24017=CARTESIAN_POINT('Ctrl Pts',(40.5888309240076,39.2750160935208,47.3357329176423));
#24018=CARTESIAN_POINT('Ctrl Pts',(40.5910625614552,39.2745864041359,47.3296795356606));
#24019=CARTESIAN_POINT('Ctrl Pts',(40.5949634532207,39.2738484320678,47.3192596146288));
#24020=CARTESIAN_POINT('Ctrl Pts',(40.5966182707184,39.2735393141178,47.3148877849963));
#24021=CARTESIAN_POINT('Ctrl Pts',(40.6001404397498,39.2728896713182,47.3056838215192));
#24022=CARTESIAN_POINT('Ctrl Pts',(40.6020113929379,39.2725493757342,47.3008531182257));
#24023=CARTESIAN_POINT('Ctrl Pts',(40.6066962963271,39.2717088804307,47.2889001287027));
#24024=CARTESIAN_POINT('Ctrl Pts',(40.6095332778297,39.271210044207,47.2817868546033));
#24025=CARTESIAN_POINT('Ctrl Pts',(40.6203511862378,39.2693447142586,47.2551251919791));
#24026=CARTESIAN_POINT('Ctrl Pts',(40.6286108505886,39.2679939012571,47.2356905404024));
#24027=CARTESIAN_POINT('Ctrl Pts',(40.6957596493483,39.2575348292537,47.0846315185017));
#24028=CARTESIAN_POINT('Ctrl Pts',(40.7689270280666,39.2491101547511,46.9598332643251));
#24029=CARTESIAN_POINT('Ctrl Pts',(40.9212756821805,39.2338835330702,46.7562014504121));
#24030=CARTESIAN_POINT('Ctrl Pts',(40.994634592764,39.227201349917,46.6738764092354));
#24031=CARTESIAN_POINT('Ctrl Pts',(41.0869948728352,39.2191273242738,46.5865464982635));
#24032=CARTESIAN_POINT('Ctrl Pts',(41.0995382544105,39.2180376452817,46.5749973740234));
#24033=CARTESIAN_POINT('Ctrl Pts',(41.1204299091927,39.2162327954686,46.5562672888958));
#24034=CARTESIAN_POINT('Ctrl Pts',(41.1286896755948,39.2155217491854,46.5489886943392));
#24035=CARTESIAN_POINT('Ctrl Pts',(41.1437133203832,39.2142326858313,46.5359764513183));
#24036=CARTESIAN_POINT('Ctrl Pts',(41.1504553349946,39.2136557232901,46.5302179419323));
#24037=CARTESIAN_POINT('Ctrl Pts',(41.1649937129591,39.2124146622441,46.5179727110113));
#24038=CARTESIAN_POINT('Ctrl Pts',(41.1728019845625,39.2117499891727,46.5115006084769));
#24039=CARTESIAN_POINT('Ctrl Pts',(41.1942935696943,39.2099253990083,46.4939707634743));
#24040=CARTESIAN_POINT('Ctrl Pts',(41.2080774072111,39.208760490584,46.4830383804725));
#24041=CARTESIAN_POINT('Ctrl Pts',(41.2890526385286,39.2019456662222,46.4205994790996));
#24042=CARTESIAN_POINT('Ctrl Pts',(41.3594176076335,39.1961304518185,46.3733793444299));
#24043=CARTESIAN_POINT('Ctrl Pts',(41.5319026431404,39.1821374384727,46.2734107427961));
#24044=CARTESIAN_POINT('Ctrl Pts',(41.6360890500218,39.1738734558777,46.2248547046026));
#24045=CARTESIAN_POINT('Ctrl Pts',(41.7775097994723,39.1632037352662,46.1737138321046));
#24046=CARTESIAN_POINT('Ctrl Pts',(41.8113895807534,39.1606883272452,46.162514431062));
#24047=CARTESIAN_POINT('Ctrl Pts',(41.8822463478663,39.15553467628,46.1412529397935));
#24048=CARTESIAN_POINT('Ctrl Pts',(41.9192535767295,39.1529020568492,46.131339296387));
#24049=CARTESIAN_POINT('Ctrl Pts',(41.9661011507873,39.14966293581,46.1202736961043));
#24050=CARTESIAN_POINT('Ctrl Pts',(41.9756854348441,39.1490051351641,46.1180870506836));
#24051=CARTESIAN_POINT('Ctrl Pts',(41.9908092716992,39.1479752467331,46.1147579767026));
#24052=CARTESIAN_POINT('Ctrl Pts',(41.9963376890241,39.147600478758,46.1135665187244));
#24053=CARTESIAN_POINT('Ctrl Pts',(42.0067818552093,39.1468957856102,46.1113636577592));
#24054=CARTESIAN_POINT('Ctrl Pts',(42.011696271132,39.1465655909001,46.1103471331056));
#24055=CARTESIAN_POINT('Ctrl Pts',(42.0232183998512,39.1457946110378,46.1080106808329));
#24056=CARTESIAN_POINT('Ctrl Pts',(42.029829128553,39.1453547038684,46.1067061803977));
#24057=CARTESIAN_POINT('Ctrl Pts',(42.0514382506145,39.1439242805252,46.1025595432674));
#24058=CARTESIAN_POINT('Ctrl Pts',(42.0664640089414,39.1429414883017,46.0998607003952));
#24059=CARTESIAN_POINT('Ctrl Pts',(42.149402338378,39.1375739015709,46.0859779573723));
#24060=CARTESIAN_POINT('Ctrl Pts',(42.2178510210939,39.1333537973385,46.0782551227953));
#24061=CARTESIAN_POINT('Ctrl Pts',(42.4066888467311,39.1219332133013,46.067132769227));
#24062=CARTESIAN_POINT('Ctrl Pts',(42.5272025950652,39.1148755555931,46.0713111293193));
#24063=CARTESIAN_POINT('Ctrl Pts',(42.721195806884,39.1030056823874,46.0963084994355));
#24064=CARTESIAN_POINT('Ctrl Pts',(42.7952133723485,39.0983569312193,46.1102877210163));
#24065=CARTESIAN_POINT('Ctrl Pts',(42.8851943505182,39.0924557974302,46.1328001780605));
#24066=CARTESIAN_POINT('Ctrl Pts',(42.9021099918791,39.0913355171407,46.1372777296383));
#24067=CARTESIAN_POINT('Ctrl Pts',(42.9288076673937,39.0895489658275,46.1447346528061));
#24068=CARTESIAN_POINT('Ctrl Pts',(42.938631210012,39.0888876116105,46.1475628295367));
#24069=CARTESIAN_POINT('Ctrl Pts',(42.9569251776393,39.0876483347286,46.1529874428265));
#24070=CARTESIAN_POINT('Ctrl Pts',(42.9654011277285,39.0870710625808,46.1555644223251));
#24071=CARTESIAN_POINT('Ctrl Pts',(42.9842652903852,39.0857792280311,46.1614420234705));
#24072=CARTESIAN_POINT('Ctrl Pts',(42.994643818116,39.0850637001294,46.1647724708143));
#24073=CARTESIAN_POINT('Ctrl Pts',(43.0251290005625,39.082947493201,46.1748408404315));
#24074=CARTESIAN_POINT('Ctrl Pts',(43.0451528755385,39.0815388274328,46.1818223598861));
#24075=CARTESIAN_POINT('Ctrl Pts',(43.0904926017613,39.0783053079238,46.1984737693127));
#24076=CARTESIAN_POINT('Ctrl Pts',(43.1157274847944,39.0764739283183,46.2083496892094));
#24077=CARTESIAN_POINT('Ctrl Pts',(43.200170055643,39.0702366648794,46.2434657756511));
#24078=CARTESIAN_POINT('Ctrl Pts',(43.2583157339956,39.0657562925065,46.2711340994453));
#24079=CARTESIAN_POINT('Ctrl Pts',(43.4186632612192,39.0529023988584,46.3575195785736));
#24080=CARTESIAN_POINT('Ctrl Pts',(43.5170217130359,39.0443979853303,46.4227625782621));
#24081=CARTESIAN_POINT('Ctrl Pts',(43.6166302380897,39.0353902583729,46.5028513719334));
#24082=CARTESIAN_POINT('Ctrl Pts',(43.6243976426928,39.0346851569305,46.5091970054033));
#24083=CARTESIAN_POINT('Ctrl Pts',(43.6680935891876,39.0307047187082,46.5454665780805));
#24084=CARTESIAN_POINT('Ctrl Pts',(43.7029776770778,39.0274731622907,46.5766311789618));
#24085=CARTESIAN_POINT('Ctrl Pts',(43.7441440353361,39.0236265394354,46.6161914774334));
#24086=CARTESIAN_POINT('Ctrl Pts',(43.7515331385909,39.0229347412754,46.6234073217633));
#24087=CARTESIAN_POINT('Ctrl Pts',(43.7629991483236,39.0218596255801,46.6347857987943));
#24088=CARTESIAN_POINT('Ctrl Pts',(43.767115621351,39.0214733103927,46.6389080216273));
#24089=CARTESIAN_POINT('Ctrl Pts',(43.7747211942386,39.0207590478848,46.6465935333712));
#24090=CARTESIAN_POINT('Ctrl Pts',(43.778215138132,39.0204307321622,46.6501516901234));
#24091=CARTESIAN_POINT('Ctrl Pts',(43.7862019958432,39.019679742385,46.658348672111));
#24092=CARTESIAN_POINT('Ctrl Pts',(43.7906854469215,39.0192578009104,46.6629965409169));
#24093=CARTESIAN_POINT('Ctrl Pts',(43.8046333246866,39.0179436475635,46.6776019874962));
#24094=CARTESIAN_POINT('Ctrl Pts',(43.814015029175,39.0170575224528,46.6876384630627));
#24095=CARTESIAN_POINT('Ctrl Pts',(43.8358425391412,39.0149881731168,46.7114952061302));
#24096=CARTESIAN_POINT('Ctrl Pts',(43.8481974861094,39.0138108110424,46.7253971217567));
#24097=CARTESIAN_POINT('Ctrl Pts',(43.8920818162645,39.0095972988479,46.7762382662281));
#24098=CARTESIAN_POINT('Ctrl Pts',(43.9224164973262,39.0066239413646,46.8141882136135));
#24099=CARTESIAN_POINT('Ctrl Pts',(44.0486865858999,38.99377438918,46.9850018057142));
#24100=CARTESIAN_POINT('Ctrl Pts',(44.1288993006195,38.9842572057103,47.1286235283099));
#24101=CARTESIAN_POINT('Ctrl Pts',(44.2055763545409,38.9714957029341,47.3194250648631));
#24102=CARTESIAN_POINT('Ctrl Pts',(44.2198913317623,38.9688682491835,47.3586862269963));
#24103=CARTESIAN_POINT('Ctrl Pts',(44.2374793407569,38.9652644095579,47.4122704776094));
#24104=CARTESIAN_POINT('Ctrl Pts',(44.24188076888,38.9643251348417,47.4262129896059));
#24105=CARTESIAN_POINT('Ctrl Pts',(44.2488787914039,38.9627672067203,47.449291412655));
#24106=CARTESIAN_POINT('Ctrl Pts',(44.2515672060382,38.962151578104,47.4583990310013));
#24107=CARTESIAN_POINT('Ctrl Pts',(44.2566839328357,38.9609454518536,47.4762165666444));
#24108=CARTESIAN_POINT('Ctrl Pts',(44.2591184700721,38.9603551754785,47.4849244511377));
#24109=CARTESIAN_POINT('Ctrl Pts',(44.2647290631648,38.9589549320483,47.5055506025358));
#24110=CARTESIAN_POINT('Ctrl Pts',(44.2678521781921,38.9581432701149,47.517482731882));
#24111=CARTESIAN_POINT('Ctrl Pts',(44.2779331130477,38.9554109810469,47.5575630072758));
#24112=CARTESIAN_POINT('Ctrl Pts',(44.2843704287005,38.9534737696925,47.5858367456617));
#24113=CARTESIAN_POINT('Ctrl Pts',(44.309146871886,38.9451098020085,47.7072388296506));
#24114=CARTESIAN_POINT('Ctrl Pts',(44.3212345010496,38.9384922981646,47.8014947948279));
#24115=CARTESIAN_POINT('Ctrl Pts',(44.3321439783103,38.9241022856435,48.0040437749043));
#24116=CARTESIAN_POINT('Ctrl Pts',(44.3288913655582,38.9163190100983,48.1121376370611));
#24117=CARTESIAN_POINT('Ctrl Pts',(44.3108184602381,38.9051505583447,48.2700231215503));
#24118=CARTESIAN_POINT('Ctrl Pts',(44.3030181609168,38.9016194268671,48.3204099815791));
#24119=CARTESIAN_POINT('Ctrl Pts',(44.2912006234036,38.8974710449596,48.3808077071793));
#24120=CARTESIAN_POINT('Ctrl Pts',(44.2890854288227,38.8967626597076,48.3911656463099));
#24121=CARTESIAN_POINT('Ctrl Pts',(44.2856612322629,38.895667405426,48.4072577252834));
#24122=CARTESIAN_POINT('Ctrl Pts',(44.2844110135683,38.8952773609034,48.4130039611114));
#24123=CARTESIAN_POINT('Ctrl Pts',(44.2820533998654,38.8945597493575,48.423606378354));
#24124=CARTESIAN_POINT('Ctrl Pts',(44.2809534768241,38.8942317828576,48.428463980641));
#24125=CARTESIAN_POINT('Ctrl Pts',(44.2784013938672,38.8934860894097,48.4395355267987));
#24126=CARTESIAN_POINT('Ctrl Pts',(44.2769372068717,38.8930690552023,48.4457465649162));
#24127=CARTESIAN_POINT('Ctrl Pts',(44.2723175624508,38.8917855812395,48.4649165388688));
#24128=CARTESIAN_POINT('Ctrl Pts',(44.2690584350834,38.8909248294404,48.477850429498));
#24129=CARTESIAN_POINT('Ctrl Pts',(44.261112014321,38.8889243433001,48.5080600359224));
#24130=CARTESIAN_POINT('Ctrl Pts',(44.256317841084,38.8877899530337,48.5253066269653));
#24131=CARTESIAN_POINT('Ctrl Pts',(44.2384012239809,38.8837875737641,48.5864489084932));
#24132=CARTESIAN_POINT('Ctrl Pts',(44.2239553937596,38.8809758064384,48.6299433905435));
#24133=CARTESIAN_POINT('Ctrl Pts',(44.1601953046972,38.8698940029453,48.801260277132));
#24134=CARTESIAN_POINT('Ctrl Pts',(44.0988807443618,38.8618992627093,48.9241815550249));
#24135=CARTESIAN_POINT('Ctrl Pts',(43.9886465595339,38.8494320888307,49.0964995169153));
#24136=CARTESIAN_POINT('Ctrl Pts',(43.9492686837471,38.8452421134808,49.1514660817397));
#24137=CARTESIAN_POINT('Ctrl Pts',(43.8963544494236,38.8398456097511,49.2176870545653));
#24138=CARTESIAN_POINT('Ctrl Pts',(43.8854384194936,38.8387437517679,49.2309797204837));
#24139=CARTESIAN_POINT('Ctrl Pts',(43.8678606077272,38.8369862460035,49.2518102621233));
#24140=CARTESIAN_POINT('Ctrl Pts',(43.8613149330871,38.8363353481609,49.2594452572637));
#24141=CARTESIAN_POINT('Ctrl Pts',(43.8494628323335,38.8351629311323,49.2730529761167));
#24142=CARTESIAN_POINT('Ctrl Pts',(43.8441783986887,38.8346423350809,49.2790446168286));
#24143=CARTESIAN_POINT('Ctrl Pts',(43.8317206122763,38.8334199275515,49.2929939774011));
#24144=CARTESIAN_POINT('Ctrl Pts',(43.824517941207,38.8327168884227,49.3009250418483));
#24145=CARTESIAN_POINT('Ctrl Pts',(43.8034818287595,38.8306739669742,49.3237043244996));
#24146=CARTESIAN_POINT('Ctrl Pts',(43.7894800324291,38.8293269126964,49.3383943993127));
#24147=CARTESIAN_POINT('Ctrl Pts',(43.6823586979531,38.8191119260573,49.4472885374793));
#24148=CARTESIAN_POINT('Ctrl Pts',(43.5800071337812,38.809820019025,49.5318807818622));
#24149=CARTESIAN_POINT('Ctrl Pts',(43.3644824381448,38.7913458446355,49.6755120273465));
#24150=CARTESIAN_POINT('Ctrl Pts',(43.2524819043023,38.7822289632951,49.7351791451136));
#24151=CARTESIAN_POINT('Ctrl Pts',(43.1210208775772,38.7725601031495,49.7893894383931));
#24152=CARTESIAN_POINT('Ctrl Pts',(43.1065342315239,38.7715082902099,49.7951587912484));
#24153=CARTESIAN_POINT('Ctrl Pts',(43.0860916350656,38.7700447144953,49.8030143094472));
#24154=CARTESIAN_POINT('Ctrl Pts',(43.0801934360561,38.7696248332792,49.8052476905077));
#24155=CARTESIAN_POINT('Ctrl Pts',(43.0695068487902,38.7688685392684,49.8092344062377));
#24156=CARTESIAN_POINT('Ctrl Pts',(43.0647222675997,38.7685315432248,49.8109977543844));
#24157=CARTESIAN_POINT('Ctrl Pts',(43.0549157284213,38.7678442026703,49.8145678350829));
#24158=CARTESIAN_POINT('Ctrl Pts',(43.0498931782063,38.7674939668654,49.8163727310496));
#24159=CARTESIAN_POINT('Ctrl Pts',(43.036957588152,38.7665963845983,49.8209607209855));
#24160=CARTESIAN_POINT('Ctrl Pts',(43.0290336689952,38.7660508238317,49.8237131260307));
#24161=CARTESIAN_POINT('Ctrl Pts',(42.9955560913265,38.7637628443871,49.8350975402084));
#24162=CARTESIAN_POINT('Ctrl Pts',(42.9698394374398,38.762046738982,49.843245299016));
#24163=CARTESIAN_POINT('Ctrl Pts',(42.8990915829143,38.7574166132156,49.8640378480051));
#24164=CARTESIAN_POINT('Ctrl Pts',(42.8537564966018,38.7545488542413,49.8755892804064));
#24165=CARTESIAN_POINT('Ctrl Pts',(42.6689347399941,38.7430938071423,49.9155871716998));
#24166=CARTESIAN_POINT('Ctrl Pts',(42.5269234233933,38.7347952420668,49.9302052107738));
#24167=CARTESIAN_POINT('Ctrl Pts',(42.3229421139634,38.7223179472847,49.9285760942051));
#24168=CARTESIAN_POINT('Ctrl Pts',(42.2613555020867,38.7184835111987,49.9251286201491));
#24169=CARTESIAN_POINT('Ctrl Pts',(42.1833784088071,38.7134892501052,49.9170024507489));
#24170=CARTESIAN_POINT('Ctrl Pts',(42.1667367471954,38.7124153726899,49.9150487033754));
#24171=CARTESIAN_POINT('Ctrl Pts',(42.1402468676717,38.7106922619895,49.9115883632989));
#24172=CARTESIAN_POINT('Ctrl Pts',(42.1303809732373,38.7100474597499,49.9102218024807));
#24173=CARTESIAN_POINT('Ctrl Pts',(42.1126079135513,38.7088801838101,49.9076195610772));
#24174=CARTESIAN_POINT('Ctrl Pts',(42.1046969653766,38.7083585807557,49.9064109514066));
#24175=CARTESIAN_POINT('Ctrl Pts',(42.0860784172047,38.7071260625944,49.9034477996196));
#24176=CARTESIAN_POINT('Ctrl Pts',(42.0753777381585,38.7064138534964,49.901652088303));
#24177=CARTESIAN_POINT('Ctrl Pts',(42.0440507928679,38.7043172451695,49.8961229104975));
#24178=CARTESIAN_POINT('Ctrl Pts',(42.0234701061044,38.7029250812669,49.8921435224594));
#24179=CARTESIAN_POINT('Ctrl Pts',(41.932298749733,38.696689819279,49.8729687183958));
#24180=CARTESIAN_POINT('Ctrl Pts',(41.8625838747428,38.6917365813973,49.8541639349618));
#24181=CARTESIAN_POINT('Ctrl Pts',(41.7941383335288,38.6866921868075,49.8315223716899));
#24182=CARTESIAN_POINT('Origin',(42.4,48.4493818343519,48.));
#24183=CARTESIAN_POINT('',(41.7941388718785,37.7199737694749,49.8315225497742));
#24184=CARTESIAN_POINT('',(41.7941388317907,37.8901046061668,49.8315225365133));
#24185=CARTESIAN_POINT('',(41.7941388317924,48.4493818343519,49.8315225365138));
#24186=CARTESIAN_POINT('',(40.4708708049845,38.3564681656839,48.001762339035));
#24187=CARTESIAN_POINT('Ctrl Pts',(41.7941388718785,37.7199737694749,49.8315225497742));
#24188=CARTESIAN_POINT('Ctrl Pts',(41.8877523316507,37.7269321000002,49.8624895484344));
#24189=CARTESIAN_POINT('Ctrl Pts',(41.9836178395209,37.7340242380728,49.8862387901888));
#24190=CARTESIAN_POINT('Ctrl Pts',(42.1540699352791,37.746299514361,49.9148281177976));
#24191=CARTESIAN_POINT('Ctrl Pts',(42.2279046256527,37.7515068157566,49.9228712970221));
#24192=CARTESIAN_POINT('Ctrl Pts',(42.3124126332644,37.7572194796111,49.9271686893187));
#24193=CARTESIAN_POINT('Ctrl Pts',(42.3228029724612,37.7579175714046,49.9276128590917));
#24194=CARTESIAN_POINT('Ctrl Pts',(42.339595075755,37.7590383149552,49.9281946973126));
#24195=CARTESIAN_POINT('Ctrl Pts',(42.3459946577612,37.7594636880468,49.9283845497075));
#24196=CARTESIAN_POINT('Ctrl Pts',(42.3573771748442,37.7602170194124,49.928665519751));
#24197=CARTESIAN_POINT('Ctrl Pts',(42.3623596385389,37.7605456589677,49.9287691923685));
#24198=CARTESIAN_POINT('Ctrl Pts',(42.3732100202436,37.7612588948147,49.9289528998913));
#24199=CARTESIAN_POINT('Ctrl Pts',(42.3790779275809,37.7616430737147,49.929025469547));
#24200=CARTESIAN_POINT('Ctrl Pts',(42.3957552273418,37.7627308111796,49.9291556136361));
#24201=CARTESIAN_POINT('Ctrl Pts',(42.4065651051185,37.7634309115056,49.9291491161159));
#24202=CARTESIAN_POINT('Ctrl Pts',(42.480999192376,37.7682210699932,49.9284787002925));
#24203=CARTESIAN_POINT('Ctrl Pts',(42.5445638419713,37.7721584675607,49.9247581881385));
#24204=CARTESIAN_POINT('Ctrl Pts',(42.7360603000483,37.7838638319947,49.904006532693));
#24205=CARTESIAN_POINT('Ctrl Pts',(42.8625708468446,37.7914036571621,49.8772873612571));
#24206=CARTESIAN_POINT('Ctrl Pts',(43.0117068161834,37.8008862719049,49.8297856211282));
#24207=CARTESIAN_POINT('Ctrl Pts',(43.0377590121689,37.8025646746312,49.8208690260277));
#24208=CARTESIAN_POINT('Ctrl Pts',(43.1146177880199,37.807596104434,49.7927115990767));
#24209=CARTESIAN_POINT('Ctrl Pts',(43.1648086639362,37.8109878777721,49.7718804527781));
#24210=CARTESIAN_POINT('Ctrl Pts',(43.2286321984564,37.8154766773523,49.7421739071562));
#24211=CARTESIAN_POINT('Ctrl Pts',(43.243127981925,37.8165082251169,49.7352050091779));
#24212=CARTESIAN_POINT('Ctrl Pts',(43.266326865696,37.818179427095,49.7236927392929));
#24213=CARTESIAN_POINT('Ctrl Pts',(43.2750855789402,37.8188151159209,49.7192626679247));
#24214=CARTESIAN_POINT('Ctrl Pts',(43.2917446232535,37.820033445157,49.7106764064012));
#24215=CARTESIAN_POINT('Ctrl Pts',(43.2996506794741,37.820615663391,49.7065318312051));
#24216=CARTESIAN_POINT('Ctrl Pts',(43.3177309421539,37.8219565460912,49.6968930937317));
#24217=CARTESIAN_POINT('Ctrl Pts',(43.3278850035971,37.8227165084903,49.6913620735717));
#24218=CARTESIAN_POINT('Ctrl Pts',(43.3594923298819,37.8251041828696,49.6737749567397));
#24219=CARTESIAN_POINT('Ctrl Pts',(43.380764302695,37.8267432748955,49.6613998386583));
#24220=CARTESIAN_POINT('Ctrl Pts',(43.4871957334718,37.8351124619477,49.5967262655778));
#24221=CARTESIAN_POINT('Ctrl Pts',(43.5684239762704,37.8420659007577,49.5382812788406));
#24222=CARTESIAN_POINT('Ctrl Pts',(43.6652471040792,37.8510528295861,49.4565068112768));
#24223=CARTESIAN_POINT('Ctrl Pts',(43.685379886816,37.8529629506852,49.438770595866));
#24224=CARTESIAN_POINT('Ctrl Pts',(43.7973844590631,37.8638137483778,49.3358710652742));
#24225=CARTESIAN_POINT('Ctrl Pts',(43.8811659973364,37.8728313751821,49.2423313698739));
#24226=CARTESIAN_POINT('Ctrl Pts',(43.9645473189848,37.8824151078907,49.128706812523));
#24227=CARTESIAN_POINT('Ctrl Pts',(43.9736509592223,37.8834706873842,49.1159794258304));
#24228=CARTESIAN_POINT('Ctrl Pts',(43.9862115013965,37.8849386802412,49.0979597157393));
#24229=CARTESIAN_POINT('Ctrl Pts',(43.9897985049483,37.8853592729924,49.092759434178));
#24230=CARTESIAN_POINT('Ctrl Pts',(43.9962366873083,37.8861165328041,49.0833268362994));
#24231=CARTESIAN_POINT('Ctrl Pts',(43.9990967362183,37.8864537870104,49.079100656333));
#24232=CARTESIAN_POINT('Ctrl Pts',(44.004912696669,37.8871412792135,49.070432743143));
#24233=CARTESIAN_POINT('Ctrl Pts',(44.0078670040356,37.8874914109149,49.0659900189884));
#24234=CARTESIAN_POINT('Ctrl Pts',(44.0154117599794,37.8883880923588,49.0545413956931));
#24235=CARTESIAN_POINT('Ctrl Pts',(44.0199751409865,37.8889328642698,49.0475176649484));
#24236=CARTESIAN_POINT('Ctrl Pts',(44.0389729966439,37.8912120978329,49.0178560234238));
#24237=CARTESIAN_POINT('Ctrl Pts',(44.052980603543,37.8929205001628,48.9949465648968));
#24238=CARTESIAN_POINT('Ctrl Pts',(44.0899013469995,37.8975233984548,48.9316292528973));
#24239=CARTESIAN_POINT('Ctrl Pts',(44.11184159907,37.900372300004,48.8906730922922));
#24240=CARTESIAN_POINT('Ctrl Pts',(44.1940642782995,37.9116931909724,48.7229000486566));
#24241=CARTESIAN_POINT('Ctrl Pts',(44.2418999831702,37.9198815061603,48.590472046673));
#24242=CARTESIAN_POINT('Ctrl Pts',(44.2899369788385,37.9323497506817,48.3920973784401));
#24243=CARTESIAN_POINT('Ctrl Pts',(44.3018539193616,37.9363080522644,48.3294731137162));
#24244=CARTESIAN_POINT('Ctrl Pts',(44.3129896610024,37.9414441089459,48.2495998958885));
#24245=CARTESIAN_POINT('Ctrl Pts',(44.3151077191802,37.9425296492652,48.2327916355552));
#24246=CARTESIAN_POINT('Ctrl Pts',(44.3181238003864,37.9442672168932,48.2060186620459));
#24247=CARTESIAN_POINT('Ctrl Pts',(44.3191661784829,37.9449146822668,48.1960708438832));
#24248=CARTESIAN_POINT('Ctrl Pts',(44.3209028636329,37.9460843610345,48.1781536751628));
#24249=CARTESIAN_POINT('Ctrl Pts',(44.3216250556844,37.9466056818446,48.1701872075138));
#24250=CARTESIAN_POINT('Ctrl Pts',(44.3232055213664,37.9478343292878,48.15145838507));
#24251=CARTESIAN_POINT('Ctrl Pts',(44.3240230262112,37.9485429229655,48.1406929506482));
#24252=CARTESIAN_POINT('Ctrl Pts',(44.3261433628525,37.9506176764822,48.1092807426832));
#24253=CARTESIAN_POINT('Ctrl Pts',(44.3272044579299,37.9519913545403,48.0886197235859));
#24254=CARTESIAN_POINT('Ctrl Pts',(44.3288578067952,37.9551319912494,48.0417070029651));
#24255=CARTESIAN_POINT('Ctrl Pts',(44.3292467477289,37.9569049520084,48.015452700315));
#24256=CARTESIAN_POINT('Ctrl Pts',(44.328756371073,37.9628721387924,47.9278640447596));
#24257=CARTESIAN_POINT('Ctrl Pts',(44.3254879901965,37.9671339013594,47.8665852240479));
#24258=CARTESIAN_POINT('Ctrl Pts',(44.3105578752507,37.977568794074,47.719202543636));
#24259=CARTESIAN_POINT('Ctrl Pts',(44.2959890040791,37.9837918243251,47.6335261818599));
#24260=CARTESIAN_POINT('Ctrl Pts',(44.2545927368263,37.996421702991,47.4613113027187));
#24261=CARTESIAN_POINT('Ctrl Pts',(44.2273403937788,38.0028100714955,47.3750754619958));
#24262=CARTESIAN_POINT('Ctrl Pts',(44.1902624491323,38.0096237644902,47.2812411071322));
#24263=CARTESIAN_POINT('Ctrl Pts',(44.1863026300751,38.0103325340234,47.2714556232835));
#24264=CARTESIAN_POINT('Ctrl Pts',(44.1797946231788,38.0114669908775,47.2557451772789));
#24265=CARTESIAN_POINT('Ctrl Pts',(44.1772967636231,38.0118955047755,47.2497997874969));
#24266=CARTESIAN_POINT('Ctrl Pts',(44.1728142871328,38.0126522403754,47.2392786754813));
#24267=CARTESIAN_POINT('Ctrl Pts',(44.1708416881168,38.0129811678504,47.2346980021741));
#24268=CARTESIAN_POINT('Ctrl Pts',(44.166522637338,38.0136925477032,47.2247746287503));
#24269=CARTESIAN_POINT('Ctrl Pts',(44.16416970015,38.0140746013856,47.2194348997332));
#24270=CARTESIAN_POINT('Ctrl Pts',(44.1574522305179,38.0151502026677,47.2043758899221));
#24271=CARTESIAN_POINT('Ctrl Pts',(44.1530312781341,38.0158404127178,47.1946817911306));
#24272=CARTESIAN_POINT('Ctrl Pts',(44.1233344374674,38.0203654980837,47.1309672089294));
#24273=CARTESIAN_POINT('Ctrl Pts',(44.0956426382716,38.0240664333629,47.0781013312181));
#24274=CARTESIAN_POINT('Ctrl Pts',(44.0210057536534,38.0330790372086,46.9503935876734));
#24275=CARTESIAN_POINT('Ctrl Pts',(43.9712895797699,38.0383040940369,46.8773318789603));
#24276=CARTESIAN_POINT('Ctrl Pts',(43.8415901525552,38.0508420181915,46.7123075731327));
#24277=CARTESIAN_POINT('Ctrl Pts',(43.7575744225633,38.0581829111807,46.6240203666063));
#24278=CARTESIAN_POINT('Ctrl Pts',(43.6529491420653,38.0669897024222,46.5330468034921));
#24279=CARTESIAN_POINT('Ctrl Pts',(43.6399359993038,38.0680793221632,46.5220311501145));
#24280=CARTESIAN_POINT('Ctrl Pts',(43.6182814563195,38.0698842033573,46.5041878183656));
#24281=CARTESIAN_POINT('Ctrl Pts',(43.609724385289,38.0705953417871,46.497258940181));
#24282=CARTESIAN_POINT('Ctrl Pts',(43.5941683541407,38.0718846607242,46.484881800432));
#24283=CARTESIAN_POINT('Ctrl Pts',(43.5871901963442,38.0724617870051,46.4794077962919));
#24284=CARTESIAN_POINT('Ctrl Pts',(43.5721485664578,38.0737033004324,46.4677750683705));
#24285=CARTESIAN_POINT('Ctrl Pts',(43.5640737850582,38.0743682632118,46.4616314748382));
#24286=CARTESIAN_POINT('Ctrl Pts',(43.5418572226091,38.0761939164913,46.4450033604784));
#24287=CARTESIAN_POINT('Ctrl Pts',(43.5276200845685,38.0773596060269,46.4346484818016));
#24288=CARTESIAN_POINT('Ctrl Pts',(43.4439644705572,38.0841864833071,46.3755380417219));
#24289=CARTESIAN_POINT('Ctrl Pts',(43.3715418859448,38.0900136533926,46.3312156399125));
#24290=CARTESIAN_POINT('Ctrl Pts',(43.1940433649751,38.1040847206503,46.2380657598986));
#24291=CARTESIAN_POINT('Ctrl Pts',(43.0870172085324,38.1124176925237,46.1936440701145));
#24292=CARTESIAN_POINT('Ctrl Pts',(42.9424480925474,38.1231621886984,46.1483578843879));
#24293=CARTESIAN_POINT('Ctrl Pts',(42.9079344253046,38.1256891277892,46.1385942649481));
#24294=CARTESIAN_POINT('Ctrl Pts',(42.8371291768762,38.1307725634051,46.1206803062474));
#24295=CARTESIAN_POINT('Ctrl Pts',(42.8008322182366,38.1333257715061,46.1126053948789));
#24296=CARTESIAN_POINT('Ctrl Pts',(42.754760839883,38.1364821090489,46.1037452445277));
#24297=CARTESIAN_POINT('Ctrl Pts',(42.7451857724544,38.1371335256212,46.1019788875023));
#24298=CARTESIAN_POINT('Ctrl Pts',(42.7300477835494,38.1381557639955,46.0993046593495));
#24299=CARTESIAN_POINT('Ctrl Pts',(42.724493711424,38.1385292008528,46.0983485727744));
#24300=CARTESIAN_POINT('Ctrl Pts',(42.7139789917127,38.1392330126092,46.0965859603361));
#24301=CARTESIAN_POINT('Ctrl Pts',(42.7090194236735,38.1395636444851,46.0957744855223));
#24302=CARTESIAN_POINT('Ctrl Pts',(42.6973604419017,38.1403378307104,46.0939136155589));
#24303=CARTESIAN_POINT('Ctrl Pts',(42.6906585945456,38.1407804853452,46.0928801500175));
#24304=CARTESIAN_POINT('Ctrl Pts',(42.6686191159204,38.142228834074,46.0896004058019));
#24305=CARTESIAN_POINT('Ctrl Pts',(42.6532593865179,38.1432265357254,46.0875035793695));
#24306=CARTESIAN_POINT('Ctrl Pts',(42.5673918001028,38.1487474431376,46.0768340706416));
#24307=CARTESIAN_POINT('Ctrl Pts',(42.4964701280656,38.1530954842667,46.0719743407672));
#24308=CARTESIAN_POINT('Ctrl Pts',(42.3243555401359,38.1634752807328,46.0697048672239));
#24309=CARTESIAN_POINT('Ctrl Pts',(42.2233272886737,38.1694308425207,46.0763189574079));
#24310=CARTESIAN_POINT('Ctrl Pts',(42.0336143009998,38.1809812381941,46.103816153472));
#24311=CARTESIAN_POINT('Ctrl Pts',(41.9449849794371,38.1865343154721,46.1231116464965));
#24312=CARTESIAN_POINT('Ctrl Pts',(41.8405433320331,38.1934510545008,46.153683832365));
#24313=CARTESIAN_POINT('Ctrl Pts',(41.8231145709406,38.1946178177491,46.1590550471593));
#24314=CARTESIAN_POINT('Ctrl Pts',(41.7958789029824,38.1964620700816,46.16787330171));
#24315=CARTESIAN_POINT('Ctrl Pts',(41.7860189488402,38.1971340868875,46.1711539703255));
#24316=CARTESIAN_POINT('Ctrl Pts',(41.7678896458641,38.198377981206,46.1773492032833));
#24317=CARTESIAN_POINT('Ctrl Pts',(41.7596126952469,38.1989490842556,46.1802408065321));
#24318=CARTESIAN_POINT('Ctrl Pts',(41.7413123925342,38.2002190427889,46.1867744427497));
#24319=CARTESIAN_POINT('Ctrl Pts',(41.7312990100742,38.2009187799918,46.1904433515382));
#24320=CARTESIAN_POINT('Ctrl Pts',(41.703037334668,38.2029077637198,46.2010650557742));
#24321=CARTESIAN_POINT('Ctrl Pts',(41.6848639053973,38.2042034705136,46.2082120078709));
#24322=CARTESIAN_POINT('Ctrl Pts',(41.6439215836784,38.2071615655797,46.225035233195));
#24323=CARTESIAN_POINT('Ctrl Pts',(41.6212244090851,38.2088292727656,46.2348759310476));
#24324=CARTESIAN_POINT('Ctrl Pts',(41.5477058314402,38.2143239514411,46.2684450117237));
#24325=CARTESIAN_POINT('Ctrl Pts',(41.4977325345518,38.2182071570383,46.2939517951274));
#24326=CARTESIAN_POINT('Ctrl Pts',(41.3308746376221,38.2316680505038,46.3885006426163));
#24327=CARTESIAN_POINT('Ctrl Pts',(41.2202028421741,38.241495192672,46.4676702495838));
#24328=CARTESIAN_POINT('Ctrl Pts',(41.0802584481814,38.2546550837173,46.5919954585786));
#24329=CARTESIAN_POINT('Ctrl Pts',(41.0431402466294,38.2582244728711,46.6277291840621));
#24330=CARTESIAN_POINT('Ctrl Pts',(41.0001563111384,38.2624112774179,46.6725616392385));
#24331=CARTESIAN_POINT('Ctrl Pts',(40.9928821435564,38.2631217430239,46.6802749129147));
#24332=CARTESIAN_POINT('Ctrl Pts',(40.9816671563294,38.2642195890141,46.6923650451294));
#24333=CARTESIAN_POINT('Ctrl Pts',(40.9776822986068,38.2646101670077,46.6967004990273));
#24334=CARTESIAN_POINT('Ctrl Pts',(40.9703630478456,38.2653283746357,46.7047372630213));
#24335=CARTESIAN_POINT('Ctrl Pts',(40.9670231437181,38.2656564074203,46.7084332370719));
#24336=CARTESIAN_POINT('Ctrl Pts',(40.9594416016885,38.2664017731188,46.7168886646609));
#24337=CARTESIAN_POINT('Ctrl Pts',(40.9552092121771,38.2668184170653,46.7216562355496));
#24338=CARTESIAN_POINT('Ctrl Pts',(40.9426280734039,38.2680588762959,46.7359705456478));
#24339=CARTESIAN_POINT('Ctrl Pts',(40.9343495551088,38.2688777066575,46.7455789431137));
#24340=CARTESIAN_POINT('Ctrl Pts',(40.8593661970961,38.2763259522985,46.8343635689892));
#24341=CARTESIAN_POINT('Ctrl Pts',(40.7990318110347,38.2825566281651,46.9187194066031));
#24342=CARTESIAN_POINT('Ctrl Pts',(40.7056194365599,38.2934067504237,47.0744175103242));
#24343=CARTESIAN_POINT('Ctrl Pts',(40.6695797137903,38.2980338761474,47.1436859391152));
#24344=CARTESIAN_POINT('Ctrl Pts',(40.6030423303135,38.3079070958165,47.2930383394611));
#24345=CARTESIAN_POINT('Ctrl Pts',(40.5734847052241,38.3131603611238,47.3733495127022));
#24346=CARTESIAN_POINT('Ctrl Pts',(40.5442665095039,38.3197399817398,47.4726289650197));
#24347=CARTESIAN_POINT('Ctrl Pts',(40.5394235313273,38.320892600617,47.4899782698166));
#24348=CARTESIAN_POINT('Ctrl Pts',(40.5321837910426,38.3227193378752,47.5173903257529));
#24349=CARTESIAN_POINT('Ctrl Pts',(40.5296237308704,38.3233881560484,47.5274091694835));
#24350=CARTESIAN_POINT('Ctrl Pts',(40.5250416628631,38.3246290190652,47.5459617882296));
#24351=CARTESIAN_POINT('Ctrl Pts',(40.5229970510513,38.3252003159665,47.5544897429874));
#24352=CARTESIAN_POINT('Ctrl Pts',(40.5185819939146,38.326474316769,47.57347472695));
#24353=CARTESIAN_POINT('Ctrl Pts',(40.5162404560886,38.3271779315351,47.5839381115833));
#24354=CARTESIAN_POINT('Ctrl Pts',(40.5115883779812,38.3286358591826,47.6055710555313));
#24355=CARTESIAN_POINT('Ctrl Pts',(40.5092894344784,38.3293905140956,47.6167426526673));
#24356=CARTESIAN_POINT('Ctrl Pts',(40.5035983753021,38.3313511438125,47.6456962735304));
#24357=CARTESIAN_POINT('Ctrl Pts',(40.5003573131292,38.332561836806,47.663506497741));
#24358=CARTESIAN_POINT('Ctrl Pts',(40.4796312963282,38.3410083164143,47.7872633835643));
#24359=CARTESIAN_POINT('Ctrl Pts',(40.4707714790782,38.3485105546629,47.8944436334601));
#24360=CARTESIAN_POINT('Ctrl Pts',(40.4708708262362,38.3561431341929,48.0017854504995));
#24361=CARTESIAN_POINT('Ctrl Pts',(41.7941388317924,38.5145390814761,49.8315225365138));
#24362=CARTESIAN_POINT('Ctrl Pts',(41.7299216957678,38.5100838283546,49.8102797353606));
#24363=CARTESIAN_POINT('Ctrl Pts',(41.6666977242728,38.5056285752331,49.7856139649871));
#24364=CARTESIAN_POINT('Ctrl Pts',(41.604857307503,38.5011733221117,49.7576378055414));
#24365=CARTESIAN_POINT('Ctrl Pts',(41.5404242173827,38.4965312815033,49.728488739333));
#24366=CARTESIAN_POINT('Ctrl Pts',(41.4774937984495,38.4918892408949,49.695745643155));
#24367=CARTESIAN_POINT('Ctrl Pts',(41.4164901120889,38.4872472002865,49.6595935819595));
#24368=CARTESIAN_POINT('Ctrl Pts',(41.3580952101157,38.4828036736333,49.6249875409874));
#24369=CARTESIAN_POINT('Ctrl Pts',(41.3014660882663,38.4783601469802,49.58725843197));
#24370=CARTESIAN_POINT('Ctrl Pts',(41.2469521014508,38.473916620327,49.5466166624446));
#24371=CARTESIAN_POINT('Ctrl Pts',(41.1924695936992,38.4694756595853,49.5059983614809));
#24372=CARTESIAN_POINT('Ctrl Pts',(41.1401001932213,38.4650346988435,49.4624710309536));
#24373=CARTESIAN_POINT('Ctrl Pts',(41.0901639809884,38.4605937381018,49.4162881628397));
#24374=CARTESIAN_POINT('Ctrl Pts',(41.040239343403,38.4561538067243,49.3701159993908));
#24375=CARTESIAN_POINT('Ctrl Pts',(40.9927471365817,38.4517138753469,49.3212898556712));
#24376=CARTESIAN_POINT('Ctrl Pts',(40.9479726604171,38.4472739439695,49.2701020281866));
#24377=CARTESIAN_POINT('Ctrl Pts',(40.9031930861608,38.4428335070545,49.2189083723763));
#24378=CARTESIAN_POINT('Ctrl Pts',(40.861132179701,38.4383930701396,49.1653528725191));
#24379=CARTESIAN_POINT('Ctrl Pts',(40.8220355921919,38.4339526332247,49.1097616341318));
#24380=CARTESIAN_POINT('Ctrl Pts',(40.7828957995435,38.4295072892396,49.0541089625772));
#24381=CARTESIAN_POINT('Ctrl Pts',(40.746727145482,38.4250619452546,48.9964164690217));
#24382=CARTESIAN_POINT('Ctrl Pts',(40.7137318736977,38.4206166012696,48.9370391470568));
#24383=CARTESIAN_POINT('Ctrl Pts',(40.6807150902982,38.4161683590957,48.8776231134209));
#24384=CARTESIAN_POINT('Ctrl Pts',(40.6508760217607,38.4117201169218,48.8165205094757));
#24385=CARTESIAN_POINT('Ctrl Pts',(40.6243696140539,38.4072718747479,48.7541082743247));
#24386=CARTESIAN_POINT('Ctrl Pts',(40.5978184275985,38.4028161179112,48.6915906027141));
#24387=CARTESIAN_POINT('Ctrl Pts',(40.5746113015034,38.3983603610744,48.627759349526));
#24388=CARTESIAN_POINT('Ctrl Pts',(40.5548536832294,38.3939046042376,48.5630076612336));
#24389=CARTESIAN_POINT('Ctrl Pts',(40.5487341383369,38.3925245186618,48.5429520625337));
#24390=CARTESIAN_POINT('Ctrl Pts',(40.5429451459992,38.391144433086,48.522808238269));
#24391=CARTESIAN_POINT('Ctrl Pts',(40.5374888394459,38.3897643475102,48.5025880357822));
#24392=CARTESIAN_POINT('Ctrl Pts',(40.5151350420091,38.3841103115601,48.4197484251217));
#24393=CARTESIAN_POINT('Ctrl Pts',(40.4982971116051,38.3784562756099,48.3353614403265));
#24394=CARTESIAN_POINT('Ctrl Pts',(40.4871470116547,38.3728022396598,48.2500719933908));
#24395=CARTESIAN_POINT('Ctrl Pts',(40.4764097519324,38.3673575483345,48.167940447719));
#24396=CARTESIAN_POINT('Ctrl Pts',(40.4709468203384,38.3619128570092,48.0849718892169));
#24397=CARTESIAN_POINT('Ctrl Pts',(40.4708708049845,38.3564681656839,48.001762339035));
#24398=CARTESIAN_POINT('',(40.470870157182,38.525946964697,47.9992212516664));
#24399=CARTESIAN_POINT('Ctrl Pts',(41.7941383335288,38.6866921868075,49.8315223716899));
#24400=CARTESIAN_POINT('Ctrl Pts',(41.7345131632266,38.6822978481676,49.811798558538));
#24401=CARTESIAN_POINT('Ctrl Pts',(41.6758511936192,38.6778350035951,49.7891631561228));
#24402=CARTESIAN_POINT('Ctrl Pts',(41.5063613798738,38.6646047384149,49.7140482245953));
#24403=CARTESIAN_POINT('Ctrl Pts',(41.3993318161974,38.6557943233053,49.6538499110831));
#24404=CARTESIAN_POINT('Ctrl Pts',(41.2857470068709,38.6463847195162,49.5748754919079));
#24405=CARTESIAN_POINT('Ctrl Pts',(41.2728763285008,38.6453178685796,49.5656898851235));
#24406=CARTESIAN_POINT('Ctrl Pts',(41.2550011804056,38.6438369540284,49.5525979874554));
#24407=CARTESIAN_POINT('Ctrl Pts',(41.2499012506518,38.6434145248567,49.5488239658133));
#24408=CARTESIAN_POINT('Ctrl Pts',(41.2410977614784,38.6426856145579,49.5422417962612));
#24409=CARTESIAN_POINT('Ctrl Pts',(41.2373855982471,38.6423783442543,49.5394453256201));
#24410=CARTESIAN_POINT('Ctrl Pts',(41.2296150603196,38.6417353974066,49.5335474358518));
#24411=CARTESIAN_POINT('Ctrl Pts',(41.2255588228935,38.6413999249021,49.530443258614));
#24412=CARTESIAN_POINT('Ctrl Pts',(41.2157684695609,38.6405904374971,49.5228890047723));
#24413=CARTESIAN_POINT('Ctrl Pts',(41.2100469840157,38.6401175626914,49.5184225572714));
#24414=CARTESIAN_POINT('Ctrl Pts',(41.1975741273322,38.6390867725923,49.5085718886914));
#24415=CARTESIAN_POINT('Ctrl Pts',(41.1908333869482,38.6385297507721,49.5031743847474));
#24416=CARTESIAN_POINT('Ctrl Pts',(41.1717853435303,38.6369551185881,49.4877110247934));
#24417=CARTESIAN_POINT('Ctrl Pts',(41.1595656274798,38.6359442446782,49.4775377960907));
#24418=CARTESIAN_POINT('Ctrl Pts',(41.024671210722,38.6247590070962,49.3623815129185));
#24419=CARTESIAN_POINT('Ctrl Pts',(40.9155015210314,38.6154184177973,49.2425340352882));
#24420=CARTESIAN_POINT('Ctrl Pts',(40.770390204396,38.6002288398038,49.0363976472431));
#24421=CARTESIAN_POINT('Ctrl Pts',(40.7235347387086,38.5946768683313,48.9587540343476));
#24422=CARTESIAN_POINT('Ctrl Pts',(40.6740101399462,38.5877615818485,48.8618781845855));
#24423=CARTESIAN_POINT('Ctrl Pts',(40.6659415151775,38.5865950808534,48.845527135437));
#24424=CARTESIAN_POINT('Ctrl Pts',(40.6536414510752,38.5847512718634,48.8196842680601));
#24425=CARTESIAN_POINT('Ctrl Pts',(40.6492527394026,38.584079433847,48.8102681674697));
#24426=CARTESIAN_POINT('Ctrl Pts',(40.641301886416,38.5828358894247,48.7928431912967));
#24427=CARTESIAN_POINT('Ctrl Pts',(40.6377178461755,38.5822649571779,48.784844562157));
#24428=CARTESIAN_POINT('Ctrl Pts',(40.6298955906118,38.580995403973,48.7670636152126));
#24429=CARTESIAN_POINT('Ctrl Pts',(40.6256837324284,38.5802959020097,48.7572700870777));
#24430=CARTESIAN_POINT('Ctrl Pts',(40.6137894100295,38.57827351474,48.7289690161755));
#24431=CARTESIAN_POINT('Ctrl Pts',(40.6063140495642,38.5769436781771,48.7103764901403));
#24432=CARTESIAN_POINT('Ctrl Pts',(40.5543563741725,38.5672557408761,48.5750969136374));
#24433=CARTESIAN_POINT('Ctrl Pts',(40.5210158307069,38.558523920786,48.4544720155103));
#24434=CARTESIAN_POINT('Ctrl Pts',(40.4804260210494,38.5416985024399,48.2217730010995));
#24435=CARTESIAN_POINT('Ctrl Pts',(40.4708251956828,38.5336760400102,48.11060071288));
#24436=CARTESIAN_POINT('Ctrl Pts',(40.470870157182,38.525946964697,47.9992212516664));
#24437=CARTESIAN_POINT('Ctrl Pts',(40.4708701582568,38.525946780244,47.999218593614));
#24438=CARTESIAN_POINT('Ctrl Pts',(40.4708828771651,38.5237677840215,47.9678182544532));
#24439=CARTESIAN_POINT('Ctrl Pts',(40.4716622495162,38.521614512766,47.9364204037251));
#24440=CARTESIAN_POINT('Ctrl Pts',(40.4735867665144,38.5189788945381,47.8973654208977));
#24441=CARTESIAN_POINT('Ctrl Pts',(40.4740116154422,38.5184622999845,47.8896797830328));
#24442=CARTESIAN_POINT('Ctrl Pts',(40.4748112955889,38.5175889646993,47.876631006523));
#24443=CARTESIAN_POINT('Ctrl Pts',(40.4751625608978,38.5172310083412,47.87126658988));
#24444=CARTESIAN_POINT('Ctrl Pts',(40.4758591479525,38.5165660252818,47.8612696260183));
#24445=CARTESIAN_POINT('Ctrl Pts',(40.4761987858263,38.5162586913329,47.8566367387658));
#24446=CARTESIAN_POINT('Ctrl Pts',(40.4769427946358,38.5156190460474,47.8469670843212));
#24447=CARTESIAN_POINT('Ctrl Pts',(40.4773502233187,38.5152869238488,47.8419306315224));
#24448=CARTESIAN_POINT('Ctrl Pts',(40.4782953772045,38.5145545771141,47.8307917642694));
#24449=CARTESIAN_POINT('Ctrl Pts',(40.4788423962425,38.5141548677088,47.8246901361843));
#24450=CARTESIAN_POINT('Ctrl Pts',(40.4808871023558,38.5127416111478,47.8030427687767));
#24451=CARTESIAN_POINT('Ctrl Pts',(40.4825445378641,38.5117365472453,47.787512228136));
#24452=CARTESIAN_POINT('Ctrl Pts',(40.4890904066313,38.5082033222473,47.7325144643651));
#24453=CARTESIAN_POINT('Ctrl Pts',(40.4950106074898,38.5057236959999,47.6931777964464));
#24454=CARTESIAN_POINT('Ctrl Pts',(40.5228658095184,38.496179636794,47.5403663602293));
#24455=CARTESIAN_POINT('Ctrl Pts',(40.5537622609088,38.4893899605038,47.4287684341477));
#24456=CARTESIAN_POINT('Ctrl Pts',(40.6322377188398,38.4760360474054,47.2202159453531));
#24457=CARTESIAN_POINT('Ctrl Pts',(40.6783120434001,38.4695130050146,47.1231689427268));
#24458=CARTESIAN_POINT('Ctrl Pts',(40.7414842708779,38.461523942277,47.0145006803006));
#24459=CARTESIAN_POINT('Ctrl Pts',(40.750990264355,38.460342831877,46.9986757834234));
#24460=CARTESIAN_POINT('Ctrl Pts',(40.7661666121303,38.4584879831545,46.9742136220707));
#24461=CARTESIAN_POINT('Ctrl Pts',(40.7716818955155,38.457819949258,46.9654810894983));
#24462=CARTESIAN_POINT('Ctrl Pts',(40.7815739647561,38.4566321366866,46.9500937369045));
#24463=CARTESIAN_POINT('Ctrl Pts',(40.7859223751219,38.4561134254891,46.9434208924532));
#24464=CARTESIAN_POINT('Ctrl Pts',(40.7960388770744,38.4549143821289,46.928104833901));
#24465=CARTESIAN_POINT('Ctrl Pts',(40.8018356882228,38.4542329782975,46.9194809782624));
#24466=CARTESIAN_POINT('Ctrl Pts',(40.8180014092799,38.4523478753954,46.8958460912822));
#24467=CARTESIAN_POINT('Ctrl Pts',(40.8285138053603,38.4511387468309,46.8809349901932));
#24468=CARTESIAN_POINT('Ctrl Pts',(40.8926322914025,38.4438597767395,46.792672784679));
#24469=CARTESIAN_POINT('Ctrl Pts',(40.9511462556602,38.4375988435618,46.7230446786938));
#24470=CARTESIAN_POINT('Ctrl Pts',(41.1266021784099,38.4198390688107,46.5419067131972));
#24471=CARTESIAN_POINT('Ctrl Pts',(41.2529561922209,38.4080714894062,46.4405554325174));
#24472=CARTESIAN_POINT('Ctrl Pts',(41.403932690626,38.3959089596003,46.3478369256697));
#24473=CARTESIAN_POINT('Ctrl Pts',(41.4175174961777,38.394830480361,46.3397225910146));
#24474=CARTESIAN_POINT('Ctrl Pts',(41.4386434202174,38.393179452719,46.3274539910938));
#24475=CARTESIAN_POINT('Ctrl Pts',(41.4461147666631,38.3926005254017,46.3231817052689));
#24476=CARTESIAN_POINT('Ctrl Pts',(41.4600581359444,38.3915296629823,46.3153319237529));
#24477=CARTESIAN_POINT('Ctrl Pts',(41.4665225897587,38.391036968115,46.3117413812084));
#24478=CARTESIAN_POINT('Ctrl Pts',(41.4774598976384,38.3902099309013,46.3057485162845));
#24479=CARTESIAN_POINT('Ctrl Pts',(41.4819218320276,38.3898743645437,46.3033265458544));
#24480=CARTESIAN_POINT('Ctrl Pts',(41.4905098397954,38.3892320688824,46.2987087109564));
#24481=CARTESIAN_POINT('Ctrl Pts',(41.4946344018336,38.3889251652736,46.2965101889044));
#24482=CARTESIAN_POINT('Ctrl Pts',(41.5044690072693,38.3881970192153,46.2913138415089));
#24483=CARTESIAN_POINT('Ctrl Pts',(41.5101862179994,38.3877766238892,46.2883295926389));
#24484=CARTESIAN_POINT('Ctrl Pts',(41.5305250086771,38.3862909671198,46.2778426695003));
#24485=CARTESIAN_POINT('Ctrl Pts',(41.5452278595765,38.3852350339145,46.2704979725989));
#24486=CARTESIAN_POINT('Ctrl Pts',(41.6534745254211,38.377578991168,46.2181418615298));
#24487=CARTESIAN_POINT('Ctrl Pts',(41.7504344936811,38.3713554792503,46.1805525576345));
#24488=CARTESIAN_POINT('Ctrl Pts',(41.9523371384044,38.3587799056597,46.1204923208798));
#24489=CARTESIAN_POINT('Ctrl Pts',(42.0570606023698,38.3524465994496,46.0985947214382));
#24490=CARTESIAN_POINT('Ctrl Pts',(42.2181705055776,38.342469653369,46.0786554619686));
#24491=CARTESIAN_POINT('Ctrl Pts',(42.2735502556596,38.3390016023127,46.0742179836061));
#24492=CARTESIAN_POINT('Ctrl Pts',(42.3446459739966,38.3344622059646,46.0716010929313));
#24493=CARTESIAN_POINT('Ctrl Pts',(42.3602573121018,38.3334601480009,46.0712162100114));
#24494=CARTESIAN_POINT('Ctrl Pts',(42.3855819168024,38.3318252874659,46.0708994355424));
#24495=CARTESIAN_POINT('Ctrl Pts',(42.3952932218594,38.3311961397296,46.0708512993016));
#24496=CARTESIAN_POINT('Ctrl Pts',(42.4139572395595,38.3299825356453,46.0708997155454));
#24497=CARTESIAN_POINT('Ctrl Pts',(42.4229097481966,38.3293984404601,46.0709852642114));
#24498=CARTESIAN_POINT('Ctrl Pts',(42.4434331495145,38.3280547528015,46.071324271756));
#24499=CARTESIAN_POINT('Ctrl Pts',(42.4550029126305,38.3272938678415,46.0716195466551));
#24500=CARTESIAN_POINT('Ctrl Pts',(42.4919142552796,38.3248551697899,46.0728940172018));
#24501=CARTESIAN_POINT('Ctrl Pts',(42.5172385930815,38.3231650781469,46.0742687864083));
#24502=CARTESIAN_POINT('Ctrl Pts',(42.6753525891751,38.3125021041073,46.0859825370008));
#24503=CARTESIAN_POINT('Ctrl Pts',(42.8067781968864,38.3031123722117,46.1095499431242));
#24504=CARTESIAN_POINT('Ctrl Pts',(43.0071000741235,38.2882257143609,46.167338233671));
#24505=CARTESIAN_POINT('Ctrl Pts',(43.0782109842461,38.2828293234543,46.1924463375233));
#24506=CARTESIAN_POINT('Ctrl Pts',(43.1794685955045,38.2751110808578,46.2350181493611));
#24507=CARTESIAN_POINT('Ctrl Pts',(43.2109020358738,38.2727106318649,46.2492371957595));
#24508=CARTESIAN_POINT('Ctrl Pts',(43.2615560057805,38.2688530675511,46.2738078965972));
#24509=CARTESIAN_POINT('Ctrl Pts',(43.281011290616,38.2673741215825,46.283655881264));
#24510=CARTESIAN_POINT('Ctrl Pts',(43.3071528421466,38.2653946509521,46.2974500365546));
#24511=CARTESIAN_POINT('Ctrl Pts',(43.3139875466697,38.2648778490537,46.3011093541202));
#24512=CARTESIAN_POINT('Ctrl Pts',(43.3253693624177,38.2640186777861,46.3072917742108));
#24513=CARTESIAN_POINT('Ctrl Pts',(43.3299286046148,38.2636749113159,46.3097922060175));
#24514=CARTESIAN_POINT('Ctrl Pts',(43.3385524028167,38.2630255060592,46.3145672256351));
#24515=CARTESIAN_POINT('Ctrl Pts',(43.3426189114209,38.2627196309846,46.3168381424467));
#24516=CARTESIAN_POINT('Ctrl Pts',(43.3522401940965,38.2619966677628,46.3222568931005));
#24517=CARTESIAN_POINT('Ctrl Pts',(43.3577876869971,38.2615803984777,46.3254176432707));
#24518=CARTESIAN_POINT('Ctrl Pts',(43.3772237379715,38.2601236447576,46.336619745097));
#24519=CARTESIAN_POINT('Ctrl Pts',(43.3910280009102,38.2590920224127,46.34480706613));
#24520=CARTESIAN_POINT('Ctrl Pts',(43.5053947930275,38.2505566087909,46.4145819410158));
#24521=CARTESIAN_POINT('Ctrl Pts',(43.6002319135202,38.2435437827632,46.4851075451388));
#24522=CARTESIAN_POINT('Ctrl Pts',(43.7920307615505,38.2281776174326,46.6571281789475));
#24523=CARTESIAN_POINT('Ctrl Pts',(43.885567937651,38.2198400748564,46.7613976280763));
#24524=CARTESIAN_POINT('Ctrl Pts',(43.979126806952,38.209673417496,46.8916987706547));
#24525=CARTESIAN_POINT('Ctrl Pts',(43.9909555891399,38.2083486029498,46.9087468912238));
#24526=CARTESIAN_POINT('Ctrl Pts',(44.008523455373,38.2063178806684,46.934959322801));
#24527=CARTESIAN_POINT('Ctrl Pts',(44.0144645268454,38.2056196053928,46.9439869156749));
#24528=CARTESIAN_POINT('Ctrl Pts',(44.0251343926841,38.204344047837,46.9605005261727));
#24529=CARTESIAN_POINT('Ctrl Pts',(44.0298881275316,38.2037677180478,46.9679701372034));
#24530=CARTESIAN_POINT('Ctrl Pts',(44.0400581925859,38.2025170270191,46.9841960387369));
#24531=CARTESIAN_POINT('Ctrl Pts',(44.0454561568118,38.2018420092287,46.9929634605411));
#24532=CARTESIAN_POINT('Ctrl Pts',(44.0600054373806,38.199991425817,47.0170238460025));
#24533=CARTESIAN_POINT('Ctrl Pts',(44.0690152352166,38.1988107505105,47.0324007649544));
#24534=CARTESIAN_POINT('Ctrl Pts',(44.1176546217441,38.1922387343321,47.1181140934827));
#24535=CARTESIAN_POINT('Ctrl Pts',(44.1530466289284,38.1866984006722,47.190750619225));
#24536=CARTESIAN_POINT('Ctrl Pts',(44.2322888929989,38.1721134479023,47.3831647708215));
#24537=CARTESIAN_POINT('Ctrl Pts',(44.2690091596579,38.1629128345966,47.505460373763));
#24538=CARTESIAN_POINT('Ctrl Pts',(44.3054362809851,38.149469917971,47.6921054779624));
#24539=CARTESIAN_POINT('Ctrl Pts',(44.3144503266707,38.145091486024,47.7543007512472));
#24540=CARTESIAN_POINT('Ctrl Pts',(44.321437675373,38.140130268204,47.8275588564956));
#24541=CARTESIAN_POINT('Ctrl Pts',(44.3223710070259,38.1394080991493,47.8382952912293));
#24542=CARTESIAN_POINT('Ctrl Pts',(44.3236729216371,38.1383006350748,47.854881466209));
#24543=CARTESIAN_POINT('Ctrl Pts',(44.3241048825643,38.1379119722042,47.860725804802));
#24544=CARTESIAN_POINT('Ctrl Pts',(44.3248548435972,38.1371956140276,47.8715429416073));
#24545=CARTESIAN_POINT('Ctrl Pts',(44.325180209317,38.1368675307165,47.8765149914305));
#24546=CARTESIAN_POINT('Ctrl Pts',(44.3258800302165,38.1361199314396,47.8878851518256));
#24547=CARTESIAN_POINT('Ctrl Pts',(44.3262418698489,38.1357011226355,47.8942839098425));
#24548=CARTESIAN_POINT('Ctrl Pts',(44.3271085100355,38.1346055335085,47.9110954244415));
#24549=CARTESIAN_POINT('Ctrl Pts',(44.3275608152474,38.1339315558168,47.9215108407627));
#24550=CARTESIAN_POINT('Ctrl Pts',(44.330602046884,38.1283935028826,48.007646448082));
#24551=CARTESIAN_POINT('Ctrl Pts',(44.3288129001901,38.1237460055738,48.0834647323864));
#24552=CARTESIAN_POINT('Ctrl Pts',(44.3134294778128,38.1124832129306,48.2694874058114));
#24553=CARTESIAN_POINT('Ctrl Pts',(44.2947827881961,38.1059655818114,48.3789917164589));
#24554=CARTESIAN_POINT('Ctrl Pts',(44.245711657485,38.0941960435457,48.5673725662768));
#24555=CARTESIAN_POINT('Ctrl Pts',(44.2193328286842,38.0890394078023,48.646984246574));
#24556=CARTESIAN_POINT('Ctrl Pts',(44.1812737444074,38.0825917940524,48.740887565833));
#24557=CARTESIAN_POINT('Ctrl Pts',(44.1744603679558,38.0814679571615,48.7570607027052));
#24558=CARTESIAN_POINT('Ctrl Pts',(44.1633666564329,38.0796834401741,48.7824214080142));
#24559=CARTESIAN_POINT('Ctrl Pts',(44.1592328354569,38.0790277670848,48.7916723115531));
#24560=CARTESIAN_POINT('Ctrl Pts',(44.1513449762753,38.0777935572384,48.8089573316478));
#24561=CARTESIAN_POINT('Ctrl Pts',(44.1476080317465,38.0772156226168,48.816998992225));
#24562=CARTESIAN_POINT('Ctrl Pts',(44.1391019866668,38.0759149699601,48.8349780413386));
#24563=CARTESIAN_POINT('Ctrl Pts',(44.1343029238249,38.0751912248091,48.8449008281262));
#24564=CARTESIAN_POINT('Ctrl Pts',(44.1218450636452,38.073337437284,48.870105930736));
#24565=CARTESIAN_POINT('Ctrl Pts',(44.1140678263621,38.0722032857657,48.885328305437));
#24566=CARTESIAN_POINT('Ctrl Pts',(44.0533122374122,38.0635127370108,49.0004430373963));
#24567=CARTESIAN_POINT('Ctrl Pts',(43.9918550135485,38.0556510387715,49.0955898828234));
#24568=CARTESIAN_POINT('Ctrl Pts',(43.8356244396221,38.0375910909269,49.2963423551251));
#24569=CARTESIAN_POINT('Ctrl Pts',(43.7368179572382,38.0273443997952,49.3980135428803));
#24570=CARTESIAN_POINT('Ctrl Pts',(43.6116223334799,38.0162341301515,49.5013171136203));
#24571=CARTESIAN_POINT('Ctrl Pts',(43.5952406139366,38.0148136520421,49.5143915339451));
#24572=CARTESIAN_POINT('Ctrl Pts',(43.5726032867357,38.0128992348627,49.5318623947231));
#24573=CARTESIAN_POINT('Ctrl Pts',(43.5665305189835,38.0123903256665,49.5364919191376));
#24574=CARTESIAN_POINT('Ctrl Pts',(43.5562956461419,38.0115406303185,49.5441987320435));
#24575=CARTESIAN_POINT('Ctrl Pts',(43.552148403139,38.0111985103501,49.5472955130144));
#24576=CARTESIAN_POINT('Ctrl Pts',(43.5442286455974,38.0105494044313,49.5531597640408));
#24577=CARTESIAN_POINT('Ctrl Pts',(43.540458462733,38.010242200991,49.5559302497188));
#24578=CARTESIAN_POINT('Ctrl Pts',(43.5314525312783,38.0095125592745,49.5624978580046));
#24579=CARTESIAN_POINT('Ctrl Pts',(43.5262076516921,38.0090909762904,49.5662824505859));
#24580=CARTESIAN_POINT('Ctrl Pts',(43.5074800908337,38.0075971290453,49.5796531503095));
#24581=CARTESIAN_POINT('Ctrl Pts',(43.4938928023392,38.0065343265305,49.5890924479047));
#24582=CARTESIAN_POINT('Ctrl Pts',(43.3990021682629,37.9992434871589,49.6532204960091));
#24583=CARTESIAN_POINT('Ctrl Pts',(43.3137462156888,37.993349422584,49.7018272747386));
#24584=CARTESIAN_POINT('Ctrl Pts',(43.1281716410722,37.9810819937308,49.7896426472311));
#24585=CARTESIAN_POINT('Ctrl Pts',(43.0275328132674,37.9747321865891,49.8273631148328));
#24586=CARTESIAN_POINT('Ctrl Pts',(42.8860712856132,37.9657252336868,49.8673119171781));
#24587=CARTESIAN_POINT('Ctrl Pts',(42.8475381334365,37.9632653987664,49.876919925449));
#24588=CARTESIAN_POINT('Ctrl Pts',(42.7809075769987,37.9589804295541,49.8913653523718));
#24589=CARTESIAN_POINT('Ctrl Pts',(42.7529484643632,37.9571730984245,49.8967816758628));
#24590=CARTESIAN_POINT('Ctrl Pts',(42.7128086705744,37.9545604135965,49.9036394835358));
#24591=CARTESIAN_POINT('Ctrl Pts',(42.7007173875253,37.9537710925186,49.9055869408502));
#24592=CARTESIAN_POINT('Ctrl Pts',(42.6796831166216,37.9523936127224,49.9087696035394));
#24593=CARTESIAN_POINT('Ctrl Pts',(42.6707483877105,37.9518071397987,49.9100574208714));
#24594=CARTESIAN_POINT('Ctrl Pts',(42.6534980129453,37.9506720690815,49.9124203555728));
#24595=CARTESIAN_POINT('Ctrl Pts',(42.645183734059,37.9501237575855,49.9135040610787));
#24596=CARTESIAN_POINT('Ctrl Pts',(42.6254354936514,37.9488183520545,49.9159472791148));
#24597=CARTESIAN_POINT('Ctrl Pts',(42.6139960114156,37.9480597561804,49.9172586772337));
#24598=CARTESIAN_POINT('Ctrl Pts',(42.573154955329,37.9453424262621,49.9215705455976));
#24599=CARTESIAN_POINT('Ctrl Pts',(42.5436982817441,37.9433658527993,49.9239975673861));
#24600=CARTESIAN_POINT('Ctrl Pts',(42.3571382620817,37.9307356183577,49.9350607728096));
#24601=CARTESIAN_POINT('Ctrl Pts',(42.1995527190802,37.9194952146165,49.925123481119));
#24602=CARTESIAN_POINT('Ctrl Pts',(41.9814009092743,37.9036617675993,49.884276695539));
#24603=CARTESIAN_POINT('Ctrl Pts',(41.9184766450361,37.8990719270222,49.8691870468411));
#24604=CARTESIAN_POINT('Ctrl Pts',(41.8355561037461,37.8930797482899,49.8448356947448));
#24605=CARTESIAN_POINT('Ctrl Pts',(41.8147908688387,37.8915841490299,49.8383541572236));
#24606=CARTESIAN_POINT('Ctrl Pts',(41.7941388317907,37.8901046061668,49.8315225365133));
#24607=CARTESIAN_POINT('Origin',(42.4,48.4493818343519,48.));
#24608=CARTESIAN_POINT('',(41.7941388333426,36.925511940895,49.8315225370267));
#24609=CARTESIAN_POINT('',(41.794138668834,37.0981147778663,49.8315224826078));
#24610=CARTESIAN_POINT('',(41.7941388317924,48.4493818343519,49.8315225365138));
#24611=CARTESIAN_POINT('Ctrl Pts',(41.7941388333426,36.925511940895,49.8315225370267));
#24612=CARTESIAN_POINT('Ctrl Pts',(41.8060345762917,36.926294977607,49.8354576066508));
#24613=CARTESIAN_POINT('Ctrl Pts',(41.817968681362,36.9270813457443,49.839276790227));
#24614=CARTESIAN_POINT('Ctrl Pts',(41.8543274298654,36.9294805522131,49.8505230830555));
#24615=CARTESIAN_POINT('Ctrl Pts',(41.8788617517728,36.9311042214315,49.8575815092058));
#24616=CARTESIAN_POINT('Ctrl Pts',(41.9148648790757,36.933497124824,49.867170081126));
#24617=CARTESIAN_POINT('Ctrl Pts',(41.9262288312078,36.9342538806049,49.8700858448245));
#24618=CARTESIAN_POINT('Ctrl Pts',(41.9463069684267,36.9355938327101,49.87504274115));
#24619=CARTESIAN_POINT('Ctrl Pts',(41.9550101639066,36.9361756099049,49.8771272437635));
#24620=CARTESIAN_POINT('Ctrl Pts',(41.9732093993492,36.9373942948904,49.8813524640453));
#24621=CARTESIAN_POINT('Ctrl Pts',(41.9827077469165,36.9380315440896,49.8834820095747));
#24622=CARTESIAN_POINT('Ctrl Pts',(42.0075782914191,36.9397034710488,49.8888606659938));
#24623=CARTESIAN_POINT('Ctrl Pts',(42.0229745216687,36.9407418223874,49.8919939684465));
#24624=CARTESIAN_POINT('Ctrl Pts',(42.088457553686,36.9451733056218,49.9044894701625));
#24625=CARTESIAN_POINT('Ctrl Pts',(42.1388625314101,36.9486227073296,49.9120526243647));
#24626=CARTESIAN_POINT('Ctrl Pts',(42.3414500871881,36.9626463664976,49.9342906382361));
#24627=CARTESIAN_POINT('Ctrl Pts',(42.4948275987231,36.9736778486032,49.9328487185738));
#24628=CARTESIAN_POINT('Ctrl Pts',(42.6942737474017,36.9879415379767,49.9071643443188));
#24629=CARTESIAN_POINT('Ctrl Pts',(42.7419067904804,36.9913362025543,49.8992033183142));
#24630=CARTESIAN_POINT('Ctrl Pts',(42.8073385398224,36.9959428616924,49.8857256079213));
#24631=CARTESIAN_POINT('Ctrl Pts',(42.8254291772253,36.9972104077715,49.8817268200415));
#24632=CARTESIAN_POINT('Ctrl Pts',(42.8567910341496,36.9993940081145,49.8743191126987));
#24633=CARTESIAN_POINT('Ctrl Pts',(42.8700885109143,37.0003155008391,49.8710283277702));
#24634=CARTESIAN_POINT('Ctrl Pts',(42.8895957424663,37.0016597745725,49.8659796849242));
#24635=CARTESIAN_POINT('Ctrl Pts',(42.8958331854637,37.002088465589,49.8643319529452));
#24636=CARTESIAN_POINT('Ctrl Pts',(42.9068344948969,37.0028424102396,49.8613666429615));
#24637=CARTESIAN_POINT('Ctrl Pts',(42.9116016937555,37.0031683909764,49.8600620133947));
#24638=CARTESIAN_POINT('Ctrl Pts',(42.9219665441837,37.0038755334002,49.8571826228401));
#24639=CARTESIAN_POINT('Ctrl Pts',(42.9275621161994,37.0042562870459,49.8556008686084));
#24640=CARTESIAN_POINT('Ctrl Pts',(42.9430257522519,37.0053059552818,49.8511540112982));
#24641=CARTESIAN_POINT('Ctrl Pts',(42.9528783804659,37.0059718535566,49.8482352796313));
#24642=CARTESIAN_POINT('Ctrl Pts',(43.0064975001434,37.009582307764,49.8318840655602));
#24643=CARTESIAN_POINT('Ctrl Pts',(43.0498023112808,37.0124493275329,49.8169744512251));
#24644=CARTESIAN_POINT('Ctrl Pts',(43.256970262587,37.0261108048817,49.7372915811473));
#24645=CARTESIAN_POINT('Ctrl Pts',(43.4119677859631,37.0362407854834,49.6518202102932));
#24646=CARTESIAN_POINT('Ctrl Pts',(43.5968909569512,37.0504280829964,49.5139228794145));
#24647=CARTESIAN_POINT('Ctrl Pts',(43.6391609562452,37.0538320189597,49.4795234811528));
#24648=CARTESIAN_POINT('Ctrl Pts',(43.6915296575464,37.0582985695638,49.4330857017385));
#24649=CARTESIAN_POINT('Ctrl Pts',(43.7030181820937,37.0592946991623,49.422647911177));
#24650=CARTESIAN_POINT('Ctrl Pts',(43.7214741274392,37.0609224030172,49.4054688321503));
#24651=CARTESIAN_POINT('Ctrl Pts',(43.728519034571,37.0615503847009,49.3988115229383));
#24652=CARTESIAN_POINT('Ctrl Pts',(43.7419810344977,37.0627634809693,49.3858967456898));
#24653=CARTESIAN_POINT('Ctrl Pts',(43.7484052881546,37.0633482474514,49.3796470784079));
#24654=CARTESIAN_POINT('Ctrl Pts',(43.7630609656262,37.0646959769885,49.3651895409924));
#24655=CARTESIAN_POINT('Ctrl Pts',(43.7712621512257,37.0654602568066,49.3569516503467));
#24656=CARTESIAN_POINT('Ctrl Pts',(43.7966406006525,37.0678575088682,49.3309945921986));
#24657=CARTESIAN_POINT('Ctrl Pts',(43.8135520596582,37.0695019057727,49.3130202017218));
#24658=CARTESIAN_POINT('Ctrl Pts',(43.9256237062896,37.0807280782194,49.1892295018467));
#24659=CARTESIAN_POINT('Ctrl Pts',(44.0091501720827,37.0907935804863,49.0735063237269));
#24660=CARTESIAN_POINT('Ctrl Pts',(44.1192965609647,37.1067772291639,48.878750262007));
#24661=CARTESIAN_POINT('Ctrl Pts',(44.154879051092,37.1126032493256,48.8053469019537));
#24662=CARTESIAN_POINT('Ctrl Pts',(44.1953884290047,37.1200577004435,48.7062412737482));
#24663=CARTESIAN_POINT('Ctrl Pts',(44.2045918771911,37.1218219853662,48.6823815916965));
#24664=CARTESIAN_POINT('Ctrl Pts',(44.2192922108447,37.1247573763274,48.6418915803677));
#24665=CARTESIAN_POINT('Ctrl Pts',(44.2250417918035,37.1259398830866,48.6253570665403));
#24666=CARTESIAN_POINT('Ctrl Pts',(44.2328119474277,37.1275860577485,48.6019913548318));
#24667=CARTESIAN_POINT('Ctrl Pts',(44.2350207761071,37.1280599014165,48.5952243116268));
#24668=CARTESIAN_POINT('Ctrl Pts',(44.2387412432922,37.1288680940063,48.5836085917102));
#24669=CARTESIAN_POINT('Ctrl Pts',(44.2402712714225,37.1292035001485,48.5787659269039));
#24670=CARTESIAN_POINT('Ctrl Pts',(44.2432109231775,37.1298538446012,48.5693321638626));
#24671=CARTESIAN_POINT('Ctrl Pts',(44.2446225388257,37.1301689069782,48.5647418088313));
#24672=CARTESIAN_POINT('Ctrl Pts',(44.2484449432028,37.1310298430793,48.5521446976991));
#24673=CARTESIAN_POINT('Ctrl Pts',(44.2508208749326,37.1315737198112,48.5441273476092));
#24674=CARTESIAN_POINT('Ctrl Pts',(44.2599107675537,37.1336903457472,48.5127058686927));
#24675=CARTESIAN_POINT('Ctrl Pts',(44.2662338646827,37.1352421570881,48.4891898049213));
#24676=CARTESIAN_POINT('Ctrl Pts',(44.3090381727509,37.1464090212368,48.3170647232475));
#24677=CARTESIAN_POINT('Ctrl Pts',(44.328171925458,37.1552965366678,48.1646866814955));
#24678=CARTESIAN_POINT('Ctrl Pts',(44.3296338122186,37.1698679015916,47.9222736510853));
#24679=CARTESIAN_POINT('Ctrl Pts',(44.3239631914961,37.1753198616714,47.8329943418672));
#24680=CARTESIAN_POINT('Ctrl Pts',(44.3090400614135,37.1824383753172,47.7213396978242));
#24681=CARTESIAN_POINT('Ctrl Pts',(44.3055350598471,37.1839229979152,47.6983021695107));
#24682=CARTESIAN_POINT('Ctrl Pts',(44.2997094343599,37.1861481075846,47.664180616244));
#24683=CARTESIAN_POINT('Ctrl Pts',(44.2977070429041,37.186878513836,47.6530438589525));
#24684=CARTESIAN_POINT('Ctrl Pts',(44.2939553795354,37.1881888307152,47.6331829647005));
#24685=CARTESIAN_POINT('Ctrl Pts',(44.292243492506,37.1887675334921,47.6244520301376));
#24686=CARTESIAN_POINT('Ctrl Pts',(44.2884894182793,37.1899975163054,47.6059831623475));
#24687=CARTESIAN_POINT('Ctrl Pts',(44.286432173291,37.1906492636461,47.5962485906201));
#24688=CARTESIAN_POINT('Ctrl Pts',(44.2807206618891,37.1924014188702,47.5702195847155));
#24689=CARTESIAN_POINT('Ctrl Pts',(44.2769300381581,37.1935061712577,47.5539562630075));
#24690=CARTESIAN_POINT('Ctrl Pts',(44.2583395928054,37.1986706530152,47.4786330029873));
#24691=CARTESIAN_POINT('Ctrl Pts',(44.2409616301131,37.2028124663578,47.4202513614452));
#24692=CARTESIAN_POINT('Ctrl Pts',(44.1736034541804,37.2169419470818,47.2277713336924));
#24693=CARTESIAN_POINT('Ctrl Pts',(44.1114826442367,37.2272698071009,47.0984318150873));
#24694=CARTESIAN_POINT('Ctrl Pts',(44.0107973237218,37.2407295459482,46.9374220286937));
#24695=CARTESIAN_POINT('Ctrl Pts',(43.9845010624469,37.244022918802,46.8985932038399));
#24696=CARTESIAN_POINT('Ctrl Pts',(43.9408598025008,37.2491159395384,46.8389558381092));
#24697=CARTESIAN_POINT('Ctrl Pts',(43.9244477134863,37.2509566001855,46.8174891852747));
#24698=CARTESIAN_POINT('Ctrl Pts',(43.9023515033295,37.2533321242968,46.7898128297121));
#24699=CARTESIAN_POINT('Ctrl Pts',(43.8970710243374,37.2538924591732,46.7832866479017));
#24700=CARTESIAN_POINT('Ctrl Pts',(43.888362451477,37.2548043296976,46.7726661909366));
#24701=CARTESIAN_POINT('Ctrl Pts',(43.8849597304916,37.2551576260458,46.7685513951476));
#24702=CARTESIAN_POINT('Ctrl Pts',(43.8782734686682,37.2558459163128,46.7605339377026));
#24703=CARTESIAN_POINT('Ctrl Pts',(43.8749914751714,37.256181009304,46.7566300965399));
#24704=CARTESIAN_POINT('Ctrl Pts',(43.8676165605556,37.2569279671385,46.7479281327418));
#24705=CARTESIAN_POINT('Ctrl Pts',(43.8635154762454,37.2573392412833,46.7431369274583));
#24706=CARTESIAN_POINT('Ctrl Pts',(43.8491985152274,37.2587612140411,46.7265758329303));
#24707=CARTESIAN_POINT('Ctrl Pts',(43.8388632413289,37.259763596078,46.7149093200139));
#24708=CARTESIAN_POINT('Ctrl Pts',(43.7431381137568,37.2688441759801,46.609457153374));
#24709=CARTESIAN_POINT('Ctrl Pts',(43.6488223123056,37.2763497065289,46.5241675166809));
#24710=CARTESIAN_POINT('Ctrl Pts',(43.4865640938745,37.2883866339599,46.4042139931791));
#24711=CARTESIAN_POINT('Ctrl Pts',(43.423784525815,37.2928638526135,46.3632291252425));
#24712=CARTESIAN_POINT('Ctrl Pts',(43.3030395794736,37.3013667031375,46.2940724315528));
#24713=CARTESIAN_POINT('Ctrl Pts',(43.2457405536162,37.3053598864243,46.2649521753635));
#24714=CARTESIAN_POINT('Ctrl Pts',(43.1721824553614,37.310495361995,46.2320792465237));
#24715=CARTESIAN_POINT('Ctrl Pts',(43.1571811669382,37.3115430235403,46.2256025842955));
#24716=CARTESIAN_POINT('Ctrl Pts',(43.1329882111123,37.3132340284976,46.2155201656794));
#24717=CARTESIAN_POINT('Ctrl Pts',(43.1238477732688,37.3138732320851,46.2117929672905));
#24718=CARTESIAN_POINT('Ctrl Pts',(43.1064002885805,37.3150941544965,46.2048340928264));
#24719=CARTESIAN_POINT('Ctrl Pts',(43.098098639228,37.3156754185127,46.2015895108764));
#24720=CARTESIAN_POINT('Ctrl Pts',(43.0790768763525,37.3170082034382,46.1943066767072));
#24721=CARTESIAN_POINT('Ctrl Pts',(43.0683427643728,37.3177609680659,46.1903061801944));
#24722=CARTESIAN_POINT('Ctrl Pts',(43.0349772913259,37.320103237105,46.1782085390536));
#24723=CARTESIAN_POINT('Ctrl Pts',(43.0122304994892,37.3217035113785,46.1704388465869));
#24724=CARTESIAN_POINT('Ctrl Pts',(42.841747099017,37.333727869541,46.1157415837748));
#24725=CARTESIAN_POINT('Ctrl Pts',(42.6890058690732,37.3447388992426,46.0863575198811));
#24726=CARTESIAN_POINT('Ctrl Pts',(42.4616007185982,37.3610206129566,46.0704719933373));
#24727=CARTESIAN_POINT('Ctrl Pts',(42.3885338187064,37.3662228527457,46.0695226495647));
#24728=CARTESIAN_POINT('Ctrl Pts',(42.2916156436767,37.3729641635258,46.0737676599795));
#24729=CARTESIAN_POINT('Ctrl Pts',(42.2676666149053,37.3746167797358,46.0752646458915));
#24730=CARTESIAN_POINT('Ctrl Pts',(42.2271184787695,37.3773858671642,46.078559656993));
#24731=CARTESIAN_POINT('Ctrl Pts',(42.2105038604399,37.3785122235328,46.0801270168205));
#24732=CARTESIAN_POINT('Ctrl Pts',(42.1869668740035,37.3800941725693,46.0826559459354));
#24733=CARTESIAN_POINT('Ctrl Pts',(42.1800267192449,37.380558934833,46.0834397755508));
#24734=CARTESIAN_POINT('Ctrl Pts',(42.1680698577809,37.3813565530821,46.0848560028054));
#24735=CARTESIAN_POINT('Ctrl Pts',(42.1630511434674,37.3816903957373,46.0854704591711));
#24736=CARTESIAN_POINT('Ctrl Pts',(42.152538837011,37.3823876265515,46.0867994831837));
#24737=CARTESIAN_POINT('Ctrl Pts',(42.1470458569659,37.3827507931034,46.0875179874896));
#24738=CARTESIAN_POINT('Ctrl Pts',(42.1323389165952,37.3837202220535,46.0895061874315));
#24739=CARTESIAN_POINT('Ctrl Pts',(42.1231307760607,37.3843241203496,46.0908188915755));
#24740=CARTESIAN_POINT('Ctrl Pts',(42.0819255196667,37.387014183275,46.096997465374));
#24741=CARTESIAN_POINT('Ctrl Pts',(42.0500423607073,37.3890623831829,46.1026017908161));
#24742=CARTESIAN_POINT('Ctrl Pts',(41.879595587157,37.3999057214379,46.1370055445229));
#24743=CARTESIAN_POINT('Ctrl Pts',(41.7443670970048,37.4081552299275,46.18018606003));
#24744=CARTESIAN_POINT('Ctrl Pts',(41.5322156671077,37.4221077569098,46.2746827502607));
#24745=CARTESIAN_POINT('Ctrl Pts',(41.4520770664198,37.4276372464387,46.3173804648249));
#24746=CARTESIAN_POINT('Ctrl Pts',(41.3553568345844,37.4348498628924,46.3780215173));
#24747=CARTESIAN_POINT('Ctrl Pts',(41.3356993450523,37.4363452071428,46.3908519083714));
#24748=CARTESIAN_POINT('Ctrl Pts',(41.3068931453071,37.4385832960766,46.4104123981866));
#24749=CARTESIAN_POINT('Ctrl Pts',(41.2975613844119,37.4393157839426,46.4168700529033));
#24750=CARTESIAN_POINT('Ctrl Pts',(41.2810130791843,37.4406284072515,46.4285388798066));
#24751=CARTESIAN_POINT('Ctrl Pts',(41.2737745456599,37.4412073182274,46.4337184152365));
#24752=CARTESIAN_POINT('Ctrl Pts',(41.2585364198354,37.4424362388853,46.4447823085724));
#24753=CARTESIAN_POINT('Ctrl Pts',(41.250545925606,37.4430867050916,46.4506786978925));
#24754=CARTESIAN_POINT('Ctrl Pts',(41.229311625625,37.4448317615975,46.4666027151973));
#24755=CARTESIAN_POINT('Ctrl Pts',(41.2161514654952,37.4459306352323,46.4767399694097));
#24756=CARTESIAN_POINT('Ctrl Pts',(41.1566781457875,37.4509779809276,46.5237884324047));
#24757=CARTESIAN_POINT('Ctrl Pts',(41.1119533659701,37.455003807069,46.5626467307444));
#24758=CARTESIAN_POINT('Ctrl Pts',(40.9512944671883,37.4703651482437,46.7157595434215));
#24759=CARTESIAN_POINT('Ctrl Pts',(40.8481814416517,37.4821848649888,46.8424728567648));
#24760=CARTESIAN_POINT('Ctrl Pts',(40.7435926760575,37.4961011672469,47.0105057331523));
#24761=CARTESIAN_POINT('Ctrl Pts',(40.7257949091819,37.498554993609,47.0409266241879));
#24762=CARTESIAN_POINT('Ctrl Pts',(40.6981867638974,37.5024882830913,47.0912291418198));
#24763=CARTESIAN_POINT('Ctrl Pts',(40.6878684074296,37.5039905798036,47.1108215721562));
#24764=CARTESIAN_POINT('Ctrl Pts',(40.6743742013247,37.5059960368236,47.1375505882188));
#24765=CARTESIAN_POINT('Ctrl Pts',(40.6709014564426,37.5065160093268,47.1445342690819));
#24766=CARTESIAN_POINT('Ctrl Pts',(40.6651793750562,37.5073790655705,47.1562185669369));
#24767=CARTESIAN_POINT('Ctrl Pts',(40.6629065911517,37.5077235715462,47.1609075150205));
#24768=CARTESIAN_POINT('Ctrl Pts',(40.6586409192041,37.5083733290271,47.1697995754708));
#24769=CARTESIAN_POINT('Ctrl Pts',(40.6566441926893,37.5086788239434,47.1740007727454));
#24770=CARTESIAN_POINT('Ctrl Pts',(40.6519548226461,37.5093996002311,47.18396015989));
#24771=CARTESIAN_POINT('Ctrl Pts',(40.6492753847375,37.5098140753305,47.1897245610128));
#24772=CARTESIAN_POINT('Ctrl Pts',(40.6400035175406,37.5112579908241,47.209932279821));
#24773=CARTESIAN_POINT('Ctrl Pts',(40.6335607236798,37.5122787737353,47.2244441070733));
#24774=CARTESIAN_POINT('Ctrl Pts',(40.5793011709017,37.5210448826691,47.3508440891409));
#24775=CARTESIAN_POINT('Ctrl Pts',(40.5419836366834,37.5282657885556,47.4669604383437));
#24776=CARTESIAN_POINT('Ctrl Pts',(40.4859803649962,37.5438238508871,47.721732834052));
#24777=CARTESIAN_POINT('Ctrl Pts',(40.4709013140451,37.5521462336006,47.8604462285944));
#24778=CARTESIAN_POINT('Ctrl Pts',(40.470866204085,37.562069016386,48.0166737762658));
#24779=CARTESIAN_POINT('Ctrl Pts',(40.4710899182901,37.563162280457,48.0337799347538));
#24780=CARTESIAN_POINT('Ctrl Pts',(40.4718319635774,37.5649719579374,48.0619047739402));
#24781=CARTESIAN_POINT('Ctrl Pts',(40.4722173529074,37.5656842098326,48.0729262294255));
#24782=CARTESIAN_POINT('Ctrl Pts',(40.4730831965717,37.5669747231676,48.092805566662));
#24783=CARTESIAN_POINT('Ctrl Pts',(40.4735302922043,37.5675519215008,48.1016646500113));
#24784=CARTESIAN_POINT('Ctrl Pts',(40.4746190292379,37.5687926765634,48.120637339368));
#24785=CARTESIAN_POINT('Ctrl Pts',(40.4752792944777,37.5694568021974,48.1307495670864));
#24786=CARTESIAN_POINT('Ctrl Pts',(40.4773003618044,37.5712777813411,48.1583557450754));
#24787=CARTESIAN_POINT('Ctrl Pts',(40.4788201922457,37.572439591095,48.1758367203876));
#24788=CARTESIAN_POINT('Ctrl Pts',(40.4889616628486,37.5791848325426,48.2765421453077));
#24789=CARTESIAN_POINT('Ctrl Pts',(40.5027507964943,37.584929520007,48.3591449415101));
#24790=CARTESIAN_POINT('Ctrl Pts',(40.5470819389444,37.5985471708437,48.5481226780583));
#24791=CARTESIAN_POINT('Ctrl Pts',(40.581498171747,37.606494200744,48.653293396967));
#24792=CARTESIAN_POINT('Ctrl Pts',(40.6545761214094,37.619765989015,48.8251416705001));
#24793=CARTESIAN_POINT('Ctrl Pts',(40.688574760283,37.6251258515477,48.8935265141757));
#24794=CARTESIAN_POINT('Ctrl Pts',(40.7317306331961,37.6309827355547,48.9687769510339));
#24795=CARTESIAN_POINT('Ctrl Pts',(40.7369958179616,37.6316833069803,48.9777875860359));
#24796=CARTESIAN_POINT('Ctrl Pts',(40.7456142923333,37.6328072367718,48.9922658989641));
#24797=CARTESIAN_POINT('Ctrl Pts',(40.7489220967485,37.6332333407615,48.9977602138346));
#24798=CARTESIAN_POINT('Ctrl Pts',(40.7548493973254,37.6339874617808,49.0074953574341));
#24799=CARTESIAN_POINT('Ctrl Pts',(40.7574579936243,37.6343161657963,49.0117426352487));
#24800=CARTESIAN_POINT('Ctrl Pts',(40.7631694910493,37.6350289582747,49.0209616965136));
#24801=CARTESIAN_POINT('Ctrl Pts',(40.7662785985618,37.6354126337587,49.025929473948));
#24802=CARTESIAN_POINT('Ctrl Pts',(40.7751669443698,37.6364974920067,49.0399885315531));
#24803=CARTESIAN_POINT('Ctrl Pts',(40.7809998711022,37.6371952453438,49.0490458522051));
#24804=CARTESIAN_POINT('Ctrl Pts',(40.8212636661896,37.6419198081871,49.1104313573072));
#24805=CARTESIAN_POINT('Ctrl Pts',(40.8581534444709,37.645798710245,49.161110312538));
#24806=CARTESIAN_POINT('Ctrl Pts',(40.9771058465114,37.6573317871873,49.3088339244236));
#24807=CARTESIAN_POINT('Ctrl Pts',(41.0663394920247,37.6647602575618,49.3996520877434));
#24808=CARTESIAN_POINT('Ctrl Pts',(41.2262347611737,37.6773613220463,49.533107857091));
#24809=CARTESIAN_POINT('Ctrl Pts',(41.2918344186456,37.6823645119123,49.5811739932347));
#24810=CARTESIAN_POINT('Ctrl Pts',(41.3752779205529,37.6886642557149,49.6345656772653));
#24811=CARTESIAN_POINT('Ctrl Pts',(41.3904245530283,37.6898051166411,49.6439640130144));
#24812=CARTESIAN_POINT('Ctrl Pts',(41.4145240807677,37.6916172890748,49.6584588717224));
#24813=CARTESIAN_POINT('Ctrl Pts',(41.4233915308754,37.692283441564,49.66369603828));
#24814=CARTESIAN_POINT('Ctrl Pts',(41.4399621205037,37.693527314986,49.6733045949206));
#24815=CARTESIAN_POINT('Ctrl Pts',(41.447654286415,37.6941043463257,49.6776944402528));
#24816=CARTESIAN_POINT('Ctrl Pts',(41.4648024645625,37.6953900229255,49.6873248064568));
#24817=CARTESIAN_POINT('Ctrl Pts',(41.474272793011,37.6960995878142,49.6925390875579));
#24818=CARTESIAN_POINT('Ctrl Pts',(41.5020541806685,37.6981800369615,49.7075323649935));
#24819=CARTESIAN_POINT('Ctrl Pts',(41.5204793775371,37.6995585026626,49.7170954804915));
#24820=CARTESIAN_POINT('Ctrl Pts',(41.6093901956069,37.7062063178128,49.7614358209183));
#24821=CARTESIAN_POINT('Ctrl Pts',(41.6817944141776,37.7116125554173,49.7921768662197));
#24822=CARTESIAN_POINT('Ctrl Pts',(41.768578352681,37.7180730212865,49.8229183237142));
#24823=CARTESIAN_POINT('Ctrl Pts',(41.7813375499239,37.7190222414624,49.8272879181221));
#24824=CARTESIAN_POINT('Ctrl Pts',(41.7941388718785,37.7199737694749,49.8315225497742));
#24825=CARTESIAN_POINT('Ctrl Pts',(41.7941388317907,37.8901046061668,49.8315225365133));
#24826=CARTESIAN_POINT('Ctrl Pts',(41.7936175134844,37.8900672581426,49.831350086264));
#24827=CARTESIAN_POINT('Ctrl Pts',(41.7930962673079,37.8900299203585,49.8311774129395));
#24828=CARTESIAN_POINT('Ctrl Pts',(41.7775906461537,37.8889193776992,49.8260335149338));
#24829=CARTESIAN_POINT('Ctrl Pts',(41.7626671831116,37.8878547612407,49.8208785575848));
#24830=CARTESIAN_POINT('Ctrl Pts',(41.741380515005,37.8863439509835,49.8132318043135));
#24831=CARTESIAN_POINT('Ctrl Pts',(41.7349651065048,37.8858896374652,49.8108886758016));
#24832=CARTESIAN_POINT('Ctrl Pts',(41.7238455115517,37.8851041279316,49.8067603542927));
#24833=CARTESIAN_POINT('Ctrl Pts',(41.7191356651461,37.8847720256459,49.8049907562126));
#24834=CARTESIAN_POINT('Ctrl Pts',(41.7091904720039,37.8840721107104,49.8012096506244));
#24835=CARTESIAN_POINT('Ctrl Pts',(41.7039569347537,37.8837045639093,49.7991937257514));
#24836=CARTESIAN_POINT('Ctrl Pts',(41.6897736712279,37.8827103990024,49.7936592746756));
#24837=CARTESIAN_POINT('Ctrl Pts',(41.6808411984499,37.8820863599445,49.7900965502503));
#24838=CARTESIAN_POINT('Ctrl Pts',(41.6387554072491,37.8791543059777,49.7729447258289));
#24839=CARTESIAN_POINT('Ctrl Pts',(41.6059559311538,37.8768931595464,49.7584995689046));
#24840=CARTESIAN_POINT('Ctrl Pts',(41.5409849409625,37.8724257336572,49.7276968973652));
#24841=CARTESIAN_POINT('Ctrl Pts',(41.508832473336,37.8702208021449,49.7113340211458));
#24842=CARTESIAN_POINT('Ctrl Pts',(41.3745965089642,37.8609637208791,49.6382094170411));
#24843=CARTESIAN_POINT('Ctrl Pts',(41.2773210319681,37.8541116161374,49.5731419845162));
#24844=CARTESIAN_POINT('Ctrl Pts',(41.1204299356666,37.8419166407192,49.4461922574094));
#24845=CARTESIAN_POINT('Ctrl Pts',(41.0579494871242,37.8366872741337,49.3884053180214));
#24846=CARTESIAN_POINT('Ctrl Pts',(40.9873772697403,37.8301577496872,49.3139062785321));
#24847=CARTESIAN_POINT('Ctrl Pts',(40.9754422334157,37.8290300671449,49.3009565032879));
#24848=CARTESIAN_POINT('Ctrl Pts',(40.9569133932338,37.8272408249234,49.2802915832768));
#24849=CARTESIAN_POINT('Ctrl Pts',(40.9502001268667,37.8265843178307,49.27268449121));
#24850=CARTESIAN_POINT('Ctrl Pts',(40.9377333252335,37.8253493754633,49.258331171475));
#24851=CARTESIAN_POINT('Ctrl Pts',(40.9319656657561,37.8247715494766,49.2515975208875));
#24852=CARTESIAN_POINT('Ctrl Pts',(40.9191442527848,37.8234722462379,49.2364181714709));
#24853=CARTESIAN_POINT('Ctrl Pts',(40.9121159791754,37.822749751237,49.2279514529624));
#24854=CARTESIAN_POINT('Ctrl Pts',(40.8943943429978,37.8209013255124,49.2062272842276));
#24855=CARTESIAN_POINT('Ctrl Pts',(40.8838036056596,37.819771326238,49.1928877221357));
#24856=CARTESIAN_POINT('Ctrl Pts',(40.8072578045933,37.8114126496384,49.0938081038673));
#24857=CARTESIAN_POINT('Ctrl Pts',(40.7484527297161,37.8039060341859,49.0028102373976));
#24858=CARTESIAN_POINT('Ctrl Pts',(40.6289008794188,37.7858878480136,48.778508882103));
#24859=CARTESIAN_POINT('Ctrl Pts',(40.5750673597407,37.7752855007878,48.642255024258));
#24860=CARTESIAN_POINT('Ctrl Pts',(40.5316112131668,37.7638334714754,48.4807451187842));
#24861=CARTESIAN_POINT('Ctrl Pts',(40.5264376966115,37.762395343422,48.4601705282495));
#24862=CARTESIAN_POINT('Ctrl Pts',(40.5198565498977,37.7604612543522,48.4320439980544));
#24863=CARTESIAN_POINT('Ctrl Pts',(40.5181532817463,37.7599499339563,48.424563709172));
#24864=CARTESIAN_POINT('Ctrl Pts',(40.5153740867943,37.7590973473114,48.4120128493432));
#24865=CARTESIAN_POINT('Ctrl Pts',(40.5142739044657,37.7587547279642,48.406947804326));
#24866=CARTESIAN_POINT('Ctrl Pts',(40.5122208635655,37.7581055481189,48.3973088421006));
#24867=CARTESIAN_POINT('Ctrl Pts',(40.5112641889311,37.7577987643148,48.3927358159358));
#24868=CARTESIAN_POINT('Ctrl Pts',(40.5090280110873,37.7570712177177,48.381849431554));
#24869=CARTESIAN_POINT('Ctrl Pts',(40.507763487663,37.7566512987757,48.3755330018968));
#24870=CARTESIAN_POINT('Ctrl Pts',(40.5033939069377,37.7551689868781,48.3531239072154));
#24871=CARTESIAN_POINT('Ctrl Pts',(40.5004622076336,37.7541158676232,48.336997602995));
#24872=CARTESIAN_POINT('Ctrl Pts',(40.4799570430327,37.746265020802,48.2154204695495));
#24873=CARTESIAN_POINT('Ctrl Pts',(40.4709685654758,37.7398674548764,48.1086955161729));
#24874=CARTESIAN_POINT('Ctrl Pts',(40.4707395022945,37.7249146031399,47.8581397620656));
#24875=CARTESIAN_POINT('Ctrl Pts',(40.4866464982344,37.7163916848305,47.7149681425424));
#24876=CARTESIAN_POINT('Ctrl Pts',(40.5237838102496,37.7057607332682,47.5505819330389));
#24877=CARTESIAN_POINT('Ctrl Pts',(40.5297466586376,37.70417471704,47.5263797537508));
#24878=CARTESIAN_POINT('Ctrl Pts',(40.5391420010776,37.7018352851868,47.4911953330941));
#24879=CARTESIAN_POINT('Ctrl Pts',(40.5422066360675,37.7010937434822,47.480116850894));
#24880=CARTESIAN_POINT('Ctrl Pts',(40.5478308879236,37.6997696252662,47.460470495555));
#24881=CARTESIAN_POINT('Ctrl Pts',(40.5503514359761,37.6991883366205,47.4518917160081));
#24882=CARTESIAN_POINT('Ctrl Pts',(40.5557446033393,37.6979691608629,47.4339967953654));
#24883=CARTESIAN_POINT('Ctrl Pts',(40.5586283793337,37.6973309219276,47.4246843088805));
#24884=CARTESIAN_POINT('Ctrl Pts',(40.5663667595188,37.6956529728556,47.4003493235536));
#24885=CARTESIAN_POINT('Ctrl Pts',(40.5713353238868,37.6946095384393,47.3853641147973));
#24886=CARTESIAN_POINT('Ctrl Pts',(40.5952411834719,37.6897395073416,47.3161208694104));
#24887=CARTESIAN_POINT('Ctrl Pts',(40.6164112624952,37.6858396957832,47.2626702934077));
#24888=CARTESIAN_POINT('Ctrl Pts',(40.6865238166123,37.6740083304901,47.1064150892322));
#24889=CARTESIAN_POINT('Ctrl Pts',(40.7422069308834,37.665881784329,47.0069182001163));
#24890=CARTESIAN_POINT('Ctrl Pts',(40.8326518509076,37.6544198064664,46.8743246238609));
#24891=CARTESIAN_POINT('Ctrl Pts',(40.8603728648284,37.6510899440287,46.8366970210532));
#24892=CARTESIAN_POINT('Ctrl Pts',(40.924688540041,37.6437993726581,46.7557285390511));
#24893=CARTESIAN_POINT('Ctrl Pts',(40.961886439201,37.6398586607133,46.7129156694088));
#24894=CARTESIAN_POINT('Ctrl Pts',(41.00775342733,37.6353654466197,46.6646009745871));
#24895=CARTESIAN_POINT('Ctrl Pts',(41.0146428686088,37.6346996604662,46.6574551385845));
#24896=CARTESIAN_POINT('Ctrl Pts',(41.0259664720512,37.6336205835688,46.645890107438));
#24897=CARTESIAN_POINT('Ctrl Pts',(41.0303674296514,37.6332048791198,46.6414388633405));
#24898=CARTESIAN_POINT('Ctrl Pts',(41.0383039207166,37.6324619250366,46.6334894514279));
#24899=CARTESIAN_POINT('Ctrl Pts',(41.0418313758721,37.6321340693116,46.6299834738834));
#24900=CARTESIAN_POINT('Ctrl Pts',(41.0496283056739,37.6314145668222,46.6222937273982));
#24901=CARTESIAN_POINT('Ctrl Pts',(41.0539036840771,37.6310233985328,46.6181161419839));
#24902=CARTESIAN_POINT('Ctrl Pts',(41.0663395786764,37.6298950464938,46.6060771796823));
#24903=CARTESIAN_POINT('Ctrl Pts',(41.074550192666,37.6291617406367,46.5982675820099));
#24904=CARTESIAN_POINT('Ctrl Pts',(41.1428721001029,37.6231504363752,46.5344197209621));
#24905=CARTESIAN_POINT('Ctrl Pts',(41.206447132777,37.6181282114454,46.4821952781277));
#24906=CARTESIAN_POINT('Ctrl Pts',(41.2800162989781,37.6126734931055,46.4292516873316));
#24907=CARTESIAN_POINT('Ctrl Pts',(41.2868972695629,37.6121665814886,46.4243680425329));
#24908=CARTESIAN_POINT('Ctrl Pts',(41.4153981859246,37.6027565893435,46.3344287290135));
#24909=CARTESIAN_POINT('Ctrl Pts',(41.5463907047871,37.5940538132914,46.263648288005));
#24910=CARTESIAN_POINT('Ctrl Pts',(41.719954421196,37.5824224106004,46.1942970769385));
#24911=CARTESIAN_POINT('Ctrl Pts',(41.7561263990339,37.5799963032222,46.1810850749619));
#24912=CARTESIAN_POINT('Ctrl Pts',(41.8061235608414,37.5766279050356,46.1645016169033));
#24913=CARTESIAN_POINT('Ctrl Pts',(41.8196279948348,37.5757166446797,46.1601870047517));
#24914=CARTESIAN_POINT('Ctrl Pts',(41.8412670820739,37.5742536320947,46.1535353534401));
#24915=CARTESIAN_POINT('Ctrl Pts',(41.8493718578679,37.5737050407088,46.151102271662));
#24916=CARTESIAN_POINT('Ctrl Pts',(41.8661105023714,37.5725706213813,46.1461970942401));
#24917=CARTESIAN_POINT('Ctrl Pts',(41.8747461367017,37.5719845865806,46.1437318125979));
#24918=CARTESIAN_POINT('Ctrl Pts',(41.8949206400934,37.5706135382331,46.1381244908785));
#24919=CARTESIAN_POINT('Ctrl Pts',(41.9064720342812,37.5698270241417,46.1350293012116));
#24920=CARTESIAN_POINT('Ctrl Pts',(41.9440074348758,37.5672660839849,46.1253448556922));
#24921=CARTESIAN_POINT('Ctrl Pts',(41.970099211458,37.5654777867601,46.1191899834915));
#24922=CARTESIAN_POINT('Ctrl Pts',(42.0321655376173,37.5612026386333,46.1059078997389));
#24923=CARTESIAN_POINT('Ctrl Pts',(42.0682307381263,37.5587016719349,46.0992591088863));
#24924=CARTESIAN_POINT('Ctrl Pts',(42.2091978696957,37.5488617276344,46.0774052850129));
#24925=CARTESIAN_POINT('Ctrl Pts',(42.3150834827794,37.5413194780256,46.0698288971812));
#24926=CARTESIAN_POINT('Ctrl Pts',(42.525959346993,37.5262536441428,46.0721292676597));
#24927=CARTESIAN_POINT('Ctrl Pts',(42.6306178711824,37.5187576441944,46.081831348923));
#24928=CARTESIAN_POINT('Ctrl Pts',(42.7501625820139,37.5104944031991,46.10284454583));
#24929=CARTESIAN_POINT('Ctrl Pts',(42.7663126206386,37.5093847316243,46.1058965816952));
#24930=CARTESIAN_POINT('Ctrl Pts',(42.7887434953279,37.5078546165903,46.1104332127845));
#24931=CARTESIAN_POINT('Ctrl Pts',(42.7950583252172,37.5074250849347,46.1117433778411));
#24932=CARTESIAN_POINT('Ctrl Pts',(42.8059381656325,37.506687310305,46.1140576340681));
#24933=CARTESIAN_POINT('Ctrl Pts',(42.8105062667067,37.50637823307,46.1150466827802));
#24934=CARTESIAN_POINT('Ctrl Pts',(42.8201303920262,37.505728589119,46.1171670672088));
#24935=CARTESIAN_POINT('Ctrl Pts',(42.8251855330876,37.5053882521536,46.1183021861466));
#24936=CARTESIAN_POINT('Ctrl Pts',(42.8377042526321,37.5045475089004,46.121166256214));
#24937=CARTESIAN_POINT('Ctrl Pts',(42.8451623214394,37.5040484678945,46.1229193512287));
#24938=CARTESIAN_POINT('Ctrl Pts',(42.8731574200033,37.5021814562977,46.1296761222987));
#24939=CARTESIAN_POINT('Ctrl Pts',(42.8936230707684,37.5008292029739,46.1349730016387));
#24940=CARTESIAN_POINT('Ctrl Pts',(43.0533899702802,37.4903421419444,46.1791378891239));
#24941=CARTESIAN_POINT('Ctrl Pts',(43.1880250547904,37.4818946920488,46.2332274868453));
#24942=CARTESIAN_POINT('Ctrl Pts',(43.4118692999527,37.4666676403285,46.353888520676));
#24943=CARTESIAN_POINT('Ctrl Pts',(43.5037536390697,37.4600110566575,46.4140347763983));
#24944=CARTESIAN_POINT('Ctrl Pts',(43.6034428752972,37.4519655766891,46.4921676617587));
#24945=CARTESIAN_POINT('Ctrl Pts',(43.616718643532,37.4508761759025,46.5028597837532));
#24946=CARTESIAN_POINT('Ctrl Pts',(43.6383314795768,37.4490716922599,46.5207438100603));
#24947=CARTESIAN_POINT('Ctrl Pts',(43.6467519383969,37.4483607310096,46.5278337985858));
#24948=CARTESIAN_POINT('Ctrl Pts',(43.6618443988954,37.4470717587842,46.5407639383377));
#24949=CARTESIAN_POINT('Ctrl Pts',(43.6685377356452,37.4464948016611,46.5465788017551));
#24950=CARTESIAN_POINT('Ctrl Pts',(43.682801521875,37.4452536822939,46.5591441122663));
#24951=CARTESIAN_POINT('Ctrl Pts',(43.69035926602,37.4445889449673,46.5659085134983));
#24952=CARTESIAN_POINT('Ctrl Pts',(43.7108823808683,37.4427639959479,46.5845708790155));
#24953=CARTESIAN_POINT('Ctrl Pts',(43.7237385882742,37.4415987896344,46.5965869004962));
#24954=CARTESIAN_POINT('Ctrl Pts',(43.7975477872308,37.4347776365027,46.6674890377287));
#24955=CARTESIAN_POINT('Ctrl Pts',(43.8547232309565,37.4289560223963,46.7301566948169));
#24956=CARTESIAN_POINT('Ctrl Pts',(43.9794718063388,37.4149215863325,46.8864088297881));
#24957=CARTESIAN_POINT('Ctrl Pts',(44.0431429491775,37.4066210530261,46.9827021105529));
#24958=CARTESIAN_POINT('Ctrl Pts',(44.1148208351882,37.3959118100115,47.1155727297766));
#24959=CARTESIAN_POINT('Ctrl Pts',(44.1309258246779,37.3933904116179,47.1475223686525));
#24960=CARTESIAN_POINT('Ctrl Pts',(44.1621634790723,37.3882738203714,47.2140329172255));
#24961=CARTESIAN_POINT('Ctrl Pts',(44.1771904329341,37.3856830271622,47.2486285882515));
#24962=CARTESIAN_POINT('Ctrl Pts',(44.1948263426804,37.3824875404477,47.2927259324309));
#24963=CARTESIAN_POINT('Ctrl Pts',(44.1983890263743,37.3818331429623,47.301834456016));
#24964=CARTESIAN_POINT('Ctrl Pts',(44.203898339984,37.3808073683962,47.3162418604289));
#24965=CARTESIAN_POINT('Ctrl Pts',(44.2058911893622,37.3804333456778,47.3215227132426));
#24966=CARTESIAN_POINT('Ctrl Pts',(44.2096131108994,37.3797292204236,47.3315180183997));
#24967=CARTESIAN_POINT('Ctrl Pts',(44.2113469400763,37.3793988548974,47.3362304359815));
#24968=CARTESIAN_POINT('Ctrl Pts',(44.2153714338275,37.3786263606993,47.3473019105476));
#24969=CARTESIAN_POINT('Ctrl Pts',(44.217647103664,37.378185120806,47.3536663023927));
#24970=CARTESIAN_POINT('Ctrl Pts',(44.2249922240706,37.3767458088115,47.3745541099661));
#24971=CARTESIAN_POINT('Ctrl Pts',(44.2299215731768,37.3757555941091,47.3891266486942));
#24972=CARTESIAN_POINT('Ctrl Pts',(44.2562877589714,37.3703115103879,47.4702570380722));
#24973=CARTESIAN_POINT('Ctrl Pts',(44.2742701688066,37.3660275235868,47.5378903571943));
#24974=CARTESIAN_POINT('Ctrl Pts',(44.2953692404926,37.3597885861315,47.639115402867));
#24975=CARTESIAN_POINT('Ctrl Pts',(44.3013438573136,37.357785516413,47.6720459313911));
#24976=CARTESIAN_POINT('Ctrl Pts',(44.3293467788555,37.3468450213011,47.8530878921842));
#24977=CARTESIAN_POINT('Ctrl Pts',(44.334927978243,37.3379856866592,48.003203323262));
#24978=CARTESIAN_POINT('Ctrl Pts',(44.3211599374976,37.3269905122201,48.176883887801));
#24979=CARTESIAN_POINT('Ctrl Pts',(44.3187573750752,37.3254302265982,48.2012795669041));
#24980=CARTESIAN_POINT('Ctrl Pts',(44.314555210387,37.323121750736,48.2369626495734));
#24981=CARTESIAN_POINT('Ctrl Pts',(44.3131190536956,37.3223849834513,48.2482910148551));
#24982=CARTESIAN_POINT('Ctrl Pts',(44.3103806003394,37.3210663081327,48.2684553564751));
#24983=CARTESIAN_POINT('Ctrl Pts',(44.3091173448619,37.32048565043,48.2772963678373));
#24984=CARTESIAN_POINT('Ctrl Pts',(44.3063412809526,37.3192646107851,48.2958060962498));
#24985=CARTESIAN_POINT('Ctrl Pts',(44.3048162004491,37.3186238546289,48.3054726870846));
#24986=CARTESIAN_POINT('Ctrl Pts',(44.3006107914344,37.3169319824356,48.3308713549115));
#24987=CARTESIAN_POINT('Ctrl Pts',(44.2978087273593,37.3158770282695,48.3465822301078));
#24988=CARTESIAN_POINT('Ctrl Pts',(44.2836428882995,37.3108605820911,48.4206778793085));
#24989=CARTESIAN_POINT('Ctrl Pts',(44.2697788671548,37.3068203569583,48.4785458213757));
#24990=CARTESIAN_POINT('Ctrl Pts',(44.2239113359991,37.2953936279628,48.6372326013979));
#24991=CARTESIAN_POINT('Ctrl Pts',(44.186261663696,37.2878570981544,48.7361949094014));
#24992=CARTESIAN_POINT('Ctrl Pts',(44.0974802087398,37.273144194891,48.9220397609233));
#24993=CARTESIAN_POINT('Ctrl Pts',(44.0472662095272,37.2659941472145,49.0090165512006));
#24994=CARTESIAN_POINT('Ctrl Pts',(43.9812032349665,37.2580465122039,49.1052644473512));
#24995=CARTESIAN_POINT('Ctrl Pts',(43.9717204712065,37.2569357584839,49.1187081717325));
#24996=CARTESIAN_POINT('Ctrl Pts',(43.9582805050011,37.2554043957846,49.1372537321468));
#24997=CARTESIAN_POINT('Ctrl Pts',(43.9544682413488,37.2549746800725,49.1424590465889));
#24998=CARTESIAN_POINT('Ctrl Pts',(43.947848957908,37.2542366750473,49.1514026280646));
#24999=CARTESIAN_POINT('Ctrl Pts',(43.9450543629053,37.253927550299,49.1551499579051));
#25000=CARTESIAN_POINT('Ctrl Pts',(43.9391342436043,37.2532779076783,49.1630284482156));
#25001=CARTESIAN_POINT('Ctrl Pts',(43.936005652029,37.2529376189908,49.1671572427157));
#25002=CARTESIAN_POINT('Ctrl Pts',(43.9282112460747,37.2520971650225,49.1773578809224));
#25003=CARTESIAN_POINT('Ctrl Pts',(43.9235257761273,37.2515983629403,49.1834147230486));
#25004=CARTESIAN_POINT('Ctrl Pts',(43.9057880512276,37.2497333132278,49.2060640791116));
#25005=CARTESIAN_POINT('Ctrl Pts',(43.8924992399637,37.2483827402351,49.2224705826886));
#25006=CARTESIAN_POINT('Ctrl Pts',(43.7864039689174,37.2379283220036,49.3491472525141));
#25007=CARTESIAN_POINT('Ctrl Pts',(43.6817620436271,37.2295074347663,49.4489346340064));
#25008=CARTESIAN_POINT('Ctrl Pts',(43.4792516554998,37.2142808846742,49.6027765346566));
#25009=CARTESIAN_POINT('Ctrl Pts',(43.3860023521216,37.2075944492648,49.661767546029));
#25010=CARTESIAN_POINT('Ctrl Pts',(43.2731012140215,37.1995156788889,49.7203277483209));
#25011=CARTESIAN_POINT('Ctrl Pts',(43.2578621779031,37.1984259519915,49.7279773567782));
#25012=CARTESIAN_POINT('Ctrl Pts',(43.2326202035982,37.1966210391263,49.7402319845528));
#25013=CARTESIAN_POINT('Ctrl Pts',(43.2226754777222,37.1959099782016,49.7449552468613));
#25014=CARTESIAN_POINT('Ctrl Pts',(43.2046496533096,37.1946208991545,49.7533282944777));
#25015=CARTESIAN_POINT('Ctrl Pts',(43.196582730267,37.1940439356789,49.7570080028878));
#25016=CARTESIAN_POINT('Ctrl Pts',(43.1792349555457,37.1928028846678,49.7647771233372));
#25017=CARTESIAN_POINT('Ctrl Pts',(43.1699466819887,37.1921382226546,49.768849205335));
#25018=CARTESIAN_POINT('Ctrl Pts',(43.1444601646397,37.1903136942465,49.7797840020163));
#25019=CARTESIAN_POINT('Ctrl Pts',(43.1281998036609,37.1891488370865,49.7864985422583));
#25020=CARTESIAN_POINT('Ctrl Pts',(43.0331782900985,37.182335100671,49.8242238571027));
#25021=CARTESIAN_POINT('Ctrl Pts',(42.9525470534217,37.1765209863044,49.8502420410682));
#25022=CARTESIAN_POINT('Ctrl Pts',(42.7593007523353,37.162534957377,49.8988384664183));
#25023=CARTESIAN_POINT('Ctrl Pts',(42.6458559570098,37.1542771136271,49.9168298509069));
#25024=CARTESIAN_POINT('Ctrl Pts',(42.4959203772501,37.1436140163687,49.9270737825472));
#25025=CARTESIAN_POINT('Ctrl Pts',(42.4602826792262,37.1410995972006,49.9285176444353));
#25026=CARTESIAN_POINT('Ctrl Pts',(42.3862269337409,37.1359396937168,49.9294629909972));
#25027=CARTESIAN_POINT('Ctrl Pts',(42.347820607805,37.1333000374757,49.9288066040749));
#25028=CARTESIAN_POINT('Ctrl Pts',(42.2996288349812,37.1300535770805,49.9265422351811));
#25029=CARTESIAN_POINT('Ctrl Pts',(42.2898045073605,37.1293952034604,49.9260052747159));
#25030=CARTESIAN_POINT('Ctrl Pts',(42.2743383435585,37.1283646225048,49.9250412222961));
#25031=CARTESIAN_POINT('Ctrl Pts',(42.2686937076775,37.1279897291444,49.924664443243));
#25032=CARTESIAN_POINT('Ctrl Pts',(42.258045306268,37.1272849397764,49.9239065993204));
#25033=CARTESIAN_POINT('Ctrl Pts',(42.2530414107192,37.1269547731323,49.9235308449851));
#25034=CARTESIAN_POINT('Ctrl Pts',(42.241325219988,37.126184044992,49.922605062305));
#25035=CARTESIAN_POINT('Ctrl Pts',(42.2346142704908,37.1257443596817,49.922039405226));
#25036=CARTESIAN_POINT('Ctrl Pts',(42.2127214800651,37.124315412343,49.9200785768345));
#25037=CARTESIAN_POINT('Ctrl Pts',(42.1975527434189,37.1233338522199,49.9185385397944));
#25038=CARTESIAN_POINT('Ctrl Pts',(42.1141964382157,37.1179788914244,49.9090759563455));
#25039=CARTESIAN_POINT('Ctrl Pts',(42.0464437575831,37.1137693319594,49.8976972121558));
#25040=CARTESIAN_POINT('Ctrl Pts',(41.9168262889714,37.1057501864126,49.8687432203114));
#25041=CARTESIAN_POINT('Ctrl Pts',(41.8549849134989,37.1019392963471,49.8516502108444));
#25042=CARTESIAN_POINT('Ctrl Pts',(41.794138668834,37.0981147778663,49.8315224826078));
#25043=CARTESIAN_POINT('Origin',(42.4,48.4493818343519,48.));
#25044=CARTESIAN_POINT('',(41.7941388330275,36.1345714126848,49.8315225369224));
#25045=CARTESIAN_POINT('',(41.7941388317569,36.3061495715672,49.8315225365021));
#25046=CARTESIAN_POINT('',(41.7941388317924,48.4493818343519,49.8315225365138));
#25047=CARTESIAN_POINT('',(40.4708706606089,36.7697993578986,47.9984035036532));
#25048=CARTESIAN_POINT('Ctrl Pts',(41.7941388330275,36.1345714126848,49.8315225369224));
#25049=CARTESIAN_POINT('Ctrl Pts',(41.8009572806551,36.1350086104464,49.833778055243));
#25050=CARTESIAN_POINT('Ctrl Pts',(41.8077888007653,36.1354448604187,49.8359956555078));
#25051=CARTESIAN_POINT('Ctrl Pts',(41.9455836056583,36.1442111378064,49.8798764128082));
#25052=CARTESIAN_POINT('Ctrl Pts',(42.0806146586887,36.1522315503165,49.9074654288939));
#25053=CARTESIAN_POINT('Ctrl Pts',(42.2841799109813,36.1646978117889,49.9268169322791));
#25054=CARTESIAN_POINT('Ctrl Pts',(42.3512044109253,36.1688560477862,49.929677515734));
#25055=CARTESIAN_POINT('Ctrl Pts',(42.4354047530644,36.1742170632708,49.9288814942915));
#25056=CARTESIAN_POINT('Ctrl Pts',(42.4525691265035,36.1753169335038,49.9284900237877));
#25057=CARTESIAN_POINT('Ctrl Pts',(42.4797707775054,36.1770721158391,49.9275062174923));
#25058=CARTESIAN_POINT('Ctrl Pts',(42.4898128466723,36.177722701858,49.9270644103481));
#25059=CARTESIAN_POINT('Ctrl Pts',(42.5078325914792,36.1788950326237,49.9261304650688));
#25060=CARTESIAN_POINT('Ctrl Pts',(42.5158115829642,36.1794158579891,49.9256671857462));
#25061=CARTESIAN_POINT('Ctrl Pts',(42.5344928357372,36.180639426134,49.9244659817669));
#25062=CARTESIAN_POINT('Ctrl Pts',(42.5451921896351,36.1813434025495,49.9236883474193));
#25063=CARTESIAN_POINT('Ctrl Pts',(42.5761700197746,36.1833911804766,49.9211769557397));
#25064=CARTESIAN_POINT('Ctrl Pts',(42.5964277291924,36.1847422042499,49.9192115214702));
#25065=CARTESIAN_POINT('Ctrl Pts',(42.6422030676289,36.1878230626574,49.9140380182859));
#25066=CARTESIAN_POINT('Ctrl Pts',(42.6676948359833,36.1895585761448,49.9106394818276));
#25067=CARTESIAN_POINT('Ctrl Pts',(42.7518620571181,36.1953557499667,49.8977009816661));
#25068=CARTESIAN_POINT('Ctrl Pts',(42.8101600314783,36.1994807566417,49.8859595800851));
#25069=CARTESIAN_POINT('Ctrl Pts',(43.0033079610357,36.2134873853851,49.837679631603));
#25070=CARTESIAN_POINT('Ctrl Pts',(43.1347104660036,36.2236161020049,49.7892023279416));
#25071=CARTESIAN_POINT('Ctrl Pts',(43.2983030526839,36.2363931871989,49.7077620660429));
#25072=CARTESIAN_POINT('Ctrl Pts',(43.3362301453234,36.2393647182202,49.6872680312452));
#25073=CARTESIAN_POINT('Ctrl Pts',(43.3821561796756,36.242946989608,49.6604257511065));
#25074=CARTESIAN_POINT('Ctrl Pts',(43.3908305787249,36.2436228661545,49.6552640911219));
#25075=CARTESIAN_POINT('Ctrl Pts',(43.4044023747732,36.2446786882718,49.6470433381782));
#25076=CARTESIAN_POINT('Ctrl Pts',(43.4093270843368,36.2450614643382,49.6440300262716));
#25077=CARTESIAN_POINT('Ctrl Pts',(43.4180620812676,36.2457396818177,49.6386312466677));
#25078=CARTESIAN_POINT('Ctrl Pts',(43.4218775540147,36.2460356752885,49.6362545734473));
#25079=CARTESIAN_POINT('Ctrl Pts',(43.4309909645052,36.2467420965395,49.6305334829408));
#25080=CARTESIAN_POINT('Ctrl Pts',(43.4362809518388,36.2471516939045,49.6271765729215));
#25081=CARTESIAN_POINT('Ctrl Pts',(43.4522763039183,36.2483891178528,49.6169166302427));
#25082=CARTESIAN_POINT('Ctrl Pts',(43.46292999451,36.2492118309391,49.6099331218116));
#25083=CARTESIAN_POINT('Ctrl Pts',(43.5595209897823,36.2566650191664,49.5452407572224));
#25084=CARTESIAN_POINT('Ctrl Pts',(43.6407648190996,36.2628959960399,49.4807993335028));
#25085=CARTESIAN_POINT('Ctrl Pts',(43.8292169004898,36.278302792853,49.3048676443737));
#25086=CARTESIAN_POINT('Ctrl Pts',(43.9289341128406,36.2874108156162,49.186463417218));
#25087=CARTESIAN_POINT('Ctrl Pts',(44.0266999911801,36.298671602816,49.0372901679564));
#25088=CARTESIAN_POINT('Ctrl Pts',(44.0395351919021,36.3002066290058,49.0168815199937));
#25089=CARTESIAN_POINT('Ctrl Pts',(44.0579069099156,36.3024926957422,48.9864171387052));
#25090=CARTESIAN_POINT('Ctrl Pts',(44.0637418732611,36.3032328152226,48.9765434262065));
#25091=CARTESIAN_POINT('Ctrl Pts',(44.0739552557175,36.3045539492513,48.9589034534954));
#25092=CARTESIAN_POINT('Ctrl Pts',(44.0783685685713,36.305133678329,48.9511577023916));
#25093=CARTESIAN_POINT('Ctrl Pts',(44.0875516082019,36.3063589719796,48.9347777398681));
#25094=CARTESIAN_POINT('Ctrl Pts',(44.092309103392,36.3070049548786,48.926137001601));
#25095=CARTESIAN_POINT('Ctrl Pts',(44.1047549801387,36.3087251919349,48.9031162195246));
#25096=CARTESIAN_POINT('Ctrl Pts',(44.1123275208251,36.3098035183433,48.8886747896752));
#25097=CARTESIAN_POINT('Ctrl Pts',(44.1486263152331,36.3151331092247,48.8172632866138));
#25098=CARTESIAN_POINT('Ctrl Pts',(44.1746942181496,36.3194756439799,48.7589941478702));
#25099=CARTESIAN_POINT('Ctrl Pts',(44.2465816683818,36.3332280347396,48.5742442184276));
#25100=CARTESIAN_POINT('Ctrl Pts',(44.2821006647031,36.3429146200307,48.4441963964617));
#25101=CARTESIAN_POINT('Ctrl Pts',(44.3158528097258,36.3577608374964,48.237933784063));
#25102=CARTESIAN_POINT('Ctrl Pts',(44.3236197499801,36.3629956320636,48.1636889931486));
#25103=CARTESIAN_POINT('Ctrl Pts',(44.3275489082023,36.3687343087476,48.0787784743352));
#25104=CARTESIAN_POINT('Ctrl Pts',(44.3279458195893,36.3694328518889,48.0683796020343));
#25105=CARTESIAN_POINT('Ctrl Pts',(44.3284510474268,36.3705541754809,48.0515764333418));
#25106=CARTESIAN_POINT('Ctrl Pts',(44.3286116446584,36.3709796816807,48.0451740834075));
#25107=CARTESIAN_POINT('Ctrl Pts',(44.3288405185264,36.3717331567373,48.0337882806378));
#25108=CARTESIAN_POINT('Ctrl Pts',(44.3289213705609,36.3720618079144,48.0288052417905));
#25109=CARTESIAN_POINT('Ctrl Pts',(44.3290553592587,36.3727749624879,48.0179554183574));
#25110=CARTESIAN_POINT('Ctrl Pts',(44.3291010451083,36.3731590492992,48.0120886787781));
#25111=CARTESIAN_POINT('Ctrl Pts',(44.3291548070831,36.3742462598663,47.9954191406808));
#25112=CARTESIAN_POINT('Ctrl Pts',(44.3290989099084,36.3749459306643,47.9846161504112));
#25113=CARTESIAN_POINT('Ctrl Pts',(44.3280910718764,36.3797239490435,47.9103755652056));
#25114=CARTESIAN_POINT('Ctrl Pts',(44.3241007971104,36.3836505217062,47.8470109472369));
#25115=CARTESIAN_POINT('Ctrl Pts',(44.3025826947547,36.3953281363148,47.656081049615));
#25116=CARTESIAN_POINT('Ctrl Pts',(44.2754136488311,36.4028511752207,47.5299712337034));
#25117=CARTESIAN_POINT('Ctrl Pts',(44.2116427354186,36.4154277965226,47.3323733059094));
#25118=CARTESIAN_POINT('Ctrl Pts',(44.182810293558,36.4202944950793,47.2588117373764));
#25119=CARTESIAN_POINT('Ctrl Pts',(44.1420959732181,36.4264408876067,47.1711709034922));
#25120=CARTESIAN_POINT('Ctrl Pts',(44.1344157607817,36.427574241417,47.155217195752));
#25121=CARTESIAN_POINT('Ctrl Pts',(44.1219348894102,36.4293771125267,47.1301791577639));
#25122=CARTESIAN_POINT('Ctrl Pts',(44.1172792651016,36.4300415600776,47.1210233337375));
#25123=CARTESIAN_POINT('Ctrl Pts',(44.1084727881656,36.4312838549264,47.1040414299086));
#25124=CARTESIAN_POINT('Ctrl Pts',(44.1043406993559,36.4318610269098,47.0962058844363));
#25125=CARTESIAN_POINT('Ctrl Pts',(44.095030401762,36.4331490697278,47.078841982025));
#25126=CARTESIAN_POINT('Ctrl Pts',(44.0898255502881,36.4338608770641,47.0693283294348));
#25127=CARTESIAN_POINT('Ctrl Pts',(44.0743444780676,36.4359545060972,47.0415893999121));
#25128=CARTESIAN_POINT('Ctrl Pts',(44.063851917181,36.4373440565229,47.0234873024757));
#25129=CARTESIAN_POINT('Ctrl Pts',(44.0393371339341,36.4405267074739,46.9827361368184));
#25130=CARTESIAN_POINT('Ctrl Pts',(44.0251362931791,36.4423260432584,46.9602000594332));
#25131=CARTESIAN_POINT('Ctrl Pts',(43.9759623109439,36.4484142832456,46.8856323631042));
#25132=CARTESIAN_POINT('Ctrl Pts',(43.9389233599734,36.4527737926352,46.8350167285073));
#25133=CARTESIAN_POINT('Ctrl Pts',(43.8520976515911,36.4625033669065,46.7277464059677));
#25134=CARTESIAN_POINT('Ctrl Pts',(43.8013186451659,36.4678927262991,46.6720233519219));
#25135=CARTESIAN_POINT('Ctrl Pts',(43.7228114364217,36.4757249590862,46.5954024267692));
#25136=CARTESIAN_POINT('Ctrl Pts',(43.6975704097303,36.4781751260998,46.5720519737054));
#25137=CARTESIAN_POINT('Ctrl Pts',(43.6222225686771,36.4852702805575,46.5059962378081));
#25138=CARTESIAN_POINT('Ctrl Pts',(43.5705325842715,36.4898697908531,46.4651610442292));
#25139=CARTESIAN_POINT('Ctrl Pts',(43.5084877348528,36.4950055596224,46.4211071304611));
#25140=CARTESIAN_POINT('Ctrl Pts',(43.5000774800546,36.4956939013415,46.4152358847721));
#25141=CARTESIAN_POINT('Ctrl Pts',(43.4863770367598,36.4968021065985,46.4058331529704));
#25142=CARTESIAN_POINT('Ctrl Pts',(43.4811156393179,36.4972245968493,46.4022603530433));
#25143=CARTESIAN_POINT('Ctrl Pts',(43.4717025469631,36.4979748293884,46.3959360946856));
#25144=CARTESIAN_POINT('Ctrl Pts',(43.4675577744175,36.4983032304236,46.3931746324963));
#25145=CARTESIAN_POINT('Ctrl Pts',(43.4584794484624,36.4990182858207,46.3871768152563));
#25146=CARTESIAN_POINT('Ctrl Pts',(43.4535417216059,36.4994045050021,46.3839470271071));
#25147=CARTESIAN_POINT('Ctrl Pts',(43.4393903201526,36.500503940726,46.3747829612085));
#25148=CARTESIAN_POINT('Ctrl Pts',(43.4301406117594,36.5012135808167,46.3689043576677));
#25149=CARTESIAN_POINT('Ctrl Pts',(43.3631742485993,36.5062907868552,46.3271411406001));
#25150=CARTESIAN_POINT('Ctrl Pts',(43.3036402425044,36.5104839565738,46.2942456597732));
#25151=CARTESIAN_POINT('Ctrl Pts',(43.1180360963973,36.5229890073882,46.2041422765265));
#25152=CARTESIAN_POINT('Ctrl Pts',(42.9874479961017,36.5310611392555,46.157288033414));
#25153=CARTESIAN_POINT('Ctrl Pts',(42.7888060176593,36.5435272366493,46.1093044985585));
#25154=CARTESIAN_POINT('Ctrl Pts',(42.7238964608718,36.5476232114347,46.0971102814945));
#25155=CARTESIAN_POINT('Ctrl Pts',(42.6415484750845,36.5529142552284,46.0859756261338));
#25156=CARTESIAN_POINT('Ctrl Pts',(42.6245733460683,36.5540098162237,46.0839097746938));
#25157=CARTESIAN_POINT('Ctrl Pts',(42.5975947827078,36.5557597017254,46.0809899431215));
#25158=CARTESIAN_POINT('Ctrl Pts',(42.5876080233734,36.5564093497652,46.0799878855096));
#25159=CARTESIAN_POINT('Ctrl Pts',(42.5696536332314,36.5575808770428,46.0783277824564));
#25160=CARTESIAN_POINT('Ctrl Pts',(42.5616888172968,36.5581018449284,46.0776412431434));
#25161=CARTESIAN_POINT('Ctrl Pts',(42.5430063339167,36.5593269089645,46.076147806392));
#25162=CARTESIAN_POINT('Ctrl Pts',(42.5322858227665,36.5600322486143,46.0753809396336));
#25163=CARTESIAN_POINT('Ctrl Pts',(42.5011492706283,36.5620879736502,46.0734150353505));
#25164=CARTESIAN_POINT('Ctrl Pts',(42.4807203970856,36.5634456678922,46.0724510477104));
#25165=CARTESIAN_POINT('Ctrl Pts',(42.4344188785877,36.5665441049198,46.0710035288296));
#25166=CARTESIAN_POINT('Ctrl Pts',(42.4085445063989,36.5682906205869,46.0707154362865));
#25167=CARTESIAN_POINT('Ctrl Pts',(42.3226799045727,36.5741375221424,46.0714866753528));
#25168=CARTESIAN_POINT('Ctrl Pts',(42.2627497625028,36.5783024655663,46.0748238390646));
#25169=CARTESIAN_POINT('Ctrl Pts',(42.1257891429925,36.5879922453757,46.0888780023973));
#25170=CARTESIAN_POINT('Ctrl Pts',(42.0490540534555,36.5935485658404,46.1014703664577));
#25171=CARTESIAN_POINT('Ctrl Pts',(41.8817581829358,36.6057983577597,46.1394147961711));
#25172=CARTESIAN_POINT('Ctrl Pts',(41.791852492104,36.6124734034057,46.1668300494897));
#25173=CARTESIAN_POINT('Ctrl Pts',(41.6889784090794,36.6199820789853,46.2066064457459));
#25174=CARTESIAN_POINT('Ctrl Pts',(41.6737397850468,36.6210906892824,46.2127232202605));
#25175=CARTESIAN_POINT('Ctrl Pts',(41.6526280758012,36.6226196577722,46.2215120647586));
#25176=CARTESIAN_POINT('Ctrl Pts',(41.646687998176,36.623049085284,46.2240199438821));
#25177=CARTESIAN_POINT('Ctrl Pts',(41.6364633661507,36.6237867883855,46.2283972749394));
#25178=CARTESIAN_POINT('Ctrl Pts',(41.6321728735536,36.6240958972375,46.2302525853289));
#25179=CARTESIAN_POINT('Ctrl Pts',(41.6231388719413,36.6247457400443,46.2341981386607));
#25180=CARTESIAN_POINT('Ctrl Pts',(41.6183969685774,36.6250862433636,46.2362919379391));
#25181=CARTESIAN_POINT('Ctrl Pts',(41.6069257491492,36.6259086484721,46.2414124325074));
#25182=CARTESIAN_POINT('Ctrl Pts',(41.6002051635955,36.6263893682201,46.24445870914));
#25183=CARTESIAN_POINT('Ctrl Pts',(41.5754567372873,36.6281561432442,46.2558481812904));
#25184=CARTESIAN_POINT('Ctrl Pts',(41.5575398783452,36.6294283966347,46.2644314543195));
#25185=CARTESIAN_POINT('Ctrl Pts',(41.5124210643545,36.6326228291553,46.2869095242789));
#25186=CARTESIAN_POINT('Ctrl Pts',(41.4854098995034,36.6345264331339,46.3011767309174));
#25187=CARTESIAN_POINT('Ctrl Pts',(41.3588961211328,36.6434539001505,46.3718935219641));
#25188=CARTESIAN_POINT('Ctrl Pts',(41.2642004126601,36.6501819496267,46.4364812258942));
#25189=CARTESIAN_POINT('Ctrl Pts',(41.0901678247078,36.6636621416798,46.5793826026087));
#25190=CARTESIAN_POINT('Ctrl Pts',(41.0107800366663,36.6703842196541,46.656915037007));
#25191=CARTESIAN_POINT('Ctrl Pts',(40.9273521396177,36.6785029912698,46.7537488581037));
#25192=CARTESIAN_POINT('Ctrl Pts',(40.9163884808457,36.6795933394521,46.7668209944236));
#25193=CARTESIAN_POINT('Ctrl Pts',(40.8986347094142,36.6813991794055,46.7885685610281));
#25194=CARTESIAN_POINT('Ctrl Pts',(40.8917428217386,36.6821105404719,46.7971599678215));
#25195=CARTESIAN_POINT('Ctrl Pts',(40.8794346298839,36.6834000980226,46.8127754312641));
#25196=CARTESIAN_POINT('Ctrl Pts',(40.8739924438112,36.6839772385048,46.8197787684332));
#25197=CARTESIAN_POINT('Ctrl Pts',(40.8624300144788,36.6852185993072,46.8348716844132));
#25198=CARTESIAN_POINT('Ctrl Pts',(40.8563249186648,36.6858833939101,46.8429724771036));
#25199=CARTESIAN_POINT('Ctrl Pts',(40.8398069183229,36.6877081079555,46.8652535057699));
#25200=CARTESIAN_POINT('Ctrl Pts',(40.8295238662872,36.6888730178222,46.8795283418628));
#25201=CARTESIAN_POINT('Ctrl Pts',(40.7709365156526,36.6956833330119,46.9632499057979));
#25202=CARTESIAN_POINT('Ctrl Pts',(40.7270533897486,36.7014937554484,47.0356636124512));
#25203=CARTESIAN_POINT('Ctrl Pts',(40.661535844037,36.7114692725471,47.1617890949728));
#25204=CARTESIAN_POINT('Ctrl Pts',(40.6373044749432,36.715560480507,47.2140235135481));
#25205=CARTESIAN_POINT('Ctrl Pts',(40.5907323562836,36.7243121413339,47.3274478437722));
#25206=CARTESIAN_POINT('Ctrl Pts',(40.5690796922284,36.7289721003683,47.3888478644616));
#25207=CARTESIAN_POINT('Ctrl Pts',(40.5324931790245,36.7380700826651,47.5121483578574));
#25208=CARTESIAN_POINT('Ctrl Pts',(40.5174350806266,36.7425051278411,47.5739342508564));
#25209=CARTESIAN_POINT('Ctrl Pts',(40.5035350550902,36.7474811980011,47.6463520758601));
#25210=CARTESIAN_POINT('Ctrl Pts',(40.5016956336781,36.7481641647341,47.6563625670655));
#25211=CARTESIAN_POINT('Ctrl Pts',(40.4988397481347,36.7492654512868,47.6726280407071));
#25212=CARTESIAN_POINT('Ctrl Pts',(40.4977747530299,36.7496863462597,47.6788741436277));
#25213=CARTESIAN_POINT('Ctrl Pts',(40.4959278740491,36.7504348752451,47.6900376065054));
#25214=CARTESIAN_POINT('Ctrl Pts',(40.4951342347208,36.7507631555098,47.6949528490451));
#25215=CARTESIAN_POINT('Ctrl Pts',(40.4936236219974,36.7514012208612,47.7045443494784));
#25216=CARTESIAN_POINT('Ctrl Pts',(40.4929048209998,36.7517111136964,47.7092201598197));
#25217=CARTESIAN_POINT('Ctrl Pts',(40.4913332108834,36.7524031734755,47.7197000562021));
#25218=CARTESIAN_POINT('Ctrl Pts',(40.4904896572616,36.7527848304333,47.7255055127927));
#25219=CARTESIAN_POINT('Ctrl Pts',(40.4884319193051,36.7537425276665,47.7401358440947));
#25220=CARTESIAN_POINT('Ctrl Pts',(40.4872523373952,36.7543167518144,47.7489655543143));
#25221=CARTESIAN_POINT('Ctrl Pts',(40.4760359757809,36.7600459676455,47.837598533665));
#25222=CARTESIAN_POINT('Ctrl Pts',(40.4709372370669,36.7649585678963,47.9179557164651));
#25223=CARTESIAN_POINT('Ctrl Pts',(40.4708706606089,36.7697993578986,47.9984035036532));
#25224=CARTESIAN_POINT('Ctrl Pts',(40.4708706624223,36.7697992261421,47.9984013140282));
#25225=CARTESIAN_POINT('Ctrl Pts',(40.4707569252598,36.7780577578374,48.1356475905335));
#25226=CARTESIAN_POINT('Ctrl Pts',(40.4852891210741,36.7860953737044,48.2725153539239));
#25227=CARTESIAN_POINT('Ctrl Pts',(40.5257982606741,36.7979099669867,48.460352132471));
#25228=CARTESIAN_POINT('Ctrl Pts',(40.5396557529755,36.8013392905584,48.513492618657));
#25229=CARTESIAN_POINT('Ctrl Pts',(40.5603242358317,36.8058347654552,48.5808422919918));
#25230=CARTESIAN_POINT('Ctrl Pts',(40.565069059847,36.8068333305538,48.5956619068988));
#25231=CARTESIAN_POINT('Ctrl Pts',(40.5730622252872,36.808464023713,48.6196249172202));
#25232=CARTESIAN_POINT('Ctrl Pts',(40.5762012489584,36.8090925340274,48.6288042467116));
#25233=CARTESIAN_POINT('Ctrl Pts',(40.5823723405563,36.8103059670176,48.6464151358981));
#25234=CARTESIAN_POINT('Ctrl Pts',(40.5853941839218,36.8108905363832,48.654850031664));
#25235=CARTESIAN_POINT('Ctrl Pts',(40.5924648089623,36.8122368309938,48.6741615383886));
#25236=CARTESIAN_POINT('Ctrl Pts',(40.5965531697579,36.8129998637378,48.6850231872972));
#25237=CARTESIAN_POINT('Ctrl Pts',(40.6099470246769,36.815451861123,48.7196558507389));
#25238=CARTESIAN_POINT('Ctrl Pts',(40.6196261066162,36.8171532906534,48.7432784747977));
#25239=CARTESIAN_POINT('Ctrl Pts',(40.6761888861681,36.8267266070038,48.8738757613358));
#25240=CARTESIAN_POINT('Ctrl Pts',(40.7322362040158,36.8349105836414,48.976595710591));
#25241=CARTESIAN_POINT('Ctrl Pts',(40.8516279067285,36.8501935261282,49.1548358867709));
#25242=CARTESIAN_POINT('Ctrl Pts',(40.9121384244596,36.857224964475,49.2318161402958));
#25243=CARTESIAN_POINT('Ctrl Pts',(40.9988947501641,36.8662112869134,49.3264169120343));
#25244=CARTESIAN_POINT('Ctrl Pts',(41.0200982243359,36.8683320553846,49.3484617329203));
#25245=CARTESIAN_POINT('Ctrl Pts',(41.055872782144,36.8717760531038,49.3839278378523));
#25246=CARTESIAN_POINT('Ctrl Pts',(41.0701418204504,36.8731164110648,49.3976449962793));
#25247=CARTESIAN_POINT('Ctrl Pts',(41.089975502176,36.8749314146436,49.4161327523362));
#25248=CARTESIAN_POINT('Ctrl Pts',(41.0953593875194,36.8754193679366,49.4210943085137));
#25249=CARTESIAN_POINT('Ctrl Pts',(41.1046229880529,36.8762506886312,49.4295342252387));
#25250=CARTESIAN_POINT('Ctrl Pts',(41.1084887483931,36.8765951729143,49.4330277014369));
#25251=CARTESIAN_POINT('Ctrl Pts',(41.1158325428134,36.8772449247393,49.4396104116713));
#25252=CARTESIAN_POINT('Ctrl Pts',(41.1193076673501,36.8775504354563,49.4427027918916));
#25253=CARTESIAN_POINT('Ctrl Pts',(41.1275586557853,36.8782712926793,49.4499917244929));
#25254=CARTESIAN_POINT('Ctrl Pts',(41.132344182394,36.8786858324727,49.4541773297817));
#25255=CARTESIAN_POINT('Ctrl Pts',(41.1491568500165,36.8801301942742,49.4687362675003));
#25256=CARTESIAN_POINT('Ctrl Pts',(41.1612917120652,36.8811513517883,49.4789849985772));
#25257=CARTESIAN_POINT('Ctrl Pts',(41.267190321235,36.8898943984561,49.5662058622677));
#25258=CARTESIAN_POINT('Ctrl Pts',(41.367908044144,36.8970950927505,49.6343356640115));
#25259=CARTESIAN_POINT('Ctrl Pts',(41.5573348998316,36.9099720537676,49.7379296876064));
#25260=CARTESIAN_POINT('Ctrl Pts',(41.6435181852034,36.9156155288907,49.7771374697818));
#25261=CARTESIAN_POINT('Ctrl Pts',(41.7527389599502,36.9227892690317,49.8174360782789));
#25262=CARTESIAN_POINT('Ctrl Pts',(41.7733804888912,36.924145523862,49.8246557502234));
#25263=CARTESIAN_POINT('Ctrl Pts',(41.7941388333426,36.925511940895,49.8315225370267));
#25264=CARTESIAN_POINT('',(40.4708700028765,36.9418246930855,47.9998946523509));
#25265=CARTESIAN_POINT('Ctrl Pts',(41.794138668834,37.0981147778663,49.8315224826078));
#25266=CARTESIAN_POINT('Ctrl Pts',(41.7454310361826,37.0950532373841,49.815410165431));
#25267=CARTESIAN_POINT('Ctrl Pts',(41.6973610717923,37.091983196828,49.7973531909593));
#25268=CARTESIAN_POINT('Ctrl Pts',(41.5766700783443,37.0840521298605,49.7464285821558));
#25269=CARTESIAN_POINT('Ctrl Pts',(41.5052907762867,37.0791449949644,49.710958237956));
#25270=CARTESIAN_POINT('Ctrl Pts',(41.4209724660933,37.0729555239317,49.6623360721082));
#25271=CARTESIAN_POINT('Ctrl Pts',(41.4057552262409,37.0718222576782,49.6532795967791));
#25272=CARTESIAN_POINT('Ctrl Pts',(41.3820247275679,37.0700281489059,49.63871037718));
#25273=CARTESIAN_POINT('Ctrl Pts',(41.3734263389798,37.0693724405478,49.6333376465228));
#25274=CARTESIAN_POINT('Ctrl Pts',(41.3580770133011,37.0681915414317,49.6235774896652));
#25275=CARTESIAN_POINT('Ctrl Pts',(41.3513103884722,37.0676672896392,49.6192150785249));
#25276=CARTESIAN_POINT('Ctrl Pts',(41.3375614442115,37.0665944740949,49.6102288664108));
#25277=CARTESIAN_POINT('Ctrl Pts',(41.3305815375667,37.0660457917976,49.6056017051235));
#25278=CARTESIAN_POINT('Ctrl Pts',(41.3102370988762,37.0644344994713,49.5919233364144));
#25279=CARTESIAN_POINT('Ctrl Pts',(41.2969560432276,37.0633672790527,49.5827498513841));
#25280=CARTESIAN_POINT('Ctrl Pts',(41.2334528888738,37.0581884089966,49.5376994940218));
#25281=CARTESIAN_POINT('Ctrl Pts',(41.1848619101246,37.0539916450362,49.4995965720038));
#25282=CARTESIAN_POINT('Ctrl Pts',(41.038747219693,37.0406094233033,49.3732496309346));
#25283=CARTESIAN_POINT('Ctrl Pts',(40.9483668961227,37.0311543843263,49.2773324207762));
#25284=CARTESIAN_POINT('Ctrl Pts',(40.8199206676892,37.0161258388123,49.1096225847369));
#25285=CARTESIAN_POINT('Ctrl Pts',(40.7753633117638,37.0105087196857,49.0432984151213));
#25286=CARTESIAN_POINT('Ctrl Pts',(40.7297413294677,37.004409723654,48.9653437547797));
#25287=CARTESIAN_POINT('Ctrl Pts',(40.7245167852918,37.0037054663072,48.9562471441007));
#25288=CARTESIAN_POINT('Ctrl Pts',(40.7162106812862,37.0025768666194,48.9415080496272));
#25289=CARTESIAN_POINT('Ctrl Pts',(40.7130827545468,37.0021497418739,48.9358921344244));
#25290=CARTESIAN_POINT('Ctrl Pts',(40.7075794086608,37.0013946023317,48.9258941309088));
#25291=CARTESIAN_POINT('Ctrl Pts',(40.7051928389852,37.0010658919909,48.9215183604213));
#25292=CARTESIAN_POINT('Ctrl Pts',(40.7000437638187,37.0003540028192,48.9119898744771));
#25293=CARTESIAN_POINT('Ctrl Pts',(40.6972877088918,36.9999712298017,48.9068338282324));
#25294=CARTESIAN_POINT('Ctrl Pts',(40.6895485471102,36.9988912027357,48.8921956750119));
#25295=CARTESIAN_POINT('Ctrl Pts',(40.6846208209799,36.9981973312007,48.882684303784));
#25296=CARTESIAN_POINT('Ctrl Pts',(40.6521097475877,36.9935739404767,48.8186316325582));
#25297=CARTESIAN_POINT('Ctrl Pts',(40.627049591588,36.9897851675397,48.7628411188254));
#25298=CARTESIAN_POINT('Ctrl Pts',(40.5727654199779,36.9807557946529,48.6247893259087));
#25299=CARTESIAN_POINT('Ctrl Pts',(40.5463909450823,36.975593039245,48.5415557795884));
#25300=CARTESIAN_POINT('Ctrl Pts',(40.4971987142562,36.9631828912664,48.3397278068748));
#25301=CARTESIAN_POINT('Ctrl Pts',(40.4796982803696,36.9559069732899,48.2202350126324));
#25302=CARTESIAN_POINT('Ctrl Pts',(40.4724802446671,36.947056890077,48.0810365037881));
#25303=CARTESIAN_POINT('Ctrl Pts',(40.4717792364017,36.9458494637154,48.0621608277055));
#25304=CARTESIAN_POINT('Ctrl Pts',(40.4711555394033,36.9440594710842,48.0343666126744));
#25305=CARTESIAN_POINT('Ctrl Pts',(40.4710173343154,36.9434836384135,48.0254536503816));
#25306=CARTESIAN_POINT('Ctrl Pts',(40.4708933347106,36.9425462252616,48.010991735587));
#25307=CARTESIAN_POINT('Ctrl Pts',(40.4708696998777,36.9421858346456,48.0054431776609));
#25308=CARTESIAN_POINT('Ctrl Pts',(40.4708700028765,36.9418246930855,47.9998946523509));
#25309=CARTESIAN_POINT('Ctrl Pts',(40.4708700028783,36.9418246909392,47.9998946193751));
#25310=CARTESIAN_POINT('Ctrl Pts',(40.4708703171738,36.9414502021496,47.994141029262));
#25311=CARTESIAN_POINT('Ctrl Pts',(40.4708963714056,36.9410749081892,47.9883875098055));
#25312=CARTESIAN_POINT('Ctrl Pts',(40.4710383629421,36.9400437949537,47.9726145800584));
#25313=CARTESIAN_POINT('Ctrl Pts',(40.4712066235956,36.9393863442948,47.9625959473324));
#25314=CARTESIAN_POINT('Ctrl Pts',(40.4719114878001,36.9374977927137,47.933929941959));
#25315=CARTESIAN_POINT('Ctrl Pts',(40.472640525301,36.9362607098083,47.915288861529));
#25316=CARTESIAN_POINT('Ctrl Pts',(40.4796010678418,36.9275846167825,47.7855351380816));
#25317=CARTESIAN_POINT('Ctrl Pts',(40.4951657822964,36.9198518695679,47.6751521228974));
#25318=CARTESIAN_POINT('Ctrl Pts',(40.5522539584392,36.9018142395651,47.4274540122385));
#25319=CARTESIAN_POINT('Ctrl Pts',(40.5997378559718,36.8914466171965,47.2921628362161));
#25320=CARTESIAN_POINT('Ctrl Pts',(40.6708608603666,36.8802200109951,47.1443930266558));
#25321=CARTESIAN_POINT('Ctrl Pts',(40.6802981116673,36.8787934437358,47.125579642263));
#25322=CARTESIAN_POINT('Ctrl Pts',(40.6935825187309,36.8768722364856,47.1001442158016));
#25323=CARTESIAN_POINT('Ctrl Pts',(40.6971635819629,36.8763624925994,47.0933858643113));
#25324=CARTESIAN_POINT('Ctrl Pts',(40.7032364820796,36.8755117967366,47.0820877298892));
#25325=CARTESIAN_POINT('Ctrl Pts',(40.7057065471878,36.8751695042738,47.0775364130618));
#25326=CARTESIAN_POINT('Ctrl Pts',(40.7104420437151,36.8745203745675,47.0688940249943));
#25327=CARTESIAN_POINT('Ctrl Pts',(40.7127040626889,36.8742133178133,47.0648011733126));
#25328=CARTESIAN_POINT('Ctrl Pts',(40.7181256018287,36.873484407005,47.0550752525117));
#25329=CARTESIAN_POINT('Ctrl Pts',(40.7212985967575,36.8730634042505,47.0494497007954));
#25330=CARTESIAN_POINT('Ctrl Pts',(40.7326726248818,36.8715735878042,47.0295187396789));
#25331=CARTESIAN_POINT('Ctrl Pts',(40.7410290216617,36.8705141699155,47.0153021838153));
#25332=CARTESIAN_POINT('Ctrl Pts',(40.8007555556011,36.8631698525741,46.9166097071062));
#25333=CARTESIAN_POINT('Ctrl Pts',(40.8583776778178,36.8572254473591,46.8360743456382));
#25334=CARTESIAN_POINT('Ctrl Pts',(40.9929134129562,36.8447176937851,46.67566926447));
#25335=CARTESIAN_POINT('Ctrl Pts',(41.0710326544027,36.8381800291895,46.5972923459725));
#25336=CARTESIAN_POINT('Ctrl Pts',(41.1986442560613,36.8279227753285,46.4895410397143));
#25337=CARTESIAN_POINT('Ctrl Pts',(41.2434417872356,36.8243925523091,46.4549711773303));
#25338=CARTESIAN_POINT('Ctrl Pts',(41.3025355347381,36.8197824086446,46.4133806246838));
#25339=CARTESIAN_POINT('Ctrl Pts',(41.3154905477751,36.8187745507199,46.4044974086333));
#25340=CARTESIAN_POINT('Ctrl Pts',(41.3354943708255,36.8172218648858,46.3911370436227));
#25341=CARTESIAN_POINT('Ctrl Pts',(41.3424663801117,36.8166813516314,46.3865456665564));
#25342=CARTESIAN_POINT('Ctrl Pts',(41.3563078658337,36.8156094332521,46.3775586931019));
#25343=CARTESIAN_POINT('Ctrl Pts',(41.3631758536137,36.8150781168087,46.3731611169891));
#25344=CARTESIAN_POINT('Ctrl Pts',(41.378808142928,36.8138699264588,46.3632909519611));
#25345=CARTESIAN_POINT('Ctrl Pts',(41.3875888843045,36.8131920855955,46.3578450004252));
#25346=CARTESIAN_POINT('Ctrl Pts',(41.4122654394281,36.8112891451264,46.3428133629127));
#25347=CARTESIAN_POINT('Ctrl Pts',(41.4282561261429,36.8100583033561,46.3333863930788));
#25348=CARTESIAN_POINT('Ctrl Pts',(41.5498200343681,36.8007155297687,46.2640652601025));
#25349=CARTESIAN_POINT('Ctrl Pts',(41.6606798664753,36.7922496489529,46.2140349069197));
#25350=CARTESIAN_POINT('Ctrl Pts',(41.8587370595397,36.7773564422047,46.1462687793514));
#25351=CARTESIAN_POINT('Ctrl Pts',(41.9438412272781,36.7710326115839,46.1235127492855));
#25352=CARTESIAN_POINT('Ctrl Pts',(42.0892086906285,36.7605756588918,46.0951204906196));
#25353=CARTESIAN_POINT('Ctrl Pts',(42.1487286345174,36.7563902633524,46.0863591179395));
#25354=CARTESIAN_POINT('Ctrl Pts',(42.2191853672955,36.7516177176654,46.0793327957863));
#25355=CARTESIAN_POINT('Ctrl Pts',(42.2298132372096,36.7509026816564,46.0783619177059));
#25356=CARTESIAN_POINT('Ctrl Pts',(42.2462666527663,36.7498037900726,46.0769964394007));
#25357=CARTESIAN_POINT('Ctrl Pts',(42.2520866519703,36.7494166460545,46.0765400238514));
#25358=CARTESIAN_POINT('Ctrl Pts',(42.262880528788,36.7487016487293,46.0757428287392));
#25359=CARTESIAN_POINT('Ctrl Pts',(42.2678536390572,36.7483734200831,46.0753949104563));
#25360=CARTESIAN_POINT('Ctrl Pts',(42.2792543960875,36.7476236498434,46.0746417133527));
#25361=CARTESIAN_POINT('Ctrl Pts',(42.285682767818,36.7472028317202,46.0742493395556));
#25362=CARTESIAN_POINT('Ctrl Pts',(42.3026271525625,36.7460984425102,46.0733002367636));
#25363=CARTESIAN_POINT('Ctrl Pts',(42.3131461361322,36.7454177472603,46.0727973984728));
#25364=CARTESIAN_POINT('Ctrl Pts',(42.4067927897772,36.7393971853489,46.0690891228776));
#25365=CARTESIAN_POINT('Ctrl Pts',(42.4900538123251,36.7343189004283,46.0711773376252));
#25366=CARTESIAN_POINT('Ctrl Pts',(42.5945455641111,36.7280091183409,46.0805819565372));
#25367=CARTESIAN_POINT('Ctrl Pts',(42.6161276451181,36.72670944365,46.0828921614466));
#25368=CARTESIAN_POINT('Ctrl Pts',(42.7188888398743,36.7205209147854,46.0956493950066));
#25369=CARTESIAN_POINT('Ctrl Pts',(42.799386582122,36.7156685448763,46.1108913979855));
#25370=CARTESIAN_POINT('Ctrl Pts',(42.9595498656809,36.7056711001515,46.1519152932779));
#25371=CARTESIAN_POINT('Ctrl Pts',(43.0389894577895,36.7005320899267,46.1778575697527));
#25372=CARTESIAN_POINT('Ctrl Pts',(43.1327732108063,36.6941043262898,46.215373027404));
#25373=CARTESIAN_POINT('Ctrl Pts',(43.1489633193507,36.6929814361813,46.222106886383));
#25374=CARTESIAN_POINT('Ctrl Pts',(43.1743576194729,36.6911980825739,46.2330774108851));
#25375=CARTESIAN_POINT('Ctrl Pts',(43.1836243354947,36.6905426148878,46.2371676049385));
#25376=CARTESIAN_POINT('Ctrl Pts',(43.2009425939524,36.6893085848252,46.2449751688662));
#25377=CARTESIAN_POINT('Ctrl Pts',(43.2090015791004,36.6887306228197,46.2486754620328));
#25378=CARTESIAN_POINT('Ctrl Pts',(43.2270238403651,36.6874296347854,46.2571013457235));
#25379=CARTESIAN_POINT('Ctrl Pts',(43.2369726199378,36.6867055793159,46.261857032208));
#25380=CARTESIAN_POINT('Ctrl Pts',(43.262252197299,36.6848504602083,46.2742084643575));
#25381=CARTESIAN_POINT('Ctrl Pts',(43.2775234489809,36.6837152773168,46.2819232146027));
#25382=CARTESIAN_POINT('Ctrl Pts',(43.396286603507,36.674770443648,46.3439166134479));
#25383=CARTESIAN_POINT('Ctrl Pts',(43.4947369566645,36.6666332820997,46.4072849135489));
#25384=CARTESIAN_POINT('Ctrl Pts',(43.6722368003156,36.6506318504383,46.5458022813326));
#25385=CARTESIAN_POINT('Ctrl Pts',(43.7518728604917,36.6428232846468,46.6195225679128));
#25386=CARTESIAN_POINT('Ctrl Pts',(43.8454498597295,36.6331059731979,46.7220538090091));
#25387=CARTESIAN_POINT('Ctrl Pts',(43.8654635755177,36.6309921989567,46.7450543911489));
#25388=CARTESIAN_POINT('Ctrl Pts',(43.897650542614,36.6275452610939,46.7838656263321));
#25389=CARTESIAN_POINT('Ctrl Pts',(43.9101382799499,36.626195331275,46.7994074733848));
#25390=CARTESIAN_POINT('Ctrl Pts',(43.9269836714137,36.6243598470176,46.821051518329));
#25391=CARTESIAN_POINT('Ctrl Pts',(43.9315495404351,36.6238608320935,46.8269890601568));
#25392=CARTESIAN_POINT('Ctrl Pts',(43.939194213498,36.6230229642824,46.8370510689767));
#25393=CARTESIAN_POINT('Ctrl Pts',(43.9422912736149,36.622682856252,46.8411614984653));
#25394=CARTESIAN_POINT('Ctrl Pts',(43.9481899563555,36.6220338777575,46.8490557872351));
#25395=CARTESIAN_POINT('Ctrl Pts',(43.9509942176807,36.6217248144004,46.8528375617343));
#25396=CARTESIAN_POINT('Ctrl Pts',(43.9576849073498,36.6209860270682,46.8619298829991));
#25397=CARTESIAN_POINT('Ctrl Pts',(43.9615580943989,36.6205572084981,46.8672501676447));
#25398=CARTESIAN_POINT('Ctrl Pts',(43.9733571173195,36.619247005931,46.8836330652246));
#25399=CARTESIAN_POINT('Ctrl Pts',(43.9811933807205,36.6183713976806,46.8947600851909));
#25400=CARTESIAN_POINT('Ctrl Pts',(44.0668265734546,36.6087302944878,47.0191291596374));
#25401=CARTESIAN_POINT('Ctrl Pts',(44.1324423102089,36.6006465526967,47.1403061533718));
#25402=CARTESIAN_POINT('Ctrl Pts',(44.2256530564769,36.5859913907075,47.3673829199694));
#25403=CARTESIAN_POINT('Ctrl Pts',(44.2582048357959,36.5794939006893,47.4705808835711));
#25404=CARTESIAN_POINT('Ctrl Pts',(44.2885606998226,36.5708282070692,47.6053025247742));
#25405=CARTESIAN_POINT('Ctrl Pts',(44.2944858313437,36.568920987599,47.6348002030437));
#25406=CARTESIAN_POINT('Ctrl Pts',(44.3018952892932,36.5661894706214,47.6767455411945));
#25407=CARTESIAN_POINT('Ctrl Pts',(44.3039519999358,36.5653833249849,47.6890885875231));
#25408=CARTESIAN_POINT('Ctrl Pts',(44.3072925900086,36.5639860587674,47.7104143400978));
#25409=CARTESIAN_POINT('Ctrl Pts',(44.3086334566281,36.5633967640545,47.7193878088022));
#25410=CARTESIAN_POINT('Ctrl Pts',(44.3110829109165,36.5622629949858,47.73661066461));
#25411=CARTESIAN_POINT('Ctrl Pts',(44.3122015101052,36.561718852178,47.744858440342));
#25412=CARTESIAN_POINT('Ctrl Pts',(44.3147090216696,36.5604338947866,47.7642905694446));
#25413=CARTESIAN_POINT('Ctrl Pts',(44.3160533535948,36.5596916883663,47.7754802674773));
#25414=CARTESIAN_POINT('Ctrl Pts',(44.3204036438068,36.5570898788824,47.8145804208853));
#25415=CARTESIAN_POINT('Ctrl Pts',(44.3228982653626,36.5552143506592,47.8425430372192));
#25416=CARTESIAN_POINT('Ctrl Pts',(44.3367613252612,36.5412730738972,48.0486700571453));
#25417=CARTESIAN_POINT('Ctrl Pts',(44.3239545659027,36.5284201795127,48.2275668539296));
#25418=CARTESIAN_POINT('Ctrl Pts',(44.2724220942797,36.510858713565,48.4693708413194));
#25419=CARTESIAN_POINT('Ctrl Pts',(44.254496451837,36.5060264124634,48.5358342369383));
#25420=CARTESIAN_POINT('Ctrl Pts',(44.2283007855537,36.5003168344293,48.6157042070648));
#25421=CARTESIAN_POINT('Ctrl Pts',(44.2233729200037,36.4992883665514,48.6301481282379));
#25422=CARTESIAN_POINT('Ctrl Pts',(44.2160230574539,36.4978193823372,48.6508826325433));
#25423=CARTESIAN_POINT('Ctrl Pts',(44.213738836856,36.4973713342049,48.6572209534226));
#25424=CARTESIAN_POINT('Ctrl Pts',(44.2096953084201,36.4965929570195,48.6682594039745));
#25425=CARTESIAN_POINT('Ctrl Pts',(44.2079507998602,36.4962617701558,48.6729648192413));
#25426=CARTESIAN_POINT('Ctrl Pts',(44.2042011645192,36.4955597100276,48.6829587847218));
#25427=CARTESIAN_POINT('Ctrl Pts',(44.2021911305572,36.4951891316179,48.6882453593436));
#25428=CARTESIAN_POINT('Ctrl Pts',(44.1966231514421,36.4941780102849,48.7026980015945));
#25429=CARTESIAN_POINT('Ctrl Pts',(44.193018276199,36.4935401974951,48.7118459811861));
#25430=CARTESIAN_POINT('Ctrl Pts',(44.1750204674084,36.4904347231155,48.7565141793475));
#25431=CARTESIAN_POINT('Ctrl Pts',(44.1596401187362,36.4880208939262,48.7916302674852));
#25432=CARTESIAN_POINT('Ctrl Pts',(44.1279568928906,36.4834364418977,48.8584741371831));
#25433=CARTESIAN_POINT('Ctrl Pts',(44.1118009444526,36.4812615443856,48.8902531256488));
#25434=CARTESIAN_POINT('Ctrl Pts',(44.0399735493278,36.4721678416991,49.0223445057281));
#25435=CARTESIAN_POINT('Ctrl Pts',(43.9762943400279,36.4654331111313,49.118033451548));
#25436=CARTESIAN_POINT('Ctrl Pts',(43.8514954980191,36.45338344161,49.2735271518019));
#25437=CARTESIAN_POINT('Ctrl Pts',(43.7942187906395,36.448175242888,49.3359872341358));
#25438=CARTESIAN_POINT('Ctrl Pts',(43.7203131965847,36.441669558159,49.4066361040174));
#25439=CARTESIAN_POINT('Ctrl Pts',(43.7074307665747,36.4405429847606,49.4186179273792));
#25440=CARTESIAN_POINT('Ctrl Pts',(43.6868665142056,36.4387551053353,49.4372264922803));
#25441=CARTESIAN_POINT('Ctrl Pts',(43.6792930037712,36.4380988387308,49.4439718901251));
#25442=CARTESIAN_POINT('Ctrl Pts',(43.6649993634062,36.4368641080045,49.4565018993982));
#25443=CARTESIAN_POINT('Ctrl Pts',(43.658291831643,36.4362862511102,49.4623005280588));
#25444=CARTESIAN_POINT('Ctrl Pts',(43.6431668386492,36.4349865607776,49.4751948915058));
#25445=CARTESIAN_POINT('Ctrl Pts',(43.6347281860772,36.4342637069014,49.4822651768796));
#25446=CARTESIAN_POINT('Ctrl Pts',(43.6130673077097,36.4324137424148,49.5001003179589));
#25447=CARTESIAN_POINT('Ctrl Pts',(43.5997622665717,36.4312825516223,49.5107626315234));
#25448=CARTESIAN_POINT('Ctrl Pts',(43.4995172303082,36.4227955398117,49.5889369836959));
#25449=CARTESIAN_POINT('Ctrl Pts',(43.4070974827407,36.4151513156321,49.6490621791765));
#25450=CARTESIAN_POINT('Ctrl Pts',(43.1829061684697,36.3971160210018,49.7690111933048));
#25451=CARTESIAN_POINT('Ctrl Pts',(43.0485107674243,36.3866510859355,49.8225748784175));
#25452=CARTESIAN_POINT('Ctrl Pts',(42.8890322850437,36.3753309627018,49.8662357383775));
#25453=CARTESIAN_POINT('Ctrl Pts',(42.8685753319509,36.3738995615024,49.8714768649011));
#25454=CARTESIAN_POINT('Ctrl Pts',(42.8405868291907,36.3719729664018,49.8781598568549));
#25455=CARTESIAN_POINT('Ctrl Pts',(42.8331275368688,36.3714625620198,49.8798940777791));
#25456=CARTESIAN_POINT('Ctrl Pts',(42.820605372883,36.3706110741624,49.8827268820315));
#25457=CARTESIAN_POINT('Ctrl Pts',(42.8155481055648,36.3702686449195,49.8838495603618));
#25458=CARTESIAN_POINT('Ctrl Pts',(42.8059188798285,36.3696194950306,49.8859465184157));
#25459=CARTESIAN_POINT('Ctrl Pts',(42.801347822297,36.3693125532805,49.8869245703072));
#25460=CARTESIAN_POINT('Ctrl Pts',(42.7904597057428,36.3685842165975,49.8892129037964));
#25461=CARTESIAN_POINT('Ctrl Pts',(42.7841394904624,36.3681636698291,49.8905081413376));
#25462=CARTESIAN_POINT('Ctrl Pts',(42.7616836474814,36.366676981367,49.8949928816099));
#25463=CARTESIAN_POINT('Ctrl Pts',(42.7455133236641,36.3656201846239,49.8980078157847));
#25464=CARTESIAN_POINT('Ctrl Pts',(42.6299433809009,36.3581522688903,49.9180296674882));
#25465=CARTESIAN_POINT('Ctrl Pts',(42.5293706754951,36.3520959837909,49.9274284002903));
#25466=CARTESIAN_POINT('Ctrl Pts',(42.3232388480361,36.3397833729224,49.9304754319349));
#25467=CARTESIAN_POINT('Ctrl Pts',(42.2180195067605,36.3335462658379,49.9234108632692));
#25468=CARTESIAN_POINT('Ctrl Pts',(42.0750336026653,36.3246833716208,49.9019685403077));
#25469=CARTESIAN_POINT('Ctrl Pts',(42.036351914111,36.3222474545379,49.8949531028532));
#25470=CARTESIAN_POINT('Ctrl Pts',(41.9702743615923,36.3180003441819,49.880871349407));
#25471=CARTESIAN_POINT('Ctrl Pts',(41.9427694664882,36.3162065200763,49.8743748999336));
#25472=CARTESIAN_POINT('Ctrl Pts',(41.9035994731228,36.313609944394,49.8642097963953));
#25473=CARTESIAN_POINT('Ctrl Pts',(41.8918102943711,36.312822949022,49.8610305907989));
#25474=CARTESIAN_POINT('Ctrl Pts',(41.8713651988944,36.3114481890472,49.8553083790504));
#25475=CARTESIAN_POINT('Ctrl Pts',(41.8626953763152,36.3108620910395,49.8528161460451));
#25476=CARTESIAN_POINT('Ctrl Pts',(41.8448952240478,36.3096521723843,49.847563861332));
#25477=CARTESIAN_POINT('Ctrl Pts',(41.8357672619247,36.309028133631,49.8447967220602));
#25478=CARTESIAN_POINT('Ctrl Pts',(41.8157889717394,36.3076542533022,49.8385781649168));
#25479=CARTESIAN_POINT('Ctrl Pts',(41.8049480515291,36.3069034943769,49.835098188119));
#25480=CARTESIAN_POINT('Ctrl Pts',(41.7941388317569,36.3061495715672,49.8315225365021));
#25481=CARTESIAN_POINT('Origin',(42.4,48.4493818343519,48.));
#25482=CARTESIAN_POINT('',(41.7941388318214,35.3402141276758,49.8315225365235));
#25483=CARTESIAN_POINT('',(41.7941383590443,35.5100558711261,49.8315223801304));
#25484=CARTESIAN_POINT('',(41.7941388317924,48.4493818343519,49.8315225365138));
#25485=CARTESIAN_POINT('Ctrl Pts',(41.7941388318214,35.3402141276758,49.8315225365234));
#25486=CARTESIAN_POINT('Ctrl Pts',(41.8033302780717,35.3409038661738,49.8345630343887));
#25487=CARTESIAN_POINT('Ctrl Pts',(41.812544588084,35.3415928991055,49.8375343336986));
#25488=CARTESIAN_POINT('Ctrl Pts',(41.8888872174798,35.3472800816834,49.8615192786733));
#25489=CARTESIAN_POINT('Ctrl Pts',(41.9571036059003,35.3522261553391,49.8789186026669));
#25490=CARTESIAN_POINT('Ctrl Pts',(42.0412603432048,35.3580545162817,49.8955438416919));
#25491=CARTESIAN_POINT('Ctrl Pts',(42.056432293349,35.3590945200303,49.8983524080361));
#25492=CARTESIAN_POINT('Ctrl Pts',(42.0783062494708,35.3605769491042,49.9021307776737));
#25493=CARTESIAN_POINT('Ctrl Pts',(42.084981757483,35.3610270909399,49.9032477176702));
#25494=CARTESIAN_POINT('Ctrl Pts',(42.0966222704121,35.3618079237036,49.9051324751577));
#25495=CARTESIAN_POINT('Ctrl Pts',(42.101584594612,35.3621394880998,49.9059160639689));
#25496=CARTESIAN_POINT('Ctrl Pts',(42.1121266725425,35.3628410595028,49.907538555089));
#25497=CARTESIAN_POINT('Ctrl Pts',(42.1177070830929,35.3632107806761,49.9083723700837));
#25498=CARTESIAN_POINT('Ctrl Pts',(42.1329564517591,35.3642167901322,49.9105825500303));
#25499=CARTESIAN_POINT('Ctrl Pts',(42.1426324898158,35.3648503952973,49.9119100166115));
#25500=CARTESIAN_POINT('Ctrl Pts',(42.1895318375846,35.367900406053,49.9179816883714));
#25501=CARTESIAN_POINT('Ctrl Pts',(42.2268808268281,35.3702652685993,49.9217129844686));
#25502=CARTESIAN_POINT('Ctrl Pts',(42.300000531919,35.3748117286257,49.9268685110003));
#25503=CARTESIAN_POINT('Ctrl Pts',(42.3357481680346,35.3769958187494,49.928391581943));
#25504=CARTESIAN_POINT('Ctrl Pts',(42.4868752137132,35.3861408098428,49.9306230087209));
#25505=CARTESIAN_POINT('Ctrl Pts',(42.6021524449234,35.392912627826,49.921975047383));
#25506=CARTESIAN_POINT('Ctrl Pts',(42.7996080457485,35.4050085530928,49.8891914717841));
#25507=CARTESIAN_POINT('Ctrl Pts',(42.8822316284253,35.4102238279034,49.869807742403));
#25508=CARTESIAN_POINT('Ctrl Pts',(42.9801412610197,35.4167376910143,49.8399153541119));
#25509=CARTESIAN_POINT('Ctrl Pts',(42.9969046888878,35.4178648489885,49.8345454893335));
#25510=CARTESIAN_POINT('Ctrl Pts',(43.0232107565205,35.4196535666268,49.8257200899659));
#25511=CARTESIAN_POINT('Ctrl Pts',(43.0328038950717,35.4203100808338,49.822417273238));
#25512=CARTESIAN_POINT('Ctrl Pts',(43.0507333286609,35.4215452250147,49.8160857227827));
#25513=CARTESIAN_POINT('Ctrl Pts',(43.0590756871328,35.4221232469345,49.8130748610368));
#25514=CARTESIAN_POINT('Ctrl Pts',(43.0777281259963,35.4234232414845,49.8061972180578));
#25515=CARTESIAN_POINT('Ctrl Pts',(43.0880263890052,35.4241462345755,49.8022994986282));
#25516=CARTESIAN_POINT('Ctrl Pts',(43.1141855822169,35.4259964313371,49.7921418074748));
#25517=CARTESIAN_POINT('Ctrl Pts',(43.1299976406923,35.4271277151774,49.7857594229469));
#25518=CARTESIAN_POINT('Ctrl Pts',(43.2470824220886,35.435603420777,49.736684380505));
#25519=CARTESIAN_POINT('Ctrl Pts',(43.3446088698674,35.4432352910934,49.6856238950551));
#25520=CARTESIAN_POINT('Ctrl Pts',(43.5589761464888,35.461268422096,49.5489225952098));
#25521=CARTESIAN_POINT('Ctrl Pts',(43.6716094957436,35.4717449957763,49.4578747941354));
#25522=CARTESIAN_POINT('Ctrl Pts',(43.7878719216008,35.48307648185,49.3400747652066));
#25523=CARTESIAN_POINT('Ctrl Pts',(43.8024642967664,35.4845086051447,49.3247953932939));
#25524=CARTESIAN_POINT('Ctrl Pts',(43.8220027532965,35.4864360967266,49.3036523365457));
#25525=CARTESIAN_POINT('Ctrl Pts',(43.8271686096639,35.4869466903525,49.2979949959321));
#25526=CARTESIAN_POINT('Ctrl Pts',(43.835772045806,35.4877984753721,49.2884595614572));
#25527=CARTESIAN_POINT('Ctrl Pts',(43.8392279069567,35.4881410136081,49.2845981640024));
#25528=CARTESIAN_POINT('Ctrl Pts',(43.8457724308015,35.4887903607895,49.2772260952095));
#25529=CARTESIAN_POINT('Ctrl Pts',(43.8488639442129,35.4890973910311,49.273718058393));
#25530=CARTESIAN_POINT('Ctrl Pts',(43.8561917023474,35.4898259320701,49.2653418221002));
#25531=CARTESIAN_POINT('Ctrl Pts',(43.860416368106,35.4902465942611,49.2604635002365));
#25532=CARTESIAN_POINT('Ctrl Pts',(43.8753241716578,35.4917336682518,49.2430735336266));
#25533=CARTESIAN_POINT('Ctrl Pts',(43.8858720069806,35.4927907305562,49.2304461157585));
#25534=CARTESIAN_POINT('Ctrl Pts',(43.9595323284834,35.5002207476962,49.1399343489077));
#25535=CARTESIAN_POINT('Ctrl Pts',(44.0166592637935,35.5062431981322,49.0573596350628));
#25536=CARTESIAN_POINT('Ctrl Pts',(44.1203081332262,35.5185469002135,48.8793511025263));
#25537=CARTESIAN_POINT('Ctrl Pts',(44.1659006178351,35.5248081372512,48.7837806045677));
#25538=CARTESIAN_POINT('Ctrl Pts',(44.2174211053208,35.5337019972348,48.6481318962427));
#25539=CARTESIAN_POINT('Ctrl Pts',(44.2302762596672,35.5361431828442,48.6108870151002));
#25540=CARTESIAN_POINT('Ctrl Pts',(44.25039427698,35.5403987310147,48.5462462604069));
#25541=CARTESIAN_POINT('Ctrl Pts',(44.2582104534106,35.5421956313585,48.5190353903268));
#25542=CARTESIAN_POINT('Ctrl Pts',(44.2685394077921,35.5447960126869,48.4798462116819));
#25543=CARTESIAN_POINT('Ctrl Pts',(44.2715416178398,35.545583675958,48.4679998576269));
#25544=CARTESIAN_POINT('Ctrl Pts',(44.2765648423415,35.5469593518779,48.4473571233139));
#25545=CARTESIAN_POINT('Ctrl Pts',(44.2786370790861,35.5475456933324,48.4385735100676));
#25546=CARTESIAN_POINT('Ctrl Pts',(44.282517747946,35.5486812991517,48.4215921666877));
#25547=CARTESIAN_POINT('Ctrl Pts',(44.2843344549966,35.5492302823014,48.413396521851));
#25548=CARTESIAN_POINT('Ctrl Pts',(44.2885229323607,35.5505385452273,48.3938997697985));
#25549=CARTESIAN_POINT('Ctrl Pts',(44.2908468160997,35.5512993411058,48.3825888169371));
#25550=CARTESIAN_POINT('Ctrl Pts',(44.298795008162,35.5540322159728,48.3420604505009));
#25551=CARTESIAN_POINT('Ctrl Pts',(44.3038445068806,35.5560223998313,48.3127359274706));
#25552=CARTESIAN_POINT('Ctrl Pts',(44.3341200523289,35.5699575131201,48.1088155663776));
#25553=CARTESIAN_POINT('Ctrl Pts',(44.3359651641253,35.5826613566377,47.9316181871203));
#25554=CARTESIAN_POINT('Ctrl Pts',(44.3050852516379,35.6000507892934,47.6887364079094));
#25555=CARTESIAN_POINT('Ctrl Pts',(44.2928315150079,35.6048625665033,47.6212842600879));
#25556=CARTESIAN_POINT('Ctrl Pts',(44.2734970491747,35.6105508409513,47.5398007282598));
#25557=CARTESIAN_POINT('Ctrl Pts',(44.2698049527442,35.6115773539234,47.5250220664612));
#25558=CARTESIAN_POINT('Ctrl Pts',(44.2642288070903,35.6130441499113,47.5037754048378));
#25559=CARTESIAN_POINT('Ctrl Pts',(44.2624854373206,35.6134919328008,47.4972715512534));
#25560=CARTESIAN_POINT('Ctrl Pts',(44.2593831730957,35.6142700898996,47.4859358376487));
#25561=CARTESIAN_POINT('Ctrl Pts',(44.2580394246438,35.6146013193269,47.4810999651133));
#25562=CARTESIAN_POINT('Ctrl Pts',(44.2551399889293,35.6153037434277,47.470821182123));
#25563=CARTESIAN_POINT('Ctrl Pts',(44.2535792094199,35.615674641107,47.4653798392673));
#25564=CARTESIAN_POINT('Ctrl Pts',(44.2492369480064,35.6166872387055,47.4504890420384));
#25565=CARTESIAN_POINT('Ctrl Pts',(44.2464069623751,35.6173261962535,47.441053739516));
#25566=CARTESIAN_POINT('Ctrl Pts',(44.2321571334049,35.6204450335939,47.3948336665334));
#25567=CARTESIAN_POINT('Ctrl Pts',(44.2197088382456,35.6228705310141,47.3583721736087));
#25568=CARTESIAN_POINT('Ctrl Pts',(44.1936662520892,35.627464050469,47.2889640981841));
#25569=CARTESIAN_POINT('Ctrl Pts',(44.1802349988333,35.6296367702057,47.2559742891568));
#25570=CARTESIAN_POINT('Ctrl Pts',(44.1197835874882,35.6387176826446,47.1185194841136));
#25571=CARTESIAN_POINT('Ctrl Pts',(44.0644222262479,35.6454430282479,47.0179800221821));
#25572=CARTESIAN_POINT('Ctrl Pts',(43.9532145863593,35.6574809902782,46.8527293430705));
#25573=CARTESIAN_POINT('Ctrl Pts',(43.9013984947038,35.6626874036156,46.7857078552327));
#25574=CARTESIAN_POINT('Ctrl Pts',(43.833701161272,35.6691912866582,46.7091269959231));
#25575=CARTESIAN_POINT('Ctrl Pts',(43.8218684200407,35.6703179789034,46.6961049522164));
#25576=CARTESIAN_POINT('Ctrl Pts',(43.8029354741763,35.672106124299,46.6758332745595));
#25577=CARTESIAN_POINT('Ctrl Pts',(43.7959531686412,35.6727625375185,46.6684744816957));
#25578=CARTESIAN_POINT('Ctrl Pts',(43.78275794,35.6739975928945,46.6547856305013));
#25579=CARTESIAN_POINT('Ctrl Pts',(43.7765587457916,35.674575627863,46.6484426628917));
#25580=CARTESIAN_POINT('Ctrl Pts',(43.7625640817177,35.6758757853019,46.6343195922553));
#25581=CARTESIAN_POINT('Ctrl Pts',(43.7547453335138,35.6765989293644,46.6265630973217));
#25582=CARTESIAN_POINT('Ctrl Pts',(43.7346478432983,35.678449773532,46.6069642174193));
#25583=CARTESIAN_POINT('Ctrl Pts',(43.7222778648127,35.6795815587051,46.5952171792515));
#25584=CARTESIAN_POINT('Ctrl Pts',(43.628538139522,35.6881056045999,46.5085332549671));
#25585=CARTESIAN_POINT('Ctrl Pts',(43.5410273426897,35.6957892969913,46.4405680380701));
#25586=CARTESIAN_POINT('Ctrl Pts',(43.3275591281659,35.7138287250294,46.3024062509263));
#25587=CARTESIAN_POINT('Ctrl Pts',(43.1985800840218,35.7242535564755,46.2380513281266));
#25588=CARTESIAN_POINT('Ctrl Pts',(43.0438461358926,35.7355353344091,46.1813605534341));
#25589=CARTESIAN_POINT('Ctrl Pts',(43.0239260948757,35.7369648983567,46.1744306089116));
#25590=CARTESIAN_POINT('Ctrl Pts',(42.9966245569341,35.7388895376939,46.1654318480802));
#25591=CARTESIAN_POINT('Ctrl Pts',(42.9893393207583,35.7393997819224,46.1630785711183));
#25592=CARTESIAN_POINT('Ctrl Pts',(42.9771006999296,35.7402511479475,46.1592055573119));
#25593=CARTESIAN_POINT('Ctrl Pts',(42.9721549114014,35.7405936137911,46.1576623117492));
#25594=CARTESIAN_POINT('Ctrl Pts',(42.9627328283422,35.7412429501227,46.1547639194843));
#25595=CARTESIAN_POINT('Ctrl Pts',(42.9582577449077,35.7415500410646,46.1534051011798));
#25596=CARTESIAN_POINT('Ctrl Pts',(42.9475924973663,35.742278885269,46.1502090101486));
#25597=CARTESIAN_POINT('Ctrl Pts',(42.9413979146882,35.7426997882691,46.1483865008586));
#25598=CARTESIAN_POINT('Ctrl Pts',(42.9193670539494,35.7441885097917,46.142024810198));
#25599=CARTESIAN_POINT('Ctrl Pts',(42.9034813877032,35.7452469520633,46.1376572607379));
#25600=CARTESIAN_POINT('Ctrl Pts',(42.7882470058594,35.7528297287946,46.1075574467411));
#25601=CARTESIAN_POINT('Ctrl Pts',(42.6870280143813,35.7589864323924,46.089582520301));
#25602=CARTESIAN_POINT('Ctrl Pts',(42.4776974887853,35.7715431291362,46.0694318675237));
#25603=CARTESIAN_POINT('Ctrl Pts',(42.3698779855397,35.7779231960003,46.0681042451951));
#25604=CARTESIAN_POINT('Ctrl Pts',(42.2068783852868,35.7879645727898,46.0797506246203));
#25605=CARTESIAN_POINT('Ctrl Pts',(42.1514464770122,35.7914472096446,46.0861364021845));
#25606=CARTESIAN_POINT('Ctrl Pts',(42.080927083342,35.7960033896666,46.0973755869808));
#25607=CARTESIAN_POINT('Ctrl Pts',(42.0655123784125,35.7970070020544,46.1000249499417));
#25608=CARTESIAN_POINT('Ctrl Pts',(42.0405744557355,35.7986438912036,46.10462397202));
#25609=CARTESIAN_POINT('Ctrl Pts',(42.0310305653726,35.7992734978333,46.1064587250703));
#25610=CARTESIAN_POINT('Ctrl Pts',(42.0127209129363,35.8004876402576,46.1101223204696));
#25611=CARTESIAN_POINT('Ctrl Pts',(42.0039532022826,35.8010718120072,46.111940238151));
#25612=CARTESIAN_POINT('Ctrl Pts',(41.9838884793858,35.8024151841456,46.1162464148082));
#25613=CARTESIAN_POINT('Ctrl Pts',(41.9726006469372,35.8031756731564,46.1187753588755));
#25614=CARTESIAN_POINT('Ctrl Pts',(41.9366831413262,35.8056110576489,46.1271623213788));
#25615=CARTESIAN_POINT('Ctrl Pts',(41.9121466022736,35.8072981816249,46.1334035143323));
#25616=CARTESIAN_POINT('Ctrl Pts',(41.7579383176441,35.8180550401724,46.1758765896848));
#25617=CARTESIAN_POINT('Ctrl Pts',(41.6322578000882,35.8275517630079,46.2251115547733));
#25618=CARTESIAN_POINT('Ctrl Pts',(41.4467387002653,35.8424713223208,46.3212023606692));
#25619=CARTESIAN_POINT('Ctrl Pts',(41.3827593667456,35.8477938873122,46.3591798238934));
#25620=CARTESIAN_POINT('Ctrl Pts',(41.2927309666345,35.8554231763513,46.4199141275866));
#25621=CARTESIAN_POINT('Ctrl Pts',(41.2648458632006,35.8578067979939,46.4398264707362));
#25622=CARTESIAN_POINT('Ctrl Pts',(41.2201887959747,35.8616405563775,46.4735469672153));
#25623=CARTESIAN_POINT('Ctrl Pts',(41.2030941675991,35.8631122080513,46.4869137947167));
#25624=CARTESIAN_POINT('Ctrl Pts',(41.1802122628839,35.8650836733035,46.5054364072132));
#25625=CARTESIAN_POINT('Ctrl Pts',(41.1742259127801,35.8655995971504,46.5103422041754));
#25626=CARTESIAN_POINT('Ctrl Pts',(41.1642684820652,35.866457782343,46.5186029589881));
#25627=CARTESIAN_POINT('Ctrl Pts',(41.1602811984603,35.8668014332912,46.5219381363983));
#25628=CARTESIAN_POINT('Ctrl Pts',(41.1527438123534,35.8674509862469,46.5282947679145));
#25629=CARTESIAN_POINT('Ctrl Pts',(41.1491911117259,35.8677571222345,46.5313130306487));
#25630=CARTESIAN_POINT('Ctrl Pts',(41.1407890093403,35.8684811643652,46.5385037929997));
#25631=CARTESIAN_POINT('Ctrl Pts',(41.1359493155519,35.8688982464469,46.5426876271479));
#25632=CARTESIAN_POINT('Ctrl Pts',(41.1189902317767,35.870360238262,46.5574965177927));
#25633=CARTESIAN_POINT('Ctrl Pts',(41.1069828718956,35.8713962040948,46.5682496482087));
#25634=CARTESIAN_POINT('Ctrl Pts',(41.0096141195906,35.879817860873,46.6576719015802));
#25635=CARTESIAN_POINT('Ctrl Pts',(40.9313663533926,35.8867284689508,46.743759473144));
#25636=CARTESIAN_POINT('Ctrl Pts',(40.8021594920841,35.8995046798798,46.9146104820451));
#25637=CARTESIAN_POINT('Ctrl Pts',(40.7490474419872,35.9053478185504,46.9972445070508));
#25638=CARTESIAN_POINT('Ctrl Pts',(40.6857641258392,35.9135497513982,47.1144651653818));
#25639=CARTESIAN_POINT('Ctrl Pts',(40.6699242881312,35.9157351135803,47.1458253177254));
#25640=CARTESIAN_POINT('Ctrl Pts',(40.6438905627417,35.9195831747945,47.201066198481));
#25641=CARTESIAN_POINT('Ctrl Pts',(40.6333060076736,35.921232701729,47.2247530651251));
#25642=CARTESIAN_POINT('Ctrl Pts',(40.6186040843262,35.9236566831083,47.2595200502337));
#25643=CARTESIAN_POINT('Ctrl Pts',(40.6141054950346,35.9244181856518,47.2704365885575));
#25644=CARTESIAN_POINT('Ctrl Pts',(40.6063698229777,35.9257635656237,47.2897087723692));
#25645=CARTESIAN_POINT('Ctrl Pts',(40.6030901870596,35.9263459855643,47.2980470389086));
#25646=CARTESIAN_POINT('Ctrl Pts',(40.5963810828625,35.9275630733627,47.3154596721654));
#25647=CARTESIAN_POINT('Ctrl Pts',(40.5929617435125,35.9281980620767,47.3245376454294));
#25648=CARTESIAN_POINT('Ctrl Pts',(40.5842371558487,35.9298574775942,47.3482409257297));
#25649=CARTESIAN_POINT('Ctrl Pts',(40.5790401940719,35.9308854772998,47.362905063542));
#25650=CARTESIAN_POINT('Ctrl Pts',(40.558040970974,35.9352113449188,47.4245149422172));
#25651=CARTESIAN_POINT('Ctrl Pts',(40.5438736871017,35.9385621867252,47.4719938729788));
#25652=CARTESIAN_POINT('Ctrl Pts',(40.5232940881895,35.9442469674777,47.5520957435843));
#25653=CARTESIAN_POINT('Ctrl Pts',(40.5158690386701,35.946550328313,47.5844357698192));
#25654=CARTESIAN_POINT('Ctrl Pts',(40.4836525613635,35.9579079144048,47.7434548103538));
#25655=CARTESIAN_POINT('Ctrl Pts',(40.4707855165445,35.9672308213055,47.8722096932965));
#25656=CARTESIAN_POINT('Ctrl Pts',(40.4708892210066,35.9783792649736,48.0298529101713));
#25657=CARTESIAN_POINT('Ctrl Pts',(40.4715433127891,35.980388420854,48.058433939243));
#25658=CARTESIAN_POINT('Ctrl Pts',(40.4745029935232,35.9849562189986,48.1240017126534));
#25659=CARTESIAN_POINT('Ctrl Pts',(40.4772396008765,35.9875006195136,48.160959697775));
#25660=CARTESIAN_POINT('Ctrl Pts',(40.4820365303732,35.9906477441484,48.2074928195425));
#25661=CARTESIAN_POINT('Ctrl Pts',(40.483106973208,35.9912984267554,48.2171595602671));
#25662=CARTESIAN_POINT('Ctrl Pts',(40.48491283704,35.9923197775349,48.2324122391863));
#25663=CARTESIAN_POINT('Ctrl Pts',(40.4855996816826,35.9926930533686,48.2380036006194));
#25664=CARTESIAN_POINT('Ctrl Pts',(40.4869456863818,35.9933967447851,48.2485779822284));
#25665=CARTESIAN_POINT('Ctrl Pts',(40.4875998221225,35.9937274159223,48.2535613935973));
#25666=CARTESIAN_POINT('Ctrl Pts',(40.4891828443403,35.9945019400442,48.2652666539683));
#25667=CARTESIAN_POINT('Ctrl Pts',(40.4901277284859,35.994944890912,48.2719862312696));
#25668=CARTESIAN_POINT('Ctrl Pts',(40.4933512971333,35.9963952288634,48.2940652637638));
#25669=CARTESIAN_POINT('Ctrl Pts',(40.495780033281,35.9973945932102,48.3094026678246));
#25670=CARTESIAN_POINT('Ctrl Pts',(40.5103908968587,36.0029329080415,48.3949686755102));
#25671=CARTESIAN_POINT('Ctrl Pts',(40.5262740071337,36.0072954823843,48.4645169124358));
#25672=CARTESIAN_POINT('Ctrl Pts',(40.5600992665858,36.0146766533295,48.582169941512));
#25673=CARTESIAN_POINT('Ctrl Pts',(40.5761742080762,36.0177232058786,48.6307267644071));
#25674=CARTESIAN_POINT('Ctrl Pts',(40.6395398287821,36.0284671413047,48.7993535669446));
#25675=CARTESIAN_POINT('Ctrl Pts',(40.6969134736692,36.0361772909899,48.9152470742577));
#25676=CARTESIAN_POINT('Ctrl Pts',(40.778941962411,36.0459147116489,49.0461174750438));
#25677=CARTESIAN_POINT('Ctrl Pts',(40.7928905407786,36.047534341355,49.0674221386184));
#25678=CARTESIAN_POINT('Ctrl Pts',(40.8137977561194,36.0499142845872,49.0980161298463));
#25679=CARTESIAN_POINT('Ctrl Pts',(40.8204253568025,36.0506621232496,49.1075291945575));
#25680=CARTESIAN_POINT('Ctrl Pts',(40.8323250300456,36.0519936024174,49.1242855482265));
#25681=CARTESIAN_POINT('Ctrl Pts',(40.8375626076014,36.0525759063517,49.1315530017028));
#25682=CARTESIAN_POINT('Ctrl Pts',(40.8485803594892,36.053793269538,49.1466184507041));
#25683=CARTESIAN_POINT('Ctrl Pts',(40.8543691393466,36.0544286532587,49.1544098099055));
#25684=CARTESIAN_POINT('Ctrl Pts',(40.8696049201544,36.0560902556816,49.1745962434354));
#25685=CARTESIAN_POINT('Ctrl Pts',(40.8791436051263,36.0571200648081,49.1869209060955));
#25686=CARTESIAN_POINT('Ctrl Pts',(40.9231176019948,36.0618218832734,49.2423379684117));
#25687=CARTESIAN_POINT('Ctrl Pts',(40.9592390822894,36.0655610290211,49.2840530303269));
#25688=CARTESIAN_POINT('Ctrl Pts',(41.0695135055077,36.0766418746174,49.4008852294146));
#25689=CARTESIAN_POINT('Ctrl Pts',(41.1480967349268,36.0841481440338,49.471532332966));
#25690=CARTESIAN_POINT('Ctrl Pts',(41.2700500592625,36.0950946170216,49.5643002220425));
#25691=CARTESIAN_POINT('Ctrl Pts',(41.3091103143498,36.0985054552505,49.5917857678542));
#25692=CARTESIAN_POINT('Ctrl Pts',(41.4045201770809,36.106562000376,49.6537598907998));
#25693=CARTESIAN_POINT('Ctrl Pts',(41.4617059300286,36.1111761188832,49.6868633639615));
#25694=CARTESIAN_POINT('Ctrl Pts',(41.5296176820638,36.1163260843162,49.7216511038361));
#25695=CARTESIAN_POINT('Ctrl Pts',(41.538790164072,36.117014927706,49.7262576668846));
#25696=CARTESIAN_POINT('Ctrl Pts',(41.5537069929559,36.1181237784755,49.7336006392286));
#25697=CARTESIAN_POINT('Ctrl Pts',(41.5594287343966,36.1185464174024,49.7363821527584));
#25698=CARTESIAN_POINT('Ctrl Pts',(41.5696542805438,36.1192968091254,49.7412907135717));
#25699=CARTESIAN_POINT('Ctrl Pts',(41.574152661941,36.1196252218318,49.7434286733582));
#25700=CARTESIAN_POINT('Ctrl Pts',(41.583996553106,36.1203401805565,49.748060560429));
#25701=CARTESIAN_POINT('Ctrl Pts',(41.5893452434245,36.1207262923272,49.7505474047297));
#25702=CARTESIAN_POINT('Ctrl Pts',(41.6046568312521,36.1218251110056,49.7575812161948));
#25703=CARTESIAN_POINT('Ctrl Pts',(41.6146473479717,36.1225342477433,49.7620680217135));
#25704=CARTESIAN_POINT('Ctrl Pts',(41.6801092164973,36.1271334040668,49.7908000016156));
#25705=CARTESIAN_POINT('Ctrl Pts',(41.736659542496,36.1308858498512,49.8125085912373));
#25706=CARTESIAN_POINT('Ctrl Pts',(41.7941388330275,36.1345714126848,49.8315225369224));
#25707=CARTESIAN_POINT('Ctrl Pts',(41.7941388317569,36.3061495715672,49.8315225365021));
#25708=CARTESIAN_POINT('Ctrl Pts',(41.7908818344471,36.3059224021124,49.8304451333276));
#25709=CARTESIAN_POINT('Ctrl Pts',(41.7876277152645,36.3056949455745,49.8293590436659));
#25710=CARTESIAN_POINT('Ctrl Pts',(41.7433255545585,36.3025916264315,49.8144413694751));
#25711=CARTESIAN_POINT('Ctrl Pts',(41.7027548568271,36.2996709716044,49.7992408149969));
#25712=CARTESIAN_POINT('Ctrl Pts',(41.5129913184719,36.2856236380944,49.7207602334871));
#25713=CARTESIAN_POINT('Ctrl Pts',(41.3716646382245,36.2739304407638,49.6402166971355));
#25714=CARTESIAN_POINT('Ctrl Pts',(41.2033214709907,36.2589999196495,49.5138868096297));
#25715=CARTESIAN_POINT('Ctrl Pts',(41.1656541819422,36.2555903400025,49.4833353647865));
#25716=CARTESIAN_POINT('Ctrl Pts',(41.1152000832895,36.2509656751783,49.4391583623508));
#25717=CARTESIAN_POINT('Ctrl Pts',(41.1014013252953,36.2496946090662,49.4267197188221));
#25718=CARTESIAN_POINT('Ctrl Pts',(41.0777227243126,36.2475056167022,49.404746865659));
#25719=CARTESIAN_POINT('Ctrl Pts',(41.0677611731111,36.2465822161296,49.3953030799677));
#25720=CARTESIAN_POINT('Ctrl Pts',(41.0532637890158,36.2452357783986,49.3812623963285));
#25721=CARTESIAN_POINT('Ctrl Pts',(41.0486491424598,36.2448068032589,49.3767480133658));
#25722=CARTESIAN_POINT('Ctrl Pts',(41.040510145783,36.244049651584,49.3687055049526));
#25723=CARTESIAN_POINT('Ctrl Pts',(41.0369767183921,36.2437207650918,49.3651867853233));
#25724=CARTESIAN_POINT('Ctrl Pts',(41.0293438611388,36.2430099399321,49.357526523088));
#25725=CARTESIAN_POINT('Ctrl Pts',(41.0252495324038,36.2426283962253,49.3533800892379));
#25726=CARTESIAN_POINT('Ctrl Pts',(41.013946139364,36.2415741298078,49.3418286232391));
#25727=CARTESIAN_POINT('Ctrl Pts',(41.0067775679538,36.2409044674379,49.3343839871123));
#25728=CARTESIAN_POINT('Ctrl Pts',(40.9674302083481,36.2372204400329,49.2928585671319));
#25729=CARTESIAN_POINT('Ctrl Pts',(40.9364391153363,36.2342874434137,49.2576684068972));
#25730=CARTESIAN_POINT('Ctrl Pts',(40.7958803198214,36.2206358269088,49.0858233743734));
#25731=CARTESIAN_POINT('Ctrl Pts',(40.7039737120503,36.2105604331078,48.9357966911778));
#25732=CARTESIAN_POINT('Ctrl Pts',(40.6117241073231,36.1964440349564,48.7256487404426));
#25733=CARTESIAN_POINT('Ctrl Pts',(40.5919917965607,36.193047714367,48.674983157969));
#25734=CARTESIAN_POINT('Ctrl Pts',(40.5694133467828,36.1885900208047,48.6088805628605));
#25735=CARTESIAN_POINT('Ctrl Pts',(40.56457813582,36.1875948067407,48.5941461036755));
#25736=CARTESIAN_POINT('Ctrl Pts',(40.5570117615196,36.1859683469113,48.5701146930645));
#25737=CARTESIAN_POINT('Ctrl Pts',(40.5541720195687,36.1853406851394,48.5608524506284));
#25738=CARTESIAN_POINT('Ctrl Pts',(40.5488401839491,36.1841280339897,48.5429826767567));
#25739=CARTESIAN_POINT('Ctrl Pts',(40.5463380586566,36.1835433911786,48.534378381351));
#25740=CARTESIAN_POINT('Ctrl Pts',(40.5407276538539,36.1821957008626,48.5145717158341));
#25741=CARTESIAN_POINT('Ctrl Pts',(40.5376605375903,36.181431335032,48.5033581473886));
#25742=CARTESIAN_POINT('Ctrl Pts',(40.5283953939592,36.1790328871414,48.4682398882855));
#25743=CARTESIAN_POINT('Ctrl Pts',(40.5225551060856,36.1773873613241,48.4442442662499));
#25744=CARTESIAN_POINT('Ctrl Pts',(40.4862671368741,36.1661856084915,48.2816243005021));
#25745=CARTESIAN_POINT('Ctrl Pts',(40.4707431824734,36.1561485615077,48.1401412126996));
#25746=CARTESIAN_POINT('Ctrl Pts',(40.4709683571867,36.1382629653343,47.8897689155703));
#25747=CARTESIAN_POINT('Ctrl Pts',(40.4802186425955,36.1305007920714,47.7814640440312));
#25748=CARTESIAN_POINT('Ctrl Pts',(40.5012919379288,36.1219987210722,47.6583590742255));
#25749=CARTESIAN_POINT('Ctrl Pts',(40.5042611201627,36.1208928690299,47.64225012882));
#25750=CARTESIAN_POINT('Ctrl Pts',(40.5086831317974,36.1193671354483,47.619862481187));
#25751=CARTESIAN_POINT('Ctrl Pts',(40.5099626809845,36.1189382312745,47.613550825054));
#25752=CARTESIAN_POINT('Ctrl Pts',(40.5122249145439,36.1182012418579,47.6026719156325));
#25753=CARTESIAN_POINT('Ctrl Pts',(40.5131926166968,36.1178923263549,47.5981016554198));
#25754=CARTESIAN_POINT('Ctrl Pts',(40.5152690945295,36.117242676471,47.5884676923484));
#25755=CARTESIAN_POINT('Ctrl Pts',(40.5163816950951,36.1169021737739,47.5834048622162));
#25756=CARTESIAN_POINT('Ctrl Pts',(40.5191919991851,36.1160604389258,47.5708581706228));
#25757=CARTESIAN_POINT('Ctrl Pts',(40.5209139994945,36.1155605792031,47.5633797379441));
#25758=CARTESIAN_POINT('Ctrl Pts',(40.5275677143037,36.1136868309566,47.53525212076));
#25759=CARTESIAN_POINT('Ctrl Pts',(40.5327957564722,36.1123288065494,47.5146736573835));
#25760=CARTESIAN_POINT('Ctrl Pts',(40.5767323183008,36.1017285302389,47.352966529564));
#25761=CARTESIAN_POINT('Ctrl Pts',(40.6310507611253,36.0931889930527,47.2165540505824));
#25762=CARTESIAN_POINT('Ctrl Pts',(40.7512827782719,36.0779600412097,46.9925768559419));
#25763=CARTESIAN_POINT('Ctrl Pts',(40.810151556689,36.0714072727013,46.9020258410857));
#25764=CARTESIAN_POINT('Ctrl Pts',(40.8867142086564,36.0634773229606,46.803422104243));
#25765=CARTESIAN_POINT('Ctrl Pts',(40.8973354425698,36.0623889670591,46.7901108542115));
#25766=CARTESIAN_POINT('Ctrl Pts',(40.915106928134,36.0605858587203,46.7684334436592));
#25767=CARTESIAN_POINT('Ctrl Pts',(40.9221551601202,36.059875216884,46.7599845813372));
#25768=CARTESIAN_POINT('Ctrl Pts',(40.9350126821654,36.0585865868372,46.7448373322373));
#25769=CARTESIAN_POINT('Ctrl Pts',(40.9407966492126,36.0580096499316,46.738117778635));
#25770=CARTESIAN_POINT('Ctrl Pts',(40.9532987577343,36.056768310838,46.7237942867901));
#25771=CARTESIAN_POINT('Ctrl Pts',(40.9600309578135,36.0561033316268,46.7162030309824));
#25772=CARTESIAN_POINT('Ctrl Pts',(40.9786130049928,36.0542770315661,46.6955798952041));
#25773=CARTESIAN_POINT('Ctrl Pts',(40.9905817006012,36.0531107037025,46.6826569081918));
#25774=CARTESIAN_POINT('Ctrl Pts',(41.0613941440343,36.0462656170772,46.6082681923181));
#25775=CARTESIAN_POINT('Ctrl Pts',(41.1240679172102,36.0404197920014,46.5505943433962));
#25776=CARTESIAN_POINT('Ctrl Pts',(41.2816697756335,36.0262161761693,46.4237299087403));
#25777=CARTESIAN_POINT('Ctrl Pts',(41.3795146820032,36.0177641336662,46.3586905121666));
#25778=CARTESIAN_POINT('Ctrl Pts',(41.5425881991134,36.004625859593,46.2705405070667));
#25779=CARTESIAN_POINT('Ctrl Pts',(41.6042094893347,35.9998586933071,46.2413344087271));
#25780=CARTESIAN_POINT('Ctrl Pts',(41.676822816558,35.9945598539716,46.2115189883723));
#25781=CARTESIAN_POINT('Ctrl Pts',(41.6864238503438,35.9938654994304,46.2076667001465));
#25782=CARTESIAN_POINT('Ctrl Pts',(41.7020003727046,35.9927496242606,46.2015618317022));
#25783=CARTESIAN_POINT('Ctrl Pts',(41.7079567197463,35.9923254182321,46.1992614220683));
#25784=CARTESIAN_POINT('Ctrl Pts',(41.71857971423,35.9915734324963,46.1952191933506));
#25785=CARTESIAN_POINT('Ctrl Pts',(41.7232417949656,35.9912449800183,46.1934658321132));
#25786=CARTESIAN_POINT('Ctrl Pts',(41.7334202243369,35.9905313223843,46.189682760773));
#25787=CARTESIAN_POINT('Ctrl Pts',(41.7389390819324,35.990146540647,46.1876601949854));
#25788=CARTESIAN_POINT('Ctrl Pts',(41.7546796651775,35.9890550258491,46.1819730112076));
#25789=CARTESIAN_POINT('Ctrl Pts',(41.7649234019374,35.9883517901926,46.178369358411));
#25790=CARTESIAN_POINT('Ctrl Pts',(41.836746004218,35.983467054265,46.153782331771));
#25791=CARTESIAN_POINT('Ctrl Pts',(41.8993283958585,35.9794452234469,46.1358367517752));
#25792=CARTESIAN_POINT('Ctrl Pts',(42.0895849158426,35.9675848869307,46.0915567467151));
#25793=CARTESIAN_POINT('Ctrl Pts',(42.2191311079365,35.9599710796708,46.0749541098837));
#25794=CARTESIAN_POINT('Ctrl Pts',(42.4252953261542,35.947460117554,46.0695409812214));
#25795=CARTESIAN_POINT('Ctrl Pts',(42.5012685751251,35.9427705950798,46.0720335745036));
#25796=CARTESIAN_POINT('Ctrl Pts',(42.5943548472393,35.9368236097639,46.0806052236105));
#25797=CARTESIAN_POINT('Ctrl Pts',(42.6117950567736,35.9357008495776,46.0824513211891));
#25798=CARTESIAN_POINT('Ctrl Pts',(42.6393662543867,35.9339112247117,46.0857505290942));
#25799=CARTESIAN_POINT('Ctrl Pts',(42.6495152871925,35.9332493058624,46.0870469542192));
#25800=CARTESIAN_POINT('Ctrl Pts',(42.6684311192652,35.9320095158898,46.0896163313034));
#25801=CARTESIAN_POINT('Ctrl Pts',(42.6772004288766,35.931432300051,46.0908690602191));
#25802=CARTESIAN_POINT('Ctrl Pts',(42.6967285598873,35.9301412959678,46.0937961098347));
#25803=CARTESIAN_POINT('Ctrl Pts',(42.7074823920295,35.9294265480794,46.0955011999353));
#25804=CARTESIAN_POINT('Ctrl Pts',(42.7390791986472,35.9273149556571,46.1007856659793));
#25805=CARTESIAN_POINT('Ctrl Pts',(42.7598778519137,35.9259101769431,46.1046167510428));
#25806=CARTESIAN_POINT('Ctrl Pts',(42.9195269029133,35.9150088225237,46.1367463244995));
#25807=CARTESIAN_POINT('Ctrl Pts',(43.0549154811712,35.905023343791,46.1799194009701));
#25808=CARTESIAN_POINT('Ctrl Pts',(43.2894912819307,35.8866877203995,46.2843087196769));
#25809=CARTESIAN_POINT('Ctrl Pts',(43.3902617793463,35.8784322864802,46.3404284612018));
#25810=CARTESIAN_POINT('Ctrl Pts',(43.4987940954171,35.8694980836158,46.4142965997338));
#25811=CARTESIAN_POINT('Ctrl Pts',(43.5120400941541,35.8684071984331,46.4235576100569));
#25812=CARTESIAN_POINT('Ctrl Pts',(43.530370224039,35.8668986388196,46.4367192449479));
#25813=CARTESIAN_POINT('Ctrl Pts',(43.5355532456459,35.8664721966729,46.4404800765311));
#25814=CARTESIAN_POINT('Ctrl Pts',(43.5444774267305,35.8657382843932,46.4470235952228));
#25815=CARTESIAN_POINT('Ctrl Pts',(43.5482273623742,35.8654299996637,46.4497941363977));
#25816=CARTESIAN_POINT('Ctrl Pts',(43.5561336524867,35.8647803051973,46.4556799187319));
#25817=CARTESIAN_POINT('Ctrl Pts',(43.560287539906,35.8644391347943,46.4587984032688));
#25818=CARTESIAN_POINT('Ctrl Pts',(43.5705879124514,35.8635934273743,46.4665965394425));
#25819=CARTESIAN_POINT('Ctrl Pts',(43.5767190602598,35.8630902914826,46.4712964669936));
#25820=CARTESIAN_POINT('Ctrl Pts',(43.5998868653791,35.8611893685858,46.4892780844755));
#25821=CARTESIAN_POINT('Ctrl Pts',(43.6167289914218,35.8598080454703,46.5028093468635));
#25822=CARTESIAN_POINT('Ctrl Pts',(43.659523046865,35.8562892674483,46.5383900580429));
#25823=CARTESIAN_POINT('Ctrl Pts',(43.6851256357352,35.8541752557778,46.5608494513904));
#25824=CARTESIAN_POINT('Ctrl Pts',(43.7640530244159,35.8475803960898,46.6338739839171));
#25825=CARTESIAN_POINT('Ctrl Pts',(43.8150927130189,35.8431965802839,46.6868150365677));
#25826=CARTESIAN_POINT('Ctrl Pts',(43.9515701068735,35.8307077584285,46.8455996379022));
#25827=CARTESIAN_POINT('Ctrl Pts',(44.0290021969505,35.8226131942831,46.9577157924064));
#25828=CARTESIAN_POINT('Ctrl Pts',(44.1060999263628,35.8124518070186,47.0992202502094));
#25829=CARTESIAN_POINT('Ctrl Pts',(44.1177522934067,35.8108442477041,47.121644673214));
#25830=CARTESIAN_POINT('Ctrl Pts',(44.1340868762421,35.8084789273793,47.1546486936775));
#25831=CARTESIAN_POINT('Ctrl Pts',(44.1391200498942,35.8077334244621,47.1650523561697));
#25832=CARTESIAN_POINT('Ctrl Pts',(44.1478847548956,35.8064047692532,47.1835922879146));
#25833=CARTESIAN_POINT('Ctrl Pts',(44.151653742113,35.805822936036,47.1917105518709));
#25834=CARTESIAN_POINT('Ctrl Pts',(44.159397203458,35.8046052028596,47.2086982265415));
#25835=CARTESIAN_POINT('Ctrl Pts',(44.1633614081801,35.8039689691548,47.2175720132274));
#25836=CARTESIAN_POINT('Ctrl Pts',(44.1735338007928,35.8023021150283,47.2408126986027));
#25837=CARTESIAN_POINT('Ctrl Pts',(44.1796344003739,35.801267860115,47.255225619736));
#25838=CARTESIAN_POINT('Ctrl Pts',(44.2067286928707,35.7965105598589,47.3214712301686));
#25839=CARTESIAN_POINT('Ctrl Pts',(44.2256358791604,35.792718398557,47.3741226822582));
#25840=CARTESIAN_POINT('Ctrl Pts',(44.2743292114223,35.7813950574353,47.5308158564398));
#25841=CARTESIAN_POINT('Ctrl Pts',(44.2976815220094,35.7736898371534,47.6366216758149));
#25842=CARTESIAN_POINT('Ctrl Pts',(44.3255694417088,35.7586877520378,47.8447628892218));
#25843=CARTESIAN_POINT('Ctrl Pts',(44.3310806472305,35.7514197856597,47.9466348595874));
#25844=CARTESIAN_POINT('Ctrl Pts',(44.3281053434859,35.7433574317197,48.0650064486664));
#25845=CARTESIAN_POINT('Ctrl Pts',(44.3274772022601,35.7422406665573,48.0815336351079));
#25846=CARTESIAN_POINT('Ctrl Pts',(44.3263078909733,35.7407023889753,48.1045097348343));
#25847=CARTESIAN_POINT('Ctrl Pts',(44.3259467303238,35.7402716663708,48.1109665283876));
#25848=CARTESIAN_POINT('Ctrl Pts',(44.3252683415991,35.7395324003787,48.1220911822459));
#25849=CARTESIAN_POINT('Ctrl Pts',(44.324966591475,35.7392230151275,48.1267598786032));
#25850=CARTESIAN_POINT('Ctrl Pts',(44.3242952234058,35.7385733765292,48.1365915133954));
#25851=CARTESIAN_POINT('Ctrl Pts',(44.3239218052795,35.7382333492813,48.1417541413393));
#25852=CARTESIAN_POINT('Ctrl Pts',(44.3229459950402,35.7373944653599,48.1545301998701));
#25853=CARTESIAN_POINT('Ctrl Pts',(44.3223191543518,35.7368969605862,48.1621417779022));
#25854=CARTESIAN_POINT('Ctrl Pts',(44.3198023000726,35.7350425317222,48.1906337806709));
#25855=CARTESIAN_POINT('Ctrl Pts',(44.3176170663376,35.7337010525619,48.2114875494207));
#25856=CARTESIAN_POINT('Ctrl Pts',(44.2980550952698,35.7234208661009,48.3727555854374));
#25857=CARTESIAN_POINT('Ctrl Pts',(44.2656163398082,35.7151418460771,48.5109269395549));
#25858=CARTESIAN_POINT('Ctrl Pts',(44.1806386617376,35.6999187395425,48.7507439527265));
#25859=CARTESIAN_POINT('Ctrl Pts',(44.1336637610375,35.6930747396447,48.8536366432757));
#25860=CARTESIAN_POINT('Ctrl Pts',(44.0695340042166,35.6848191184534,48.9666906860437));
#25861=CARTESIAN_POINT('Ctrl Pts',(44.0609042017732,35.6837268516629,48.9814437713339));
#25862=CARTESIAN_POINT('Ctrl Pts',(44.0463888459172,35.6819185960345,49.0055186731209));
#25863=CARTESIAN_POINT('Ctrl Pts',(44.040617275999,35.6812067590532,49.0149083600578));
#25864=CARTESIAN_POINT('Ctrl Pts',(44.030057571624,35.6799168475957,49.0317623285321));
#25865=CARTESIAN_POINT('Ctrl Pts',(44.0252977953554,35.6793398339539,49.0392440817163));
#25866=CARTESIAN_POINT('Ctrl Pts',(44.0149887796606,35.6780993117596,49.0552044713717));
#25867=CARTESIAN_POINT('Ctrl Pts',(44.0094239996943,35.6774352334189,49.0636727021876));
#25868=CARTESIAN_POINT('Ctrl Pts',(43.9940386556873,35.6756139639149,49.0866882640076));
#25869=CARTESIAN_POINT('Ctrl Pts',(43.9840860617096,35.6744518118159,49.1011457366162));
#25870=CARTESIAN_POINT('Ctrl Pts',(43.9254614808539,35.6676949988011,49.1838659003381));
#25871=CARTESIAN_POINT('Ctrl Pts',(43.8725847103486,35.6619383982858,49.2490244175262));
#25872=CARTESIAN_POINT('Ctrl Pts',(43.7402008631107,35.6482660365202,49.3920264201861));
#25873=CARTESIAN_POINT('Ctrl Pts',(43.6578626556174,35.6402746536078,49.4668519994474));
#25874=CARTESIAN_POINT('Ctrl Pts',(43.509472614925,35.6270165480556,49.579974857547));
#25875=CARTESIAN_POINT('Ctrl Pts',(43.4467459490937,35.6217111008548,49.622213174375));
#25876=CARTESIAN_POINT('Ctrl Pts',(43.3727258784532,35.6159057663049,49.6659698428098));
#25877=CARTESIAN_POINT('Ctrl Pts',(43.3637121254195,35.6152062067954,49.671200198315));
#25878=CARTESIAN_POINT('Ctrl Pts',(43.3490881131025,35.6140836415366,49.6795283173277));
#25879=CARTESIAN_POINT('Ctrl Pts',(43.343504171802,35.6136578995824,49.6826715353452));
#25880=CARTESIAN_POINT('Ctrl Pts',(43.3335504885774,35.6129042573395,49.6882093674803));
#25881=CARTESIAN_POINT('Ctrl Pts',(43.3291870242795,35.6125756722893,49.6906149351736));
#25882=CARTESIAN_POINT('Ctrl Pts',(43.3196705225722,35.6118629593536,49.6958133853857));
#25883=CARTESIAN_POINT('Ctrl Pts',(43.3145140552627,35.6114792455463,49.6985997036153));
#25884=CARTESIAN_POINT('Ctrl Pts',(43.2998373278348,35.6103938436981,49.7064441264416));
#25885=CARTESIAN_POINT('Ctrl Pts',(43.2902870760184,35.609695591704,49.7114460869402));
#25886=CARTESIAN_POINT('Ctrl Pts',(43.2247278569441,35.6049534876024,49.7450855450891));
#25887=CARTESIAN_POINT('Ctrl Pts',(43.1673829522442,35.6010588212352,49.7710518822208));
#25888=CARTESIAN_POINT('Ctrl Pts',(42.9901470169952,35.589472670939,49.8410766492329));
#25889=CARTESIAN_POINT('Ctrl Pts',(42.8670642537494,35.5820080623583,49.87608368658));
#25890=CARTESIAN_POINT('Ctrl Pts',(42.6623813635971,35.5694203850802,49.9128899579544));
#25891=CARTESIAN_POINT('Ctrl Pts',(42.5825392710102,35.564473379798,49.9221521976864));
#25892=CARTESIAN_POINT('Ctrl Pts',(42.4845441131643,35.5582328768642,49.9273590998363));
#25893=CARTESIAN_POINT('Ctrl Pts',(42.4667179102826,35.5570911111399,49.9280584775813));
#25894=CARTESIAN_POINT('Ctrl Pts',(42.4385884009676,35.5552779361556,49.9287715212269));
#25895=CARTESIAN_POINT('Ctrl Pts',(42.4282900071768,35.5546116976225,49.9289500549391));
#25896=CARTESIAN_POINT('Ctrl Pts',(42.4091374495548,35.5533679297623,49.929128677219));
#25897=CARTESIAN_POINT('Ctrl Pts',(42.4002837218606,35.5527910919753,49.9291502951684));
#25898=CARTESIAN_POINT('Ctrl Pts',(42.3806281957251,35.5515061874931,49.9290629791344));
#25899=CARTESIAN_POINT('Ctrl Pts',(42.3698268949531,35.5507972044922,49.9289242649511));
#25900=CARTESIAN_POINT('Ctrl Pts',(42.3383070151142,35.5487195603028,49.9282546681654));
#25901=CARTESIAN_POINT('Ctrl Pts',(42.3175956792675,35.5473433464123,49.9274806251665));
#25902=CARTESIAN_POINT('Ctrl Pts',(42.2706210967749,35.5441958828675,49.9249665696704));
#25903=CARTESIAN_POINT('Ctrl Pts',(42.2443733704894,35.5424185919533,49.9230224733435));
#25904=CARTESIAN_POINT('Ctrl Pts',(42.1568846838623,35.5364311704053,49.9147395729691));
#25905=CARTESIAN_POINT('Ctrl Pts',(42.0959131381018,35.5321529878954,49.9060069846049));
#25906=CARTESIAN_POINT('Ctrl Pts',(41.9536932002289,35.5219496391987,49.8786398142167));
#25907=CARTESIAN_POINT('Ctrl Pts',(41.8730838033419,35.5159882853997,49.8576372761027));
#25908=CARTESIAN_POINT('Ctrl Pts',(41.7941383590443,35.5100558711261,49.8315223801304));
#25909=CARTESIAN_POINT('Origin',(42.4,48.4493818343519,48.));
#25910=CARTESIAN_POINT('',(41.7941388327286,34.5440062296316,49.8315225368236));
#25911=CARTESIAN_POINT('',(41.7941388232987,34.7154586800303,49.8315225337042));
#25912=CARTESIAN_POINT('',(41.7941388317924,48.4493818343519,49.8315225365138));
#25913=CARTESIAN_POINT('',(40.4708707108034,35.1798577040826,48.000956906968));
#25914=CARTESIAN_POINT('Ctrl Pts',(41.7941388327286,34.5440062296316,49.8315225368236));
#25915=CARTESIAN_POINT('Ctrl Pts',(41.8146287093069,34.5454435391173,49.8383005154132));
#25916=CARTESIAN_POINT('Ctrl Pts',(41.835230775212,34.5468920470605,49.8447341404695));
#25917=CARTESIAN_POINT('Ctrl Pts',(41.9672793190937,34.5561994466028,49.8835508693276));
#25918=CARTESIAN_POINT('Ctrl Pts',(42.0813312735382,34.5643645427599,49.9061619822515));
#25919=CARTESIAN_POINT('Ctrl Pts',(42.3230981793342,34.5817048271349,49.9317823813768));
#25920=CARTESIAN_POINT('Ctrl Pts',(42.4505144809719,34.5908603568565,49.9326537421973));
#25921=CARTESIAN_POINT('Ctrl Pts',(42.5926065073978,34.600562613785,49.9195540731544));
#25922=CARTESIAN_POINT('Ctrl Pts',(42.6080974763127,34.6016131908161,49.9179365434389));
#25923=CARTESIAN_POINT('Ctrl Pts',(42.6298299468512,34.6030754112146,49.9154008722497));
#25924=CARTESIAN_POINT('Ctrl Pts',(42.6360886351394,34.6034951522501,49.9146395130674));
#25925=CARTESIAN_POINT('Ctrl Pts',(42.6474027119971,34.6042513355798,49.9132068524194));
#25926=CARTESIAN_POINT('Ctrl Pts',(42.6524593771967,34.6045883598486,49.9125461633796));
#25927=CARTESIAN_POINT('Ctrl Pts',(42.6628057918334,34.6052759366926,49.9111525814178));
#25928=CARTESIAN_POINT('Ctrl Pts',(42.6680952091926,34.6056263793087,49.9104177643177));
#25929=CARTESIAN_POINT('Ctrl Pts',(42.6816948079461,34.6065248086319,49.9084708847781));
#25930=CARTESIAN_POINT('Ctrl Pts',(42.6900003555086,34.6070710041341,49.9072264896981));
#25931=CARTESIAN_POINT('Ctrl Pts',(42.7250194690417,34.6093644351759,49.9017456312102));
#25932=CARTESIAN_POINT('Ctrl Pts',(42.7516519727824,34.611085205183,49.89700162607));
#25933=CARTESIAN_POINT('Ctrl Pts',(42.8242197198431,34.615731450677,49.882494301995));
#25934=CARTESIAN_POINT('Ctrl Pts',(42.8699138399239,34.6186102778029,49.8716112728415));
#25935=CARTESIAN_POINT('Ctrl Pts',(43.0535027705824,34.63014880764,49.8207368408108));
#25936=CARTESIAN_POINT('Ctrl Pts',(43.1871248014931,34.6385165746292,49.7670836490106));
#25937=CARTESIAN_POINT('Ctrl Pts',(43.3666926883881,34.6509975308675,49.6705349140436));
#25938=CARTESIAN_POINT('Ctrl Pts',(43.4184506412074,34.6547518753377,49.6394934714114));
#25939=CARTESIAN_POINT('Ctrl Pts',(43.4825409500819,34.6596564275427,49.5968485823097));
#25940=CARTESIAN_POINT('Ctrl Pts',(43.4962952787383,34.6607246403997,49.5874372230593));
#25941=CARTESIAN_POINT('Ctrl Pts',(43.5180575197084,34.6624409074155,49.5721287446336));
#25942=CARTESIAN_POINT('Ctrl Pts',(43.5261449589909,34.6630845948328,49.5663457256502));
#25943=CARTESIAN_POINT('Ctrl Pts',(43.5413853743694,34.6643089862316,49.5552688411638));
#25944=CARTESIAN_POINT('Ctrl Pts',(43.5485471498627,34.6648891946331,49.5499874777499));
#25945=CARTESIAN_POINT('Ctrl Pts',(43.5647421955796,34.6662124380743,49.5378707661184));
#25946=CARTESIAN_POINT('Ctrl Pts',(43.5737522450526,34.6669566526071,49.5310050729344));
#25947=CARTESIAN_POINT('Ctrl Pts',(43.6011611657212,34.66924568802,49.5097352081183));
#25948=CARTESIAN_POINT('Ctrl Pts',(43.6193586628681,34.6708005851701,49.4950762234985));
#25949=CARTESIAN_POINT('Ctrl Pts',(43.7062350914774,34.6783996728495,49.4224517086445));
#25950=CARTESIAN_POINT('Ctrl Pts',(43.7710637003188,34.6846227879505,49.3600732441528));
#25951=CARTESIAN_POINT('Ctrl Pts',(43.9299984607576,34.701363813366,49.1841945611365));
#25952=CARTESIAN_POINT('Ctrl Pts',(44.0158667269027,34.7120617658262,49.0640425893564));
#25953=CARTESIAN_POINT('Ctrl Pts',(44.1010605963668,34.724196908709,48.9103562469663));
#25954=CARTESIAN_POINT('Ctrl Pts',(44.1143316096657,34.7261431175128,48.8851118518895));
#25955=CARTESIAN_POINT('Ctrl Pts',(44.1309961406682,34.7286546009758,48.8516300806256));
#25956=CARTESIAN_POINT('Ctrl Pts',(44.1348985799097,34.7292479495889,48.8436517991411));
#25957=CARTESIAN_POINT('Ctrl Pts',(44.1411052651546,34.7301998493542,48.8307374313458));
#25958=CARTESIAN_POINT('Ctrl Pts',(44.143443891996,34.730560456305,48.8258181527966));
#25959=CARTESIAN_POINT('Ctrl Pts',(44.1479303311284,34.7312559399559,48.8162769676413));
#25960=CARTESIAN_POINT('Ctrl Pts',(44.1500806937478,34.7315909619938,48.8116563905705));
#25961=CARTESIAN_POINT('Ctrl Pts',(44.1552327396933,34.7323978372744,48.8004702999377));
#25962=CARTESIAN_POINT('Ctrl Pts',(44.1582159681456,34.7328685669796,48.7938962684301));
#25963=CARTESIAN_POINT('Ctrl Pts',(44.168564436003,34.7345145203125,48.7707472736971));
#25964=CARTESIAN_POINT('Ctrl Pts',(44.1757330303006,34.7356784473682,48.7540847345965));
#25965=CARTESIAN_POINT('Ctrl Pts',(44.1929153853969,34.7385350098019,48.7125420129986));
#25966=CARTESIAN_POINT('Ctrl Pts',(44.2026476083617,34.7402138716442,48.6875488684417));
#25967=CARTESIAN_POINT('Ctrl Pts',(44.2423281036799,34.7473685102786,48.5790046056423));
#25968=CARTESIAN_POINT('Ctrl Pts',(44.2670140746638,34.752654504719,48.4936395543732));
#25969=CARTESIAN_POINT('Ctrl Pts',(44.3136383257669,34.765839146129,48.2775497515533));
#25970=CARTESIAN_POINT('Ctrl Pts',(44.3281615562322,34.7737332214481,48.1457160683761));
#25971=CARTESIAN_POINT('Ctrl Pts',(44.3292600608276,34.7836740217639,47.9880535280753));
#25972=CARTESIAN_POINT('Ctrl Pts',(44.328935767948,34.7852889497652,47.9626662677429));
#25973=CARTESIAN_POINT('Ctrl Pts',(44.3277341735545,34.7876632483594,47.9257193055318));
#25974=CARTESIAN_POINT('Ctrl Pts',(44.3272535423683,34.7884102291815,47.914148737586));
#25975=CARTESIAN_POINT('Ctrl Pts',(44.3262165100452,34.7897407221687,47.8936387028876));
#25976=CARTESIAN_POINT('Ctrl Pts',(44.3257019688389,34.7903229045364,47.8846973904783));
#25977=CARTESIAN_POINT('Ctrl Pts',(44.3244996747751,34.7915405621749,47.8660675720539));
#25978=CARTESIAN_POINT('Ctrl Pts',(44.3238009766147,34.7921763657448,47.8563800501922));
#25979=CARTESIAN_POINT('Ctrl Pts',(44.3217884363655,34.7938402923106,47.831134568534));
#25980=CARTESIAN_POINT('Ctrl Pts',(44.3203588414175,34.7948720243876,47.8155868123115));
#25981=CARTESIAN_POINT('Ctrl Pts',(44.3129911160381,34.799596831881,47.7448823566654));
#25982=CARTESIAN_POINT('Ctrl Pts',(44.3048647643674,34.8033578560222,47.689985168909));
#25983=CARTESIAN_POINT('Ctrl Pts',(44.2742463006614,34.8145378656633,47.5308462042116));
#25984=CARTESIAN_POINT('Ctrl Pts',(44.2454685454515,34.8221252419197,47.4280334946921));
#25985=CARTESIAN_POINT('Ctrl Pts',(44.1721060353499,34.8371737681846,47.2305752110992));
#25986=CARTESIAN_POINT('Ctrl Pts',(44.1280200981106,34.8446068017118,47.1360989317836));
#25987=CARTESIAN_POINT('Ctrl Pts',(44.0683827459427,34.8528138956646,47.0313347922527));
#25988=CARTESIAN_POINT('Ctrl Pts',(44.0600600875846,34.8539248652839,47.0171399786565));
#25989=CARTESIAN_POINT('Ctrl Pts',(44.0482214396729,34.8554565479837,46.9975279106373));
#25990=CARTESIAN_POINT('Ctrl Pts',(44.0448586166162,34.8558863708531,46.9920196735845));
#25991=CARTESIAN_POINT('Ctrl Pts',(44.0390116847532,34.8566245687974,46.9825496976155));
#25992=CARTESIAN_POINT('Ctrl Pts',(44.0365407230539,34.8569337796565,46.9785799671355));
#25993=CARTESIAN_POINT('Ctrl Pts',(44.0313010219741,34.8575836193096,46.9702299361213));
#25994=CARTESIAN_POINT('Ctrl Pts',(44.0285290240318,34.8579240186846,46.9658517380292));
#25995=CARTESIAN_POINT('Ctrl Pts',(44.0216155114455,34.8587647820698,46.955029008799));
#25996=CARTESIAN_POINT('Ctrl Pts',(44.0174531324553,34.8592637816368,46.9485977893396));
#25997=CARTESIAN_POINT('Ctrl Pts',(44.0016700040355,34.8611298153396,46.9245271106344));
#25998=CARTESIAN_POINT('Ctrl Pts',(43.9897976183614,34.8624811563245,46.9070533594576));
#25999=CARTESIAN_POINT('Ctrl Pts',(43.8945879819627,34.8729480400896,46.7717593033089));
#26000=CARTESIAN_POINT('Ctrl Pts',(43.798544494788,34.8813789900665,46.663417414426));
#26001=CARTESIAN_POINT('Ctrl Pts',(43.6096183868487,34.8966051438272,46.4931972528051));
#26002=CARTESIAN_POINT('Ctrl Pts',(43.5218038554396,34.9032796625362,46.4267287112272));
#26003=CARTESIAN_POINT('Ctrl Pts',(43.4143897058633,34.9113453271464,46.3590104055715));
#26004=CARTESIAN_POINT('Ctrl Pts',(43.3998455492641,34.9124351143861,46.3501084362172));
#26005=CARTESIAN_POINT('Ctrl Pts',(43.3757184565577,34.914240216041,46.3357772682404));
#26006=CARTESIAN_POINT('Ctrl Pts',(43.3662034459825,34.914951405667,46.3302351363042));
#26007=CARTESIAN_POINT('Ctrl Pts',(43.3489398915821,34.9162407794639,46.3203767386885));
#26008=CARTESIAN_POINT('Ctrl Pts',(43.3412079839978,34.9168179090004,46.3160318458434));
#26009=CARTESIAN_POINT('Ctrl Pts',(43.3245676235295,34.9180593872843,46.3068313135474));
#26010=CARTESIAN_POINT('Ctrl Pts',(43.3156503077847,34.9187243113538,46.3019923444137));
#26011=CARTESIAN_POINT('Ctrl Pts',(43.2911590916462,34.9205497484386,46.2889512440294));
#26012=CARTESIAN_POINT('Ctrl Pts',(43.2755107668893,34.9217152585066,46.2808917329298));
#26013=CARTESIAN_POINT('Ctrl Pts',(43.1838649163437,34.9285383163638,46.2352662931577));
#26014=CARTESIAN_POINT('Ctrl Pts',(43.1055780297647,34.9343616236151,46.2025336385534));
#26015=CARTESIAN_POINT('Ctrl Pts',(42.9162923775565,34.9484067728668,46.1376660373835));
#26016=CARTESIAN_POINT('Ctrl Pts',(42.8040520637093,34.9567167124944,46.1101363008273));
#26017=CARTESIAN_POINT('Ctrl Pts',(42.6546459115141,34.9674361954427,46.0874155089848));
#26018=CARTESIAN_POINT('Ctrl Pts',(42.6191112912591,34.9699592329286,46.0830194450237));
#26019=CARTESIAN_POINT('Ctrl Pts',(42.5460978498607,34.97506576778,46.0760437476119));
#26020=CARTESIAN_POINT('Ctrl Pts',(42.508622916386,34.9776451999554,46.0735644960774));
#26021=CARTESIAN_POINT('Ctrl Pts',(42.4613351979706,34.9808289455994,46.0718205563258));
#26022=CARTESIAN_POINT('Ctrl Pts',(42.451570841787,34.9814825307748,46.0715346952266));
#26023=CARTESIAN_POINT('Ctrl Pts',(42.4361631572987,34.9825073913876,46.0712007303808));
#26024=CARTESIAN_POINT('Ctrl Pts',(42.4305212298557,34.9828813037757,46.0711032031259));
#26025=CARTESIAN_POINT('Ctrl Pts',(42.4198555492208,34.9835854728689,46.0709656426138));
#26026=CARTESIAN_POINT('Ctrl Pts',(42.4148321090907,34.9839159907461,46.0709204775525));
#26027=CARTESIAN_POINT('Ctrl Pts',(42.4030411243004,34.9846891879588,46.0708605272238));
#26028=CARTESIAN_POINT('Ctrl Pts',(42.3962736067944,34.9851309746168,46.0708617283214));
#26029=CARTESIAN_POINT('Ctrl Pts',(42.3740822399987,34.9865735058102,46.0709824444975));
#26030=CARTESIAN_POINT('Ctrl Pts',(42.3586593402792,34.9875663461566,46.0712513264068));
#26031=CARTESIAN_POINT('Ctrl Pts',(42.2729735814096,34.9930365788061,46.0737734822425));
#26032=CARTESIAN_POINT('Ctrl Pts',(42.2028639518154,34.9973423091948,46.0796813146554));
#26033=CARTESIAN_POINT('Ctrl Pts',(42.0989437653756,35.0036721499642,46.0941915309639));
#26034=CARTESIAN_POINT('Ctrl Pts',(42.0647954063096,35.0057434285244,46.0999003319764));
#26035=CARTESIAN_POINT('Ctrl Pts',(41.8856022494722,35.0166439346524,46.1348386251313));
#26036=CARTESIAN_POINT('Ctrl Pts',(41.7441426418191,35.0254054379438,46.1797589456742));
#26037=CARTESIAN_POINT('Ctrl Pts',(41.586741495243,35.0362944427867,46.2504972118644));
#26038=CARTESIAN_POINT('Ctrl Pts',(41.564468449651,35.0378623323715,46.2610243412815));
#26039=CARTESIAN_POINT('Ctrl Pts',(41.5321533793324,35.0401800885492,46.2770618839465));
#26040=CARTESIAN_POINT('Ctrl Pts',(41.5219485488789,35.0409184008936,46.2822400782885));
#26041=CARTESIAN_POINT('Ctrl Pts',(41.5040849495459,35.0422223909537,46.2915053032089));
#26042=CARTESIAN_POINT('Ctrl Pts',(41.4964064996441,35.0427866984068,46.2955538469719));
#26043=CARTESIAN_POINT('Ctrl Pts',(41.4881122493073,35.0434004687712,46.2999988764588));
#26044=CARTESIAN_POINT('Ctrl Pts',(41.4874689564455,35.043448099662,46.3003440982211));
#26045=CARTESIAN_POINT('Ctrl Pts',(41.478288531475,35.0441282333387,46.3052774683052));
#26046=CARTESIAN_POINT('Ctrl Pts',(41.4697860325811,35.0447630067461,46.3099294512836));
#26047=CARTESIAN_POINT('Ctrl Pts',(41.4524129202297,35.0460702103982,46.3196056390169));
#26048=CARTESIAN_POINT('Ctrl Pts',(41.4435463705405,35.0467428649969,46.3246364782388));
#26049=CARTESIAN_POINT('Ctrl Pts',(41.4215962689952,35.0484220343456,46.337321900789));
#26050=CARTESIAN_POINT('Ctrl Pts',(41.408562463227,35.0494315664336,46.3450607531512));
#26051=CARTESIAN_POINT('Ctrl Pts',(41.3720933263432,35.0522920930632,46.3672998263619));
#26052=CARTESIAN_POINT('Ctrl Pts',(41.3488763433923,35.0541555211183,46.3821492915892));
#26053=CARTESIAN_POINT('Ctrl Pts',(41.2711288938089,35.0605426066289,46.4342561984722));
#26054=CARTESIAN_POINT('Ctrl Pts',(41.2182006495391,35.0651447501022,46.473811143081));
#26055=CARTESIAN_POINT('Ctrl Pts',(41.0586929126367,35.079792566348,46.6062960609028));
#26056=CARTESIAN_POINT('Ctrl Pts',(40.9602319003895,35.0900495046597,46.7082636237771));
#26057=CARTESIAN_POINT('Ctrl Pts',(40.853772554026,35.1021180941536,46.8459659331852));
#26058=CARTESIAN_POINT('Ctrl Pts',(40.8344132325379,35.1043592485135,46.8723687117982));
#26059=CARTESIAN_POINT('Ctrl Pts',(40.8104074911616,35.1071872937489,46.9069193289909));
#26060=CARTESIAN_POINT('Ctrl Pts',(40.8051366416773,35.1078114444317,46.9146242243038));
#26061=CARTESIAN_POINT('Ctrl Pts',(40.7968230835735,35.1088006802971,46.9269682657223));
#26062=CARTESIAN_POINT('Ctrl Pts',(40.7937441786555,35.1091681114713,46.9315826815033));
#26063=CARTESIAN_POINT('Ctrl Pts',(40.7878985430584,35.1098676794292,46.9404260354128));
#26064=CARTESIAN_POINT('Ctrl Pts',(40.7851284937373,35.1102000255627,46.9446526104218));
#26065=CARTESIAN_POINT('Ctrl Pts',(40.7785790708313,35.1109879341656,46.9547319652195));
#26066=CARTESIAN_POINT('Ctrl Pts',(40.7748146925348,35.1114425062394,46.9605944900198));
#26067=CARTESIAN_POINT('Ctrl Pts',(40.762197250136,35.1129724329873,46.9804806325943));
#26068=CARTESIAN_POINT('Ctrl Pts',(40.7534929940613,35.1140385036843,46.994598432447));
#26069=CARTESIAN_POINT('Ctrl Pts',(40.7029142705954,35.1203086426507,47.0790531662067));
#26070=CARTESIAN_POINT('Ctrl Pts',(40.6653642216589,35.1252815775282,47.1518933474097));
#26071=CARTESIAN_POINT('Ctrl Pts',(40.5779738226526,35.1383676459323,47.3516854730591));
#26072=CARTESIAN_POINT('Ctrl Pts',(40.5367643163965,35.1463626087072,47.4818856220333));
#26073=CARTESIAN_POINT('Ctrl Pts',(40.4998866399512,35.1577774497081,47.6631184298773));
#26074=CARTESIAN_POINT('Ctrl Pts',(40.4919799584223,35.1608313585747,47.7112459894529));
#26075=CARTESIAN_POINT('Ctrl Pts',(40.4839777704355,35.164929856896,47.7749653076872));
#26076=CARTESIAN_POINT('Ctrl Pts',(40.4822351270031,35.1659225519383,47.7903343941973));
#26077=CARTESIAN_POINT('Ctrl Pts',(40.4797025763691,35.1675460408309,47.8153541692377));
#26078=CARTESIAN_POINT('Ctrl Pts',(40.4788001633346,35.1681732774932,47.824992971788));
#26079=CARTESIAN_POINT('Ctrl Pts',(40.4772376416884,35.1693586662352,47.8431544187014));
#26080=CARTESIAN_POINT('Ctrl Pts',(40.4765615538733,35.16991629992,47.8516754811227));
#26081=CARTESIAN_POINT('Ctrl Pts',(40.4753116091618,35.1710451685827,47.8688784638694));
#26082=CARTESIAN_POINT('Ctrl Pts',(40.4747398144819,35.1716164550315,47.877560329559));
#26083=CARTESIAN_POINT('Ctrl Pts',(40.4732507108879,35.1732800145079,47.9027697016922));
#26084=CARTESIAN_POINT('Ctrl Pts',(40.4724873877035,35.1743770835538,47.9193051782206));
#26085=CARTESIAN_POINT('Ctrl Pts',(40.4712150432388,35.176928393239,47.9575449889482));
#26086=CARTESIAN_POINT('Ctrl Pts',(40.4708594482203,35.1783872376127,47.9792516976681));
#26087=CARTESIAN_POINT('Ctrl Pts',(40.4708702383276,35.1798570188309,48.0009589212152));
#26088=CARTESIAN_POINT('Ctrl Pts',(40.470870237355,35.1798568862125,48.000956962571));
#26089=CARTESIAN_POINT('Ctrl Pts',(40.4709100302208,35.1852883880148,48.081174939798));
#26090=CARTESIAN_POINT('Ctrl Pts',(40.4759531835995,35.1908675616307,48.1613049946017));
#26091=CARTESIAN_POINT('Ctrl Pts',(40.5061098364464,35.2079432831597,48.4009270850374));
#26092=CARTESIAN_POINT('Ctrl Pts',(40.5462442780223,35.219701532293,48.557812136919));
#26093=CARTESIAN_POINT('Ctrl Pts',(40.6112379328665,35.2317426179312,48.7225806417626));
#26094=CARTESIAN_POINT('Ctrl Pts',(40.6172200976197,35.2328087880833,48.7372166411818));
#26095=CARTESIAN_POINT('Ctrl Pts',(40.6260452844213,35.2343214721451,48.7580725157763));
#26096=CARTESIAN_POINT('Ctrl Pts',(40.6287422958384,35.2347761307598,48.7643529427421));
#26097=CARTESIAN_POINT('Ctrl Pts',(40.6334832510485,35.2355621137002,48.7752331683621));
#26098=CARTESIAN_POINT('Ctrl Pts',(40.6355119016407,35.2358943464401,48.7798394981041));
#26099=CARTESIAN_POINT('Ctrl Pts',(40.6398392070688,35.2365944103947,48.7895619009939));
#26100=CARTESIAN_POINT('Ctrl Pts',(40.642142160466,35.2369619764881,48.7946759279418));
#26101=CARTESIAN_POINT('Ctrl Pts',(40.648452757878,35.2379559383835,48.8085278127995));
#26102=CARTESIAN_POINT('Ctrl Pts',(40.6525035270755,35.2385797579921,48.8172460167642));
#26103=CARTESIAN_POINT('Ctrl Pts',(40.6719347363676,35.2415078838264,48.8582614026467));
#26104=CARTESIAN_POINT('Ctrl Pts',(40.6881474603223,35.2437654796842,48.8901592315938));
#26105=CARTESIAN_POINT('Ctrl Pts',(40.7174590431839,35.2475778805207,48.9440618604684));
#26106=CARTESIAN_POINT('Ctrl Pts',(40.7301251654887,35.2491491837437,48.9662892948409));
#26107=CARTESIAN_POINT('Ctrl Pts',(40.8197978511772,35.2598156051154,49.1166213496377));
#26108=CARTESIAN_POINT('Ctrl Pts',(40.91102378168,35.268499514009,49.2356518021253));
#26109=CARTESIAN_POINT('Ctrl Pts',(41.045113969837,35.2802627543142,49.3739314389018));
#26110=CARTESIAN_POINT('Ctrl Pts',(41.0761756782416,35.2829275312723,49.403884803761));
#26111=CARTESIAN_POINT('Ctrl Pts',(41.123579819503,35.2869317443521,49.4466243903317));
#26112=CARTESIAN_POINT('Ctrl Pts',(41.1391672204477,35.2882389050776,49.4602298639794));
#26113=CARTESIAN_POINT('Ctrl Pts',(41.1644879576153,35.2903494662493,49.4816233703533));
#26114=CARTESIAN_POINT('Ctrl Pts',(41.1740834410048,35.2911464072972,49.4895725551921));
#26115=CARTESIAN_POINT('Ctrl Pts',(41.1923829451665,35.2926613327077,49.504435825919));
#26116=CARTESIAN_POINT('Ctrl Pts',(41.2010710606666,35.2933785263995,49.5113687489618));
#26117=CARTESIAN_POINT('Ctrl Pts',(41.2165872589449,35.2946560276261,49.5235323476396));
#26118=CARTESIAN_POINT('Ctrl Pts',(41.2233913778625,35.2952151126472,49.528793209131));
#26119=CARTESIAN_POINT('Ctrl Pts',(41.2369778324198,35.2963294001881,49.5391536627439));
#26120=CARTESIAN_POINT('Ctrl Pts',(41.2437590889536,35.2968845420465,49.5442543545477));
#26121=CARTESIAN_POINT('Ctrl Pts',(41.2620506463989,35.298379379519,49.557824780394));
#26122=CARTESIAN_POINT('Ctrl Pts',(41.2736215933389,35.2993222743936,49.5662114940219));
#26123=CARTESIAN_POINT('Ctrl Pts',(41.3173614785961,35.3028771979908,49.5971791043714));
#26124=CARTESIAN_POINT('Ctrl Pts',(41.3501229381969,35.3055213910521,49.6189024155884));
#26125=CARTESIAN_POINT('Ctrl Pts',(41.5090293379316,35.3182688100887,49.7174165848119));
#26126=CARTESIAN_POINT('Ctrl Pts',(41.6430385116812,35.3288445252337,49.7805461196931));
#26127=CARTESIAN_POINT('Ctrl Pts',(41.7866459223646,35.3396514468648,49.8290311424881));
#26128=CARTESIAN_POINT('Ctrl Pts',(41.7903904758723,35.3399328460002,49.8302825936515));
#26129=CARTESIAN_POINT('Ctrl Pts',(41.7941388318214,35.3402141276758,49.8315225365234));
#26130=CARTESIAN_POINT('',(40.4708702390927,35.3509292085261,48.0009604591324));
#26131=CARTESIAN_POINT('Ctrl Pts',(41.7941383590443,35.5100558711261,49.8315223801304));
#26132=CARTESIAN_POINT('Ctrl Pts',(41.7402688807148,35.5060078090118,49.8137025320672));
#26133=CARTESIAN_POINT('Ctrl Pts',(41.6871740605304,35.5019746911376,49.7935022709993));
#26134=CARTESIAN_POINT('Ctrl Pts',(41.5985161358713,35.4952389641539,49.755205567771));
#26135=CARTESIAN_POINT('Ctrl Pts',(41.5625139060136,35.4925036623722,49.738315429417));
#26136=CARTESIAN_POINT('Ctrl Pts',(41.5182730832123,35.4891644365375,49.7158663167832));
#26137=CARTESIAN_POINT('Ctrl Pts',(41.5095235635153,35.4885051449714,49.7113419585414));
#26138=CARTESIAN_POINT('Ctrl Pts',(41.4957512860461,35.4874695880772,49.7040861184335));
#26139=CARTESIAN_POINT('Ctrl Pts',(41.4907055038788,35.4870906612229,49.7013990587629));
#26140=CARTESIAN_POINT('Ctrl Pts',(41.4813506868729,35.4863891207655,49.6963637807018));
#26141=CARTESIAN_POINT('Ctrl Pts',(41.4770386946081,35.4860661579224,49.6940215660913));
#26142=CARTESIAN_POINT('Ctrl Pts',(41.4671183748088,35.4853240077362,49.6885838631581));
#26143=CARTESIAN_POINT('Ctrl Pts',(41.4615164830773,35.4849055580117,49.6854768704729));
#26144=CARTESIAN_POINT('Ctrl Pts',(41.4496637552893,35.4840213069379,49.6788255451118));
#26145=CARTESIAN_POINT('Ctrl Pts',(41.4434170169081,35.4835559483533,49.6752740639169));
#26146=CARTESIAN_POINT('Ctrl Pts',(41.4266517927132,35.482308401588,49.665618119815));
#26147=CARTESIAN_POINT('Ctrl Pts',(41.4161707595854,35.4815299723222,49.6594488531917));
#26148=CARTESIAN_POINT('Ctrl Pts',(41.3834890743421,35.4791051251109,49.6397935212714));
#26149=CARTESIAN_POINT('Ctrl Pts',(41.3615011986949,35.4774772603582,49.6259574499811));
#26150=CARTESIAN_POINT('Ctrl Pts',(41.2697896953883,35.4706730307226,49.5656274646212));
#26151=CARTESIAN_POINT('Ctrl Pts',(41.2028505569246,35.4656680059165,49.5150577699913));
#26152=CARTESIAN_POINT('Ctrl Pts',(41.0341413280169,35.4523719212485,49.3694200855606));
#26153=CARTESIAN_POINT('Ctrl Pts',(40.9390211678361,35.444101326672,49.2674449061153));
#26154=CARTESIAN_POINT('Ctrl Pts',(40.8406223051401,35.4337466277066,49.1360088050042));
#26155=CARTESIAN_POINT('Ctrl Pts',(40.8259486756661,35.4321468862919,49.1155882462738));
#26156=CARTESIAN_POINT('Ctrl Pts',(40.8051324009717,35.4297909576824,49.0853906869873));
#26157=CARTESIAN_POINT('Ctrl Pts',(40.7986713569576,35.4290468884698,49.0758355679571));
#26158=CARTESIAN_POINT('Ctrl Pts',(40.7873514190651,35.427719877505,49.0587668126784));
#26159=CARTESIAN_POINT('Ctrl Pts',(40.7824583407555,35.4271382435244,49.0512761698526));
#26160=CARTESIAN_POINT('Ctrl Pts',(40.772353399109,35.4259199987667,49.0355692955649));
#26161=CARTESIAN_POINT('Ctrl Pts',(40.7671512457259,35.4252830477511,49.0273471482827));
#26162=CARTESIAN_POINT('Ctrl Pts',(40.7537181136943,35.4236122241937,49.0057559265244));
#26163=CARTESIAN_POINT('Ctrl Pts',(40.745587885794,35.4225746851317,48.9923253319292));
#26164=CARTESIAN_POINT('Ctrl Pts',(40.7089714182371,35.417777439464,48.9301363753035));
#26165=CARTESIAN_POINT('Ctrl Pts',(40.6824733250095,35.4139471793126,48.8802456189056));
#26166=CARTESIAN_POINT('Ctrl Pts',(40.5834855215002,35.398050051463,48.672331570749));
#26167=CARTESIAN_POINT('Ctrl Pts',(40.5303324488016,35.3853919410592,48.5060468796598));
#26168=CARTESIAN_POINT('Ctrl Pts',(40.4932818941363,35.370442066012,48.2958716787038));
#26169=CARTESIAN_POINT('Ctrl Pts',(40.4876042984503,35.3676986420534,48.2566264638591));
#26170=CARTESIAN_POINT('Ctrl Pts',(40.4816948812438,35.3641396210497,48.2044814807771));
#26171=CARTESIAN_POINT('Ctrl Pts',(40.4803771739966,35.3632752261565,48.1917170621141));
#26172=CARTESIAN_POINT('Ctrl Pts',(40.4785940050237,35.3619901209192,48.1725758214111));
#26173=CARTESIAN_POINT('Ctrl Pts',(40.4780327471933,35.3615644775972,48.1662085848358));
#26174=CARTESIAN_POINT('Ctrl Pts',(40.4771170845702,35.3608315623895,48.1551952319816));
#26175=CARTESIAN_POINT('Ctrl Pts',(40.4767478509666,35.360523480978,48.150550452937));
#26176=CARTESIAN_POINT('Ctrl Pts',(40.4760423140712,35.359908606055,48.1412486448363));
#26177=CARTESIAN_POINT('Ctrl Pts',(40.4757060835667,35.3596018224487,48.1365916577401));
#26178=CARTESIAN_POINT('Ctrl Pts',(40.4750344638594,35.3589585419743,48.1267942318297));
#26179=CARTESIAN_POINT('Ctrl Pts',(40.4747027483597,35.358622249535,48.1216535526852));
#26180=CARTESIAN_POINT('Ctrl Pts',(40.4739614927812,35.3578236326744,48.1094026801593));
#26181=CARTESIAN_POINT('Ctrl Pts',(40.4735707234394,35.3573623096458,48.1022913675388));
#26182=CARTESIAN_POINT('Ctrl Pts',(40.4716692387488,35.354876560639,48.0637977357197));
#26183=CARTESIAN_POINT('Ctrl Pts',(40.470885883251,35.3528888685554,48.0323825261852));
#26184=CARTESIAN_POINT('Ctrl Pts',(40.4708702390927,35.3509292085261,48.0009604591324));
#26185=CARTESIAN_POINT('Ctrl Pts',(40.4708702403991,35.350929371948,48.0009630795115));
#26186=CARTESIAN_POINT('Ctrl Pts',(40.4707910326032,35.3410344229544,47.8423031615214));
#26187=CARTESIAN_POINT('Ctrl Pts',(40.4902846846639,35.3318563635985,47.6842154128848));
#26188=CARTESIAN_POINT('Ctrl Pts',(40.5492871826736,35.3172044227034,47.4491870401164));
#26189=CARTESIAN_POINT('Ctrl Pts',(40.5748924597533,35.3120584573135,47.3695138903177));
#26190=CARTESIAN_POINT('Ctrl Pts',(40.6120213416988,35.3056228606644,47.2754432141581));
#26191=CARTESIAN_POINT('Ctrl Pts',(40.6186829448132,35.3044995962526,47.25921680992));
#26192=CARTESIAN_POINT('Ctrl Pts',(40.6295395438284,35.3027157827095,47.2337657290518));
#26193=CARTESIAN_POINT('Ctrl Pts',(40.6335876517912,35.3020602338153,47.2244791463582));
#26194=CARTESIAN_POINT('Ctrl Pts',(40.6413160825334,35.3008261327034,47.2071241757825));
#26195=CARTESIAN_POINT('Ctrl Pts',(40.6449792742929,35.3002481815543,47.1990484146391));
#26196=CARTESIAN_POINT('Ctrl Pts',(40.653321488198,35.2989473262594,47.1809894459627));
#26197=CARTESIAN_POINT('Ctrl Pts',(40.658030645887,35.2982233935928,47.1710205841216));
#26198=CARTESIAN_POINT('Ctrl Pts',(40.6702623740337,35.2963688014655,47.1456916161123));
#26199=CARTESIAN_POINT('Ctrl Pts',(40.6779041054205,35.2952340267535,47.1303904513169));
#26200=CARTESIAN_POINT('Ctrl Pts',(40.7398154420948,35.2862215227583,47.0104415047958));
#26201=CARTESIAN_POINT('Ctrl Pts',(40.8033604325451,35.2780101349555,46.910884842358));
#26202=CARTESIAN_POINT('Ctrl Pts',(40.9420680301487,35.2619202148804,46.7320300148092));
#26203=CARTESIAN_POINT('Ctrl Pts',(41.0156710569347,35.2541000536149,46.6520579796041));
#26204=CARTESIAN_POINT('Ctrl Pts',(41.1175401158697,35.244428105604,46.5585682870385));
#26205=CARTESIAN_POINT('Ctrl Pts',(41.1399367493887,35.2423652604611,46.5389491665068));
#26206=CARTESIAN_POINT('Ctrl Pts',(41.1730358061858,35.2394174299215,46.5112823954314));
#26207=CARTESIAN_POINT('Ctrl Pts',(41.1833810859736,35.2385098238655,46.5028160835447));
#26208=CARTESIAN_POINT('Ctrl Pts',(41.1997936702361,35.2370924702989,46.4896669132269));
#26209=CARTESIAN_POINT('Ctrl Pts',(41.2058020970208,35.2365782653914,46.4849116724714));
#26210=CARTESIAN_POINT('Ctrl Pts',(41.2170232915207,35.2356268357001,46.4761391235322));
#26211=CARTESIAN_POINT('Ctrl Pts',(41.222228567798,35.2351889973718,46.4721124647835));
#26212=CARTESIAN_POINT('Ctrl Pts',(41.2313766593163,35.2344257820294,46.4651102836687));
#26213=CARTESIAN_POINT('Ctrl Pts',(41.2353104649982,35.2340996009585,46.4621231378867));
#26214=CARTESIAN_POINT('Ctrl Pts',(41.2436358564932,35.2334135762023,46.4558514979612));
#26215=CARTESIAN_POINT('Ctrl Pts',(41.2480300183165,35.2330539793792,46.4525705858092));
#26216=CARTESIAN_POINT('Ctrl Pts',(41.2597152560727,35.2321041158962,46.4439231327865));
#26217=CARTESIAN_POINT('Ctrl Pts',(41.2670303258039,35.2315160505334,46.4385890229912));
#26218=CARTESIAN_POINT('Ctrl Pts',(41.2987921764028,35.2289895744355,46.4157691904611));
#26219=CARTESIAN_POINT('Ctrl Pts',(41.323609643877,35.2270837263489,46.3988035824811));
#26220=CARTESIAN_POINT('Ctrl Pts',(41.4520312474011,35.2175080686372,46.3153485600807));
#26221=CARTESIAN_POINT('Ctrl Pts',(41.5614411559388,35.2102641733051,46.2582995067582));
#26222=CARTESIAN_POINT('Ctrl Pts',(41.7704204520914,35.1967898889338,46.1736238516972));
#26223=CARTESIAN_POINT('Ctrl Pts',(41.868187684998,35.1906169339228,46.1427997978727));
#26224=CARTESIAN_POINT('Ctrl Pts',(41.9971085864832,35.1823151196081,46.1131726920815));
#26225=CARTESIAN_POINT('Ctrl Pts',(42.0264358370739,35.1804170379924,46.1071480664431));
#26226=CARTESIAN_POINT('Ctrl Pts',(42.0681791444727,35.1776963703515,46.0995807151031));
#26227=CARTESIAN_POINT('Ctrl Pts',(42.0804892098758,35.1768917368142,46.0974723703642));
#26228=CARTESIAN_POINT('Ctrl Pts',(42.1017718063175,35.1754962563156,46.0940396788511));
#26229=CARTESIAN_POINT('Ctrl Pts',(42.1107349073189,35.174907222545,46.0926587870153));
#26230=CARTESIAN_POINT('Ctrl Pts',(42.1279473712841,35.1737733676104,46.0901310810871));
#26231=CARTESIAN_POINT('Ctrl Pts',(42.136195095606,35.1732288740278,46.0889743882014));
#26232=CARTESIAN_POINT('Ctrl Pts',(42.1556414032248,35.171942178823,46.0863754498353));
#26233=CARTESIAN_POINT('Ctrl Pts',(42.1668455705668,35.1711985760671,46.0849780561066));
#26234=CARTESIAN_POINT('Ctrl Pts',(42.2060702344192,35.1685870379329,46.0804352488309));
#26235=CARTESIAN_POINT('Ctrl Pts',(42.2341457191482,35.1667030205057,46.077805992582));
#26236=CARTESIAN_POINT('Ctrl Pts',(42.4401768850435,35.152762308989,46.0630585232234));
#26237=CARTESIAN_POINT('Ctrl Pts',(42.6189678031594,35.1399205916771,46.075062518069));
#26238=CARTESIAN_POINT('Ctrl Pts',(42.8608282290547,35.1223719875436,46.1254579197731));
#26239=CARTESIAN_POINT('Ctrl Pts',(42.9273529071344,35.1175411813774,46.1430747158722));
#26240=CARTESIAN_POINT('Ctrl Pts',(43.007320433484,35.1118331643388,46.1688972566215));
#26241=CARTESIAN_POINT('Ctrl Pts',(43.0217846940913,35.1108048476503,46.1737581770791));
#26242=CARTESIAN_POINT('Ctrl Pts',(43.0425502220222,35.1093360387243,46.181012052417));
#26243=CARTESIAN_POINT('Ctrl Pts',(43.0488985794319,35.1088880171073,46.1832670591772));
#26244=CARTESIAN_POINT('Ctrl Pts',(43.0599550355147,35.1081096699595,46.1872597839482));
#26245=CARTESIAN_POINT('Ctrl Pts',(43.0646683505914,35.1077784868233,46.1889826820685));
#26246=CARTESIAN_POINT('Ctrl Pts',(43.0746795499291,35.107076416936,46.1926865100509));
#26247=CARTESIAN_POINT('Ctrl Pts',(43.0799754803225,35.1067058251663,46.1946723582017));
#26248=CARTESIAN_POINT('Ctrl Pts',(43.0944545843509,35.105694628989,46.2001744310183));
#26249=CARTESIAN_POINT('Ctrl Pts',(43.1036198807677,35.1050567553901,46.2037376801119));
#26250=CARTESIAN_POINT('Ctrl Pts',(43.1483814677261,35.1019504984579,46.2215350981755));
#26251=CARTESIAN_POINT('Ctrl Pts',(43.1835779088949,35.0995359800672,46.2367591333242));
#26252=CARTESIAN_POINT('Ctrl Pts',(43.2505743275295,35.0949509912259,46.2681408680256));
#26253=CARTESIAN_POINT('Ctrl Pts',(43.2824251605889,35.0927762211357,46.2841507033565));
#26254=CARTESIAN_POINT('Ctrl Pts',(43.4148334958615,35.0836832440711,46.3553686232979));
#26255=CARTESIAN_POINT('Ctrl Pts',(43.510804973805,35.0769490411829,46.4186041567725));
#26256=CARTESIAN_POINT('Ctrl Pts',(43.6668603086326,35.0649000318803,46.5426821727144));
#26257=CARTESIAN_POINT('Ctrl Pts',(43.7295810104769,35.0596919360414,46.5996707648466));
#26258=CARTESIAN_POINT('Ctrl Pts',(43.8005667697892,35.0531863671815,46.6732502924301));
#26259=CARTESIAN_POINT('Ctrl Pts',(43.8126074833879,35.0520597991942,46.6860775791096));
#26260=CARTESIAN_POINT('Ctrl Pts',(43.8313100851585,35.0502719264175,46.7065562032921));
#26261=CARTESIAN_POINT('Ctrl Pts',(43.8380901301796,35.0496156609864,46.7140986872734));
#26262=CARTESIAN_POINT('Ctrl Pts',(43.8506855445385,35.0483809312922,46.7283347046998));
#26263=CARTESIAN_POINT('Ctrl Pts',(43.8565148729506,35.0478030742465,46.7350155760447));
#26264=CARTESIAN_POINT('Ctrl Pts',(43.8694784794013,35.0465033820213,46.7500813003261));
#26265=CARTESIAN_POINT('Ctrl Pts',(43.8765874051512,35.0457805263911,46.7584874613569));
#26266=CARTESIAN_POINT('Ctrl Pts',(43.8945217621835,35.0439305543827,46.780066410711));
#26267=CARTESIAN_POINT('Ctrl Pts',(43.9052450307496,35.0427993577656,46.7933224849028));
#26268=CARTESIAN_POINT('Ctrl Pts',(43.983883608601,35.0343117662949,46.8932147988588));
#26269=CARTESIAN_POINT('Ctrl Pts',(44.0444360973722,35.0266669205856,46.9853654748048));
#26270=CARTESIAN_POINT('Ctrl Pts',(44.1654091204863,35.0086315499937,47.2090063529896));
#26271=CARTESIAN_POINT('Ctrl Pts',(44.2195845043396,34.9981672353549,47.3431474463877));
#26272=CARTESIAN_POINT('Ctrl Pts',(44.2639737984576,34.986847708075,47.5024157689889));
#26273=CARTESIAN_POINT('Ctrl Pts',(44.2693085596672,34.98541633751,47.5228480455898));
#26274=CARTESIAN_POINT('Ctrl Pts',(44.2761197078823,34.9834897765473,47.5508051172287));
#26275=CARTESIAN_POINT('Ctrl Pts',(44.2778881025543,34.9829793763453,47.5582563184348));
#26276=CARTESIAN_POINT('Ctrl Pts',(44.2807782840316,34.9821278935009,47.5707652877429));
#26277=CARTESIAN_POINT('Ctrl Pts',(44.28192413927,34.9817854651245,47.5758173412128));
#26278=CARTESIAN_POINT('Ctrl Pts',(44.2840652326116,34.9811363153673,47.585436848361));
#26279=CARTESIAN_POINT('Ctrl Pts',(44.2850642385299,34.9808293728925,47.5900033838992));
#26280=CARTESIAN_POINT('Ctrl Pts',(44.2874024902125,34.9801010325886,47.6008809473366));
#26281=CARTESIAN_POINT('Ctrl Pts',(44.2887267061933,34.9796804829437,47.6071952005278));
#26282=CARTESIAN_POINT('Ctrl Pts',(44.2933144363477,34.9781937748502,47.6296305413415));
#26283=CARTESIAN_POINT('Ctrl Pts',(44.2964035368075,34.9771369616707,47.6457871264666));
#26284=CARTESIAN_POINT('Ctrl Pts',(44.3169410161658,34.9696741669035,47.7611849111638));
#26285=CARTESIAN_POINT('Ctrl Pts',(44.3267991839944,34.9636224366732,47.8616322056378));
#26286=CARTESIAN_POINT('Ctrl Pts',(44.3308895465952,34.9510878852683,48.0714600661437));
#26287=CARTESIAN_POINT('Ctrl Pts',(44.3237620215163,34.9446275369778,48.1804966275108));
#26288=CARTESIAN_POINT('Ctrl Pts',(44.299062238229,34.934476137338,48.3438912680237));
#26289=CARTESIAN_POINT('Ctrl Pts',(44.2882436519479,34.9309691664652,48.3990408313915));
#26290=CARTESIAN_POINT('Ctrl Pts',(44.2713494562757,34.9263854749343,48.4688703812571));
#26291=CARTESIAN_POINT('Ctrl Pts',(44.2674783415885,34.9253797720401,48.4840587176716));
#26292=CARTESIAN_POINT('Ctrl Pts',(44.2609064035717,34.9237404364646,48.5085906712521));
#26293=CARTESIAN_POINT('Ctrl Pts',(44.2583191876121,34.9231104965663,48.5179641927033));
#26294=CARTESIAN_POINT('Ctrl Pts',(44.2532151072212,34.9218963733623,48.5359257475557));
#26295=CARTESIAN_POINT('Ctrl Pts',(44.2507091271093,34.9213125589365,48.5445166322527));
#26296=CARTESIAN_POINT('Ctrl Pts',(44.2448330791886,34.91997095172,48.5641513872732));
#26297=CARTESIAN_POINT('Ctrl Pts',(44.2414234760309,34.9192118798823,48.5751829707751));
#26298=CARTESIAN_POINT('Ctrl Pts',(44.2302546745037,34.9167849900989,48.610201567812));
#26299=CARTESIAN_POINT('Ctrl Pts',(44.2221244811639,34.9151050605648,48.6340665574879));
#26300=CARTESIAN_POINT('Ctrl Pts',(44.1666592338434,34.9041664322035,48.7869903754927));
#26301=CARTESIAN_POINT('Ctrl Pts',(44.1061196249513,34.8944604748934,48.9108136201175));
#26302=CARTESIAN_POINT('Ctrl Pts',(43.9877161565048,34.8785772710473,49.0990537908569));
#26303=CARTESIAN_POINT('Ctrl Pts',(43.9377729480523,34.8724948295363,49.1679116577878));
#26304=CARTESIAN_POINT('Ctrl Pts',(43.866716044311,34.8647503090157,49.2533841444767));
#26305=CARTESIAN_POINT('Ctrl Pts',(43.8495730441084,34.8629429605096,49.2731715904035));
#26306=CARTESIAN_POINT('Ctrl Pts',(43.8200964089438,34.8599438900837,49.3058277224253));
#26307=CARTESIAN_POINT('Ctrl Pts',(43.8079779468813,34.8587401551891,49.3188851383942));
#26308=CARTESIAN_POINT('Ctrl Pts',(43.790732492187,34.8570698796681,49.3369581332117));
#26309=CARTESIAN_POINT('Ctrl Pts',(43.7857561942951,34.8565927695146,49.3421153783514));
#26310=CARTESIAN_POINT('Ctrl Pts',(43.7771994086913,34.8557808244713,49.3508849732577));
#26311=CARTESIAN_POINT('Ctrl Pts',(43.7736331919415,34.8554449064301,49.3545110847558));
#26312=CARTESIAN_POINT('Ctrl Pts',(43.7662061707503,34.8547505080362,49.3620033431059));
#26313=CARTESIAN_POINT('Ctrl Pts',(43.7623432387804,34.8543921999436,49.3658672370415));
#26314=CARTESIAN_POINT('Ctrl Pts',(43.752100855387,34.8534495116636,49.3760254894496));
#26315=CARTESIAN_POINT('Ctrl Pts',(43.7456937778531,34.8528672738467,49.3822919860276));
#26316=CARTESIAN_POINT('Ctrl Pts',(43.7182011406565,34.8503992269926,49.408809062208));
#26317=CARTESIAN_POINT('Ctrl Pts',(43.6966991771984,34.8485441541264,49.4286247529707));
#26318=CARTESIAN_POINT('Ctrl Pts',(43.5817327160059,34.838958364565,49.5298398547034));
#26319=CARTESIAN_POINT('Ctrl Pts',(43.48102658351,34.8316658507289,49.6025886101786));
#26320=CARTESIAN_POINT('Ctrl Pts',(43.2738953751537,34.817326565828,49.7237477629708));
#26321=CARTESIAN_POINT('Ctrl Pts',(43.1686983903165,34.8103202804322,49.7731602450541));
#26322=CARTESIAN_POINT('Ctrl Pts',(43.0399753166011,34.8016411173085,49.8200041543026));
#26323=CARTESIAN_POINT('Ctrl Pts',(43.0201267719649,34.8003006256163,49.8268624083264));
#26324=CARTESIAN_POINT('Ctrl Pts',(42.9898516257488,34.7982507809556,49.8367731252652));
#26325=CARTESIAN_POINT('Ctrl Pts',(42.9795042623673,34.7975492864027,49.8400639271551));
#26326=CARTESIAN_POINT('Ctrl Pts',(42.9606674079949,34.7962703604362,49.8458800216732));
#26327=CARTESIAN_POINT('Ctrl Pts',(42.9521872018552,34.7956939072857,49.8484345502355));
#26328=CARTESIAN_POINT('Ctrl Pts',(42.9338505096312,34.7944458174774,49.8538207452563));
#26329=CARTESIAN_POINT('Ctrl Pts',(42.9239884718509,34.7937735458424,49.8566323805848));
#26330=CARTESIAN_POINT('Ctrl Pts',(42.8971016034674,34.7919377531545,49.8640664574837));
#26331=CARTESIAN_POINT('Ctrl Pts',(42.8800353778499,34.7907692568002,49.8685341213847));
#26332=CARTESIAN_POINT('Ctrl Pts',(42.7873740701533,34.7844056379229,49.8914381538581));
#26333=CARTESIAN_POINT('Ctrl Pts',(42.7107869000632,34.7790726081068,49.9055197886155));
#26334=CARTESIAN_POINT('Ctrl Pts',(42.5051008804217,34.7645718249996,49.9306075358704));
#26335=CARTESIAN_POINT('Ctrl Pts',(42.3753871547979,34.7552242677233,49.9333084875517));
#26336=CARTESIAN_POINT('Ctrl Pts',(42.1826551680896,34.741549554268,49.917913597022));
#26337=CARTESIAN_POINT('Ctrl Pts',(42.1191997759921,34.7370886048187,49.9096555631087));
#26338=CARTESIAN_POINT('Ctrl Pts',(42.0456199791526,34.7320470361389,49.8963318283593));
#26339=CARTESIAN_POINT('Ctrl Pts',(42.0349904446744,34.7313219854366,49.8943145568442));
#26340=CARTESIAN_POINT('Ctrl Pts',(42.0186212939061,34.7302110600325,49.8910651196483));
#26341=CARTESIAN_POINT('Ctrl Pts',(42.0128695920834,34.729821785173,49.8898960431079));
#26342=CARTESIAN_POINT('Ctrl Pts',(42.0022458314604,34.7291048736054,49.8876861488563));
#26343=CARTESIAN_POINT('Ctrl Pts',(41.9973724785929,34.7287768438049,49.8866527118456));
#26344=CARTESIAN_POINT('Ctrl Pts',(41.9862508695943,34.7280300966293,49.884249221513));
#26345=CARTESIAN_POINT('Ctrl Pts',(41.9800053836516,34.727612079981,49.8828669620595));
#26346=CARTESIAN_POINT('Ctrl Pts',(41.9636401959279,34.7265199539365,49.8791595166354));
#26347=CARTESIAN_POINT('Ctrl Pts',(41.9535320307828,34.7258486186065,49.8767836133903));
#26348=CARTESIAN_POINT('Ctrl Pts',(41.893116594292,34.7218527854595,49.8620673518438));
#26349=CARTESIAN_POINT('Ctrl Pts',(41.8433080751587,34.7186276828276,49.8477875483252));
#26350=CARTESIAN_POINT('Ctrl Pts',(41.7941388232987,34.7154586800303,49.8315225337042));
#26351=CARTESIAN_POINT('Origin',(42.4,48.4493818343519,48.));
#26352=CARTESIAN_POINT('',(41.7941388605861,33.7518842900812,49.8315225460387));
#26353=CARTESIAN_POINT('',(41.7941388307093,33.9245485747014,49.8315225361556));
#26354=CARTESIAN_POINT('',(41.7941388317924,48.4493818343519,49.8315225365138));
#26355=CARTESIAN_POINT('Ctrl Pts',(41.7941388605861,33.7518842900812,49.8315225460387));
#26356=CARTESIAN_POINT('Ctrl Pts',(41.822232866932,33.7536518916214,49.8408159433448));
#26357=CARTESIAN_POINT('Ctrl Pts',(41.8505427048789,33.7554237930209,49.8494635973993));
#26358=CARTESIAN_POINT('Ctrl Pts',(41.9390087870209,33.7609551756864,49.8742753243044));
#26359=CARTESIAN_POINT('Ctrl Pts',(41.9997463210171,33.7647460998173,49.8881782151908));
#26360=CARTESIAN_POINT('Ctrl Pts',(42.0871543217508,33.7702702333918,49.903778733364));
#26361=CARTESIAN_POINT('Ctrl Pts',(42.1133543773063,33.7719344596225,49.9078993867084));
#26362=CARTESIAN_POINT('Ctrl Pts',(42.1602908109223,33.7749363406311,49.914292779316));
#26363=CARTESIAN_POINT('Ctrl Pts',(42.1809950745463,33.7762675639675,49.91677179882));
#26364=CARTESIAN_POINT('Ctrl Pts',(42.2125073581935,33.7783062277639,49.9200276957443));
#26365=CARTESIAN_POINT('Ctrl Pts',(42.2232888838593,33.7790059447404,49.9210499776618));
#26366=CARTESIAN_POINT('Ctrl Pts',(42.2420512235811,33.7802277014822,49.92266970193));
#26367=CARTESIAN_POINT('Ctrl Pts',(42.2500282833642,33.7807484300427,49.9233083683212));
#26368=CARTESIAN_POINT('Ctrl Pts',(42.2679610254475,33.7819220376976,49.9246318735474));
#26369=CARTESIAN_POINT('Ctrl Pts',(42.2779184515369,33.7825757694634,49.9252891285832));
#26370=CARTESIAN_POINT('Ctrl Pts',(42.3046863918602,33.7843389299273,49.926847495933));
#26371=CARTESIAN_POINT('Ctrl Pts',(42.3215040257394,33.7854527986798,49.9276058486636));
#26372=CARTESIAN_POINT('Ctrl Pts',(42.4009561856744,33.7907453579105,49.9301470983325));
#26373=CARTESIAN_POINT('Ctrl Pts',(42.4636370639459,33.7950112832498,49.929097602358));
#26374=CARTESIAN_POINT('Ctrl Pts',(42.6529815685964,33.8081735173773,49.9166893733019));
#26375=CARTESIAN_POINT('Ctrl Pts',(42.7786717357399,33.8173093371442,49.8958637648311));
#26376=CARTESIAN_POINT('Ctrl Pts',(42.9809484443892,33.8322197798767,49.8414208014523));
#26377=CARTESIAN_POINT('Ctrl Pts',(43.0590691797337,33.8380239895011,49.8149277386139));
#26378=CARTESIAN_POINT('Ctrl Pts',(43.145745860273,33.8443511675098,49.7791948218707));
#26379=CARTESIAN_POINT('Ctrl Pts',(43.1561898664617,33.8451115677599,49.7747811142232));
#26380=CARTESIAN_POINT('Ctrl Pts',(43.172082132481,33.8462649352774,49.7678991760523));
#26381=CARTESIAN_POINT('Ctrl Pts',(43.1775586212095,33.8466617091395,49.7654973545625));
#26382=CARTESIAN_POINT('Ctrl Pts',(43.1875706076989,33.8473857196794,49.7610507785014));
#26383=CARTESIAN_POINT('Ctrl Pts',(43.1921093776766,33.847713410377,49.7590139401158));
#26384=CARTESIAN_POINT('Ctrl Pts',(43.2023422647975,33.8484510431897,49.7543741455057));
#26385=CARTESIAN_POINT('Ctrl Pts',(43.2080316209621,33.8488603562039,49.7517610152487));
#26386=CARTESIAN_POINT('Ctrl Pts',(43.2227085533099,33.849914448055,49.7449331591289));
#26387=CARTESIAN_POINT('Ctrl Pts',(43.2316766320263,33.850556758547,49.7406766165279));
#26388=CARTESIAN_POINT('Ctrl Pts',(43.291606577009,33.8548397688464,49.7116630047079));
#26389=CARTESIAN_POINT('Ctrl Pts',(43.3414945753509,33.8583601345675,49.6847379095925));
#26390=CARTESIAN_POINT('Ctrl Pts',(43.5000139619265,33.8696313080522,49.5899386099328));
#26391=CARTESIAN_POINT('Ctrl Pts',(43.6030868347116,33.8771162984925,49.5134465912978));
#26392=CARTESIAN_POINT('Ctrl Pts',(43.7617847498799,33.8900687937594,49.3691450268038));
#26393=CARTESIAN_POINT('Ctrl Pts',(43.821755891981,33.8953819176344,49.3067605727313));
#26394=CARTESIAN_POINT('Ctrl Pts',(43.888708870321,33.9020059845809,49.2270293897812));
#26395=CARTESIAN_POINT('Ctrl Pts',(43.8998929007683,33.9031381900633,49.2133327971986));
#26396=CARTESIAN_POINT('Ctrl Pts',(43.9172059670459,33.9049331095973,49.1915250311266));
#26397=CARTESIAN_POINT('Ctrl Pts',(43.9234620486964,33.9055907181354,49.1835156212978));
#26398=CARTESIAN_POINT('Ctrl Pts',(43.9350574786617,33.9068268289098,49.168426173626));
#26399=CARTESIAN_POINT('Ctrl Pts',(43.9404118844503,33.9074047137297,49.161358001576));
#26400=CARTESIAN_POINT('Ctrl Pts',(43.9522911470585,33.9087029632722,49.145449896967));
#26401=CARTESIAN_POINT('Ctrl Pts',(43.9587895524967,33.9094243363076,49.1365906889546));
#26402=CARTESIAN_POINT('Ctrl Pts',(43.9751326445211,33.9112675886956,49.1139065253));
#26403=CARTESIAN_POINT('Ctrl Pts',(43.9848710461081,33.9123934958351,49.1000065139391));
#26404=CARTESIAN_POINT('Ctrl Pts',(44.0634051406204,33.9217063028889,48.9847035949815));
#26405=CARTESIAN_POINT('Ctrl Pts',(44.1225667772653,33.9302559084962,48.8771040053248));
#26406=CARTESIAN_POINT('Ctrl Pts',(44.2057662416209,33.9451935126621,48.6843912200507));
#26407=CARTESIAN_POINT('Ctrl Pts',(44.234918345372,33.9514748609294,48.6018787104879));
#26408=CARTESIAN_POINT('Ctrl Pts',(44.2744041595347,33.9618614540488,48.4601301510694));
#26409=CARTESIAN_POINT('Ctrl Pts',(44.2877539665317,33.9660189564635,48.4018671269507));
#26410=CARTESIAN_POINT('Ctrl Pts',(44.3002745969006,33.970764309379,48.3325847339285));
#26411=CARTESIAN_POINT('Ctrl Pts',(44.3020830922692,33.9714784137988,48.3220808465803));
#26412=CARTESIAN_POINT('Ctrl Pts',(44.3047470050473,33.9725762548199,48.3058029772046));
#26413=CARTESIAN_POINT('Ctrl Pts',(44.3056633960849,33.9729632690532,48.3000393926898));
#26414=CARTESIAN_POINT('Ctrl Pts',(44.3073144007316,33.9736782628013,48.2893427150847));
#26415=CARTESIAN_POINT('Ctrl Pts',(44.3080560377137,33.9740066158058,48.2844109488446));
#26416=CARTESIAN_POINT('Ctrl Pts',(44.3097126228468,33.9747569820751,48.2730967317232));
#26417=CARTESIAN_POINT('Ctrl Pts',(44.3106147069066,33.9751782686558,48.2667125258596));
#26418=CARTESIAN_POINT('Ctrl Pts',(44.3129086928837,33.9762844969707,48.2498684293201));
#26419=CARTESIAN_POINT('Ctrl Pts',(44.3142468349627,33.9769665484997,48.2394012658995));
#26420=CARTESIAN_POINT('Ctrl Pts',(44.3257343374219,33.9831849895461,48.143280453926));
#26421=CARTESIAN_POINT('Ctrl Pts',(44.3302157675812,33.9884399286319,48.0570355704692));
#26422=CARTESIAN_POINT('Ctrl Pts',(44.3276721578753,33.9985245239661,47.8891793323548));
#26423=CARTESIAN_POINT('Ctrl Pts',(44.3212602332266,34.0033524974198,47.8077488620513));
#26424=CARTESIAN_POINT('Ctrl Pts',(44.2966692910322,34.0137850425702,47.6357481252508));
#26425=CARTESIAN_POINT('Ctrl Pts',(44.2771100328848,34.0193981362937,47.5455896322356));
#26426=CARTESIAN_POINT('Ctrl Pts',(44.2445294432212,34.0267122473274,47.4344796095866));
#26427=CARTESIAN_POINT('Ctrl Pts',(44.2374562652596,34.0282190477954,47.4119042816743));
#26428=CARTESIAN_POINT('Ctrl Pts',(44.2263673909003,34.0304709975937,47.3786673279568));
#26429=CARTESIAN_POINT('Ctrl Pts',(44.2226693515696,34.0312057004179,47.3679014621302));
#26430=CARTESIAN_POINT('Ctrl Pts',(44.2159090450167,34.0325207850789,47.3487733177477));
#26431=CARTESIAN_POINT('Ctrl Pts',(44.2128837225318,34.033099924758,47.3403982598858));
#26432=CARTESIAN_POINT('Ctrl Pts',(44.2063690206875,34.0343277501909,47.3227469160133));
#26433=CARTESIAN_POINT('Ctrl Pts',(44.202865932548,34.0349768811725,47.3134760006393));
#26434=CARTESIAN_POINT('Ctrl Pts',(44.1933332323262,34.0367145428095,47.2888239280374));
#26435=CARTESIAN_POINT('Ctrl Pts',(44.1871773215702,34.037807293458,47.273492821955));
#26436=CARTESIAN_POINT('Ctrl Pts',(44.1584582388205,34.0427780331259,47.2045434525091));
#26437=CARTESIAN_POINT('Ctrl Pts',(44.1336758491486,34.0467304939546,47.1518883694762));
#26438=CARTESIAN_POINT('Ctrl Pts',(44.0386686874587,34.0608229742627,46.9716508100176));
#26439=CARTESIAN_POINT('Ctrl Pts',(43.9564258887153,34.0713329470031,46.8509715297968));
#26440=CARTESIAN_POINT('Ctrl Pts',(43.8305802676179,34.0849998679582,46.7049271815965));
#26441=CARTESIAN_POINT('Ctrl Pts',(43.7984418401567,34.088319077317,46.6702878052449));
#26442=CARTESIAN_POINT('Ctrl Pts',(43.7458736411927,34.0934469748352,46.6176454355684));
#26443=CARTESIAN_POINT('Ctrl Pts',(43.7262802320962,34.0952973005341,46.5988358662521));
#26444=CARTESIAN_POINT('Ctrl Pts',(43.700106436352,34.0976832655497,46.5747503585811));
#26445=CARTESIAN_POINT('Ctrl Pts',(43.6938805498566,34.098244647818,46.5690959447452));
#26446=CARTESIAN_POINT('Ctrl Pts',(43.6836392776758,34.099157787683,46.559916215332));
#26447=CARTESIAN_POINT('Ctrl Pts',(43.6796459530222,34.0995113150944,46.5563666190093));
#26448=CARTESIAN_POINT('Ctrl Pts',(43.6718136874222,34.1001996894999,46.5494626896049));
#26449=CARTESIAN_POINT('Ctrl Pts',(43.6679761272525,34.1005346379584,46.5461069207236));
#26450=CARTESIAN_POINT('Ctrl Pts',(43.6593679387113,34.1012808933833,46.538639464254));
#26451=CARTESIAN_POINT('Ctrl Pts',(43.6545903417644,34.1016916133191,46.5345358081608));
#26452=CARTESIAN_POINT('Ctrl Pts',(43.6379587537702,34.1031098144803,46.5203912639077));
#26453=CARTESIAN_POINT('Ctrl Pts',(43.6260032655341,34.1041090369793,46.510469900359));
#26454=CARTESIAN_POINT('Ctrl Pts',(43.5144048639429,34.113265076725,46.4201131076715));
#26455=CARTESIAN_POINT('Ctrl Pts',(43.4070898477608,34.1208376588896,46.3496302408002));
#26456=CARTESIAN_POINT('Ctrl Pts',(43.1786794086179,34.1362127229208,46.2302526907813));
#26457=CARTESIAN_POINT('Ctrl Pts',(43.0580482310038,34.1439878431679,46.1819478068621));
#26458=CARTESIAN_POINT('Ctrl Pts',(42.9131658630505,34.1535383970897,46.1402551869565));
#26459=CARTESIAN_POINT('Ctrl Pts',(42.8927444220757,34.1548884716449,46.1347405406489));
#26460=CARTESIAN_POINT('Ctrl Pts',(42.8616774375999,34.1569501218697,46.1268969292018));
#26461=CARTESIAN_POINT('Ctrl Pts',(42.8510956127996,34.1576537004727,46.1243204137463));
#26462=CARTESIAN_POINT('Ctrl Pts',(42.8318658413446,34.1589349807853,46.1198103902428));
#26463=CARTESIAN_POINT('Ctrl Pts',(42.8232252530903,34.1595116886301,46.1178465911896));
#26464=CARTESIAN_POINT('Ctrl Pts',(42.8045757816949,34.1607586916989,46.1137429265483));
#26465=CARTESIAN_POINT('Ctrl Pts',(42.7945628234948,34.1614296100013,46.1116230562385));
#26466=CARTESIAN_POINT('Ctrl Pts',(42.7673414443359,34.1632576027063,46.1060858992027));
#26467=CARTESIAN_POINT('Ctrl Pts',(42.7501028552816,34.164419580178,46.1028235944153));
#26468=CARTESIAN_POINT('Ctrl Pts',(42.6579389246497,34.1706568500298,46.0866809810984));
#26469=CARTESIAN_POINT('Ctrl Pts',(42.5823550218172,34.1758634698669,46.0780046345243));
#26470=CARTESIAN_POINT('Ctrl Pts',(42.3764480937858,34.1902812780343,46.066623744375));
#26471=CARTESIAN_POINT('Ctrl Pts',(42.2460421317458,34.1996848832864,46.0726207067847));
#26472=CARTESIAN_POINT('Ctrl Pts',(42.0529119774787,34.2135001337758,46.1012365076659));
#26473=CARTESIAN_POINT('Ctrl Pts',(41.9890891160381,34.2180403938353,46.1140182900721));
#26474=CARTESIAN_POINT('Ctrl Pts',(41.9155003542557,34.2231591837011,46.1326701960611));
#26475=CARTESIAN_POINT('Ctrl Pts',(41.9049953446786,34.2238870637065,46.1354274194632));
#26476=CARTESIAN_POINT('Ctrl Pts',(41.8888402157113,34.2250014560545,46.1398137739898));
#26477=CARTESIAN_POINT('Ctrl Pts',(41.8831735240769,34.2253913999013,46.1413802119356));
#26478=CARTESIAN_POINT('Ctrl Pts',(41.8727177472141,34.2261090285339,46.1443220086038));
#26479=CARTESIAN_POINT('Ctrl Pts',(41.8679268370499,34.2264371112157,46.1456900118711));
#26480=CARTESIAN_POINT('Ctrl Pts',(41.8570058982627,34.2271833349804,46.1488542026762));
#26481=CARTESIAN_POINT('Ctrl Pts',(41.8508794513008,34.2276007805745,46.1506622852088));
#26482=CARTESIAN_POINT('Ctrl Pts',(41.8348500160493,34.2286901989678,46.1554796901142));
#26483=CARTESIAN_POINT('Ctrl Pts',(41.824961912613,34.2293594209598,46.1585383828746));
#26484=CARTESIAN_POINT('Ctrl Pts',(41.7501110949605,34.2344073203972,46.1823537487832));
#26485=CARTESIAN_POINT('Ctrl Pts',(41.6862578720286,34.2386111744229,46.2064649945738));
#26486=CARTESIAN_POINT('Ctrl Pts',(41.5165427710139,34.2498404528727,46.2810542431062));
#26487=CARTESIAN_POINT('Ctrl Pts',(41.4137929734696,34.2567139827875,46.3378723595751));
#26488=CARTESIAN_POINT('Ctrl Pts',(41.2464251629701,34.2689351904334,46.4514371182954));
#26489=CARTESIAN_POINT('Ctrl Pts',(41.1792645126794,34.2741681040886,46.5038101457411));
#26490=CARTESIAN_POINT('Ctrl Pts',(41.102638404023,34.2807018327569,46.5721674471779));
#26491=CARTESIAN_POINT('Ctrl Pts',(41.0896539549867,34.2818299135345,46.5840741125088));
#26492=CARTESIAN_POINT('Ctrl Pts',(41.0694492480694,34.2836197650522,46.6031176660628));
#26493=CARTESIAN_POINT('Ctrl Pts',(41.0621189340754,34.2842764793782,46.6101367674373));
#26494=CARTESIAN_POINT('Ctrl Pts',(41.0484874040636,34.2855117997793,46.6233973286953));
#26495=CARTESIAN_POINT('Ctrl Pts',(41.0421731589124,34.2860897960855,46.6296250597706));
#26496=CARTESIAN_POINT('Ctrl Pts',(41.0281192077104,34.2873894689447,46.643678947646));
#26497=CARTESIAN_POINT('Ctrl Pts',(41.0204031390884,34.2881121637219,46.6515281989891));
#26498=CARTESIAN_POINT('Ctrl Pts',(41.0009159954926,34.2899610812866,46.6716940291253));
#26499=CARTESIAN_POINT('Ctrl Pts',(40.9892403401556,34.2910913745722,46.6841010850821));
#26500=CARTESIAN_POINT('Ctrl Pts',(40.8936505525185,34.30053715089,46.7884134603802));
#26501=CARTESIAN_POINT('Ctrl Pts',(40.8186616933008,34.3092274526194,46.8880695941978));
#26502=CARTESIAN_POINT('Ctrl Pts',(40.7036961735488,34.3249268822896,47.0762404764824));
#26503=CARTESIAN_POINT('Ctrl Pts',(40.6597895922981,34.3318390663899,47.1618790247895));
#26504=CARTESIAN_POINT('Ctrl Pts',(40.6094580324446,34.3409325254711,47.2812374673108));
#26505=CARTESIAN_POINT('Ctrl Pts',(40.597270890511,34.3432569320642,47.3123750029397));
#26506=CARTESIAN_POINT('Ctrl Pts',(40.5786469511589,34.3470064002948,47.3638631204653));
#26507=CARTESIAN_POINT('Ctrl Pts',(40.5717278269332,34.348451890723,47.3840308349642));
#26508=CARTESIAN_POINT('Ctrl Pts',(40.5627702807873,34.3503942691453,47.4116220472493));
#26509=CARTESIAN_POINT('Ctrl Pts',(40.5604401227929,34.3509066791423,47.4189482642897));
#26510=CARTESIAN_POINT('Ctrl Pts',(40.5566110700961,34.35176064346,47.4312410710871));
#26511=CARTESIAN_POINT('Ctrl Pts',(40.5550883199822,34.3521035591689,47.4362000699688));
#26512=CARTESIAN_POINT('Ctrl Pts',(40.5522324946862,34.3527529681196,47.4456358415189));
#26513=CARTESIAN_POINT('Ctrl Pts',(40.550895650163,34.3530596870152,47.4501113944811));
#26514=CARTESIAN_POINT('Ctrl Pts',(40.5477560653823,34.3537866687357,47.4607631708681));
#26515=CARTESIAN_POINT('Ctrl Pts',(40.5459679271681,34.3542060914673,47.4669436924442));
#26516=CARTESIAN_POINT('Ctrl Pts',(40.5397491837934,34.3556844769308,47.4888480452854));
#26517=CARTESIAN_POINT('Ctrl Pts',(40.5354872685443,34.3567342316163,47.5046196039287));
#26518=CARTESIAN_POINT('Ctrl Pts',(40.5039981188426,34.3648008905328,47.6273160302459));
#26519=CARTESIAN_POINT('Ctrl Pts',(40.4857856548616,34.3713906875167,47.7363592224183));
#26520=CARTESIAN_POINT('Ctrl Pts',(40.4729574251635,34.381001334332,47.8969355725878));
#26521=CARTESIAN_POINT('Ctrl Pts',(40.4709138645376,34.3840211774907,47.947636469111));
#26522=CARTESIAN_POINT('Ctrl Pts',(40.4707861256103,34.3930358092416,48.0977350015402));
#26523=CARTESIAN_POINT('Ctrl Pts',(40.4783802582461,34.3990998965189,48.1969569761711));
#26524=CARTESIAN_POINT('Ctrl Pts',(40.4961681072347,34.4064865455506,48.3118534100388));
#26525=CARTESIAN_POINT('Ctrl Pts',(40.4989743511027,34.4075672804918,48.328526830668));
#26526=CARTESIAN_POINT('Ctrl Pts',(40.5039616422314,34.40936046529,48.3559513875274));
#26527=CARTESIAN_POINT('Ctrl Pts',(40.5060159146132,34.410068885306,48.3667248566709));
#26528=CARTESIAN_POINT('Ctrl Pts',(40.5098967328105,34.4113552991853,48.3861745728868));
#26529=CARTESIAN_POINT('Ctrl Pts',(40.5116914518943,34.4119322605123,48.394856916009));
#26530=CARTESIAN_POINT('Ctrl Pts',(40.5156747691385,34.413175678189,48.413478606991));
#26531=CARTESIAN_POINT('Ctrl Pts',(40.517882293313,34.4138427268711,48.4234135868458));
#26532=CARTESIAN_POINT('Ctrl Pts',(40.5241549233981,34.4156800395814,48.4506248946602));
#26533=CARTESIAN_POINT('Ctrl Pts',(40.5283799102703,34.4168554100861,48.4678629616182));
#26534=CARTESIAN_POINT('Ctrl Pts',(40.5549316371666,34.4238949726744,48.57007368465));
#26535=CARTESIAN_POINT('Ctrl Pts',(40.582800968148,34.4299378299245,48.6534867852099));
#26536=CARTESIAN_POINT('Ctrl Pts',(40.6464316700164,34.4416829137335,48.8079729171388));
#26537=CARTESIAN_POINT('Ctrl Pts',(40.6810960239106,34.4473483890802,48.8793122636293));
#26538=CARTESIAN_POINT('Ctrl Pts',(40.7430166382132,34.4563440869029,48.9890056276619));
#26539=CARTESIAN_POINT('Ctrl Pts',(40.7674581965911,34.4596748902882,49.0288505782284));
#26540=CARTESIAN_POINT('Ctrl Pts',(40.824926217424,34.4669968685006,49.1153229112449));
#26541=CARTESIAN_POINT('Ctrl Pts',(40.8586282703096,34.4709673971012,49.1614547548541));
#26542=CARTESIAN_POINT('Ctrl Pts',(40.9005475816166,34.4754900603971,49.2137890641451));
#26543=CARTESIAN_POINT('Ctrl Pts',(40.9068245480763,34.4761571194766,49.2215025694966));
#26544=CARTESIAN_POINT('Ctrl Pts',(40.9171534908594,34.4772379022806,49.2339967787161));
#26545=CARTESIAN_POINT('Ctrl Pts',(40.9211695155563,34.4776540510741,49.2388067728988));
#26546=CARTESIAN_POINT('Ctrl Pts',(40.9284161351557,34.4783975626133,49.2474005921585));
#26547=CARTESIAN_POINT('Ctrl Pts',(40.9316379861234,34.4787255343173,49.2511915546809));
#26548=CARTESIAN_POINT('Ctrl Pts',(40.938761774172,34.4794450204533,49.259508280677));
#26549=CARTESIAN_POINT('Ctrl Pts',(40.9426700885461,34.4798360582377,49.2640283989205));
#26550=CARTESIAN_POINT('Ctrl Pts',(40.9540404841992,34.4809633185002,49.2770558677993));
#26551=CARTESIAN_POINT('Ctrl Pts',(40.9615566492439,34.4816956758803,49.2855159868407));
#26552=CARTESIAN_POINT('Ctrl Pts',(41.0237176309969,34.4876535480489,49.3542558866026));
#26553=CARTESIAN_POINT('Ctrl Pts',(41.0820586461966,34.4926284061482,49.4110975074084));
#26554=CARTESIAN_POINT('Ctrl Pts',(41.1636066726752,34.499097073166,49.4810650375875));
#26555=CARTESIAN_POINT('Ctrl Pts',(41.183733102733,34.5006577960072,49.497637131573));
#26556=CARTESIAN_POINT('Ctrl Pts',(41.3237425838724,34.5113172752224,49.6082364214939));
#26557=CARTESIAN_POINT('Ctrl Pts',(41.4540469681758,34.5203205575784,49.6881711066788));
#26558=CARTESIAN_POINT('Ctrl Pts',(41.612259052673,34.5313176092528,49.7611034498652));
#26559=CARTESIAN_POINT('Ctrl Pts',(41.6322804190894,34.5327092175118,49.7699230900791));
#26560=CARTESIAN_POINT('Ctrl Pts',(41.662747235911,34.5348289892727,49.7827298630114));
#26561=CARTESIAN_POINT('Ctrl Pts',(41.6730848933726,34.5355486080241,49.7869700114368));
#26562=CARTESIAN_POINT('Ctrl Pts',(41.6911659544066,34.5368081644647,49.7942033782588));
#26563=CARTESIAN_POINT('Ctrl Pts',(41.6988930012064,34.5373467295258,49.7972368901701));
#26564=CARTESIAN_POINT('Ctrl Pts',(41.7151285381673,34.5384790448898,49.8034900597894));
#26565=CARTESIAN_POINT('Ctrl Pts',(41.7236406861229,34.5390731192959,49.8066995845257));
#26566=CARTESIAN_POINT('Ctrl Pts',(41.7440293527125,34.5404972112604,49.8142228979678));
#26567=CARTESIAN_POINT('Ctrl Pts',(41.7559260520934,34.5413290818809,49.8184803959012));
#26568=CARTESIAN_POINT('Ctrl Pts',(41.7766008805053,34.5427765967051,49.825651012675));
#26569=CARTESIAN_POINT('Ctrl Pts',(41.7853595582974,34.5433903872487,49.828618383941));
#26570=CARTESIAN_POINT('Ctrl Pts',(41.7941388327286,34.5440062296316,49.8315225368236));
#26571=CARTESIAN_POINT('Ctrl Pts',(41.7941388232987,34.7154586800303,49.8315225337042));
#26572=CARTESIAN_POINT('Ctrl Pts',(41.7736344100669,34.714137152034,49.8247397463239));
#26573=CARTESIAN_POINT('Ctrl Pts',(41.7532411651284,34.7128254112523,49.8176117253353));
#26574=CARTESIAN_POINT('Ctrl Pts',(41.6271329352352,34.7047064784872,49.7711411799934));
#26575=CARTESIAN_POINT('Ctrl Pts',(41.5249219055423,34.6980803716224,49.7229346514742));
#26576=CARTESIAN_POINT('Ctrl Pts',(41.3547263418778,34.6861683763357,49.6235908599801));
#26577=CARTESIAN_POINT('Ctrl Pts',(41.2848160891351,34.6809832881044,49.5763903433538));
#26578=CARTESIAN_POINT('Ctrl Pts',(41.2043303672012,34.6745036307842,49.5140097467574));
#26579=CARTESIAN_POINT('Ctrl Pts',(41.1905885079584,34.6733782777764,49.5030552864632));
#26580=CARTESIAN_POINT('Ctrl Pts',(41.1691584495875,34.6715918978665,49.485487936064));
#26581=CARTESIAN_POINT('Ctrl Pts',(41.1613692318657,34.6709358959196,49.4789993725914));
#26582=CARTESIAN_POINT('Ctrl Pts',(41.1468637234907,34.6697013977175,49.4667210548757));
#26583=CARTESIAN_POINT('Ctrl Pts',(41.1401354822522,34.6691235064202,49.4609457802432));
#26584=CARTESIAN_POINT('Ctrl Pts',(41.1251388869164,34.6678233882103,49.447892616609));
#26585=CARTESIAN_POINT('Ctrl Pts',(41.1168926267176,34.6671001378894,49.4405899301812));
#26586=CARTESIAN_POINT('Ctrl Pts',(41.0960280359407,34.6652484731519,49.4217914893404));
#26587=CARTESIAN_POINT('Ctrl Pts',(41.0834991368043,34.664115965684,49.4101983432949));
#26588=CARTESIAN_POINT('Ctrl Pts',(40.9901410290625,34.6555176897455,49.3214844283058));
#26589=CARTESIAN_POINT('Ctrl Pts',(40.9160080019861,34.6477543087434,49.2376523656323));
#26590=CARTESIAN_POINT('Ctrl Pts',(40.7646708514727,34.6297048927616,49.0332428084735));
#26591=CARTESIAN_POINT('Ctrl Pts',(40.6927653889899,34.6193591071956,48.909530119822));
#26592=CARTESIAN_POINT('Ctrl Pts',(40.6266638153182,34.6081534980392,48.7597786306435));
#26593=CARTESIAN_POINT('Ctrl Pts',(40.6184864860376,34.6067280235633,48.7404015671077));
#26594=CARTESIAN_POINT('Ctrl Pts',(40.6077700144833,34.6048080346261,48.713801581663));
#26595=CARTESIAN_POINT('Ctrl Pts',(40.6049549031321,34.6042984403167,48.7066923829105));
#26596=CARTESIAN_POINT('Ctrl Pts',(40.6003044281203,34.6034479237766,48.6947411138338));
#26597=CARTESIAN_POINT('Ctrl Pts',(40.5984461786398,34.6031056622551,48.6899081080428));
#26598=CARTESIAN_POINT('Ctrl Pts',(40.5949466041338,34.602456536956,48.6806957222437));
#26599=CARTESIAN_POINT('Ctrl Pts',(40.5933017158332,34.6021494540292,48.6763177798676));
#26600=CARTESIAN_POINT('Ctrl Pts',(40.5894226091523,34.6014204126906,48.6658782188268));
#26601=CARTESIAN_POINT('Ctrl Pts',(40.5872028686953,34.6009993062913,48.6598112261992));
#26602=CARTESIAN_POINT('Ctrl Pts',(40.5794225896686,34.599508774122,48.6382105136989));
#26603=CARTESIAN_POINT('Ctrl Pts',(40.5740307096626,34.5984487558299,48.6226162231555));
#26604=CARTESIAN_POINT('Ctrl Pts',(40.5377887331214,34.5911151990029,48.5132753584692));
#26605=CARTESIAN_POINT('Ctrl Pts',(40.5139684058475,34.5851808520025,48.4173394212657));
#26606=CARTESIAN_POINT('Ctrl Pts',(40.4798757025177,34.5729010128965,48.2146520463806));
#26607=CARTESIAN_POINT('Ctrl Pts',(40.470937742682,34.5665778950104,48.1080289255605));
#26608=CARTESIAN_POINT('Ctrl Pts',(40.4708333613994,34.5564348863422,47.9425099688844));
#26609=CARTESIAN_POINT('Ctrl Pts',(40.4734761269368,34.5527783222373,47.8838373373454));
#26610=CARTESIAN_POINT('Ctrl Pts',(40.4802886718039,34.5479826264789,47.8088839201435));
#26611=CARTESIAN_POINT('Ctrl Pts',(40.4820004146344,34.5469207897803,47.7924078457148));
#26612=CARTESIAN_POINT('Ctrl Pts',(40.4850759691509,34.5452124806315,47.7661049639124));
#26613=CARTESIAN_POINT('Ctrl Pts',(40.4863038044424,34.5445703048624,47.756262853006));
#26614=CARTESIAN_POINT('Ctrl Pts',(40.488777293159,34.5433473166793,47.7376080584221));
#26615=CARTESIAN_POINT('Ctrl Pts',(40.490008147775,34.5427669876256,47.7287936466426));
#26616=CARTESIAN_POINT('Ctrl Pts',(40.492948963966,34.5414414167135,47.7087475776204));
#26617=CARTESIAN_POINT('Ctrl Pts',(40.4946972276487,34.5406949776956,47.697521961392));
#26618=CARTESIAN_POINT('Ctrl Pts',(40.5003738303096,34.5383914862416,47.6630763254425));
#26619=CARTESIAN_POINT('Ctrl Pts',(40.5046281589263,34.5368241686635,47.6399130003809));
#26620=CARTESIAN_POINT('Ctrl Pts',(40.5274451431771,34.5291132401199,47.5273247891242));
#26621=CARTESIAN_POINT('Ctrl Pts',(40.5519156806787,34.5227845801798,47.4392294293796));
#26622=CARTESIAN_POINT('Ctrl Pts',(40.5938546242095,34.5139449615261,47.3213817972854));
#26623=CARTESIAN_POINT('Ctrl Pts',(40.606014716584,34.5115432484839,47.2898588304252));
#26624=CARTESIAN_POINT('Ctrl Pts',(40.6684763460492,34.4999529559415,47.1397978064199));
#26625=CARTESIAN_POINT('Ctrl Pts',(40.7297373496898,34.4906722932919,47.0261674606001));
#26626=CARTESIAN_POINT('Ctrl Pts',(40.8105494858338,34.4808633455891,46.9066428596439));
#26627=CARTESIAN_POINT('Ctrl Pts',(40.8193852843851,34.4798179224778,46.8939078105948));
#26628=CARTESIAN_POINT('Ctrl Pts',(40.8320219355145,34.4783617239059,46.8761552962382));
#26629=CARTESIAN_POINT('Ctrl Pts',(40.8356950351829,34.4779429339551,46.8710482257117));
#26630=CARTESIAN_POINT('Ctrl Pts',(40.8423880914217,34.4771880181418,46.8618375968035));
#26631=CARTESIAN_POINT('Ctrl Pts',(40.8453994436085,34.4768513156563,46.8577278669155));
#26632=CARTESIAN_POINT('Ctrl Pts',(40.8516022775547,34.4761638615906,46.8493325414793));
#26633=CARTESIAN_POINT('Ctrl Pts',(40.8547953360493,34.4758132234346,46.8450482022128));
#26634=CARTESIAN_POINT('Ctrl Pts',(40.8630639234661,34.4749133805269,46.8340493591683));
#26635=CARTESIAN_POINT('Ctrl Pts',(40.8681657341044,34.474365978798,46.8273546195002));
#26636=CARTESIAN_POINT('Ctrl Pts',(40.8899579860983,34.4720595443514,46.7991431410104));
#26637=CARTESIAN_POINT('Ctrl Pts',(40.9070601148937,34.4703273563418,46.7779464984727));
#26638=CARTESIAN_POINT('Ctrl Pts',(40.9551641154516,34.4656406715753,46.7208434696636));
#26639=CARTESIAN_POINT('Ctrl Pts',(40.9870514483697,34.4627338248905,46.6857058268726));
#26640=CARTESIAN_POINT('Ctrl Pts',(41.1230594356058,34.4509512566825,46.5465127260641));
#26641=CARTESIAN_POINT('Ctrl Pts',(41.2376204997747,34.4423777813987,46.4533656544679));
#26642=CARTESIAN_POINT('Ctrl Pts',(41.4094368960537,34.4298669406586,46.3436362567685));
#26643=CARTESIAN_POINT('Ctrl Pts',(41.4585308642693,34.4263319487138,46.3152474816919));
#26644=CARTESIAN_POINT('Ctrl Pts',(41.5232640980222,34.4216794729383,46.2815289692503));
#26645=CARTESIAN_POINT('Ctrl Pts',(41.5378226533404,34.4206337603073,46.2741788267945));
#26646=CARTESIAN_POINT('Ctrl Pts',(41.5613320777075,34.4189452705604,46.2626813927565));
#26647=CARTESIAN_POINT('Ctrl Pts',(41.5702248176386,34.4183066128894,46.2584165343914));
#26648=CARTESIAN_POINT('Ctrl Pts',(41.5872145536802,34.4170863214498,46.2504281107125));
#26649=CARTESIAN_POINT('Ctrl Pts',(41.5953054363182,34.4165051389295,46.2466920885897));
#26650=CARTESIAN_POINT('Ctrl Pts',(41.6138614546028,34.4151719588054,46.2382792125491));
#26651=CARTESIAN_POINT('Ctrl Pts',(41.6243428875763,34.4144187129018,46.233639340402));
#26652=CARTESIAN_POINT('Ctrl Pts',(41.6569739743552,34.4120727323447,46.2195408052784));
#26653=CARTESIAN_POINT('Ctrl Pts',(41.679259138378,34.4104691756755,46.2104036377965));
#26654=CARTESIAN_POINT('Ctrl Pts',(41.7908416108944,34.4024298586531,46.1670757824099));
#26655=CARTESIAN_POINT('Ctrl Pts',(41.8824110558163,34.3957904454417,46.1391448249262));
#26656=CARTESIAN_POINT('Ctrl Pts',(42.0765388355219,34.3817022610537,46.0953716637936));
#26657=CARTESIAN_POINT('Ctrl Pts',(42.1790789029037,34.3742532981493,46.0807737329932));
#26658=CARTESIAN_POINT('Ctrl Pts',(42.3045996033678,34.3653671237185,46.0731007426699));
#26659=CARTESIAN_POINT('Ctrl Pts',(42.3269285160482,34.3637957572839,46.0721248480569));
#26660=CARTESIAN_POINT('Ctrl Pts',(42.3900835719622,34.3593858541335,46.0704634951674));
#26661=CARTESIAN_POINT('Ctrl Pts',(42.4309245140834,34.3565747163837,46.0706856937661));
#26662=CARTESIAN_POINT('Ctrl Pts',(42.4816550139389,34.3531571768992,46.0725733110281));
#26663=CARTESIAN_POINT('Ctrl Pts',(42.4915764605684,34.3524923511301,46.073019215219));
#26664=CARTESIAN_POINT('Ctrl Pts',(42.5072215255904,34.3514500513356,46.0738434659282));
#26665=CARTESIAN_POINT('Ctrl Pts',(42.5129474911528,34.3510698597161,46.074170745972));
#26666=CARTESIAN_POINT('Ctrl Pts',(42.5231629178346,34.3503939669628,46.0748003486684));
#26667=CARTESIAN_POINT('Ctrl Pts',(42.52765276865,34.3500977345464,46.0750928404023));
#26668=CARTESIAN_POINT('Ctrl Pts',(42.5384417123617,34.3493878605732,46.0758336022027));
#26669=CARTESIAN_POINT('Ctrl Pts',(42.5447396709526,34.348975074723,46.0762970955537));
#26670=CARTESIAN_POINT('Ctrl Pts',(42.5639917450296,34.3477178146806,46.0778090188657));
#26671=CARTESIAN_POINT('Ctrl Pts',(42.5769379543931,34.3468786985053,46.0789574593663));
#26672=CARTESIAN_POINT('Ctrl Pts',(42.6070985618807,34.3449365433872,46.0819404596966));
#26673=CARTESIAN_POINT('Ctrl Pts',(42.6243020729385,34.3438384305827,46.0838760896714));
#26674=CARTESIAN_POINT('Ctrl Pts',(42.6846920885585,34.3400104591402,46.0914953052686));
#26675=CARTESIAN_POINT('Ctrl Pts',(42.7277122577768,34.3373316629538,46.0984098926137));
#26676=CARTESIAN_POINT('Ctrl Pts',(42.8979650741293,34.3267943054036,46.131724777663));
#26677=CARTESIAN_POINT('Ctrl Pts',(43.0226210813281,34.319200828351,46.1694900570796));
#26678=CARTESIAN_POINT('Ctrl Pts',(43.2135143751342,34.3066600068771,46.2491000313097));
#26679=CARTESIAN_POINT('Ctrl Pts',(43.2826496305194,34.3019143930515,46.282914128506));
#26680=CARTESIAN_POINT('Ctrl Pts',(43.3648896758272,34.2959043319797,46.3294192913414));
#26681=CARTESIAN_POINT('Ctrl Pts',(43.3800822120019,34.294778212502,46.3382867830182));
#26682=CARTESIAN_POINT('Ctrl Pts',(43.4039264307158,34.2929844244083,46.3526447831909));
#26683=CARTESIAN_POINT('Ctrl Pts',(43.4126595222887,34.2923217410566,46.3579987290396));
#26684=CARTESIAN_POINT('Ctrl Pts',(43.4288636403157,34.2910812537836,46.3681113331778));
#26685=CARTESIAN_POINT('Ctrl Pts',(43.436345364754,34.2905041115909,46.3728524062623));
#26686=CARTESIAN_POINT('Ctrl Pts',(43.452937656056,34.2892142194341,46.3835275869757));
#26687=CARTESIAN_POINT('Ctrl Pts',(43.4620311817534,34.2885005176829,46.3894874945066));
#26688=CARTESIAN_POINT('Ctrl Pts',(43.4885985306213,34.2863951060906,46.4072226214974));
#26689=CARTESIAN_POINT('Ctrl Pts',(43.5059299081967,34.284995532206,46.4192073139162));
#26690=CARTESIAN_POINT('Ctrl Pts',(43.5449147628843,34.2817861684991,46.4471203621731));
#26691=CARTESIAN_POINT('Ctrl Pts',(43.5664382155553,34.2799699909406,46.463221957552));
#26692=CARTESIAN_POINT('Ctrl Pts',(43.6377105715531,34.2738034232425,46.5189004658649));
#26693=CARTESIAN_POINT('Ctrl Pts',(43.685834317894,34.2693803966815,46.5604820103819));
#26694=CARTESIAN_POINT('Ctrl Pts',(43.8164074579208,34.2566491297421,46.6850836931713));
#26695=CARTESIAN_POINT('Ctrl Pts',(43.8934820205152,34.248209175436,46.7733277084184));
#26696=CARTESIAN_POINT('Ctrl Pts',(43.9960217720389,34.2358812936198,46.9148268861911));
#26697=CARTESIAN_POINT('Ctrl Pts',(44.027833738085,34.2318585489961,46.9631562856298));
#26698=CARTESIAN_POINT('Ctrl Pts',(44.0625315462494,34.227284725118,47.0214138525988));
#26699=CARTESIAN_POINT('Ctrl Pts',(44.0675677480391,34.2266158074294,47.030020718664));
#26700=CARTESIAN_POINT('Ctrl Pts',(44.0756632346923,34.2255326904695,47.0441053224634));
#26701=CARTESIAN_POINT('Ctrl Pts',(44.0787628613103,34.2251160483018,47.0495594869302));
#26702=CARTESIAN_POINT('Ctrl Pts',(44.0842723809218,34.2243721102896,47.0593651904989));
#26703=CARTESIAN_POINT('Ctrl Pts',(44.0866920942789,34.2240442009699,47.0637110067902));
#26704=CARTESIAN_POINT('Ctrl Pts',(44.0919770294843,34.2233253979913,47.0732897546476));
#26705=CARTESIAN_POINT('Ctrl Pts',(44.0948347989453,34.2229349764343,47.0785266396701));
#26706=CARTESIAN_POINT('Ctrl Pts',(44.1030234076882,34.2218109574066,47.0936992974386));
#26707=CARTESIAN_POINT('Ctrl Pts',(44.1082915996159,34.2210811921113,47.1036688580291));
#26708=CARTESIAN_POINT('Ctrl Pts',(44.1500506195605,34.2152376746012,47.1843995987182));
#26709=CARTESIAN_POINT('Ctrl Pts',(44.1822211566163,34.2103638776719,47.2573209482297));
#26710=CARTESIAN_POINT('Ctrl Pts',(44.2261060932149,34.2027279359412,47.3762227334435));
#26711=CARTESIAN_POINT('Ctrl Pts',(44.2407929808769,34.1999194035777,47.4209983456804));
#26712=CARTESIAN_POINT('Ctrl Pts',(44.2901736097783,34.1892744357211,47.5925132829831));
#26713=CARTESIAN_POINT('Ctrl Pts',(44.3135261446433,34.181431994643,47.7221257827038));
#26714=CARTESIAN_POINT('Ctrl Pts',(44.3254635815525,34.1715483270752,47.8784343190382));
#26715=CARTESIAN_POINT('Ctrl Pts',(44.3268976819529,34.1699320239683,47.9038051682644));
#26716=CARTESIAN_POINT('Ctrl Pts',(44.3282553253072,34.1675562038338,47.9407706925516));
#26717=CARTESIAN_POINT('Ctrl Pts',(44.3285761737111,34.1668091025453,47.9523487356526));
#26718=CARTESIAN_POINT('Ctrl Pts',(44.3289601657586,34.1654786114553,47.9728814676753));
#26719=CARTESIAN_POINT('Ctrl Pts',(44.3290652575292,34.1648965533401,47.9818351016017));
#26720=CARTESIAN_POINT('Ctrl Pts',(44.3291543594468,34.1636793767602,48.000496218967));
#26721=CARTESIAN_POINT('Ctrl Pts',(44.3291274379879,34.1630439317222,48.0102034778088));
#26722=CARTESIAN_POINT('Ctrl Pts',(44.3288662832867,34.1613814427322,48.0355061024532));
#26723=CARTESIAN_POINT('Ctrl Pts',(44.3285161806463,34.1603507993887,48.0510993021979));
#26724=CARTESIAN_POINT('Ctrl Pts',(44.3260644755211,34.1556369434249,48.1219810445436));
#26725=CARTESIAN_POINT('Ctrl Pts',(44.3217741909449,34.1518861599262,48.1771627790495));
#26726=CARTESIAN_POINT('Ctrl Pts',(44.3023561440426,34.1407520101972,48.3374004372218));
#26727=CARTESIAN_POINT('Ctrl Pts',(44.2809280236383,34.133202004805,48.4414783396028));
#26728=CARTESIAN_POINT('Ctrl Pts',(44.2215524234029,34.1181391953374,48.6437914149364));
#26729=CARTESIAN_POINT('Ctrl Pts',(44.1839023151928,34.1106540765545,48.7417664032641));
#26730=CARTESIAN_POINT('Ctrl Pts',(44.1313511312328,34.1024004279503,48.8510206023347));
#26731=CARTESIAN_POINT('Ctrl Pts',(44.1240359668639,34.1012904341845,48.8657440928809));
#26732=CARTESIAN_POINT('Ctrl Pts',(44.113589698086,34.0997599475827,48.8861120163784));
#26733=CARTESIAN_POINT('Ctrl Pts',(44.1106173914101,34.0993303610339,48.8918364772232));
#26734=CARTESIAN_POINT('Ctrl Pts',(44.1054417204342,34.0985925176906,48.9016833934746));
#26735=CARTESIAN_POINT('Ctrl Pts',(44.1032520046775,34.098283426285,48.9058129020926));
#26736=CARTESIAN_POINT('Ctrl Pts',(44.0986036244992,34.0976337827002,48.914502664616));
#26737=CARTESIAN_POINT('Ctrl Pts',(44.0961415605915,34.0972934601029,48.9190610449175));
#26738=CARTESIAN_POINT('Ctrl Pts',(44.0899937586306,34.0964528030713,48.9303345249455));
#26739=CARTESIAN_POINT('Ctrl Pts',(44.0862862822213,34.0959538332971,48.9370377856661));
#26740=CARTESIAN_POINT('Ctrl Pts',(44.0722024681212,34.094087407084,48.9621475556392));
#26741=CARTESIAN_POINT('Ctrl Pts',(44.0615634464517,34.0927356551824,48.9804060462587));
#26742=CARTESIAN_POINT('Ctrl Pts',(43.9758500720868,34.0822583505986,49.1221011685673));
#26743=CARTESIAN_POINT('Ctrl Pts',(43.8874148799443,34.0738188392439,49.2369408846394));
#26744=CARTESIAN_POINT('Ctrl Pts',(43.7106633216603,34.0585919388743,49.4197740122959));
#26745=CARTESIAN_POINT('Ctrl Pts',(43.6277647783039,34.0519264285021,49.4920407261029));
#26746=CARTESIAN_POINT('Ctrl Pts',(43.525420231481,34.0438709979065,49.5669277164846));
#26747=CARTESIAN_POINT('Ctrl Pts',(43.5115301556426,34.0427815018497,49.5768112916504));
#26748=CARTESIAN_POINT('Ctrl Pts',(43.4884581062062,34.0409768927757,49.5927720144369));
#26749=CARTESIAN_POINT('Ctrl Pts',(43.4793516640338,34.0402659023675,49.5989570713383));
#26750=CARTESIAN_POINT('Ctrl Pts',(43.462815903176,34.0389768988408,49.6099824617884));
#26751=CARTESIAN_POINT('Ctrl Pts',(43.4554051507959,34.0383999398061,49.6148501895122));
#26752=CARTESIAN_POINT('Ctrl Pts',(43.4394457314425,34.0371588402641,49.6251762976705));
#26753=CARTESIAN_POINT('Ctrl Pts',(43.4308870772458,34.0364941248507,49.6306186722871));
#26754=CARTESIAN_POINT('Ctrl Pts',(43.4073641967515,34.0346692984092,49.645317457184));
#26755=CARTESIAN_POINT('Ctrl Pts',(43.3923159207897,34.0335041938853,49.6544368341254));
#26756=CARTESIAN_POINT('Ctrl Pts',(43.3040973561307,34.0266852062186,49.7062614211115));
#26757=CARTESIAN_POINT('Ctrl Pts',(43.2283122551228,34.0208657820593,49.7443094033136));
#26758=CARTESIAN_POINT('Ctrl Pts',(43.0442965321068,34.0068456735775,49.8219932047957));
#26759=CARTESIAN_POINT('Ctrl Pts',(42.934524557441,33.9985578098691,49.8571639739744));
#26760=CARTESIAN_POINT('Ctrl Pts',(42.7874137792579,33.9878622838169,49.8901667252651));
#26761=CARTESIAN_POINT('Ctrl Pts',(42.7523312915999,33.9853429822515,49.8970193922127));
#26762=CARTESIAN_POINT('Ctrl Pts',(42.6796802841621,33.9802135813446,49.9091251551202));
#26763=CARTESIAN_POINT('Ctrl Pts',(42.6421046813481,33.977608306934,49.9142533009877));
#26764=CARTESIAN_POINT('Ctrl Pts',(42.5946572175901,33.9743977082551,49.9193090201219));
#26765=CARTESIAN_POINT('Ctrl Pts',(42.5849068868708,33.9737421302353,49.9202728973442));
#26766=CARTESIAN_POINT('Ctrl Pts',(42.5695246532774,33.9727149284583,49.9216752715797));
#26767=CARTESIAN_POINT('Ctrl Pts',(42.5638976063124,33.9723406470981,49.9221633734295));
#26768=CARTESIAN_POINT('Ctrl Pts',(42.5532649692532,33.9716363255582,49.923038639793));
#26769=CARTESIAN_POINT('Ctrl Pts',(42.5482600526952,33.971306020113,49.923430975703));
#26770=CARTESIAN_POINT('Ctrl Pts',(42.5365205609455,33.9705340550481,49.9243051413645));
#26771=CARTESIAN_POINT('Ctrl Pts',(42.5297849179846,33.9700932804375,49.9247711601863));
#26772=CARTESIAN_POINT('Ctrl Pts',(42.5077366134428,33.9686570758189,49.9261803497274));
#26773=CARTESIAN_POINT('Ctrl Pts',(42.4924146729377,33.9676694564246,49.9269762534963));
#26774=CARTESIAN_POINT('Ctrl Pts',(42.407601478846,33.9622522050573,49.9303679329371));
#26775=CARTESIAN_POINT('Ctrl Pts',(42.338011332789,33.9579906248667,49.9293878959466));
#26776=CARTESIAN_POINT('Ctrl Pts',(42.2558673635155,33.9530216921476,49.9237805773473));
#26777=CARTESIAN_POINT('Ctrl Pts',(42.2431242641098,33.9522526453641,49.9227833825839));
#26778=CARTESIAN_POINT('Ctrl Pts',(42.0879226409082,33.942898762641,49.9090850916708));
#26779=CARTESIAN_POINT('Ctrl Pts',(41.9473024329846,33.934513571059,49.8807077063168));
#26780=CARTESIAN_POINT('Ctrl Pts',(41.8054451023481,33.9252876654991,49.83523361896));
#26781=CARTESIAN_POINT('Ctrl Pts',(41.7997875373724,33.9249184736924,49.8333911083169));
#26782=CARTESIAN_POINT('Ctrl Pts',(41.7941388307093,33.9245485747014,49.8315225361556));
#26783=CARTESIAN_POINT('Origin',(42.4,48.4493818343519,48.));
#26784=CARTESIAN_POINT('',(41.7941388318293,32.9600825139687,49.8315225365261));
#26785=CARTESIAN_POINT('',(41.7941386107368,33.1302767167271,49.8315224633894));
#26786=CARTESIAN_POINT('',(41.7941388317924,48.4493818343519,49.8315225365138));
#26787=CARTESIAN_POINT('',(40.4708700098857,33.595812472054,47.9998047017072));
#26788=CARTESIAN_POINT('Ctrl Pts',(41.7941388318293,32.9600825139687,49.8315225365261));
#26789=CARTESIAN_POINT('Ctrl Pts',(41.7953186904234,32.9601663481406,49.8319128295701));
#26790=CARTESIAN_POINT('Ctrl Pts',(41.7964989385408,32.96025012569,49.8323019866228));
#26791=CARTESIAN_POINT('Ctrl Pts',(41.8074347217258,32.9610255945063,49.8358960726686));
#26792=CARTESIAN_POINT('Ctrl Pts',(41.8172155782641,32.9617133763165,49.8390242869177));
#26793=CARTESIAN_POINT('Ctrl Pts',(41.8325719318299,32.9627836727442,49.8438008937735));
#26794=CARTESIAN_POINT('Ctrl Pts',(41.8381305218923,32.9631691422879,49.8455023815245));
#26795=CARTESIAN_POINT('Ctrl Pts',(41.8484292519326,32.963879613329,49.8486039852025));
#26796=CARTESIAN_POINT('Ctrl Pts',(41.853167063099,32.9642049968126,49.8500110064993));
#26797=CARTESIAN_POINT('Ctrl Pts',(41.8641032042128,32.9649527583359,49.8532131069759));
#26798=CARTESIAN_POINT('Ctrl Pts',(41.8703051771815,32.9653743871948,49.8549953081474));
#26799=CARTESIAN_POINT('Ctrl Pts',(41.8897094124839,32.9666862959985,49.8604660633937));
#26800=CARTESIAN_POINT('Ctrl Pts',(41.9029424657429,32.9675705193253,49.8640451417003));
#26801=CARTESIAN_POINT('Ctrl Pts',(41.934163780273,32.969634628917,49.872133282967));
#26802=CARTESIAN_POINT('Ctrl Pts',(41.9521813974567,32.9708086936235,49.8765247044895));
#26803=CARTESIAN_POINT('Ctrl Pts',(42.0173909704829,32.9750055970131,49.8914254355859));
#26804=CARTESIAN_POINT('Ctrl Pts',(42.0649132838724,32.9779661704232,49.9004203193478));
#26805=CARTESIAN_POINT('Ctrl Pts',(42.2701120368626,32.9905209442041,49.9313217360774));
#26806=CARTESIAN_POINT('Ctrl Pts',(42.4298198635288,32.9997730285489,49.9354550882161));
#26807=CARTESIAN_POINT('Ctrl Pts',(42.6337471679586,33.0124489288368,49.9154626299033));
#26808=CARTESIAN_POINT('Ctrl Pts',(42.6790939757978,33.0153187514563,49.9093823248533));
#26809=CARTESIAN_POINT('Ctrl Pts',(42.7390826266652,33.0192044457541,49.8991561530089));
#26810=CARTESIAN_POINT('Ctrl Pts',(42.7539552427885,33.0201751233684,49.8964405569936));
#26811=CARTESIAN_POINT('Ctrl Pts',(42.7782215459435,33.0217715719931,49.8917143726683));
#26812=CARTESIAN_POINT('Ctrl Pts',(42.7876350334175,33.0223940088909,49.8898078952314));
#26813=CARTESIAN_POINT('Ctrl Pts',(42.8058355595821,33.0236037187869,49.88598010434));
#26814=CARTESIAN_POINT('Ctrl Pts',(42.8146241848908,33.0241906990608,49.8840674712064));
#26815=CARTESIAN_POINT('Ctrl Pts',(42.8351429601558,33.0255679193441,49.8794515321867));
#26816=CARTESIAN_POINT('Ctrl Pts',(42.8468617121143,33.0263596998118,49.8766997779757));
#26817=CARTESIAN_POINT('Ctrl Pts',(42.8850194248434,33.0289553197575,49.8673620680394));
#26818=CARTESIAN_POINT('Ctrl Pts',(42.9113437233241,33.0307735580331,49.8603258861709));
#26819=CARTESIAN_POINT('Ctrl Pts',(42.9734838867121,33.0351335756086,49.8422979954103));
#26820=CARTESIAN_POINT('Ctrl Pts',(43.0091448939716,33.0376902351268,49.8308161715355));
#26821=CARTESIAN_POINT('Ctrl Pts',(43.1483926194421,33.0478895167737,49.7814637033356));
#26822=CARTESIAN_POINT('Ctrl Pts',(43.2489772839104,33.0557523263012,49.7357813889152));
#26823=CARTESIAN_POINT('Ctrl Pts',(43.4315226840048,33.0707100241287,49.6331967620152));
#26824=CARTESIAN_POINT('Ctrl Pts',(43.5140842262934,33.077776278928,49.5780338907871));
#26825=CARTESIAN_POINT('Ctrl Pts',(43.6050026831629,33.0856492456122,49.506579795194));
#26826=CARTESIAN_POINT('Ctrl Pts',(43.6178294314941,33.0867620416732,49.496230485587));
#26827=CARTESIAN_POINT('Ctrl Pts',(43.6354959037276,33.0882958077293,49.4815985053386));
#26828=CARTESIAN_POINT('Ctrl Pts',(43.6404486907668,33.0887259199215,49.4774543335341));
#26829=CARTESIAN_POINT('Ctrl Pts',(43.6489522536572,33.0894644614497,49.4702661990964));
#26830=CARTESIAN_POINT('Ctrl Pts',(43.6525129035598,33.0897737286028,49.4672340834742));
#26831=CARTESIAN_POINT('Ctrl Pts',(43.6599945078234,33.0904235385697,49.4608159483897));
#26832=CARTESIAN_POINT('Ctrl Pts',(43.6639129112251,33.090763852916,49.4574270303344));
#26833=CARTESIAN_POINT('Ctrl Pts',(43.6735864582969,33.0916041003394,49.4489922948326));
#26834=CARTESIAN_POINT('Ctrl Pts',(43.6793253923399,33.0921026726923,49.4439278661354));
#26835=CARTESIAN_POINT('Ctrl Pts',(43.7007525059521,33.0939651711712,49.4247910772649));
#26836=CARTESIAN_POINT('Ctrl Pts',(43.7162405514744,33.0953134812532,49.4104955138197));
#26837=CARTESIAN_POINT('Ctrl Pts',(43.8352730273186,33.1057215945155,49.2969592282737));
#26838=CARTESIAN_POINT('Ctrl Pts',(43.9277054657483,33.114104716562,49.186692474482));
#26839=CARTESIAN_POINT('Ctrl Pts',(44.0684071870154,33.129330097107,48.9748105176583));
#26840=CARTESIAN_POINT('Ctrl Pts',(44.1216618013576,33.1360583872588,48.8773334182646));
#26841=CARTESIAN_POINT('Ctrl Pts',(44.1731093514986,33.1441841280524,48.7602084695542));
#26842=CARTESIAN_POINT('Ctrl Pts',(44.1797636101396,33.145274588024,48.7444965760592));
#26843=CARTESIAN_POINT('Ctrl Pts',(44.1903691091641,33.1470805903501,48.7185000605846));
#26844=CARTESIAN_POINT('Ctrl Pts',(44.1944423039464,33.1477920010868,48.7082659765924));
#26845=CARTESIAN_POINT('Ctrl Pts',(44.2016367961264,33.1490816338544,48.689728992555));
#26846=CARTESIAN_POINT('Ctrl Pts',(44.2047889167095,33.1496587996724,48.6814383244502));
#26847=CARTESIAN_POINT('Ctrl Pts',(44.2114232035588,33.150900198946,48.663619946832));
#26848=CARTESIAN_POINT('Ctrl Pts',(44.2148876040374,33.1515650065902,48.6540859532607));
#26849=CARTESIAN_POINT('Ctrl Pts',(44.2241542407218,33.1533897162905,48.6279437516083));
#26850=CARTESIAN_POINT('Ctrl Pts',(44.2298046190934,33.1545546082354,48.6112831341076));
#26851=CARTESIAN_POINT('Ctrl Pts',(44.2612933771678,33.1613640205664,48.5140849419269));
#26852=CARTESIAN_POINT('Ctrl Pts',(44.2820370660458,33.1671734954347,48.4320061139792));
#26853=CARTESIAN_POINT('Ctrl Pts',(44.3179971184581,33.1811309907199,48.2364212826673));
#26854=CARTESIAN_POINT('Ctrl Pts',(44.3286331670262,33.1893639050772,48.1223901988786));
#26855=CARTESIAN_POINT('Ctrl Pts',(44.3293184578406,33.2009469725281,47.9591607664161));
#26856=CARTESIAN_POINT('Ctrl Pts',(44.3276616290696,33.2043904701352,47.9102289745482));
#26857=CARTESIAN_POINT('Ctrl Pts',(44.3221671059239,33.2096670442245,47.8339444162044));
#26858=CARTESIAN_POINT('Ctrl Pts',(44.3196008534083,33.211545062821,47.8065223693508));
#26859=CARTESIAN_POINT('Ctrl Pts',(44.3154446220935,33.2139825251905,47.7704541251514));
#26860=CARTESIAN_POINT('Ctrl Pts',(44.3143816983917,33.2145680886297,47.7617519589095));
#26861=CARTESIAN_POINT('Ctrl Pts',(44.312565460166,33.2155105616394,47.7476801410565));
#26862=CARTESIAN_POINT('Ctrl Pts',(44.3118487806834,33.2158694557297,47.742306010448));
#26863=CARTESIAN_POINT('Ctrl Pts',(44.3104126404319,33.2165640847963,47.7318727713187));
#26864=CARTESIAN_POINT('Ctrl Pts',(44.3096957252774,33.2168999481932,47.7268134245772));
#26865=CARTESIAN_POINT('Ctrl Pts',(44.3079069675801,33.2177123768437,47.714541188286));
#26866=CARTESIAN_POINT('Ctrl Pts',(44.3068143001939,33.2181877795474,47.707331315447));
#26867=CARTESIAN_POINT('Ctrl Pts',(44.3027885625952,33.2198685171367,47.6817478591484));
#26868=CARTESIAN_POINT('Ctrl Pts',(44.2996304879592,33.2210619116883,47.6634100264469));
#26869=CARTESIAN_POINT('Ctrl Pts',(44.2911018851939,33.2240057298827,47.6178396992821));
#26870=CARTESIAN_POINT('Ctrl Pts',(44.2854079298247,33.2257412685869,47.590671361096));
#26871=CARTESIAN_POINT('Ctrl Pts',(44.2577342328735,33.233305196498,47.471499711805));
#26872=CARTESIAN_POINT('Ctrl Pts',(44.2295903638975,33.2389211727187,47.3810566933012));
#26873=CARTESIAN_POINT('Ctrl Pts',(44.1492324289635,33.2520011945866,47.1770340505047));
#26874=CARTESIAN_POINT('Ctrl Pts',(44.0924104824532,33.259468182306,47.0657469356983));
#26875=CARTESIAN_POINT('Ctrl Pts',(44.011507463395,33.2689353248774,46.9392279370948));
#26876=CARTESIAN_POINT('Ctrl Pts',(43.9973361392626,33.2705583094985,46.9180060837714));
#26877=CARTESIAN_POINT('Ctrl Pts',(43.9761144432601,33.2729422803106,46.8875520389554));
#26878=CARTESIAN_POINT('Ctrl Pts',(43.9693946658616,33.2736907307929,46.878091992469));
#26879=CARTESIAN_POINT('Ctrl Pts',(43.9573358549892,33.2750229145319,46.8614360508531));
#26880=CARTESIAN_POINT('Ctrl Pts',(43.9520312193295,33.2756053063924,46.8542155869397));
#26881=CARTESIAN_POINT('Ctrl Pts',(43.9408779912796,33.2768224642894,46.8392538162203));
#26882=CARTESIAN_POINT('Ctrl Pts',(43.9350209236629,33.2774575520803,46.8315191720671));
#26883=CARTESIAN_POINT('Ctrl Pts',(43.9196164281323,33.2791175132561,46.8114922309382));
#26884=CARTESIAN_POINT('Ctrl Pts',(43.9099782965825,33.2801459639018,46.7992709192493));
#26885=CARTESIAN_POINT('Ctrl Pts',(43.8656534700592,33.2848316080301,46.7444440242126));
#26886=CARTESIAN_POINT('Ctrl Pts',(43.8293073318363,33.2885553696674,46.7032192061571));
#26887=CARTESIAN_POINT('Ctrl Pts',(43.6663871739683,33.3047738978995,46.5336111420908));
#26888=CARTESIAN_POINT('Ctrl Pts',(43.5239437738078,33.317925218574,46.4217836072068));
#26889=CARTESIAN_POINT('Ctrl Pts',(43.3319841340414,33.3334264671964,46.3104176019223));
#26890=CARTESIAN_POINT('Ctrl Pts',(43.2952246908517,33.3363007122261,46.2906561343631));
#26891=CARTESIAN_POINT('Ctrl Pts',(43.2488954268112,33.3397832980558,46.2676550381549));
#26892=CARTESIAN_POINT('Ctrl Pts',(43.2399058684298,33.3404526620956,46.2632787629403));
#26893=CARTESIAN_POINT('Ctrl Pts',(43.2256918169036,33.3415005546835,46.2564952940968));
#26894=CARTESIAN_POINT('Ctrl Pts',(43.2204900386621,33.3418818467267,46.254041313601));
#26895=CARTESIAN_POINT('Ctrl Pts',(43.2112003227081,33.3425587798449,46.2497095015205));
#26896=CARTESIAN_POINT('Ctrl Pts',(43.2071168009612,33.3428549607239,46.2478227079271));
#26897=CARTESIAN_POINT('Ctrl Pts',(43.1973022454277,33.3435635487638,46.2433294781586));
#26898=CARTESIAN_POINT('Ctrl Pts',(43.1915650142085,33.3439751101778,46.2407367951565));
#26899=CARTESIAN_POINT('Ctrl Pts',(43.1740398741993,33.3452245179412,46.2329201858732));
#26900=CARTESIAN_POINT('Ctrl Pts',(43.16221191232,33.346057104507,46.2277861814108));
#26901=CARTESIAN_POINT('Ctrl Pts',(43.1345489394738,33.3479816503892,46.2161070783065));
#26902=CARTESIAN_POINT('Ctrl Pts',(43.1186762272578,33.3490688069227,46.2096534902874));
#26903=CARTESIAN_POINT('Ctrl Pts',(43.0627827297541,33.352844497365,46.1877912571463));
#26904=CARTESIAN_POINT('Ctrl Pts',(43.0223339327698,33.3554834718571,46.1735054237523));
#26905=CARTESIAN_POINT('Ctrl Pts',(42.8587376015324,33.3659112582664,46.1217927081223));
#26906=CARTESIAN_POINT('Ctrl Pts',(42.7324604371075,33.3734346525349,46.095380584877));
#26907=CARTESIAN_POINT('Ctrl Pts',(42.5259986634939,33.386011197573,46.0733713862907));
#26908=CARTESIAN_POINT('Ctrl Pts',(42.447076264542,33.3908773958595,46.069830296513));
#26909=CARTESIAN_POINT('Ctrl Pts',(42.3504620928467,33.3970232202314,46.0714248713425));
#26910=CARTESIAN_POINT('Ctrl Pts',(42.3327646551156,33.3981565380207,46.0719607353575));
#26911=CARTESIAN_POINT('Ctrl Pts',(42.3048161975778,33.399959360026,46.073192251241));
#26912=CARTESIAN_POINT('Ctrl Pts',(42.2945587777466,33.4006237948302,46.0737263437411));
#26913=CARTESIAN_POINT('Ctrl Pts',(42.2754639641827,33.4018660707545,46.074873562242));
#26914=CARTESIAN_POINT('Ctrl Pts',(42.2666255449576,33.4024432366123,46.0754656989546));
#26915=CARTESIAN_POINT('Ctrl Pts',(42.2469768074779,33.4037312719323,46.0769180831016));
#26916=CARTESIAN_POINT('Ctrl Pts',(42.2361691005566,33.4044430779363,46.0778086503261));
#26917=CARTESIAN_POINT('Ctrl Pts',(42.2045327668332,33.4065367224479,46.0806842674953));
#26918=CARTESIAN_POINT('Ctrl Pts',(42.183728797864,33.4079262900342,46.0829170522529));
#26919=CARTESIAN_POINT('Ctrl Pts',(42.0420094291098,33.4174830506306,46.1004632009105));
#26920=CARTESIAN_POINT('Ctrl Pts',(41.9227661322724,33.4260031163009,46.1268648298564));
#26921=CARTESIAN_POINT('Ctrl Pts',(41.6759944079796,33.4444698487727,46.2066056006236));
#26922=CARTESIAN_POINT('Ctrl Pts',(41.5500470341744,33.4544091234816,46.2627513858675));
#26923=CARTESIAN_POINT('Ctrl Pts',(41.4184457887428,33.4647425956015,46.3391841860948));
#26924=CARTESIAN_POINT('Ctrl Pts',(41.40584203483,33.4657313362626,46.3466979073526));
#26925=CARTESIAN_POINT('Ctrl Pts',(41.3876202688925,33.467158095573,46.3578445398051));
#26926=CARTESIAN_POINT('Ctrl Pts',(41.3819338365237,33.4676029528798,46.3613638092927));
#26927=CARTESIAN_POINT('Ctrl Pts',(41.3721489303378,33.4683676108035,46.3674901754991));
#26928=CARTESIAN_POINT('Ctrl Pts',(41.3680418239031,33.4686883108822,46.370083292477));
#26929=CARTESIAN_POINT('Ctrl Pts',(41.3600178312467,33.4693143027092,46.3751919148607));
#26930=CARTESIAN_POINT('Ctrl Pts',(41.3561002351077,33.4696196825899,46.377706097262));
#26931=CARTESIAN_POINT('Ctrl Pts',(41.3475959602797,33.4702821384447,46.3832074178879));
#26932=CARTESIAN_POINT('Ctrl Pts',(41.3430127999091,33.4706388593795,46.3861999575491));
#26933=CARTESIAN_POINT('Ctrl Pts',(41.3242429816438,33.4720988375252,46.3985698311004));
#26934=CARTESIAN_POINT('Ctrl Pts',(41.3101673588831,33.4731914889035,46.4081153902553));
#26935=CARTESIAN_POINT('Ctrl Pts',(41.2760412776411,33.4758400445203,46.4319232608155));
#26936=CARTESIAN_POINT('Ctrl Pts',(41.256133482745,33.4773846325138,46.4463857051398));
#26937=CARTESIAN_POINT('Ctrl Pts',(41.175722009438,33.4836459561585,46.5071861728937));
#26938=CARTESIAN_POINT('Ctrl Pts',(41.1177090026685,33.4882182505514,46.556711637405));
#26939=CARTESIAN_POINT('Ctrl Pts',(40.954639900109,33.5017301648309,46.7135378804928));
#26940=CARTESIAN_POINT('Ctrl Pts',(40.8590178068249,33.5106056928517,46.8297782824284));
#26941=CARTESIAN_POINT('Ctrl Pts',(40.7645757458919,33.5216183625093,46.9765109416924));
#26942=CARTESIAN_POINT('Ctrl Pts',(40.7517148550166,33.5231772809653,46.9973543309314));
#26943=CARTESIAN_POINT('Ctrl Pts',(40.7334455663328,33.5254842412462,47.0282648380315));
#26944=CARTESIAN_POINT('Ctrl Pts',(40.7277239229533,33.5262208849937,47.0381446999251));
#26945=CARTESIAN_POINT('Ctrl Pts',(40.7176825507375,33.5275395657983,47.0558441064268));
#26946=CARTESIAN_POINT('Ctrl Pts',(40.7133287693741,33.5281203544738,47.063644027769));
#26947=CARTESIAN_POINT('Ctrl Pts',(40.7043163397013,33.5293419064085,47.0800568697133));
#26948=CARTESIAN_POINT('Ctrl Pts',(40.6996687951179,33.5299830457604,47.0886755646507));
#26949=CARTESIAN_POINT('Ctrl Pts',(40.6876115585847,33.5316764808529,47.1114485801996));
#26950=CARTESIAN_POINT('Ctrl Pts',(40.6803118643439,33.5327326256403,47.1256599690234));
#26951=CARTESIAN_POINT('Ctrl Pts',(40.6465937002536,33.537762133512,47.1933601627854));
#26952=CARTESIAN_POINT('Ctrl Pts',(40.6224917368732,33.5418147210434,47.2479597426087));
#26953=CARTESIAN_POINT('Ctrl Pts',(40.5315982645981,33.559234177284,47.4827631838862));
#26954=CARTESIAN_POINT('Ctrl Pts',(40.4894041321976,33.5733327954885,47.6712655305593));
#26955=CARTESIAN_POINT('Ctrl Pts',(40.4738280786925,33.5884426344774,47.8898403558821));
#26956=CARTESIAN_POINT('Ctrl Pts',(40.4724733640557,33.5902856073116,47.9168455301474));
#26957=CARTESIAN_POINT('Ctrl Pts',(40.4714386997071,33.5926726381177,47.9523919948821));
#26958=CARTESIAN_POINT('Ctrl Pts',(40.4712471664463,33.593241967605,47.9609138788479));
#26959=CARTESIAN_POINT('Ctrl Pts',(40.4710275626631,33.5941628232089,47.9747734582345));
#26960=CARTESIAN_POINT('Ctrl Pts',(40.4709651513888,33.5945161947454,47.9801103798958));
#26961=CARTESIAN_POINT('Ctrl Pts',(40.4708998108434,33.5950876399803,47.9887719463951));
#26962=CARTESIAN_POINT('Ctrl Pts',(40.4708833261889,33.5953064695646,47.992096331295));
#26963=CARTESIAN_POINT('Ctrl Pts',(40.4708719661489,33.5956207966647,47.9968821027511));
#26964=CARTESIAN_POINT('Ctrl Pts',(40.4708701578227,33.5957166803179,47.9983433992123));
#26965=CARTESIAN_POINT('Ctrl Pts',(40.4708700098857,33.595812472054,47.9998047017072));
#26966=CARTESIAN_POINT('Ctrl Pts',(40.4708700099162,33.5958124522899,47.9998044002066));
#26967=CARTESIAN_POINT('Ctrl Pts',(40.4708697946754,33.5959516095111,48.0019272426965));
#26968=CARTESIAN_POINT('Ctrl Pts',(40.470873083443,33.5960905727951,48.0040500985418));
#26969=CARTESIAN_POINT('Ctrl Pts',(40.4708990793297,33.5966216441967,48.0121741096659));
#26970=CARTESIAN_POINT('Ctrl Pts',(40.4709462852895,33.5970124153758,48.018175235026));
#26971=CARTESIAN_POINT('Ctrl Pts',(40.4712176332909,33.5984170233649,48.039825692079));
#26972=CARTESIAN_POINT('Ctrl Pts',(40.4716042156344,33.599422376138,48.0554728765029));
#26973=CARTESIAN_POINT('Ctrl Pts',(40.477090972764,33.6089007483902,48.2042121123139));
#26974=CARTESIAN_POINT('Ctrl Pts',(40.4957720003608,33.6167487655348,48.3364635187303));
#26975=CARTESIAN_POINT('Ctrl Pts',(40.5581542086279,33.6321720120768,48.5872065853432));
#26976=CARTESIAN_POINT('Ctrl Pts',(40.6001147342978,33.6397042286158,48.7054181231331));
#26977=CARTESIAN_POINT('Ctrl Pts',(40.6617330816396,33.6489138541125,48.8368827699757));
#26978=CARTESIAN_POINT('Ctrl Pts',(40.6705256046548,33.6501949526996,48.8549052097697));
#26979=CARTESIAN_POINT('Ctrl Pts',(40.6844225789574,33.6521724029519,48.8822983756932));
#26980=CARTESIAN_POINT('Ctrl Pts',(40.6893266662366,33.6528617368829,48.8917696165075));
#26981=CARTESIAN_POINT('Ctrl Pts',(40.6984047588779,33.6541228092482,48.9089516283029));
#26982=CARTESIAN_POINT('Ctrl Pts',(40.7025533012742,33.6546936324673,48.91667558488));
#26983=CARTESIAN_POINT('Ctrl Pts',(40.7117329755502,33.6559450662528,48.9334907445219));
#26984=CARTESIAN_POINT('Ctrl Pts',(40.7167851699566,33.6566264182588,48.9425700741526));
#26985=CARTESIAN_POINT('Ctrl Pts',(40.7309041500913,33.6585107104021,48.9674678409121));
#26986=CARTESIAN_POINT('Ctrl Pts',(40.7401220331586,33.6597190703504,48.9831988993021));
#26987=CARTESIAN_POINT('Ctrl Pts',(40.7964204122374,33.6669741954003,49.0762278874777));
#26988=CARTESIAN_POINT('Ctrl Pts',(40.8486634499625,33.6732105262355,49.1502541312575));
#26989=CARTESIAN_POINT('Ctrl Pts',(41.0080928153998,33.6909569061505,49.3454495183805));
#26990=CARTESIAN_POINT('Ctrl Pts',(41.1255898463136,33.7027390807372,49.4572293861175));
#26991=CARTESIAN_POINT('Ctrl Pts',(41.2745885857356,33.715446239185,49.5670180719793));
#26992=CARTESIAN_POINT('Ctrl Pts',(41.2937911710712,33.7170451371238,49.5806323541973));
#26993=CARTESIAN_POINT('Ctrl Pts',(41.3198330695504,33.7191571983177,49.5983884548569));
#26994=CARTESIAN_POINT('Ctrl Pts',(41.3264549837018,33.7196894766737,49.6028435212977));
#26995=CARTESIAN_POINT('Ctrl Pts',(41.3369754202764,33.7205273589121,49.6098269740103));
#26996=CARTESIAN_POINT('Ctrl Pts',(41.3408556649265,33.7208347381251,49.6123825296669));
#26997=CARTESIAN_POINT('Ctrl Pts',(41.3489363895087,33.7214713684119,49.6176627926158));
#26998=CARTESIAN_POINT('Ctrl Pts',(41.3531382849628,33.7218004518453,49.6203851931379));
#26999=CARTESIAN_POINT('Ctrl Pts',(41.3632499927675,33.7225878036512,49.6268808011352));
#27000=CARTESIAN_POINT('Ctrl Pts',(41.3691699455604,33.7230450365598,49.6306382557813));
#27001=CARTESIAN_POINT('Ctrl Pts',(41.3890007711875,33.7245647568971,49.6430739278929));
#27002=CARTESIAN_POINT('Ctrl Pts',(41.4030022151625,33.7256182730635,49.6516073483795));
#27003=CARTESIAN_POINT('Ctrl Pts',(41.496572606915,33.7325424930416,49.7070118121792));
#27004=CARTESIAN_POINT('Ctrl Pts',(41.5793201541263,33.7381168304548,49.7483018042725));
#27005=CARTESIAN_POINT('Ctrl Pts',(41.7072797968519,33.7463971195383,49.8010554698369));
#27006=CARTESIAN_POINT('Ctrl Pts',(41.750448339765,33.7491353965649,49.8170698772558));
#27007=CARTESIAN_POINT('Ctrl Pts',(41.7941388605861,33.7518842900812,49.8315225460387));
#27008=CARTESIAN_POINT('',(40.4708705770534,33.7661543955568,47.998507880119));
#27009=CARTESIAN_POINT('Ctrl Pts',(41.7941388307093,33.9245485747014,49.8315225361556));
#27010=CARTESIAN_POINT('Ctrl Pts',(41.7577101570787,33.9221630853456,49.8194720599174));
#27011=CARTESIAN_POINT('Ctrl Pts',(41.7216499126753,33.919747935102,49.8063376981226));
#27012=CARTESIAN_POINT('Ctrl Pts',(41.6721239936713,33.916342924668,49.7866063831014));
#27013=CARTESIAN_POINT('Ctrl Pts',(41.6583072392263,33.9153833094827,49.7809148426992));
#27014=CARTESIAN_POINT('Ctrl Pts',(41.6357568074188,33.9138004955479,49.7713177007099));
#27015=CARTESIAN_POINT('Ctrl Pts',(41.6269834246552,33.9131805208813,49.7675065552918));
#27016=CARTESIAN_POINT('Ctrl Pts',(41.6101671936861,33.9119839751127,49.7600524561992));
#27017=CARTESIAN_POINT('Ctrl Pts',(41.6021202830792,33.9114077496624,49.7564192163166));
#27018=CARTESIAN_POINT('Ctrl Pts',(41.5834579273818,33.9100627010319,49.7478383118413));
#27019=CARTESIAN_POINT('Ctrl Pts',(41.5728621269732,33.9092924530192,49.7428490036098));
#27020=CARTESIAN_POINT('Ctrl Pts',(41.5505418541287,33.9076556806712,49.7320895361342));
#27021=CARTESIAN_POINT('Ctrl Pts',(41.5388293080813,33.9067883757841,49.726296129811));
#27022=CARTESIAN_POINT('Ctrl Pts',(41.5073774945448,33.9044362483245,49.7103393033766));
#27023=CARTESIAN_POINT('Ctrl Pts',(41.4877538391498,33.9029437869971,49.699953629553));
#27024=CARTESIAN_POINT('Ctrl Pts',(41.4264463053549,33.898200848844,49.6661398347804));
#27025=CARTESIAN_POINT('Ctrl Pts',(41.3854542788225,33.8949099262014,49.6415008672024));
#27026=CARTESIAN_POINT('Ctrl Pts',(41.2664937755088,33.8850039734284,49.563838560819));
#27027=CARTESIAN_POINT('Ctrl Pts',(41.1914533101373,33.8782722009199,49.5065987327768));
#27028=CARTESIAN_POINT('Ctrl Pts',(41.1033473067491,33.8698656614669,49.4285602274032));
#27029=CARTESIAN_POINT('Ctrl Pts',(41.086076801076,33.8681918379977,49.4126918902211));
#27030=CARTESIAN_POINT('Ctrl Pts',(41.0101210583499,33.8607240253493,49.3403047716349));
#27031=CARTESIAN_POINT('Ctrl Pts',(40.9547550180589,33.8549855406866,49.2804102494003));
#27032=CARTESIAN_POINT('Ctrl Pts',(40.8967052463432,33.848772810804,49.2090318186555));
#27033=CARTESIAN_POINT('Ctrl Pts',(40.89013939599,33.8480670473135,49.2008222280647));
#27034=CARTESIAN_POINT('Ctrl Pts',(40.8796630087054,33.8469365137764,49.1875013239249));
#27035=CARTESIAN_POINT('Ctrl Pts',(40.8757104733839,33.8465089464433,49.1824235296359));
#27036=CARTESIAN_POINT('Ctrl Pts',(40.8687411854549,33.8457533265661,49.173377112424));
#27037=CARTESIAN_POINT('Ctrl Pts',(40.8657143283979,33.8454245750284,49.1694164720017));
#27038=CARTESIAN_POINT('Ctrl Pts',(40.859173633292,33.8447129445219,49.1607888651527));
#27039=CARTESIAN_POINT('Ctrl Pts',(40.8556656247062,33.8443304687488,49.1561176502947));
#27040=CARTESIAN_POINT('Ctrl Pts',(40.8457984003808,33.8432521375782,49.1428535420998));
#27041=CARTESIAN_POINT('Ctrl Pts',(40.8394891933334,33.8425596478857,49.1342234638338));
#27042=CARTESIAN_POINT('Ctrl Pts',(40.7979102660093,33.8379725222562,49.0763457873987));
#27043=CARTESIAN_POINT('Ctrl Pts',(40.7649013630548,33.8342161062244,49.0255075905095));
#27044=CARTESIAN_POINT('Ctrl Pts',(40.6716256790824,33.822957510933,48.8658624054197));
#27045=CARTESIAN_POINT('Ctrl Pts',(40.6194341382613,33.815681771896,48.7527172064729));
#27046=CARTESIAN_POINT('Ctrl Pts',(40.5583554019501,33.8044841936345,48.5776035394629));
#27047=CARTESIAN_POINT('Ctrl Pts',(40.5409769658268,33.8007472056475,48.5189538589396));
#27048=CARTESIAN_POINT('Ctrl Pts',(40.5183146786319,33.7948036316806,48.4265659547894));
#27049=CARTESIAN_POINT('Ctrl Pts',(40.5110906628393,33.7926555272956,48.3933439412882));
#27050=CARTESIAN_POINT('Ctrl Pts',(40.502227458627,33.7896146649027,48.3466763360272));
#27051=CARTESIAN_POINT('Ctrl Pts',(40.4998460770096,33.7887454647032,48.3333768956079));
#27052=CARTESIAN_POINT('Ctrl Pts',(40.4962212876742,33.7873326429179,48.3118311985335));
#27053=CARTESIAN_POINT('Ctrl Pts',(40.4948912812381,33.786791785299,48.3035998154362));
#27054=CARTESIAN_POINT('Ctrl Pts',(40.4923221345089,33.7856998811604,48.2870174053014));
#27055=CARTESIAN_POINT('Ctrl Pts',(40.4910843684486,33.7851488039661,48.2786663546546));
#27056=CARTESIAN_POINT('Ctrl Pts',(40.4886642909931,33.7840177823943,48.2615651444948));
#27057=CARTESIAN_POINT('Ctrl Pts',(40.4874871610685,33.783437687554,48.2528144652574));
#27058=CARTESIAN_POINT('Ctrl Pts',(40.4848931123223,33.7820860766254,48.2324746812769));
#27059=CARTESIAN_POINT('Ctrl Pts',(40.4835212601344,33.7813131583152,48.2208802799362));
#27060=CARTESIAN_POINT('Ctrl Pts',(40.4794041147951,33.7787897749827,48.1831516443121));
#27061=CARTESIAN_POINT('Ctrl Pts',(40.4770876389665,33.7770260544021,48.1569745700284));
#27062=CARTESIAN_POINT('Ctrl Pts',(40.4723157732544,33.7722574473275,48.0867358104789));
#27063=CARTESIAN_POINT('Ctrl Pts',(40.4708364529626,33.7692244710891,48.0426261768473));
#27064=CARTESIAN_POINT('Ctrl Pts',(40.4708705770534,33.7661543955568,47.998507880119));
#27065=CARTESIAN_POINT('Ctrl Pts',(40.470870575219,33.7661545607265,47.9985102536787));
#27066=CARTESIAN_POINT('Ctrl Pts',(40.4709446203108,33.7594822623403,47.9026264355607));
#27067=CARTESIAN_POINT('Ctrl Pts',(40.4781671589483,33.7526397519906,47.8068858209778));
#27068=CARTESIAN_POINT('Ctrl Pts',(40.5036561422422,33.7404401451449,47.6380137778734));
#27069=CARTESIAN_POINT('Ctrl Pts',(40.5191417216402,33.7350982340165,47.5646524109731));
#27070=CARTESIAN_POINT('Ctrl Pts',(40.5452646994695,33.7281964461131,47.4688759573871));
#27071=CARTESIAN_POINT('Ctrl Pts',(40.5521184949608,33.7265180951439,47.4455003667425));
#27072=CARTESIAN_POINT('Ctrl Pts',(40.5644675957776,33.7237106187548,47.4061581389536));
#27073=CARTESIAN_POINT('Ctrl Pts',(40.5697330027675,33.7225712662827,47.3901228569832));
#27074=CARTESIAN_POINT('Ctrl Pts',(40.577483951902,33.7209745010812,47.3675231131903));
#27075=CARTESIAN_POINT('Ctrl Pts',(40.5797957365942,33.7205076893603,47.3609004762885));
#27076=CARTESIAN_POINT('Ctrl Pts',(40.5838372432206,33.7197077696069,47.3495224832631));
#27077=CARTESIAN_POINT('Ctrl Pts',(40.5855496322938,33.7193736585046,47.3447610935809));
#27078=CARTESIAN_POINT('Ctrl Pts',(40.5891706845084,33.7186771656562,47.3348156176651));
#27079=CARTESIAN_POINT('Ctrl Pts',(40.5910828977674,33.7183149963777,47.3296329427092));
#27080=CARTESIAN_POINT('Ctrl Pts',(40.5962513020657,33.7173508128748,47.3158081571448));
#27081=CARTESIAN_POINT('Ctrl Pts',(40.5995473805147,33.7167511194016,47.3071809641446));
#27082=CARTESIAN_POINT('Ctrl Pts',(40.6144372449003,33.7141067638727,47.2690320626725));
#27083=CARTESIAN_POINT('Ctrl Pts',(40.6266967945813,33.712098505794,47.2397733921818));
#27084=CARTESIAN_POINT('Ctrl Pts',(40.6895788338157,33.702506035351,47.0995086561721));
#27085=CARTESIAN_POINT('Ctrl Pts',(40.749936364981,33.6953276008729,46.9931627861734));
#27086=CARTESIAN_POINT('Ctrl Pts',(40.8656691395636,33.6832711018941,46.8279401574051));
#27087=CARTESIAN_POINT('Ctrl Pts',(40.9153965532164,33.6784734587323,46.7655581759631));
#27088=CARTESIAN_POINT('Ctrl Pts',(40.9896583151381,33.6716224583645,46.6833971171577));
#27089=CARTESIAN_POINT('Ctrl Pts',(41.011032699567,33.6696830104915,46.6608672579265));
#27090=CARTESIAN_POINT('Ctrl Pts',(41.0494385482491,33.6662443569971,46.6222942784321));
#27091=CARTESIAN_POINT('Ctrl Pts',(41.0662357017407,33.6647550303344,46.6060265385081));
#27092=CARTESIAN_POINT('Ctrl Pts',(41.091531568693,33.6625307983258,46.5824037815255));
#27093=CARTESIAN_POINT('Ctrl Pts',(41.0998059447579,33.6618061048589,46.5748108601734));
#27094=CARTESIAN_POINT('Ctrl Pts',(41.1082996038705,33.6610649354082,46.56715224594));
#27095=CARTESIAN_POINT('Ctrl Pts',(41.1084532278421,33.6610515308523,46.5670137701275));
#27096=CARTESIAN_POINT('Ctrl Pts',(41.1086756462365,33.661032124901,46.5668133482176));
#27097=CARTESIAN_POINT('Ctrl Pts',(41.1087444228499,33.6610261243387,46.5667513823664));
#27098=CARTESIAN_POINT('Ctrl Pts',(41.1088890192633,33.6610135090956,46.5666211238009));
#27099=CARTESIAN_POINT('Ctrl Pts',(41.1089648402508,33.6610068943501,46.5665528319453));
#27100=CARTESIAN_POINT('Ctrl Pts',(41.1091244099496,33.6609929736928,46.5664091306749));
#27101=CARTESIAN_POINT('Ctrl Pts',(41.1092081596368,33.6609856677441,46.566333722775));
#27102=CARTESIAN_POINT('Ctrl Pts',(41.1093846143402,33.6609702751865,46.5661748716266));
#27103=CARTESIAN_POINT('Ctrl Pts',(41.1094773209908,33.6609621884952,46.5660914298952));
#27104=CARTESIAN_POINT('Ctrl Pts',(41.1096728932206,33.660945129651,46.5659154370968));
#27105=CARTESIAN_POINT('Ctrl Pts',(41.109775760615,33.6609361574151,46.5658228881514));
#27106=CARTESIAN_POINT('Ctrl Pts',(41.1099930718877,33.660917204076,46.5656274172961));
#27107=CARTESIAN_POINT('Ctrl Pts',(41.1101075181197,33.6609072228627,46.5655244980206));
#27108=CARTESIAN_POINT('Ctrl Pts',(41.116723669867,33.6603302363395,46.5595761531432));
#27109=CARTESIAN_POINT('Ctrl Pts',(41.1232649344167,33.6597613834462,46.5537750637779));
#27110=CARTESIAN_POINT('Ctrl Pts',(41.1374159057535,33.6585340503031,46.5413961696784));
#27111=CARTESIAN_POINT('Ctrl Pts',(41.14503804824,33.657874983064,46.5348330395502));
#27112=CARTESIAN_POINT('Ctrl Pts',(41.1658381770873,33.6560816395355,46.5172042440036));
#27113=CARTESIAN_POINT('Ctrl Pts',(41.1791132017874,33.6549426547532,46.5062550243418));
#27114=CARTESIAN_POINT('Ctrl Pts',(41.2446734677681,33.6493429744936,46.4536388030264));
#27115=CARTESIAN_POINT('Ctrl Pts',(41.2989484878609,33.644782300511,46.4145359965361));
#27116=CARTESIAN_POINT('Ctrl Pts',(41.4738054157305,33.6303150570237,46.3018733718941));
#27117=CARTESIAN_POINT('Ctrl Pts',(41.6005019610822,33.6201107085544,46.2386748087182));
#27118=CARTESIAN_POINT('Ctrl Pts',(41.7932950843798,33.6055762069179,46.1676273526643));
#27119=CARTESIAN_POINT('Ctrl Pts',(41.8547346921109,33.60108764539,46.1484147501434));
#27120=CARTESIAN_POINT('Ctrl Pts',(41.9275132984825,33.5960192286536,46.1295946377345));
#27121=CARTESIAN_POINT('Ctrl Pts',(41.938023881319,33.5952932350344,46.1269709074746));
#27122=CARTESIAN_POINT('Ctrl Pts',(41.9542653892263,33.5941811771665,46.1230616164485));
#27123=CARTESIAN_POINT('Ctrl Pts',(41.9599808148327,33.5937917021623,46.1217135048521));
#27124=CARTESIAN_POINT('Ctrl Pts',(41.9705560105203,33.5930746091724,46.1192700268231));
#27125=CARTESIAN_POINT('Ctrl Pts',(41.9754138581071,33.5927465964314,46.1181673875824));
#27126=CARTESIAN_POINT('Ctrl Pts',(41.9865154189666,33.5920001256666,46.1156927210258));
#27127=CARTESIAN_POINT('Ctrl Pts',(41.9927617207576,33.5915823662802,46.1143329012906));
#27128=CARTESIAN_POINT('Ctrl Pts',(42.0091580018697,33.5904913632957,46.1108487037066));
#27129=CARTESIAN_POINT('Ctrl Pts',(42.0193187109911,33.5898208845378,46.108775038394));
#27130=CARTESIAN_POINT('Ctrl Pts',(42.1007475426901,33.5844888223533,46.0928393477876));
#27131=CARTESIAN_POINT('Ctrl Pts',(42.1727385082922,33.58002594182,46.0829270902785));
#27132=CARTESIAN_POINT('Ctrl Pts',(42.3582149927332,33.5687805380094,46.0679883744019));
#27133=CARTESIAN_POINT('Ctrl Pts',(42.4718886470002,33.5621168448057,46.0688739277242));
#27134=CARTESIAN_POINT('Ctrl Pts',(42.6688548502872,33.5501567681826,46.0878322112025));
#27135=CARTESIAN_POINT('Ctrl Pts',(42.7522510928083,33.5449632010191,46.1014255062303));
#27136=CARTESIAN_POINT('Ctrl Pts',(42.851611688321,33.5384739952655,46.1243938266848));
#27137=CARTESIAN_POINT('Ctrl Pts',(42.8686851968918,33.5373481942929,46.1285872214407));
#27138=CARTESIAN_POINT('Ctrl Pts',(42.8955112093577,33.5355612644794,46.1355660368666));
#27139=CARTESIAN_POINT('Ctrl Pts',(42.9053034145217,33.5349051659131,46.1381960859865));
#27140=CARTESIAN_POINT('Ctrl Pts',(42.9236191949162,33.5336705837348,46.1432705862479));
#27141=CARTESIAN_POINT('Ctrl Pts',(42.9321475646179,33.5330927059163,46.1456968580571));
#27142=CARTESIAN_POINT('Ctrl Pts',(42.9512302314874,33.5317927472586,46.1512682535257));
#27143=CARTESIAN_POINT('Ctrl Pts',(42.961774861972,33.5310696441081,46.1544451147646));
#27144=CARTESIAN_POINT('Ctrl Pts',(42.9885856671546,33.529218608992,46.1627736697961));
#27145=CARTESIAN_POINT('Ctrl Pts',(43.0048114704977,33.5280865887297,46.1680511117441));
#27146=CARTESIAN_POINT('Ctrl Pts',(43.1262279158077,33.5195247487279,46.2093306625557));
#27147=CARTESIAN_POINT('Ctrl Pts',(43.2281819595729,33.5118003424118,46.2541447299368));
#27148=CARTESIAN_POINT('Ctrl Pts',(43.451303072693,33.4937554192538,46.3761770115563));
#27149=CARTESIAN_POINT('Ctrl Pts',(43.5688746615877,33.4833705861484,46.4586453551129));
#27150=CARTESIAN_POINT('Ctrl Pts',(43.6920322224882,33.4721274355821,46.5672967103158));
#27151=CARTESIAN_POINT('Ctrl Pts',(43.7075947682726,33.470700009798,46.5814859915852));
#27152=CARTESIAN_POINT('Ctrl Pts',(43.7284904768798,33.4687778459379,46.6011740165443));
#27153=CARTESIAN_POINT('Ctrl Pts',(43.7340272009866,33.46826798504,46.6064532619715));
#27154=CARTESIAN_POINT('Ctrl Pts',(43.7432591085678,33.4674171492287,46.615361295422));
#27155=CARTESIAN_POINT('Ctrl Pts',(43.7469713050219,33.46707483289,46.6189722376017));
#27156=CARTESIAN_POINT('Ctrl Pts',(43.7540076110993,33.466425700679,46.6258719818359));
#27157=CARTESIAN_POINT('Ctrl Pts',(43.7573343628105,33.4661186650114,46.6291579777673));
#27158=CARTESIAN_POINT('Ctrl Pts',(43.7652266711699,33.4653898581532,46.6370104955061));
#27159=CARTESIAN_POINT('Ctrl Pts',(43.769781348461,33.464968937699,46.6415879441911));
#27160=CARTESIAN_POINT('Ctrl Pts',(43.785879479902,33.4634796861801,46.6579298558259));
#27161=CARTESIAN_POINT('Ctrl Pts',(43.7972954420798,33.462420741738,46.6698196754207));
#27162=CARTESIAN_POINT('Ctrl Pts',(43.8790807914162,33.4548002532459,46.7572147631744));
#27163=CARTESIAN_POINT('Ctrl Pts',(43.9434516116396,33.4486105989604,46.8381231547602));
#27164=CARTESIAN_POINT('Ctrl Pts',(44.0608511484558,33.4360462363811,47.0127770823984));
#27165=CARTESIAN_POINT('Ctrl Pts',(44.1131334975787,33.4296908144134,47.106575372752));
#27166=CARTESIAN_POINT('Ctrl Pts',(44.1803082964872,33.4196834491732,47.2549216646809));
#27167=CARTESIAN_POINT('Ctrl Pts',(44.2010575065381,33.4162085561959,47.3065807017735));
#27168=CARTESIAN_POINT('Ctrl Pts',(44.2247354371408,33.4116613712007,47.3737993000641));
#27169=CARTESIAN_POINT('Ctrl Pts',(44.229747702195,33.4106586690996,47.3885999221372));
#27170=CARTESIAN_POINT('Ctrl Pts',(44.2375832320637,33.4090230178869,47.4126970310406));
#27171=CARTESIAN_POINT('Ctrl Pts',(44.2405171057321,33.4083937303086,47.4219570172841));
#27172=CARTESIAN_POINT('Ctrl Pts',(44.2460202418425,33.4071800353667,47.4397929258847));
#27173=CARTESIAN_POINT('Ctrl Pts',(44.248599991518,33.4065959905332,47.4483653691301));
#27174=CARTESIAN_POINT('Ctrl Pts',(44.2543765016882,33.4052526736635,47.4680562231594));
#27175=CARTESIAN_POINT('Ctrl Pts',(44.2575330748931,33.4044921115334,47.4791859665201));
#27176=CARTESIAN_POINT('Ctrl Pts',(44.2672821678355,33.4020555180509,47.5147766990358));
#27177=CARTESIAN_POINT('Ctrl Pts',(44.273492809607,33.4003672379884,47.5393385904564));
#27178=CARTESIAN_POINT('Ctrl Pts',(44.3095123852677,33.3896487011657,47.6945929645876));
#27179=CARTESIAN_POINT('Ctrl Pts',(44.3261094619838,33.3801956015534,47.8279501394247));
#27180=CARTESIAN_POINT('Ctrl Pts',(44.33022959864,33.3652891717794,48.0366626884876));
#27181=CARTESIAN_POINT('Ctrl Pts',(44.3273597465556,33.3599362648445,48.1114253059605));
#27182=CARTESIAN_POINT('Ctrl Pts',(44.3168491310644,33.3522704902663,48.2200273810585));
#27183=CARTESIAN_POINT('Ctrl Pts',(44.3126270148121,33.3498800194191,48.254127572478));
#27184=CARTESIAN_POINT('Ctrl Pts',(44.3042495367701,33.3460366210024,48.3095946972419));
#27185=CARTESIAN_POINT('Ctrl Pts',(44.300639585825,33.3445620486916,48.3310354029378));
#27186=CARTESIAN_POINT('Ctrl Pts',(44.2952531306863,33.3425874328491,48.3600251308901));
#27187=CARTESIAN_POINT('Ctrl Pts',(44.2937926297597,33.3420712116308,48.367630255532));
#27188=CARTESIAN_POINT('Ctrl Pts',(44.2912753032388,33.3412127382144,48.3803252600361));
#27189=CARTESIAN_POINT('Ctrl Pts',(44.2902436423086,33.3408690935911,48.3854199667271));
#27190=CARTESIAN_POINT('Ctrl Pts',(44.2882482533916,33.3402197128571,48.3950731545546));
#27191=CARTESIAN_POINT('Ctrl Pts',(44.2872885862118,33.339913741829,48.3996324028355));
#27192=CARTESIAN_POINT('Ctrl Pts',(44.2849734562484,33.3391902976939,48.4104369202839));
#27193=CARTESIAN_POINT('Ctrl Pts',(44.283603449281,33.3387736460443,48.4166790671348));
#27194=CARTESIAN_POINT('Ctrl Pts',(44.2786764828325,33.3373142425497,48.4386067863631));
#27195=CARTESIAN_POINT('Ctrl Pts',(44.2749542924982,33.3362803948793,48.4542550846753));
#27196=CARTESIAN_POINT('Ctrl Pts',(44.2425093830252,33.32779383224,48.5834556618117));
#27197=CARTESIAN_POINT('Ctrl Pts',(44.2036913347476,33.3208251464297,48.6942380720401));
#27198=CARTESIAN_POINT('Ctrl Pts',(44.1146336972522,33.3080297382683,48.889412988651));
#27199=CARTESIAN_POINT('Ctrl Pts',(44.0675642757087,33.302227158385,48.9748085971785));
#27200=CARTESIAN_POINT('Ctrl Pts',(43.9950999146802,33.2940772709602,49.0855516694621));
#27201=CARTESIAN_POINT('Ctrl Pts',(43.9751551546788,33.2919008363048,49.1142944795289));
#27202=CARTESIAN_POINT('Ctrl Pts',(43.93912773796,33.2880671710243,49.1633129199431));
#27203=CARTESIAN_POINT('Ctrl Pts',(43.9233978411,33.2864229762585,49.1838370073156));
#27204=CARTESIAN_POINT('Ctrl Pts',(43.8999024351224,33.2840055293503,49.2132494541325));
#27205=CARTESIAN_POINT('Ctrl Pts',(43.8924599475655,33.2832451317841,49.2223930822742));
#27206=CARTESIAN_POINT('Ctrl Pts',(43.8792175031877,33.281901155543,49.2383611489627));
#27207=CARTESIAN_POINT('Ctrl Pts',(43.8734529068069,33.2813190263296,49.2452145533517));
#27208=CARTESIAN_POINT('Ctrl Pts',(43.8613429344916,33.2801020060131,49.2594100009605));
#27209=CARTESIAN_POINT('Ctrl Pts',(43.8549894740085,33.279466790463,49.2667447838414));
#27210=CARTESIAN_POINT('Ctrl Pts',(43.8382909709405,33.2778055825467,49.285731080911));
#27211=CARTESIAN_POINT('Ctrl Pts',(43.8278597979883,33.2767760011228,49.297305554779));
#27212=CARTESIAN_POINT('Ctrl Pts',(43.7835214135272,33.2724323367416,49.3453210192894));
#27213=CARTESIAN_POINT('Ctrl Pts',(43.7483532368508,33.2690647230517,49.3805661620126));
#27214=CARTESIAN_POINT('Ctrl Pts',(43.6877403430423,33.2633811774886,49.4367845943652));
#27215=CARTESIAN_POINT('Ctrl Pts',(43.6630490104862,33.2610966942403,49.4585376821571));
#27216=CARTESIAN_POINT('Ctrl Pts',(43.5388102197891,33.2497579320187,49.5624709153666));
#27217=CARTESIAN_POINT('Ctrl Pts',(43.4317452958379,33.240434672214,49.6351457647133));
#27218=CARTESIAN_POINT('Ctrl Pts',(43.2622224315419,33.2268029387459,49.7268966899198));
#27219=CARTESIAN_POINT('Ctrl Pts',(43.204731412823,33.2223598924433,49.7544254983683));
#27220=CARTESIAN_POINT('Ctrl Pts',(43.1360089690752,33.2173357402022,49.7832414879358));
#27221=CARTESIAN_POINT('Ctrl Pts',(43.1260049059889,33.2166113051601,49.7873377679189));
#27222=CARTESIAN_POINT('Ctrl Pts',(43.1105184392174,33.2155011185706,49.7935273985152));
#27223=CARTESIAN_POINT('Ctrl Pts',(43.1050602236732,33.2151119737899,49.7956801120914));
#27224=CARTESIAN_POINT('Ctrl Pts',(43.094949353236,33.2143951819622,49.7996146180047));
#27225=CARTESIAN_POINT('Ctrl Pts',(43.0902996278164,33.2140671428868,49.8014032867925));
#27226=CARTESIAN_POINT('Ctrl Pts',(43.0796616313177,33.2133202212445,49.8054483020394));
#27227=CARTESIAN_POINT('Ctrl Pts',(43.0736690241318,33.212902040751,49.8076928813392));
#27228=CARTESIAN_POINT('Ctrl Pts',(43.0579155674641,33.211809190619,49.8135042472926));
#27229=CARTESIAN_POINT('Ctrl Pts',(43.0481367195893,33.2111373010809,49.8170221113304));
#27230=CARTESIAN_POINT('Ctrl Pts',(42.9707719748347,33.2058691534773,49.8441494240722));
#27231=CARTESIAN_POINT('Ctrl Pts',(42.9019396003338,33.201465876567,49.8640619171313));
#27232=CARTESIAN_POINT('Ctrl Pts',(42.7208009233592,33.1902279944947,49.905697629329));
#27233=CARTESIAN_POINT('Ctrl Pts',(42.6073957504876,33.1835191647837,49.9213497216503));
#27234=CARTESIAN_POINT('Ctrl Pts',(42.4087919508234,33.1715019817115,49.9309631090335));
#27235=CARTESIAN_POINT('Ctrl Pts',(42.3241462218332,33.1662989232456,49.929491999622));
#27236=CARTESIAN_POINT('Ctrl Pts',(42.2223489390126,33.159799033062,49.9210132772347));
#27237=CARTESIAN_POINT('Ctrl Pts',(42.2048424434905,33.1586727381356,49.9193137851873));
#27238=CARTESIAN_POINT('Ctrl Pts',(42.1772829802555,33.1568852053856,49.9162574262944));
#27239=CARTESIAN_POINT('Ctrl Pts',(42.1672130080796,33.156229003779,49.9150602091267));
#27240=CARTESIAN_POINT('Ctrl Pts',(42.1483570994117,33.1549943376775,49.912667514997));
#27241=CARTESIAN_POINT('Ctrl Pts',(42.1395690242208,33.15441647991,49.9114907467126));
#27242=CARTESIAN_POINT('Ctrl Pts',(42.1198869960356,33.1531167116274,49.9087169740905));
#27243=CARTESIAN_POINT('Ctrl Pts',(42.1089980475039,33.1523937800412,49.9070872128073));
#27244=CARTESIAN_POINT('Ctrl Pts',(42.0812799696924,33.1505434684253,49.902695702609));
#27245=CARTESIAN_POINT('Ctrl Pts',(42.0644727116037,33.1494120054724,49.8998038849541));
#27246=CARTESIAN_POINT('Ctrl Pts',(41.9617558750778,33.1424370821867,49.8807251295363));
#27247=CARTESIAN_POINT('Ctrl Pts',(41.8770401022699,33.1364193757565,49.8589459942695));
#27248=CARTESIAN_POINT('Ctrl Pts',(41.7941386107368,33.1302767167271,49.8315224633894));
#27249=CARTESIAN_POINT('Origin',(42.4,48.4493818343519,48.));
#27250=CARTESIAN_POINT('',(41.7941388784248,32.1635431008229,49.8315225519397));
#27251=CARTESIAN_POINT('',(41.794138831786,32.3337813919524,49.8315225365117));
#27252=CARTESIAN_POINT('',(41.7941388317924,48.4493818343519,49.8315225365138));
#27253=CARTESIAN_POINT('Ctrl Pts',(41.7941388784247,32.1635431008229,49.8315225519397));
#27254=CARTESIAN_POINT('Ctrl Pts',(41.9072674988879,32.1719168560421,49.8689450957153));
#27255=CARTESIAN_POINT('Ctrl Pts',(42.0236406174219,32.1805157140677,49.8958120447913));
#27256=CARTESIAN_POINT('Ctrl Pts',(42.20716904871,32.1936272155024,49.9206027649335));
#27257=CARTESIAN_POINT('Ctrl Pts',(42.2729945361483,32.1982372720411,49.9260764020955));
#27258=CARTESIAN_POINT('Ctrl Pts',(42.3498899796364,32.2034257326079,49.9285099792403));
#27259=CARTESIAN_POINT('Ctrl Pts',(42.3608053169991,32.2041575925035,49.9287626978604));
#27260=CARTESIAN_POINT('Ctrl Pts',(42.3776231368258,32.2052774610604,49.9290092425017));
#27261=CARTESIAN_POINT('Ctrl Pts',(42.3835242178087,32.2056689348062,49.9290686697401));
#27262=CARTESIAN_POINT('Ctrl Pts',(42.3944001447044,32.2063876162718,49.929128286455));
#27263=CARTESIAN_POINT('Ctrl Pts',(42.3993747525962,32.206715240161,49.9291363130827));
#27264=CARTESIAN_POINT('Ctrl Pts',(42.4106970710997,32.2074584357207,49.9291107850804));
#27265=CARTESIAN_POINT('Ctrl Pts',(42.4170446197297,32.2078733289184,49.9290651446303));
#27266=CARTESIAN_POINT('Ctrl Pts',(42.4336590813188,32.2089549631484,49.9288636688096));
#27267=CARTESIAN_POINT('Ctrl Pts',(42.4439253377381,32.2096189857862,49.928657191538));
#27268=CARTESIAN_POINT('Ctrl Pts',(42.5210456161652,32.2145778952333,49.9264900091652));
#27269=CARTESIAN_POINT('Ctrl Pts',(42.5877666014461,32.2187036080615,49.9211354884859));
#27270=CARTESIAN_POINT('Ctrl Pts',(42.771526612617,32.2299373844789,49.896720162025));
#27271=CARTESIAN_POINT('Ctrl Pts',(42.8872859530086,32.2368808631999,49.8703297503966));
#27272=CARTESIAN_POINT('Ctrl Pts',(43.0757791759041,32.2488584447555,49.8086569179086));
#27273=CARTESIAN_POINT('Ctrl Pts',(43.1500402324937,32.2537610988222,49.7791443966971));
#27274=CARTESIAN_POINT('Ctrl Pts',(43.2409655065399,32.2601303653587,49.7363028001725));
#27275=CARTESIAN_POINT('Ctrl Pts',(43.2595332099424,32.2614508257434,49.7271864418577));
#27276=CARTESIAN_POINT('Ctrl Pts',(43.2875279337964,32.263473811028,49.7128784018791));
#27277=CARTESIAN_POINT('Ctrl Pts',(43.2970644118627,32.2641687024878,49.7079033011462));
#27278=CARTESIAN_POINT('Ctrl Pts',(43.3135784728637,32.2653823190737,49.6991115842605));
#27279=CARTESIAN_POINT('Ctrl Pts',(43.3205750505281,32.2658997455274,49.6953310517387));
#27280=CARTESIAN_POINT('Ctrl Pts',(43.336247648067,32.2670662343823,49.6867368913846));
#27281=CARTESIAN_POINT('Ctrl Pts',(43.3449102563945,32.267716146239,49.6818994025632));
#27282=CARTESIAN_POINT('Ctrl Pts',(43.3680932681234,32.2694696130528,49.6687176049584));
#27283=CARTESIAN_POINT('Ctrl Pts',(43.382542691734,32.270577591519,49.6602508392984));
#27284=CARTESIAN_POINT('Ctrl Pts',(43.4501924220265,32.2758380482185,49.6194184627264));
#27285=CARTESIAN_POINT('Ctrl Pts',(43.5019101204656,32.2800772407709,49.5846806877562));
#27286=CARTESIAN_POINT('Ctrl Pts',(43.680809607114,32.2955474235228,49.4515206917045));
#27287=CARTESIAN_POINT('Ctrl Pts',(43.7972575939745,32.3072347153004,49.3397933837717));
#27288=CARTESIAN_POINT('Ctrl Pts',(43.920588247354,32.321009022085,49.1876810011976));
#27289=CARTESIAN_POINT('Ctrl Pts',(43.9419488358847,32.3234542644864,49.1598141515082));
#27290=CARTESIAN_POINT('Ctrl Pts',(43.9754730232617,32.3273732629032,49.1135141428578));
#27291=CARTESIAN_POINT('Ctrl Pts',(43.988101208106,32.3288699291328,49.0954285232397));
#27292=CARTESIAN_POINT('Ctrl Pts',(44.0047465253204,32.3308667354981,49.0706966286458));
#27293=CARTESIAN_POINT('Ctrl Pts',(44.0090372287352,32.3313837093015,49.064237700323));
#27294=CARTESIAN_POINT('Ctrl Pts',(44.0161279930828,32.332241610232,49.0534228385389));
#27295=CARTESIAN_POINT('Ctrl Pts',(44.0189496384977,32.3325839551696,49.0490812348157));
#27296=CARTESIAN_POINT('Ctrl Pts',(44.0242708119744,32.3332313197712,49.040821063987));
#27297=CARTESIAN_POINT('Ctrl Pts',(44.0267736899045,32.333536573062,49.0369047790675));
#27298=CARTESIAN_POINT('Ctrl Pts',(44.0326593460827,32.3342562910065,49.0276216528783));
#27299=CARTESIAN_POINT('Ctrl Pts',(44.0360298785954,32.3346699547353,49.0222470547464));
#27300=CARTESIAN_POINT('Ctrl Pts',(44.0477149962201,32.3361097203392,49.0034083205503));
#27301=CARTESIAN_POINT('Ctrl Pts',(44.0558906448,32.3371272244244,48.9898581604743));
#27302=CARTESIAN_POINT('Ctrl Pts',(44.126084419954,32.3459680817708,48.870216343279));
#27303=CARTESIAN_POINT('Ctrl Pts',(44.1780091022977,32.3532560005212,48.758509138183));
#27304=CARTESIAN_POINT('Ctrl Pts',(44.2635559725403,32.3685730568418,48.5163611983905));
#27305=CARTESIAN_POINT('Ctrl Pts',(44.2948870187581,32.3765832389472,48.3858327060392));
#27306=CARTESIAN_POINT('Ctrl Pts',(44.3152879526994,32.3864279861685,48.2316932707008));
#27307=CARTESIAN_POINT('Ctrl Pts',(44.3177634957114,32.3878070290787,48.2102209026224));
#27308=CARTESIAN_POINT('Ctrl Pts',(44.3209533750396,32.3899047584419,48.1777684170449));
#27309=CARTESIAN_POINT('Ctrl Pts',(44.3219354649262,32.3906150374623,48.1668158852367));
#27310=CARTESIAN_POINT('Ctrl Pts',(44.3235349546635,32.3918991621102,48.1470826562151));
#27311=CARTESIAN_POINT('Ctrl Pts',(44.3241860021117,32.3924719340927,48.1383049331604));
#27312=CARTESIAN_POINT('Ctrl Pts',(44.325459242284,32.3937100982808,48.1193839702669));
#27313=CARTESIAN_POINT('Ctrl Pts',(44.3260613979636,32.3943761019677,48.1092396934337));
#27314=CARTESIAN_POINT('Ctrl Pts',(44.3274654402131,32.3961743825997,48.0819415896934));
#27315=CARTESIAN_POINT('Ctrl Pts',(44.3281184584628,32.397311277062,48.0647813627441));
#27316=CARTESIAN_POINT('Ctrl Pts',(44.3302693579628,32.4031172147902,47.9776641487525));
#27317=CARTESIAN_POINT('Ctrl Pts',(44.328189180088,32.4078962732452,47.9076792845813));
#27318=CARTESIAN_POINT('Ctrl Pts',(44.3110442345745,32.4221162405019,47.7042742287412));
#27319=CARTESIAN_POINT('Ctrl Pts',(44.285858338118,32.4317985392029,47.5721256201118));
#27320=CARTESIAN_POINT('Ctrl Pts',(44.2279007330723,32.4460255095263,47.379687547101));
#27321=CARTESIAN_POINT('Ctrl Pts',(44.2053143237983,32.4506940112294,47.3167351872062));
#27322=CARTESIAN_POINT('Ctrl Pts',(44.1752770885707,32.4559392091753,47.244981069327));
#27323=CARTESIAN_POINT('Ctrl Pts',(44.1709651886289,32.4566727127537,47.2349218070907));
#27324=CARTESIAN_POINT('Ctrl Pts',(44.1641938356677,32.4577946333787,47.2194888999038));
#27325=CARTESIAN_POINT('Ctrl Pts',(44.1617949926255,32.4581865277781,47.2140891440796));
#27326=CARTESIAN_POINT('Ctrl Pts',(44.1573236891308,32.4589067273784,47.204147671498));
#27327=CARTESIAN_POINT('Ctrl Pts',(44.1552584075879,32.4592354407962,47.1996029729894));
#27328=CARTESIAN_POINT('Ctrl Pts',(44.1505115886838,32.4599820751124,47.1892642271349));
#27329=CARTESIAN_POINT('Ctrl Pts',(44.1478189150676,32.4603993080739,47.183475439117));
#27330=CARTESIAN_POINT('Ctrl Pts',(44.1406958594543,32.4614869901734,47.1683587822512));
#27331=CARTESIAN_POINT('Ctrl Pts',(44.1362191641368,32.4621547102715,47.1590527867186));
#27332=CARTESIAN_POINT('Ctrl Pts',(44.1019492792773,32.4671520972365,47.0892540723202));
#27333=CARTESIAN_POINT('Ctrl Pts',(44.0690739812981,32.4713111038475,47.0303177679003));
#27334=CARTESIAN_POINT('Ctrl Pts',(43.9704788921546,32.4825378230482,46.8734946451555));
#27335=CARTESIAN_POINT('Ctrl Pts',(43.8987796684108,32.4894476872849,46.7797216508117));
#27336=CARTESIAN_POINT('Ctrl Pts',(43.7612920859757,32.501710969413,46.6304469887103));
#27337=CARTESIAN_POINT('Ctrl Pts',(43.6995356524249,32.5069475363231,46.571715719001));
#27338=CARTESIAN_POINT('Ctrl Pts',(43.6205611780423,32.5134855858658,46.5059840691251));
#27339=CARTESIAN_POINT('Ctrl Pts',(43.6068611354089,32.5146142087247,46.4948955658153));
#27340=CARTESIAN_POINT('Ctrl Pts',(43.5850319934505,32.5164049424466,46.4777172293808));
#27341=CARTESIAN_POINT('Ctrl Pts',(43.5770032213669,32.5170619953196,46.4715010403762));
#27342=CARTESIAN_POINT('Ctrl Pts',(43.5618669668022,32.5182979714027,46.4599719335952));
#27343=CARTESIAN_POINT('Ctrl Pts',(43.5547711471058,32.5188762846609,46.4546440904322));
#27344=CARTESIAN_POINT('Ctrl Pts',(43.5387867249415,32.5201766991738,46.4428138721542));
#27345=CARTESIAN_POINT('Ctrl Pts',(43.5298787483716,32.5208998194795,46.4363383207764));
#27346=CARTESIAN_POINT('Ctrl Pts',(43.507041857916,32.5227498842846,46.4200343405437));
#27347=CARTESIAN_POINT('Ctrl Pts',(43.4930374578308,32.523880902984,46.41031379066));
#27348=CARTESIAN_POINT('Ctrl Pts',(43.3755261892693,32.5333447578064,46.3310353330669));
#27349=CARTESIAN_POINT('Ctrl Pts',(43.2656461821844,32.5420539341752,46.2714918286313));
#27350=CARTESIAN_POINT('Ctrl Pts',(43.0629307744464,32.5577232508734,46.1858426480931));
#27351=CARTESIAN_POINT('Ctrl Pts',(42.9724165083657,32.5645847819425,46.1552820997704));
#27352=CARTESIAN_POINT('Ctrl Pts',(42.847258456564,32.5736596534812,46.1231286693996));
#27353=CARTESIAN_POINT('Ctrl Pts',(42.8142878400042,32.5760118153956,46.1155764874121));
#27354=CARTESIAN_POINT('Ctrl Pts',(42.76005978089,32.5798009182823,46.104647349928));
#27355=CARTESIAN_POINT('Ctrl Pts',(42.7389150499263,32.5812587968835,46.1007524126144));
#27356=CARTESIAN_POINT('Ctrl Pts',(42.7101012725517,32.5832149873657,46.0959413764203));
#27357=CARTESIAN_POINT('Ctrl Pts',(42.7024862646245,32.583729099547,46.0947167911337));
#27358=CARTESIAN_POINT('Ctrl Pts',(42.6897323012163,32.5845851188412,46.0927441927253));
#27359=CARTESIAN_POINT('Ctrl Pts',(42.6845973682915,32.5849284008608,46.0919712107347));
#27360=CARTESIAN_POINT('Ctrl Pts',(42.6748449752091,32.5855777035339,46.0905433901941));
#27361=CARTESIAN_POINT('Ctrl Pts',(42.6702281713484,32.585883954827,46.0898845475474));
#27362=CARTESIAN_POINT('Ctrl Pts',(42.6592581644352,32.5866090550458,46.0883596381499));
#27363=CARTESIAN_POINT('Ctrl Pts',(42.652902893998,32.5870270721889,46.0875084842133));
#27364=CARTESIAN_POINT('Ctrl Pts',(42.6304603840889,32.5884963505454,46.0846166111892));
#27365=CARTESIAN_POINT('Ctrl Pts',(42.6143512496176,32.5895385409978,46.0827469915871));
#27366=CARTESIAN_POINT('Ctrl Pts',(42.4850058390888,32.5978207633293,46.069385917015));
#27367=CARTESIAN_POINT('Ctrl Pts',(42.3709627678726,32.6046046755424,46.0677317354184));
#27368=CARTESIAN_POINT('Ctrl Pts',(42.199508063046,32.6148591444999,46.0804379344875));
#27369=CARTESIAN_POINT('Ctrl Pts',(42.1418137764107,32.61831778222,46.0873434197811));
#27370=CARTESIAN_POINT('Ctrl Pts',(42.0253488323188,32.6254341855636,46.1066493960196));
#27371=CARTESIAN_POINT('Ctrl Pts',(41.9666712275647,32.6290909575149,46.1192115100373));
#27372=CARTESIAN_POINT('Ctrl Pts',(41.8836648453543,32.6344358740224,46.1410730047344));
#27373=CARTESIAN_POINT('Ctrl Pts',(41.858788533113,32.6360600985312,46.1481626369091));
#27374=CARTESIAN_POINT('Ctrl Pts',(41.8145202562716,32.638995881271,46.1617470482715));
#27375=CARTESIAN_POINT('Ctrl Pts',(41.795074576193,32.6403014119288,46.1680541423516));
#27376=CARTESIAN_POINT('Ctrl Pts',(41.7655701204336,32.6423083984655,46.1781447208892));
#27377=CARTESIAN_POINT('Ctrl Pts',(41.7554362509301,32.643002488637,46.1817053330758));
#27378=CARTESIAN_POINT('Ctrl Pts',(41.7378184886579,32.6442177117306,46.1880612545936));
#27379=CARTESIAN_POINT('Ctrl Pts',(41.7303211737441,32.6447375736612,46.1908187936251));
#27380=CARTESIAN_POINT('Ctrl Pts',(41.7134514200507,32.6459135721128,46.1971427775912));
#27381=CARTESIAN_POINT('Ctrl Pts',(41.7040892876526,32.6465705913145,46.2007358751415));
#27382=CARTESIAN_POINT('Ctrl Pts',(41.6788571043233,32.6483534441502,46.2106461389446));
#27383=CARTESIAN_POINT('Ctrl Pts',(41.6630425555437,32.6494838996218,46.2171012342195));
#27384=CARTESIAN_POINT('Ctrl Pts',(41.5866986574307,32.6550061990478,46.2494521465143));
#27385=CARTESIAN_POINT('Ctrl Pts',(41.5274425534871,32.6594949575766,46.2782222468132));
#27386=CARTESIAN_POINT('Ctrl Pts',(41.3483422745964,32.6737047918526,46.376801661231));
#27387=CARTESIAN_POINT('Ctrl Pts',(41.2344706722456,32.6837145263455,46.4565326928062));
#27388=CARTESIAN_POINT('Ctrl Pts',(41.078929807297,32.6983541272594,46.5925399494304));
#27389=CARTESIAN_POINT('Ctrl Pts',(41.0301176815546,32.7031107570334,46.6400019240119));
#27390=CARTESIAN_POINT('Ctrl Pts',(40.9764713200649,32.7084384051924,46.6979905269358));
#27391=CARTESIAN_POINT('Ctrl Pts',(40.9691002675374,32.7091727474729,46.7060956217653));
#27392=CARTESIAN_POINT('Ctrl Pts',(40.957868754177,32.7102946880727,46.7186589871109));
#27393=CARTESIAN_POINT('Ctrl Pts',(40.9539591642678,32.7106857955974,46.7230727408368));
#27394=CARTESIAN_POINT('Ctrl Pts',(40.9467856978513,32.711404357457,46.7312464631874));
#27395=CARTESIAN_POINT('Ctrl Pts',(40.9435161452909,32.7117322202043,46.7350011355502));
#27396=CARTESIAN_POINT('Ctrl Pts',(40.9361042419745,32.7124763221332,46.7435796118587));
#27397=CARTESIAN_POINT('Ctrl Pts',(40.9319711763515,32.712891880276,46.7484112664765));
#27398=CARTESIAN_POINT('Ctrl Pts',(40.9212374439471,32.7139730228975,46.7610855833468));
#27399=CARTESIAN_POINT('Ctrl Pts',(40.9146751626316,32.7146359244242,46.7689606961952));
#27400=CARTESIAN_POINT('Ctrl Pts',(40.8665597502601,32.7195140008489,46.8276468457977));
#27401=CARTESIAN_POINT('Ctrl Pts',(40.8275565177226,32.7235672602918,46.8805026272857));
#27402=CARTESIAN_POINT('Ctrl Pts',(40.7253373814637,32.734802680076,47.0349405868066));
#27403=CARTESIAN_POINT('Ctrl Pts',(40.6687627797713,32.7418105329177,47.1405502067055));
#27404=CARTESIAN_POINT('Ctrl Pts',(40.5891398750078,32.7541954312319,47.3294562505877));
#27405=CARTESIAN_POINT('Ctrl Pts',(40.5612244083232,32.7594495861638,47.4103009963779));
#27406=CARTESIAN_POINT('Ctrl Pts',(40.5341224851497,32.7660074182651,47.5097401241126));
#27407=CARTESIAN_POINT('Ctrl Pts',(40.5297182559861,32.7671368207791,47.5268194729658));
#27408=CARTESIAN_POINT('Ctrl Pts',(40.5231482510522,32.7689284119007,47.5538238027289));
#27409=CARTESIAN_POINT('Ctrl Pts',(40.5208255501855,32.7695855304553,47.5637098818977));
#27410=CARTESIAN_POINT('Ctrl Pts',(40.516620345962,32.7708213975887,47.582265240335));
#27411=CARTESIAN_POINT('Ctrl Pts',(40.5147193690435,32.7713995343598,47.5909300930363));
#27412=CARTESIAN_POINT('Ctrl Pts',(40.5105941049486,32.7726992451858,47.6103732097248));
#27413=CARTESIAN_POINT('Ctrl Pts',(40.5084021672772,32.7734218354066,47.621157944987));
#27414=CARTESIAN_POINT('Ctrl Pts',(40.5030543846781,32.7752699561995,47.6486742468806));
#27415=CARTESIAN_POINT('Ctrl Pts',(40.5000276082617,32.7763995483212,47.6654296319288));
#27416=CARTESIAN_POINT('Ctrl Pts',(40.4795850524721,32.7846844393458,47.7878348228267));
#27417=CARTESIAN_POINT('Ctrl Pts',(40.4707733022669,32.7921116273483,47.8947143130847));
#27418=CARTESIAN_POINT('Ctrl Pts',(40.4709430630594,32.8053188321743,48.0810943779638));
#27419=CARTESIAN_POINT('Ctrl Pts',(40.4759095343439,32.8110110823264,48.1603507283172));
#27420=CARTESIAN_POINT('Ctrl Pts',(40.4958199445622,32.8224447983019,48.3197732298439));
#27421=CARTESIAN_POINT('Ctrl Pts',(40.5109929409353,32.828172398129,48.3997649671017));
#27422=CARTESIAN_POINT('Ctrl Pts',(40.5337810751144,32.8343753664206,48.4887535475341));
#27423=CARTESIAN_POINT('Ctrl Pts',(40.536472685262,32.8350812860896,48.4989178941643));
#27424=CARTESIAN_POINT('Ctrl Pts',(40.5409461469989,32.8362121840939,48.5152696127213));
#27425=CARTESIAN_POINT('Ctrl Pts',(40.5426760608043,32.836639958625,48.521470794975));
#27426=CARTESIAN_POINT('Ctrl Pts',(40.5458013062818,32.837395982998,48.5324609276981));
#27427=CARTESIAN_POINT('Ctrl Pts',(40.5471842024917,32.8377249321392,48.5372532529651));
#27428=CARTESIAN_POINT('Ctrl Pts',(40.5502282394737,32.8384370248065,48.5476505853408));
#27429=CARTESIAN_POINT('Ctrl Pts',(40.5518962766661,32.8388197645047,48.5532534317115));
#27430=CARTESIAN_POINT('Ctrl Pts',(40.5566900453146,32.8398991390048,48.5690918212364));
#27431=CARTESIAN_POINT('Ctrl Pts',(40.5598755762821,32.8405923999654,48.5793092507478));
#27432=CARTESIAN_POINT('Ctrl Pts',(40.5817250468115,32.8451947037126,48.6473911697807));
#27433=CARTESIAN_POINT('Ctrl Pts',(40.6030325594261,32.8489645139326,48.7043782832065));
#27434=CARTESIAN_POINT('Ctrl Pts',(40.6614775561044,32.8579933715375,48.8406760965728));
#27435=CARTESIAN_POINT('Ctrl Pts',(40.7013874549419,32.8631725591656,48.9186475439191));
#27436=CARTESIAN_POINT('Ctrl Pts',(40.8088560185719,32.875637202009,49.097488627115));
#27437=CARTESIAN_POINT('Ctrl Pts',(40.8808926557693,32.882951708786,49.1952103076591));
#27438=CARTESIAN_POINT('Ctrl Pts',(40.9729666537279,32.8917284831323,49.2982329611719));
#27439=CARTESIAN_POINT('Ctrl Pts',(40.9844907360234,32.8928176643121,49.3107884980936));
#27440=CARTESIAN_POINT('Ctrl Pts',(41.0037301866482,32.8946219828419,49.33120034385));
#27441=CARTESIAN_POINT('Ctrl Pts',(41.0113493116389,32.8953330021545,49.3391463715941));
#27442=CARTESIAN_POINT('Ctrl Pts',(41.0252288712522,32.8966222150939,49.3533756179059));
#27443=CARTESIAN_POINT('Ctrl Pts',(41.0314654642989,32.8971993556388,49.3596817420832));
#27444=CARTESIAN_POINT('Ctrl Pts',(41.0449308612265,32.8984410221111,49.3731107653558));
#27445=CARTESIAN_POINT('Ctrl Pts',(41.05217280408,32.8991061245981,49.3802200505857));
#27446=CARTESIAN_POINT('Ctrl Pts',(41.072135949775,32.9009324807351,49.3995105666265));
#27447=CARTESIAN_POINT('Ctrl Pts',(41.0849681527182,32.9020987394458,49.4115749953383));
#27448=CARTESIAN_POINT('Ctrl Pts',(41.1606741716367,32.9089368881136,49.4808230883911));
#27449=CARTESIAN_POINT('Ctrl Pts',(41.2270979607387,32.9147754136375,49.5339695961183));
#27450=CARTESIAN_POINT('Ctrl Pts',(41.3924096041987,32.9289219182915,49.6492081059154));
#27451=CARTESIAN_POINT('Ctrl Pts',(41.4938597452921,32.9373218283312,49.7070538543969));
#27452=CARTESIAN_POINT('Ctrl Pts',(41.6227314563021,32.9473627504026,49.7657932404724));
#27453=CARTESIAN_POINT('Ctrl Pts',(41.645765002433,32.94913352297,49.7757538680722));
#27454=CARTESIAN_POINT('Ctrl Pts',(41.7101550212048,32.9540072854119,49.8021197059625));
#27455=CARTESIAN_POINT('Ctrl Pts',(41.7518972880076,32.9570810654367,49.8175491834415));
#27456=CARTESIAN_POINT('Ctrl Pts',(41.7941388318293,32.9600825139687,49.8315225365261));
#27457=CARTESIAN_POINT('Ctrl Pts',(41.7941386107368,33.1302767167271,49.8315224633894));
#27458=CARTESIAN_POINT('Ctrl Pts',(41.7615147270867,33.127859421335,49.8207305938566));
#27459=CARTESIAN_POINT('Ctrl Pts',(41.7291717434368,33.1254237180773,49.8090646017079));
#27460=CARTESIAN_POINT('Ctrl Pts',(41.6149606743047,33.1166972958759,49.7643819978487));
#27461=CARTESIAN_POINT('Ctrl Pts',(41.5350796627018,33.1103547917976,49.7266278222783));
#27462=CARTESIAN_POINT('Ctrl Pts',(41.4061633483993,33.0999288319688,49.6544993513602));
#27463=CARTESIAN_POINT('Ctrl Pts',(41.3556279388961,33.0957902366805,49.6230735941093));
#27464=CARTESIAN_POINT('Ctrl Pts',(41.297850656533,33.091063592458,49.5833264650798));
#27465=CARTESIAN_POINT('Ctrl Pts',(41.2891304590911,33.0903503774043,49.5772205762432));
#27466=CARTESIAN_POINT('Ctrl Pts',(41.2757115790359,33.0892536778906,49.5676581627451));
#27467=CARTESIAN_POINT('Ctrl Pts',(41.2709774423454,33.0888669250832,49.5642521009344));
#27468=CARTESIAN_POINT('Ctrl Pts',(41.2622246661972,33.0881522788655,49.5578943182576));
#27469=CARTESIAN_POINT('Ctrl Pts',(41.2582020374948,33.0878240133612,49.554948497781));
#27470=CARTESIAN_POINT('Ctrl Pts',(41.2490030964146,33.0870736841918,49.5481570543374));
#27471=CARTESIAN_POINT('Ctrl Pts',(41.2438346079019,33.0866523482214,49.5443010477344));
#27472=CARTESIAN_POINT('Ctrl Pts',(41.2302549001728,33.0855456816944,49.534063371676));
#27473=CARTESIAN_POINT('Ctrl Pts',(41.2218764321198,33.0848632461135,49.5276383399584));
#27474=CARTESIAN_POINT('Ctrl Pts',(41.1405643025086,33.0782391709025,49.4642172178386));
#27475=CARTESIAN_POINT('Ctrl Pts',(41.0717589759254,33.0726223398984,49.4021022875851));
#27476=CARTESIAN_POINT('Ctrl Pts',(40.9990185411646,33.0663226256873,49.3262540637331));
#27477=CARTESIAN_POINT('Ctrl Pts',(40.9904520660688,33.0655745477457,49.3171459732951));
#27478=CARTESIAN_POINT('Ctrl Pts',(40.9262198504802,33.059912931797,49.247508338125));
#27479=CARTESIAN_POINT('Ctrl Pts',(40.8743876223578,33.0550375394858,49.1835588172295));
#27480=CARTESIAN_POINT('Ctrl Pts',(40.7787915528492,33.0450471402053,49.0488590267635));
#27481=CARTESIAN_POINT('Ctrl Pts',(40.7352052952309,33.0399403918666,48.9782014859006));
#27482=CARTESIAN_POINT('Ctrl Pts',(40.688091078958,33.0335489588917,48.8895037288625));
#27483=CARTESIAN_POINT('Ctrl Pts',(40.6800897137146,33.0324278142054,48.8739322698421));
#27484=CARTESIAN_POINT('Ctrl Pts',(40.6677978270342,33.0306466047338,48.8491882413673));
#27485=CARTESIAN_POINT('Ctrl Pts',(40.6633655759673,33.0299915151533,48.8400868455566));
#27486=CARTESIAN_POINT('Ctrl Pts',(40.6551851871595,33.0287578144078,48.8229474331243));
#27487=CARTESIAN_POINT('Ctrl Pts',(40.6514204334554,33.0281798003556,48.8149176055436));
#27488=CARTESIAN_POINT('Ctrl Pts',(40.6430955762017,33.0268781883101,48.7968382438436));
#27489=CARTESIAN_POINT('Ctrl Pts',(40.6385661008055,33.0261535565662,48.7867750322433));
#27490=CARTESIAN_POINT('Ctrl Pts',(40.6272237306765,33.0242959656867,48.7609865608202));
#27491=CARTESIAN_POINT('Ctrl Pts',(40.6205337051132,33.0231588685262,48.7452086418029));
#27492=CARTESIAN_POINT('Ctrl Pts',(40.5682651120988,33.0139277823888,48.6172185293761));
#27493=CARTESIAN_POINT('Ctrl Pts',(40.5331443989851,33.005480343087,48.5010507189353));
#27494=CARTESIAN_POINT('Ctrl Pts',(40.4917450432384,32.9906207077751,48.2963315506964));
#27495=CARTESIAN_POINT('Ctrl Pts',(40.4802380464948,32.9843115903462,48.2091975567793));
#27496=CARTESIAN_POINT('Ctrl Pts',(40.4721369186006,32.9752353741278,48.0809137529819));
#27497=CARTESIAN_POINT('Ctrl Pts',(40.4708577562553,32.9723849732908,48.0401711806233));
#27498=CARTESIAN_POINT('Ctrl Pts',(40.4708773732771,32.9679288131525,47.9753400246355));
#27499=CARTESIAN_POINT('Ctrl Pts',(40.4713353791613,32.9662914876989,47.9512646773269));
#27500=CARTESIAN_POINT('Ctrl Pts',(40.4725581146939,32.9641183941057,47.9188851465437));
#27501=CARTESIAN_POINT('Ctrl Pts',(40.4729260522475,32.9635628696974,47.9105693183467));
#27502=CARTESIAN_POINT('Ctrl Pts',(40.4735907117892,32.9626919997224,47.8974680838602));
#27503=CARTESIAN_POINT('Ctrl Pts',(40.4738514622092,32.9623747088496,47.8926810773693));
#27504=CARTESIAN_POINT('Ctrl Pts',(40.4744253604253,32.9617231808707,47.8828219845888));
#27505=CARTESIAN_POINT('Ctrl Pts',(40.4747407062539,32.9613890864397,47.8777501236156));
#27506=CARTESIAN_POINT('Ctrl Pts',(40.475547395764,32.9605881755256,47.8655540033088));
#27507=CARTESIAN_POINT('Ctrl Pts',(40.4760582699671,32.9601224414514,47.8584310225197));
#27508=CARTESIAN_POINT('Ctrl Pts',(40.4779692693259,32.9585126584404,47.8337109881351));
#27509=CARTESIAN_POINT('Ctrl Pts',(40.4795714084917,32.9573792573921,47.8161298191591));
#27510=CARTESIAN_POINT('Ctrl Pts',(40.4841149842176,32.9546122004852,47.7728525498307));
#27511=CARTESIAN_POINT('Ctrl Pts',(40.487332296015,32.9529912285091,47.7471883201765));
#27512=CARTESIAN_POINT('Ctrl Pts',(40.5030641468658,32.9462333323331,47.6393198699513));
#27513=CARTESIAN_POINT('Ctrl Pts',(40.5203709789221,32.9412653538758,47.5578997366747));
#27514=CARTESIAN_POINT('Ctrl Pts',(40.5807614609927,32.9279539466273,47.3431120367659));
#27515=CARTESIAN_POINT('Ctrl Pts',(40.6331874290855,32.9196337565058,47.2129177703834));
#27516=CARTESIAN_POINT('Ctrl Pts',(40.7099032863855,32.9093818880291,47.0696092234485));
#27517=CARTESIAN_POINT('Ctrl Pts',(40.7209247792119,32.9079444066352,47.0498630447721));
#27518=CARTESIAN_POINT('Ctrl Pts',(40.7379976636677,32.9057666619252,47.0205002769766));
#27519=CARTESIAN_POINT('Ctrl Pts',(40.7437913048257,32.9050356301211,47.0107355144459));
#27520=CARTESIAN_POINT('Ctrl Pts',(40.7539917679356,32.9037618961415,46.9938841586329));
#27521=CARTESIAN_POINT('Ctrl Pts',(40.7583590416499,32.9032206478411,46.9867738917276));
#27522=CARTESIAN_POINT('Ctrl Pts',(40.7675623655489,32.9020883782403,46.9720058595979));
#27523=CARTESIAN_POINT('Ctrl Pts',(40.7724064791666,32.9014970682631,46.9643533859073));
#27524=CARTESIAN_POINT('Ctrl Pts',(40.7840204656009,32.9000901291989,46.9462889687548));
#27525=CARTESIAN_POINT('Ctrl Pts',(40.7908372837079,32.8992727607925,46.9359078361565));
#27526=CARTESIAN_POINT('Ctrl Pts',(40.8141873958028,32.8965005492696,46.9010861664034));
#27527=CARTESIAN_POINT('Ctrl Pts',(40.8311803527963,32.8945284543902,46.8769603837267));
#27528=CARTESIAN_POINT('Ctrl Pts',(40.9495979977378,32.881074625599,46.7167714976733));
#27529=CARTESIAN_POINT('Ctrl Pts',(41.0680281891642,32.8688951677033,46.5942366766812));
#27530=CARTESIAN_POINT('Ctrl Pts',(41.2651054740751,32.8509873867075,46.4378631845213));
#27531=CARTESIAN_POINT('Ctrl Pts',(41.332483331483,32.8452145362849,46.3910660896583));
#27532=CARTESIAN_POINT('Ctrl Pts',(41.4116435852658,32.8389696709358,46.3432547657331));
#27533=CARTESIAN_POINT('Ctrl Pts',(41.4206909434239,32.8382635219546,46.337890810566));
#27534=CARTESIAN_POINT('Ctrl Pts',(41.4353450787058,32.8371324903369,46.3293639335814));
#27535=CARTESIAN_POINT('Ctrl Pts',(41.4409244611659,32.8367048066551,46.3261546972988));
#27536=CARTESIAN_POINT('Ctrl Pts',(41.4508532638451,32.8359490706671,46.3205096373435));
#27537=CARTESIAN_POINT('Ctrl Pts',(41.4551961758112,32.8356203183103,46.3180626822602));
#27538=CARTESIAN_POINT('Ctrl Pts',(41.4646476200966,32.8349088020585,46.3127855540667));
#27539=CARTESIAN_POINT('Ctrl Pts',(41.4697595417082,32.8345264404781,46.3099617302722));
#27540=CARTESIAN_POINT('Ctrl Pts',(41.4842590282512,32.8334486511038,46.3020379385212));
#27541=CARTESIAN_POINT('Ctrl Pts',(41.493676421316,32.8327565844146,46.296992579891));
#27542=CARTESIAN_POINT('Ctrl Pts',(41.5566350324331,32.8281793079464,46.2639327504259));
#27543=CARTESIAN_POINT('Ctrl Pts',(41.6114310020281,32.8244316562747,46.2383659602684));
#27544=CARTESIAN_POINT('Ctrl Pts',(41.7485416370087,32.8154058173238,46.182075593339));
#27545=CARTESIAN_POINT('Ctrl Pts',(41.8319246032079,32.81020979572,46.1543188741337));
#27546=CARTESIAN_POINT('Ctrl Pts',(42.0342894251511,32.7977232185353,46.1019752839152));
#27547=CARTESIAN_POINT('Ctrl Pts',(42.1542519273775,32.7904040371647,46.0827508575401));
#27548=CARTESIAN_POINT('Ctrl Pts',(42.2922506237716,32.7816202483702,46.0738058197902));
#27549=CARTESIAN_POINT('Ctrl Pts',(42.3092985065227,32.7805293188496,46.0729278277196));
#27550=CARTESIAN_POINT('Ctrl Pts',(42.3373620300573,32.778722857676,46.0718557198696));
#27551=CARTESIAN_POINT('Ctrl Pts',(42.3483718960755,32.7780114644838,46.0715295151742));
#27552=CARTESIAN_POINT('Ctrl Pts',(42.3682480128104,32.7767220794704,46.0711109472227));
#27553=CARTESIAN_POINT('Ctrl Pts',(42.3771133139427,32.7761451453899,46.0709853909832));
#27554=CARTESIAN_POINT('Ctrl Pts',(42.3961150243766,32.7749044872833,46.0708472825056));
#27555=CARTESIAN_POINT('Ctrl Pts',(42.4062512608656,32.7742401912574,46.0708535007625));
#27556=CARTESIAN_POINT('Ctrl Pts',(42.433955540078,32.7724175289279,46.0710888406797));
#27557=CARTESIAN_POINT('Ctrl Pts',(42.4515208891821,32.7712541878074,46.0714780783368));
#27558=CARTESIAN_POINT('Ctrl Pts',(42.5532357004277,32.7644710652349,46.0751226037742));
#27559=CARTESIAN_POINT('Ctrl Pts',(42.6370937402029,32.7586878041765,46.0836448113319));
#27560=CARTESIAN_POINT('Ctrl Pts',(42.8311038473629,32.7448819182853,46.1162912055346));
#27561=CARTESIAN_POINT('Ctrl Pts',(42.9402395245262,32.736779565787,46.1446434519515));
#27562=CARTESIAN_POINT('Ctrl Pts',(43.1157247084538,32.7235535862841,46.2070375847799));
#27563=CARTESIAN_POINT('Ctrl Pts',(43.1837136784464,32.7183818255549,46.2356951968113));
#27564=CARTESIAN_POINT('Ctrl Pts',(43.2592278210297,32.7127030014276,46.2727542088044));
#27565=CARTESIAN_POINT('Ctrl Pts',(43.2685166728648,32.7120056694562,46.2774062370224));
#27566=CARTESIAN_POINT('Ctrl Pts',(43.2834647895333,32.7108859854207,46.2850441834349));
#27567=CARTESIAN_POINT('Ctrl Pts',(43.2891474252043,32.7104609186149,46.2879835438041));
#27568=CARTESIAN_POINT('Ctrl Pts',(43.299228663118,32.7097080230181,46.2932618290844));
#27569=CARTESIAN_POINT('Ctrl Pts',(43.303632935062,32.7093795146122,46.2955895760596));
#27570=CARTESIAN_POINT('Ctrl Pts',(43.3132053279991,32.7086664465512,46.3006963145658));
#27571=CARTESIAN_POINT('Ctrl Pts',(43.3183698100338,32.7082823048892,46.3034818360255));
#27572=CARTESIAN_POINT('Ctrl Pts',(43.3330142327483,32.7071944280713,46.31146693848));
#27573=CARTESIAN_POINT('Ctrl Pts',(43.3424634626311,32.7064941539107,46.3167228115757));
#27574=CARTESIAN_POINT('Ctrl Pts',(43.4073298375056,32.7016950211493,46.3535204147001));
#27575=CARTESIAN_POINT('Ctrl Pts',(43.4612038690275,32.6977495003872,46.3877169585655));
#27576=CARTESIAN_POINT('Ctrl Pts',(43.6188245052923,32.6860217710254,46.4990975467148));
#27577=CARTESIAN_POINT('Ctrl Pts',(43.7166001581044,32.678467968548,46.5840877198615));
#27578=CARTESIAN_POINT('Ctrl Pts',(43.8293819805125,32.6684938429855,46.7039826863542));
#27579=CARTESIAN_POINT('Ctrl Pts',(43.8529035644283,32.6663334550125,46.7304076329116));
#27580=CARTESIAN_POINT('Ctrl Pts',(43.9063426028066,32.661208189995,46.7938739041656));
#27581=CARTESIAN_POINT('Ctrl Pts',(43.9356402995454,32.6582249806155,46.8314040515661));
#27582=CARTESIAN_POINT('Ctrl Pts',(43.9725025054451,32.6542080375318,46.8824072071422));
#27583=CARTESIAN_POINT('Ctrl Pts',(43.9813376568428,32.6532235633975,46.8949439049024));
#27584=CARTESIAN_POINT('Ctrl Pts',(43.99548729691,32.6516102644668,46.9155388507849));
#27585=CARTESIAN_POINT('Ctrl Pts',(44.0008925529039,32.6509849133545,46.9235341495559));
#27586=CARTESIAN_POINT('Ctrl Pts',(44.0112077975302,32.6497736531223,46.9390416941349));
#27587=CARTESIAN_POINT('Ctrl Pts',(44.0161258140627,32.6491880673004,46.9465483199852));
#27588=CARTESIAN_POINT('Ctrl Pts',(44.0274511110583,32.6478203858908,46.9641006784119));
#27589=CARTESIAN_POINT('Ctrl Pts',(44.0338179963109,32.6470368124478,46.9741719113712));
#27590=CARTESIAN_POINT('Ctrl Pts',(44.0540731472851,32.6444954929287,47.0068787481755));
#27591=CARTESIAN_POINT('Ctrl Pts',(44.0675869142557,32.6427241715028,47.0297414979195));
#27592=CARTESIAN_POINT('Ctrl Pts',(44.0984068780175,32.6384970282286,47.0844299140084));
#27593=CARTESIAN_POINT('Ctrl Pts',(44.1152965745122,32.6360275145451,47.116477572618));
#27594=CARTESIAN_POINT('Ctrl Pts',(44.209513071513,32.6213025006089,47.3081469800617));
#27595=CARTESIAN_POINT('Ctrl Pts',(44.2654163227491,32.6083776283653,47.4773104515767));
#27596=CARTESIAN_POINT('Ctrl Pts',(44.3054846192847,32.5928440791353,47.6955959439858));
#27597=CARTESIAN_POINT('Ctrl Pts',(44.3120160775499,32.589764410194,47.739752635199));
#27598=CARTESIAN_POINT('Ctrl Pts',(44.3181514334363,32.5860719052369,47.7942293858239));
#27599=CARTESIAN_POINT('Ctrl Pts',(44.3192119884425,32.5853892211959,47.8043681471091));
#27600=CARTESIAN_POINT('Ctrl Pts',(44.3207493955662,32.5843251557278,47.8202838212652));
#27601=CARTESIAN_POINT('Ctrl Pts',(44.321280646642,32.583940873049,47.8260551107366));
#27602=CARTESIAN_POINT('Ctrl Pts',(44.322216999829,32.5832314044185,47.8367553397053));
#27603=CARTESIAN_POINT('Ctrl Pts',(44.3226291568514,32.5829058468177,47.841683419876));
#27604=CARTESIAN_POINT('Ctrl Pts',(44.3235375472108,32.5821561998802,47.8530719817408));
#27605=CARTESIAN_POINT('Ctrl Pts',(44.3240201877445,32.5817328729143,47.8595334266394));
#27606=CARTESIAN_POINT('Ctrl Pts',(44.3254318188024,32.5804105765569,47.8798064653185));
#27607=CARTESIAN_POINT('Ctrl Pts',(44.3262447371161,32.5795177967145,47.8936260652181));
#27608=CARTESIAN_POINT('Ctrl Pts',(44.3278097648141,32.5774304088608,47.9262115443997));
#27609=CARTESIAN_POINT('Ctrl Pts',(44.3284367594633,32.5762417983661,47.9449823059044));
#27610=CARTESIAN_POINT('Ctrl Pts',(44.3297155327105,32.5719725214781,48.013041969864));
#27611=CARTESIAN_POINT('Ctrl Pts',(44.3287524257359,32.5689563944188,48.0623449278515));
#27612=CARTESIAN_POINT('Ctrl Pts',(44.3162504896511,32.5558853102316,48.2781704342769));
#27613=CARTESIAN_POINT('Ctrl Pts',(44.285022401705,32.5461921927418,48.4428158778149));
#27614=CARTESIAN_POINT('Ctrl Pts',(44.220990190609,32.5334096322984,48.6379814136542));
#27615=CARTESIAN_POINT('Ctrl Pts',(44.2078928390235,32.5309830755487,48.6742022871535));
#27616=CARTESIAN_POINT('Ctrl Pts',(44.1885021972832,32.5276140217928,48.7231898224253));
#27617=CARTESIAN_POINT('Ctrl Pts',(44.1831382407902,32.5267025539517,48.73631625386));
#27618=CARTESIAN_POINT('Ctrl Pts',(44.1743421410815,32.5252391859063,48.7571817278413));
#27619=CARTESIAN_POINT('Ctrl Pts',(44.1710028497136,32.5246904467517,48.7649595447407));
#27620=CARTESIAN_POINT('Ctrl Pts',(44.164014236772,32.5235557022868,48.7809462400385));
#27621=CARTESIAN_POINT('Ctrl Pts',(44.1603585503434,32.5229694899477,48.7891520936953));
#27622=CARTESIAN_POINT('Ctrl Pts',(44.1517012749385,32.5215979875712,48.8082254106238));
#27623=CARTESIAN_POINT('Ctrl Pts',(44.1466556898427,32.5208111961935,48.8190723784543));
#27624=CARTESIAN_POINT('Ctrl Pts',(44.129972898071,32.5182491598198,48.8540817049404));
#27625=CARTESIAN_POINT('Ctrl Pts',(44.117933087236,32.5164600339134,48.8780475904377));
#27626=CARTESIAN_POINT('Ctrl Pts',(44.0882494272282,32.5121827663386,48.9341853765786));
#27627=CARTESIAN_POINT('Ctrl Pts',(44.0701801158531,32.5096804963287,48.9661193139892));
#27628=CARTESIAN_POINT('Ctrl Pts',(43.9963660500525,32.4998334922583,49.0883053980668));
#27629=CARTESIAN_POINT('Ctrl Pts',(43.9341310325276,32.4922852062604,49.1744064812181));
#27630=CARTESIAN_POINT('Ctrl Pts',(43.7969518240043,32.4772203905606,49.3345624314687));
#27631=CARTESIAN_POINT('Ctrl Pts',(43.7223765700516,32.469731523701,49.4084941399137));
#27632=CARTESIAN_POINT('Ctrl Pts',(43.6295781301487,32.4614744149673,49.4865902059251));
#27633=CARTESIAN_POINT('Ctrl Pts',(43.6168646142309,32.4603643981281,49.49701482067));
#27634=CARTESIAN_POINT('Ctrl Pts',(43.5989795460197,32.4588339056251,49.5113014934771));
#27635=CARTESIAN_POINT('Ctrl Pts',(43.5939199674711,32.4584043359862,49.5153017092899));
#27636=CARTESIAN_POINT('Ctrl Pts',(43.5851593075931,32.4576665117619,49.5221569627609));
#27637=CARTESIAN_POINT('Ctrl Pts',(43.5814677765303,32.4573574227233,49.5250240318914));
#27638=CARTESIAN_POINT('Ctrl Pts',(43.5736659969172,32.4567080597173,49.5310380403035));
#27639=CARTESIAN_POINT('Ctrl Pts',(43.5695534419046,32.4563680145791,49.5341818994897));
#27640=CARTESIAN_POINT('Ctrl Pts',(43.5593293723149,32.4555280737974,49.5419327276482));
#27641=CARTESIAN_POINT('Ctrl Pts',(43.5532029182652,32.4550295412523,49.546520017413));
#27642=CARTESIAN_POINT('Ctrl Pts',(43.5300763445239,32.4531648316923,49.5636226007144));
#27643=CARTESIAN_POINT('Ctrl Pts',(43.5128977574236,32.4518143452906,49.5758955714776));
#27644=CARTESIAN_POINT('Ctrl Pts',(43.3768404747242,32.4413564985689,49.6697648057039));
#27645=CARTESIAN_POINT('Ctrl Pts',(43.2493393069896,32.4329333940499,49.7380925822542));
#27646=CARTESIAN_POINT('Ctrl Pts',(43.013035733349,32.4177010972683,49.8324515719433));
#27647=CARTESIAN_POINT('Ctrl Pts',(42.9073716629756,32.4110112709358,49.8644733350024));
#27648=CARTESIAN_POINT('Ctrl Pts',(42.7828843201844,32.4029288151265,49.8908285766093));
#27649=CARTESIAN_POINT('Ctrl Pts',(42.766162744866,32.4018394593182,49.8941377783271));
#27650=CARTESIAN_POINT('Ctrl Pts',(42.7385785185858,32.4000353175995,49.8992177911765));
#27651=CARTESIAN_POINT('Ctrl Pts',(42.7277404434161,32.3993246588688,49.9011180460505));
#27652=CARTESIAN_POINT('Ctrl Pts',(42.708147300367,32.3980364239191,49.9043808171335));
#27653=CARTESIAN_POINT('Ctrl Pts',(42.6993979158559,32.3974599027952,49.9057759414372));
#27654=CARTESIAN_POINT('Ctrl Pts',(42.6806229527741,32.3962199386853,49.9086372032618));
#27655=CARTESIAN_POINT('Ctrl Pts',(42.6705948488278,32.3955559226203,49.9100847196975));
#27656=CARTESIAN_POINT('Ctrl Pts',(42.6431475437532,32.3937335437654,49.9138261449776));
#27657=CARTESIAN_POINT('Ctrl Pts',(42.6257080266696,32.3925702005636,49.9159611407884));
#27658=CARTESIAN_POINT('Ctrl Pts',(42.5243698113536,32.3857768113485,49.9269645121615));
#27659=CARTESIAN_POINT('Ctrl Pts',(42.4400022139649,32.3799825382938,49.9305585625719));
#27660=CARTESIAN_POINT('Ctrl Pts',(42.2416140427867,32.3660557013752,49.9259995763934));
#27661=CARTESIAN_POINT('Ctrl Pts',(42.1280088908297,32.357838023745,49.9132638553038));
#27662=CARTESIAN_POINT('Ctrl Pts',(41.9456239564482,32.3446288845988,49.8762387891454));
#27663=CARTESIAN_POINT('Ctrl Pts',(41.8758919321985,32.3395798094311,49.8579673498479));
#27664=CARTESIAN_POINT('Ctrl Pts',(41.8029333694424,32.3344039767775,49.8344141902643));
#27665=CARTESIAN_POINT('Ctrl Pts',(41.7985335092115,32.3340922710875,49.8329762802391));
#27666=CARTESIAN_POINT('Ctrl Pts',(41.794138831786,32.3337813919524,49.8315225365117));
#27667=CARTESIAN_POINT('Origin',(42.4,47.1748,48.));
#27668=CARTESIAN_POINT('',(40.0365300974769,46.7157731502363,48.0006787984381));
#27669=CARTESIAN_POINT('',(43.4903488624466,46.9748,50.0969334274272));
#27670=CARTESIAN_POINT('Ctrl Pts',(40.0365300974771,46.7157731502717,48.0006787990958));
#27671=CARTESIAN_POINT('Ctrl Pts',(40.0365388030446,46.7174032156133,48.030990193079));
#27672=CARTESIAN_POINT('Ctrl Pts',(40.0371305975263,46.7190332809549,48.0612934096708));
#27673=CARTESIAN_POINT('Ctrl Pts',(40.0383046853366,46.7206633462965,48.0915733672902));
#27674=CARTESIAN_POINT('Ctrl Pts',(40.0413609422814,46.7249065540677,48.1703948403946));
#27675=CARTESIAN_POINT('Ctrl Pts',(40.0483732154124,46.7291497618388,48.2492105493059));
#27676=CARTESIAN_POINT('Ctrl Pts',(40.0593432685315,46.73339296961,48.3275919814818));
#27677=CARTESIAN_POINT('Ctrl Pts',(40.0702973976645,46.737630017996,48.4058596361922));
#27678=CARTESIAN_POINT('Ctrl Pts',(40.0851978327039,46.7418670663821,48.4836938069707));
#27679=CARTESIAN_POINT('Ctrl Pts',(40.1039943670488,46.7461041147681,48.5606679715807));
#27680=CARTESIAN_POINT('Ctrl Pts',(40.1227687031728,46.7503361593095,48.6375512316929));
#27681=CARTESIAN_POINT('Ctrl Pts',(40.145429883651,46.754568203851,48.7135760523368));
#27682=CARTESIAN_POINT('Ctrl Pts',(40.1718763758854,46.7588002483924,48.7883245249022));
#27683=CARTESIAN_POINT('Ctrl Pts',(40.1983057184753,46.7630295485978,48.8630245256433));
#27684=CARTESIAN_POINT('Ctrl Pts',(40.228515344752,46.7672588488033,48.9364493817146));
#27685=CARTESIAN_POINT('Ctrl Pts',(40.2623537838844,46.7714881490088,49.0081959609255));
#27686=CARTESIAN_POINT('Ctrl Pts',(40.2961807462329,46.7757160147874,49.0799182062722));
#27687=CARTESIAN_POINT('Ctrl Pts',(40.3336338779797,46.7799438805661,49.1499628826561));
#27688=CARTESIAN_POINT('Ctrl Pts',(40.3745140131288,46.7841717463447,49.2179478469492));
#27689=CARTESIAN_POINT('Ctrl Pts',(40.4153929270747,46.7883994858252,49.2859307803428));
#27690=CARTESIAN_POINT('Ctrl Pts',(40.4596983989203,46.7926272253058,49.3518537239599));
#27691=CARTESIAN_POINT('Ctrl Pts',(40.5071865997293,46.7968549647863,49.4153613929508));
#27692=CARTESIAN_POINT('Ctrl Pts',(40.5547205133257,46.8010867739463,49.4789301952869));
#27693=CARTESIAN_POINT('Ctrl Pts',(40.6054429958083,46.8053185831063,49.5400787030201));
#27694=CARTESIAN_POINT('Ctrl Pts',(40.6590687276934,46.8095503922663,49.5984832642242));
#27695=CARTESIAN_POINT('Ctrl Pts',(40.7127192606394,46.8137841585718,49.6569148366229));
#27696=CARTESIAN_POINT('Ctrl Pts',(40.7692753849433,46.8180179248772,49.7125996052308));
#27697=CARTESIAN_POINT('Ctrl Pts',(40.8284153563963,46.8222516911827,49.7652512990759));
#27698=CARTESIAN_POINT('Ctrl Pts',(40.8876603719865,46.8264929774838,49.8179965126102));
#27699=CARTESIAN_POINT('Ctrl Pts',(40.9494980405442,46.8307342637849,49.8676975919985));
#27700=CARTESIAN_POINT('Ctrl Pts',(41.013574195887,46.834975550086,49.9141091741564));
#27701=CARTESIAN_POINT('Ctrl Pts',(41.073569654564,46.8389467296247,49.9575650298424));
#27702=CARTESIAN_POINT('Ctrl Pts',(41.1355270033101,46.8429179091634,49.998137282269));
#27703=CARTESIAN_POINT('Ctrl Pts',(41.1991358615461,46.8468890887021,50.0356610134979));
#27704=CARTESIAN_POINT('Ctrl Pts',(41.2670255033899,46.8511275228456,50.0757100372411));
#27705=CARTESIAN_POINT('Ctrl Pts',(41.3370471788954,46.8553659569892,50.1124337060636));
#27706=CARTESIAN_POINT('Ctrl Pts',(41.4088418280244,46.8596043911328,50.1455991981323));
#27707=CARTESIAN_POINT('Ctrl Pts',(41.4805339567318,46.8638367729304,50.1787173309581));
#27708=CARTESIAN_POINT('Ctrl Pts',(41.5539936093392,46.868069154728,50.2082871826824));
#27709=CARTESIAN_POINT('Ctrl Pts',(41.6288353142845,46.8723015365256,50.2341207372041));
#27710=CARTESIAN_POINT('Ctrl Pts',(41.7035917373713,46.8765290955391,50.2599248544816));
#27711=CARTESIAN_POINT('Ctrl Pts',(41.779726642607,46.8807566545526,50.2820009830718));
#27712=CARTESIAN_POINT('Ctrl Pts',(41.8568340596542,46.8849842135661,50.3002089474977));
#27713=CARTESIAN_POINT('Ctrl Pts',(41.9338934632194,46.8892091401502,50.3184055741326));
#27714=CARTESIAN_POINT('Ctrl Pts',(42.0119237218414,46.8934340667344,50.3327387101318));
#27715=CARTESIAN_POINT('Ctrl Pts',(42.090504335332,46.8976589933185,50.3431181947251));
#27716=CARTESIAN_POINT('Ctrl Pts',(42.1690604450329,46.901882602444,50.353494442684));
#27717=CARTESIAN_POINT('Ctrl Pts',(42.24816610469,46.9061062115694,50.3599194261523));
#27718=CARTESIAN_POINT('Ctrl Pts',(42.3273927376713,46.9103298206949,50.3623544667042));
#27719=CARTESIAN_POINT('Ctrl Pts',(42.4066192926496,46.9145534256619,50.3647895048586));
#27720=CARTESIAN_POINT('Ctrl Pts',(42.4859663524167,46.918777030629,50.3632345949384));
#27721=CARTESIAN_POINT('Ctrl Pts',(42.5650038545159,46.9230006355961,50.3577031553813));
#27722=CARTESIAN_POINT('Ctrl Pts',(42.6441216143524,46.9272285293751,50.3521660989864));
#27723=CARTESIAN_POINT('Ctrl Pts',(42.7229287201695,46.931456423154,50.3426444797425));
#27724=CARTESIAN_POINT('Ctrl Pts',(42.8009993411237,46.935684316933,50.3292037200121));
#27725=CARTESIAN_POINT('Ctrl Pts',(42.8791081960042,46.9399142812601,50.3157563778695));
#27726=CARTESIAN_POINT('Ctrl Pts',(42.9564793898032,46.9441442455872,50.2983861744852));
#27727=CARTESIAN_POINT('Ctrl Pts',(43.0326989421299,46.9483742099143,50.2772093644476));
#27728=CARTESIAN_POINT('Ctrl Pts',(43.1090582419274,46.9526119298211,50.2559937270284));
#27729=CARTESIAN_POINT('Ctrl Pts',(43.1842612353293,46.956849649728,50.2309576849966));
#27730=CARTESIAN_POINT('Ctrl Pts',(43.2579109006931,46.9610873696348,50.2022668610711));
#27731=CARTESIAN_POINT('Ctrl Pts',(43.3275881903807,46.9650965234593,50.1751235082784));
#27732=CARTESIAN_POINT('Ctrl Pts',(43.3958750636315,46.9691056772837,50.1447095516255));
#27733=CARTESIAN_POINT('Ctrl Pts',(43.4624562730563,46.9731148311082,50.1112027635316));
#27734=CARTESIAN_POINT('Ctrl Pts',(43.4717849733108,46.9736765540721,50.106508123928));
#27735=CARTESIAN_POINT('Ctrl Pts',(43.4810826793527,46.9742382770361,50.1017515928794));
#27736=CARTESIAN_POINT('Ctrl Pts',(43.4903488624466,46.9748,50.0969334274272));
#27737=CARTESIAN_POINT('',(41.309406738763,46.9748,50.0968063285493));
#27738=CARTESIAN_POINT('Origin',(42.4,46.9748,48.));
#27739=CARTESIAN_POINT('',(40.036080165837,46.8369518497283,48.0019190348969));
#27740=CARTESIAN_POINT('Ctrl Pts',(41.309406738763,46.9748,50.0968063285493));
#27741=CARTESIAN_POINT('Ctrl Pts',(40.6110438901808,46.9327247525314,49.7335730598435));
#27742=CARTESIAN_POINT('Ctrl Pts',(40.0689346244942,46.8867753691075,48.9289907544835));
#27743=CARTESIAN_POINT('Ctrl Pts',(40.0334053491648,46.8408259856836,48.0740634180572));
#27744=CARTESIAN_POINT('Ctrl Pts',(40.0338853815248,46.8369518497283,48.0019208166272));
#27745=CARTESIAN_POINT('',(40.0365304449332,46.0432018497572,48.0014502318932));
#27746=CARTESIAN_POINT('Ctrl Pts',(40.0365307787896,46.8369518497283,48.0019186690884));
#27747=CARTESIAN_POINT('Ctrl Pts',(40.036468137554,46.8328034394031,47.9247554765118));
#27748=CARTESIAN_POINT('Ctrl Pts',(40.0401885216025,46.8286550290779,47.8474148710146));
#27749=CARTESIAN_POINT('Ctrl Pts',(40.0477175957458,46.8245066187527,47.7703090521241));
#27750=CARTESIAN_POINT('Ctrl Pts',(40.0554430041532,46.8202500311042,47.6911925591568));
#27751=CARTESIAN_POINT('Ctrl Pts',(40.0671786223162,46.8159934434557,47.6123237804389));
#27752=CARTESIAN_POINT('Ctrl Pts',(40.0828950922958,46.8117368558072,47.5341510034429));
#27753=CARTESIAN_POINT('Ctrl Pts',(40.0981734160342,46.8075989339839,47.4581575395153));
#27754=CARTESIAN_POINT('Ctrl Pts',(40.1172134465915,46.8034610121605,47.3828222978298));
#27755=CARTESIAN_POINT('Ctrl Pts',(40.1399357060372,46.7993230903372,47.3085523678148));
#27756=CARTESIAN_POINT('Ctrl Pts',(40.1626453859003,46.7951874593657,47.2343235553977));
#27757=CARTESIAN_POINT('Ctrl Pts',(40.189033110172,46.7910518283942,47.1611593525195));
#27758=CARTESIAN_POINT('Ctrl Pts',(40.2189688712524,46.7869161974227,47.0894541986622));
#27759=CARTESIAN_POINT('Ctrl Pts',(40.2488982284564,46.7827814511479,47.0177643840154));
#27760=CARTESIAN_POINT('Ctrl Pts',(40.2823739274349,46.7786467048732,46.9475334505543));
#27761=CARTESIAN_POINT('Ctrl Pts',(40.3192175308638,46.7745119585984,46.8791366019735));
#27762=CARTESIAN_POINT('Ctrl Pts',(40.35795205641,46.7701650049809,46.8072294259084));
#27763=CARTESIAN_POINT('Ctrl Pts',(40.4004092074394,46.7658180513634,46.7373501821476));
#27764=CARTESIAN_POINT('Ctrl Pts',(40.4463276425709,46.7614710977458,46.6699042287424));
#27765=CARTESIAN_POINT('Ctrl Pts',(40.4900580006794,46.757331282488,46.6056721684177));
#27766=CARTESIAN_POINT('Ctrl Pts',(40.5369269476158,46.7531914672301,46.5436471628575));
#27767=CARTESIAN_POINT('Ctrl Pts',(40.5866664300395,46.7490516519722,46.4841465094033));
#27768=CARTESIAN_POINT('Ctrl Pts',(40.6364392548573,46.7449090616281,46.4246059702458));
#27769=CARTESIAN_POINT('Ctrl Pts',(40.6890861058771,46.7407664712841,46.3675935029111));
#27770=CARTESIAN_POINT('Ctrl Pts',(40.7443021294053,46.73662388094,46.313389493034));
#27771=CARTESIAN_POINT('Ctrl Pts',(40.7996058292231,46.7324747126693,46.2590994138211));
#27772=CARTESIAN_POINT('Ctrl Pts',(40.8574864657606,46.7283255443986,46.2076270003678));
#27773=CARTESIAN_POINT('Ctrl Pts',(40.9176070793061,46.7241763761279,46.1592116717078));
#27774=CARTESIAN_POINT('Ctrl Pts',(40.9264355250731,46.723567089148,46.1521020951723));
#27775=CARTESIAN_POINT('Ctrl Pts',(40.9353122254245,46.7229578021681,46.1450583620089));
#27776=CARTESIAN_POINT('Ctrl Pts',(40.9442360662148,46.7223485151882,46.1380811483875));
#27777=CARTESIAN_POINT('Ctrl Pts',(41.0063218352461,46.71810952756,46.0895386336163));
#27778=CARTESIAN_POINT('Ctrl Pts',(41.0709556443962,46.7138705399317,46.0440130955615));
#27779=CARTESIAN_POINT('Ctrl Pts',(41.1378123220411,46.7096315523034,46.0017826178044));
#27780=CARTESIAN_POINT('Ctrl Pts',(41.2045716917168,46.7053987343996,45.9596136052917));
#27781=CARTESIAN_POINT('Ctrl Pts',(41.2735471120876,46.7011659164958,45.9207303769664));
#27782=CARTESIAN_POINT('Ctrl Pts',(41.3443813107765,46.6969330985919,45.885370097662));
#27783=CARTESIAN_POINT('Ctrl Pts',(41.4151318134713,46.6927052820844,45.8500515992174));
#27784=CARTESIAN_POINT('Ctrl Pts',(41.48773631278,46.6884774655769,45.8182479854144));
#27785=CARTESIAN_POINT('Ctrl Pts',(41.5618109117649,46.6842496490694,45.7901517035634));
#27786=CARTESIAN_POINT('Ctrl Pts',(41.6358374850734,46.6800245736331,45.7620736377131));
#27787=CARTESIAN_POINT('Ctrl Pts',(41.7113318293812,46.6757994981968,45.7376982985315));
#27788=CARTESIAN_POINT('Ctrl Pts',(41.7878890338709,46.6715744227605,45.7171704824835));
#27789=CARTESIAN_POINT('Ctrl Pts',(41.8644204008238,46.6673507732584,45.6966495944342));
#27790=CARTESIAN_POINT('Ctrl Pts',(41.9420134635277,46.6631271237564,45.6799737721795));
#27791=CARTESIAN_POINT('Ctrl Pts',(42.020248499192,46.6589034742543,45.6672378521302));
#27792=CARTESIAN_POINT('Ctrl Pts',(42.0984814496739,46.6546799373243,45.6545022715288));
#27793=CARTESIAN_POINT('Ctrl Pts',(42.177355876536,46.6504564003943,45.645706458409));
#27794=CARTESIAN_POINT('Ctrl Pts',(42.2564436959489,46.6462328634644,45.6408938072933));
#27795=CARTESIAN_POINT('Ctrl Pts',(42.3356086411391,46.6420052077766,45.6360764629206));
#27796=CARTESIAN_POINT('Ctrl Pts',(42.4149869259069,46.6377775520889,45.6352500688633));
#27797=CARTESIAN_POINT('Ctrl Pts',(42.4941478032849,46.6335498964012,45.63840591294));
#27798=CARTESIAN_POINT('Ctrl Pts',(42.5733457062223,46.6293202633312,45.6415632330854));
#27799=CARTESIAN_POINT('Ctrl Pts',(42.6523255319369,46.6250906302612,45.6487064602432));
#27800=CARTESIAN_POINT('Ctrl Pts',(42.7306615533172,46.6208609971912,45.6597749300425));
#27801=CARTESIAN_POINT('Ctrl Pts',(42.8091383540487,46.6166237629565,45.6708632912272));
#27802=CARTESIAN_POINT('Ctrl Pts',(42.8869685772243,46.6123865287218,45.6858909022939));
#27803=CARTESIAN_POINT('Ctrl Pts',(42.9637367902861,46.6081492944871,45.7047459242651));
#27804=CARTESIAN_POINT('Ctrl Pts',(43.0363670745302,46.6041404539189,45.7225846305548));
#27805=CARTESIAN_POINT('Ctrl Pts',(43.1080465470771,46.6001316133506,45.7438487227785));
#27806=CARTESIAN_POINT('Ctrl Pts',(43.1784391621289,46.5961227727824,45.7684035060603));
#27807=CARTESIAN_POINT('Ctrl Pts',(43.2529342276332,46.59188029876,45.7943893312448));
#27808=CARTESIAN_POINT('Ctrl Pts',(43.3262630340169,46.5876378247375,45.8241569755966));
#27809=CARTESIAN_POINT('Ctrl Pts',(43.3980154719991,46.5833953507151,45.8575818432084));
#27810=CARTESIAN_POINT('Ctrl Pts',(43.4696664379429,46.5791588763841,45.8909594414932));
#27811=CARTESIAN_POINT('Ctrl Pts',(43.5397450425771,46.5749224020531,45.9279837952047));
#27812=CARTESIAN_POINT('Ctrl Pts',(43.6078584146434,46.5706859277222,45.9684812353623));
#27813=CARTESIAN_POINT('Ctrl Pts',(43.6758952397014,46.5664542144157,46.0089331637827));
#27814=CARTESIAN_POINT('Ctrl Pts',(43.741970821366,46.5622225011092,46.0528501842038));
#27815=CARTESIAN_POINT('Ctrl Pts',(43.8057156423378,46.5579907878028,46.1000121122));
#27816=CARTESIAN_POINT('Ctrl Pts',(43.8694213494987,46.5537616710749,46.1471451016455));
#27817=CARTESIAN_POINT('Ctrl Pts',(43.9307987599507,46.5495325543469,46.1975187689448));
#27818=CARTESIAN_POINT('Ctrl Pts',(43.9895072149921,46.545303437619,46.2508695719335));
#27819=CARTESIAN_POINT('Ctrl Pts',(44.0481978050543,46.5410756078111,46.3042041402762));
#27820=CARTESIAN_POINT('Ctrl Pts',(44.1042207068267,46.5368477780031,46.3605137309542));
#27821=CARTESIAN_POINT('Ctrl Pts',(44.1572693933893,46.5326199481951,46.4194954223548));
#27822=CARTESIAN_POINT('Ctrl Pts',(44.2103183446974,46.5283920972877,46.4784774081104));
#27823=CARTESIAN_POINT('Ctrl Pts',(44.2603927397304,46.5241642463803,46.5401311725002));
#27824=CARTESIAN_POINT('Ctrl Pts',(44.3072248952418,46.5199363954729,46.604119045237));
#27825=CARTESIAN_POINT('Ctrl Pts',(44.3541046881307,46.5157042440218,46.6681720060403));
#27826=CARTESIAN_POINT('Ctrl Pts',(44.3977353768617,46.5114720925707,46.734563439658));
#27827=CARTESIAN_POINT('Ctrl Pts',(44.437891733117,46.5072399411196,46.8029253469423));
#27828=CARTESIAN_POINT('Ctrl Pts',(44.4780678610049,46.5030057059002,46.8713209133193));
#27829=CARTESIAN_POINT('Ctrl Pts',(44.5147660320134,46.4987714706807,46.9416884710826));
#27830=CARTESIAN_POINT('Ctrl Pts',(44.547807487796,46.4945372354613,47.0136362555997));
#27831=CARTESIAN_POINT('Ctrl Pts',(44.5809092578639,46.4902952710161,47.0857153744996));
#27832=CARTESIAN_POINT('Ctrl Pts',(44.6103408005741,46.4860533065709,47.1593800489095));
#27833=CARTESIAN_POINT('Ctrl Pts',(44.6359720053084,46.4818113421257,47.2342195925873));
#27834=CARTESIAN_POINT('Ctrl Pts',(44.6599686046557,46.477839904876,47.304286316473));
#27835=CARTESIAN_POINT('Ctrl Pts',(44.6806345420483,46.4738684676263,47.3753823760291));
#27836=CARTESIAN_POINT('Ctrl Pts',(44.6979037062447,46.4698970303766,47.4471627746552));
#27837=CARTESIAN_POINT('Ctrl Pts',(44.7163012908706,46.465666087173,47.5236335258272));
#27838=CARTESIAN_POINT('Ctrl Pts',(44.7309131367711,46.4614351439694,47.601172016668));
#27839=CARTESIAN_POINT('Ctrl Pts',(44.7416203849523,46.4572042007659,47.6793687262976));
#27840=CARTESIAN_POINT('Ctrl Pts',(44.7523119331019,46.4529794613917,47.757450776139));
#27841=CARTESIAN_POINT('Ctrl Pts',(44.7591101888584,46.4487547220176,47.8361886662048));
#27842=CARTESIAN_POINT('Ctrl Pts',(44.7619468026331,46.4445299826435,47.9151604901508));
#27843=CARTESIAN_POINT('Ctrl Pts',(44.7647800501454,46.4403102568462,47.994038596764));
#27844=CARTESIAN_POINT('Ctrl Pts',(44.7636609808645,46.4360905310489,48.0731496179231));
#27845=CARTESIAN_POINT('Ctrl Pts',(44.7585729628223,46.4318708052516,48.1520658408181));
#27846=CARTESIAN_POINT('Ctrl Pts',(44.753488254408,46.4276538242799,48.2309307306931));
#27847=CARTESIAN_POINT('Ctrl Pts',(44.7444397511366,46.4234368433081,48.3096006055514));
#27848=CARTESIAN_POINT('Ctrl Pts',(44.7314628968383,46.4192198623364,48.3876482962253));
#27849=CARTESIAN_POINT('Ctrl Pts',(44.7184904069863,46.4150042996427,48.4656697374749));
#27850=CARTESIAN_POINT('Ctrl Pts',(44.7015922664761,46.410788736949,48.5430689462409));
#27851=CARTESIAN_POINT('Ctrl Pts',(44.6808555329728,46.4065731742553,48.6194259266509));
#27852=CARTESIAN_POINT('Ctrl Pts',(44.6601192594321,46.4023577050672,48.6957812133826));
#27853=CARTESIAN_POINT('Ctrl Pts',(44.6355446866869,46.3981422358791,48.7710938639706));
#27854=CARTESIAN_POINT('Ctrl Pts',(44.607269160561,46.393926766691,48.844957569193));
#27855=CARTESIAN_POINT('Ctrl Pts',(44.5789654189238,46.3897070909811,48.9188949813449));
#27856=CARTESIAN_POINT('Ctrl Pts',(44.5469535149943,46.3854874152712,48.9913801193012));
#27857=CARTESIAN_POINT('Ctrl Pts',(44.5114193257397,46.3812677395612,49.0620258338633));
#27858=CARTESIAN_POINT('Ctrl Pts',(44.475868192399,46.3770460517455,49.1327052350548));
#27859=CARTESIAN_POINT('Ctrl Pts',(44.4367916606371,46.3728243639297,49.2015430558924));
#27860=CARTESIAN_POINT('Ctrl Pts',(44.3944207928808,46.368602676114,49.2681782768304));
#27861=CARTESIAN_POINT('Ctrl Pts',(44.351972081892,46.3643732322658,49.3349359191698));
#27862=CARTESIAN_POINT('Ctrl Pts',(44.3062172138798,46.3601437884176,49.3994824907559));
#27863=CARTESIAN_POINT('Ctrl Pts',(44.2574295424309,46.3559143445693,49.4614875763431));
#27864=CARTESIAN_POINT('Ctrl Pts',(44.2103539895295,46.3518333257031,49.5213167012023));
#27865=CARTESIAN_POINT('Ctrl Pts',(44.160455266942,46.347752306837,49.5787795148342));
#27866=CARTESIAN_POINT('Ctrl Pts',(44.1080108339183,46.3436712879708,49.6336123873545));
#27867=CARTESIAN_POINT('Ctrl Pts',(44.0535718997629,46.3394350648955,49.6905305951521));
#27868=CARTESIAN_POINT('Ctrl Pts',(43.9961814398514,46.3351988418203,49.7448325979865));
#27869=CARTESIAN_POINT('Ctrl Pts',(43.936120942695,46.3309626187451,49.7961967849637));
#27870=CARTESIAN_POINT('Ctrl Pts',(43.876147494277,46.3267325354438,49.8474865272078));
#27871=CARTESIAN_POINT('Ctrl Pts',(43.8135120470264,46.3225024521424,49.895846606812));
#27872=CARTESIAN_POINT('Ctrl Pts',(43.7485337409041,46.3182723688411,49.9409912906923));
#27873=CARTESIAN_POINT('Ctrl Pts',(43.6836313490918,46.3140472275562,49.9860832319308));
#27874=CARTESIAN_POINT('Ctrl Pts',(43.6163919210402,46.3098220862713,50.0279669762023));
#27875=CARTESIAN_POINT('Ctrl Pts',(43.5471673742967,46.3055969449864,50.0663972164735));
#27876=CARTESIAN_POINT('Ctrl Pts',(43.4779871230811,46.3013745072925,50.104802865933));
#27877=CARTESIAN_POINT('Ctrl Pts',(43.4068246834519,46.2971520695987,50.139759170389));
#27878=CARTESIAN_POINT('Ctrl Pts',(43.3340596051936,46.2929296319048,50.1710649679007));
#27879=CARTESIAN_POINT('Ctrl Pts',(43.2613183859169,46.2887085787083,50.2023605005372));
#27880=CARTESIAN_POINT('Ctrl Pts',(43.1869760021201,46.2844875255119,50.2300077177604));
#27881=CARTESIAN_POINT('Ctrl Pts',(43.1114338203614,46.2802664723154,50.2538527813826));
#27882=CARTESIAN_POINT('Ctrl Pts',(43.0358928401895,46.2760454862598,50.2776974657211));
#27883=CARTESIAN_POINT('Ctrl Pts',(42.9591525477985,46.2718245002041,50.297739976718));
#27884=CARTESIAN_POINT('Ctrl Pts',(42.8816299450365,46.2676035141484,50.313876193089));
#27885=CARTESIAN_POINT('Ctrl Pts',(42.8040300298219,46.2633783185491,50.3300285019339));
#27886=CARTESIAN_POINT('Ctrl Pts',(42.7256467061207,46.2591531229497,50.3422666381228));
#27887=CARTESIAN_POINT('Ctrl Pts',(42.6469070693722,46.2549279273503,50.3505376704052));
#27888=CARTESIAN_POINT('Ctrl Pts',(42.5681297338577,46.2507007088224,50.3588126626718));
#27889=CARTESIAN_POINT('Ctrl Pts',(42.4889962145655,46.2464734902945,50.3631167416678));
#27890=CARTESIAN_POINT('Ctrl Pts',(42.4099360502211,46.2422462717666,50.3634491142832));
#27891=CARTESIAN_POINT('Ctrl Pts',(42.3307317140436,46.238011344605,50.3637820930037));
#27892=CARTESIAN_POINT('Ctrl Pts',(42.2516014700193,46.2337764174434,50.3601289143807));
#27893=CARTESIAN_POINT('Ctrl Pts',(42.1729719753434,46.2295414902819,50.352540906535));
#27894=CARTESIAN_POINT('Ctrl Pts',(42.0981105523535,46.2255095087095,50.3453165301439));
#27895=CARTESIAN_POINT('Ctrl Pts',(42.0237033312112,46.2214775271372,50.3345258847114));
#27896=CARTESIAN_POINT('Ctrl Pts',(41.9501083644202,46.2174455455649,50.3202560111193));
#27897=CARTESIAN_POINT('Ctrl Pts',(41.8727846904032,46.2132092826473,50.3052631508462));
#27898=CARTESIAN_POINT('Ctrl Pts',(41.7960649488134,46.2089730197297,50.2863724086812));
#27899=CARTESIAN_POINT('Ctrl Pts',(41.7203719128066,46.204736756812,50.2636466385012));
#27900=CARTESIAN_POINT('Ctrl Pts',(41.6447882987843,46.2005066178435,50.2409537207342));
#27901=CARTESIAN_POINT('Ctrl Pts',(41.570228888495,46.1962764788749,50.214436918126));
#27902=CARTESIAN_POINT('Ctrl Pts',(41.4971066353727,46.1920463399063,50.1842101577028));
#27903=CARTESIAN_POINT('Ctrl Pts',(41.4240693987772,46.1878211191631,50.1540185408109));
#27904=CARTESIAN_POINT('Ctrl Pts',(41.3524664302149,46.1835958984199,50.1201257160476));
#27905=CARTESIAN_POINT('Ctrl Pts',(41.2826944044649,46.1793706776768,50.0826950441882));
#27906=CARTESIAN_POINT('Ctrl Pts',(41.2129667851216,46.1751481460754,50.0452881950803));
#27907=CARTESIAN_POINT('Ctrl Pts',(41.1450682079941,46.170925614474,50.0043481891993));
#27908=CARTESIAN_POINT('Ctrl Pts',(41.0793731559787,46.1667030828726,49.9600855031733));
#27909=CARTESIAN_POINT('Ctrl Pts',(41.0136994210225,46.1624819214194,49.9158371797253));
#27910=CARTESIAN_POINT('Ctrl Pts',(40.9502281801745,46.1582607599662,49.8682685789824));
#27911=CARTESIAN_POINT('Ctrl Pts',(40.8893059061183,46.1540395985131,49.8176341203914));
#27912=CARTESIAN_POINT('Ctrl Pts',(40.8283843952242,46.1498184899376,49.7670002960889));
#27913=CARTESIAN_POINT('Ctrl Pts',(40.7700121475917,46.1455973813621,49.7133009911954));
#27914=CARTESIAN_POINT('Ctrl Pts',(40.7145022701864,46.1413762727866,49.656830662347));
#27915=CARTESIAN_POINT('Ctrl Pts',(40.6589367479696,46.1371509328419,49.600303725901));
#27916=CARTESIAN_POINT('Ctrl Pts',(40.6062396574617,46.1329255928971,49.5410005519791));
#27917=CARTESIAN_POINT('Ctrl Pts',(40.556686505751,46.1287002529523,49.4792517712748));
#27918=CARTESIAN_POINT('Ctrl Pts',(40.5071094875762,46.1244728779417,49.4174732502814));
#27919=CARTESIAN_POINT('Ctrl Pts',(40.4606796999622,46.1202455029312,49.3532471567354));
#27920=CARTESIAN_POINT('Ctrl Pts',(40.4176301137086,46.1160181279206,49.2869343708305));
#27921=CARTESIAN_POINT('Ctrl Pts',(40.3745018326491,46.1117830252526,49.2205003649032));
#27922=CARTESIAN_POINT('Ctrl Pts',(40.334766336029,46.1075479225846,49.1519724513163));
#27923=CARTESIAN_POINT('Ctrl Pts',(40.2986111943904,46.1033128199166,49.0817372733518));
#27924=CARTESIAN_POINT('Ctrl Pts',(40.2641984329235,46.0992818143307,49.0148868527386));
#27925=CARTESIAN_POINT('Ctrl Pts',(40.2330290190821,46.0952508087449,48.9464902572754));
#27926=CARTESIAN_POINT('Ctrl Pts',(40.2052232828249,46.0912198031591,48.8768954342714));
#27927=CARTESIAN_POINT('Ctrl Pts',(40.1722934482226,46.0864459555618,48.7944755339493));
#27928=CARTESIAN_POINT('Ctrl Pts',(40.1439755541144,46.0816721079645,48.7101123332651));
#27929=CARTESIAN_POINT('Ctrl Pts',(40.120474792554,46.0768982603672,48.6243038278903));
#27930=CARTESIAN_POINT('Ctrl Pts',(40.0970606245411,46.0721420030253,48.5388115021787));
#27931=CARTESIAN_POINT('Ctrl Pts',(40.0784282945429,46.0673857456834,48.451884719801));
#27932=CARTESIAN_POINT('Ctrl Pts',(40.0647341399482,46.0626294883415,48.3640381899976));
#27933=CARTESIAN_POINT('Ctrl Pts',(40.0511258291351,46.0579030462842,48.2767423388258));
#27934=CARTESIAN_POINT('Ctrl Pts',(40.0423940921215,46.0531766042269,48.1885384689497));
#27935=CARTESIAN_POINT('Ctrl Pts',(40.0386443754894,46.0484501621696,48.0999502650926));
#27936=CARTESIAN_POINT('Ctrl Pts',(40.0372564615572,46.0467007246988,48.0671603733686));
#27937=CARTESIAN_POINT('Ctrl Pts',(40.0365506126886,46.044951287228,48.0343179932933));
#27938=CARTESIAN_POINT('Ctrl Pts',(40.0365304449332,46.0432018497572,48.0014502318932));
#27939=CARTESIAN_POINT('',(40.0365307281522,45.2494518497012,47.9981447557607));
#27940=CARTESIAN_POINT('Ctrl Pts',(40.0365304449329,46.0432018497283,48.0014502313506));
#27941=CARTESIAN_POINT('Ctrl Pts',(40.0364813749074,46.0389453039821,47.92147987956));
#27942=CARTESIAN_POINT('Ctrl Pts',(40.0404954577654,46.0346887582359,47.8414969742251));
#27943=CARTESIAN_POINT('Ctrl Pts',(40.0485500040157,46.0304322124897,47.7619383330201));
#27944=CARTESIAN_POINT('Ctrl Pts',(40.0566059305006,46.0261749373378,47.6823660585711));
#27945=CARTESIAN_POINT('Ctrl Pts',(40.0687036493595,46.0219176621859,47.6032186482942));
#27946=CARTESIAN_POINT('Ctrl Pts',(40.0847686849002,46.0176603870341,47.5249269545835));
#27947=CARTESIAN_POINT('Ctrl Pts',(40.1013302642617,46.0132715265106,47.444215393414));
#27948=CARTESIAN_POINT('Ctrl Pts',(40.1221083414989,46.0088826659872,47.3644138266163));
#27949=CARTESIAN_POINT('Ctrl Pts',(40.146965226529,46.0044938054638,47.285979866929));
#27950=CARTESIAN_POINT('Ctrl Pts',(40.1711228133691,46.0002284166553,47.2097524880741));
#27951=CARTESIAN_POINT('Ctrl Pts',(40.1991325077043,45.9959630278468,47.1348171927995));
#27952=CARTESIAN_POINT('Ctrl Pts',(40.2308187522828,45.9916976390382,47.0615741076399));
#27953=CARTESIAN_POINT('Ctrl Pts',(40.2638808462144,45.9872470426574,46.9851507323358));
#27954=CARTESIAN_POINT('Ctrl Pts',(40.3009457822569,45.9827964462766,46.9105703714617));
#27955=CARTESIAN_POINT('Ctrl Pts',(40.3417616972024,45.9783458498957,46.8382575458404));
#27956=CARTESIAN_POINT('Ctrl Pts',(40.3825776121478,45.9738952535149,46.7659447202191));
#27957=CARTESIAN_POINT('Ctrl Pts',(40.4271441402953,45.969444657134,46.6958998578033));
#27958=CARTESIAN_POINT('Ctrl Pts',(40.475160823061,45.9649940607532,46.6285100861397));
#27959=CARTESIAN_POINT('Ctrl Pts',(40.5208583018578,45.9607584280099,46.5643752379089));
#27960=CARTESIAN_POINT('Ctrl Pts',(40.5698515301063,45.9565227952666,46.5024049717847));
#27961=CARTESIAN_POINT('Ctrl Pts',(40.6219082101963,45.9522871625233,46.4429579235189));
#27962=CARTESIAN_POINT('Ctrl Pts',(40.6738894361484,45.9480576691653,46.3835970414428));
#27963=CARTESIAN_POINT('Ctrl Pts',(40.7289249895938,45.9438281758073,46.3267524645397));
#27964=CARTESIAN_POINT('Ctrl Pts',(40.7867401564744,45.9395986824493,46.2727527339238));
#27965=CARTESIAN_POINT('Ctrl Pts',(40.844487815944,45.935374127625,46.2188160556557));
#27966=CARTESIAN_POINT('Ctrl Pts',(40.9050082980373,45.9311495728006,46.1677179413873));
#27967=CARTESIAN_POINT('Ctrl Pts',(40.9679886427238,45.9269250179762,46.1197516351472));
#27968=CARTESIAN_POINT('Ctrl Pts',(41.030928717424,45.922703164356,46.0718159988326));
#27969=CARTESIAN_POINT('Ctrl Pts',(41.0963251605837,45.9184813107357,46.0270084796002));
#27970=CARTESIAN_POINT('Ctrl Pts',(41.1638313257595,45.9142594571154,45.9855826029031));
#27971=CARTESIAN_POINT('Ctrl Pts',(41.2313154046507,45.9100389847773,45.9441702796897));
#27972=CARTESIAN_POINT('Ctrl Pts',(41.3009074352502,45.9058185124392,45.9061376473717));
#27973=CARTESIAN_POINT('Ctrl Pts',(41.3722323850144,45.901598040101,45.8716945307389));
#27974=CARTESIAN_POINT('Ctrl Pts',(41.4435562684949,45.8973776308575,45.8372519290189));
#27975=CARTESIAN_POINT('Ctrl Pts',(41.5166125964427,45.893157221614,45.8063989391994));
#27976=CARTESIAN_POINT('Ctrl Pts',(41.5910037258426,45.8889368123705,45.7792984285818));
#27977=CARTESIAN_POINT('Ctrl Pts',(41.6654692406122,45.8847121830445,45.7521708195517));
#27978=CARTESIAN_POINT('Ctrl Pts',(41.7412717810415,45.8804875537185,45.7288033462231));
#27979=CARTESIAN_POINT('Ctrl Pts',(41.8179963668233,45.8762629243925,45.7093096647803));
#27980=CARTESIAN_POINT('Ctrl Pts',(41.8947577790358,45.8720362673199,45.6898066267185));
#27981=CARTESIAN_POINT('Ctrl Pts',(41.9724416575127,45.8678096102473,45.6741811772827));
#27982=CARTESIAN_POINT('Ctrl Pts',(42.0506231235046,45.8635829531747,45.6624957242669));
#27983=CARTESIAN_POINT('Ctrl Pts',(42.1289474554155,45.8593485724654,45.6507889176867));
#27984=CARTESIAN_POINT('Ctrl Pts',(42.2077707234904,45.855114191756,45.6430365404894));
#27985=CARTESIAN_POINT('Ctrl Pts',(42.2866634220723,45.8508798110466,45.6392490048708));
#27986=CARTESIAN_POINT('Ctrl Pts',(42.3618816895894,45.8468426468135,45.6356378738978));
#27987=CARTESIAN_POINT('Ctrl Pts',(42.4371627077019,45.8428054825804,45.6356304479901));
#27988=CARTESIAN_POINT('Ctrl Pts',(42.5121381794019,45.8387683183473,45.6391917761876));
#27989=CARTESIAN_POINT('Ctrl Pts',(42.5907984845178,45.8345327388547,45.6429281336426));
#27990=CARTESIAN_POINT('Ctrl Pts',(42.6694212910057,45.8302971593621,45.6506072440683));
#27991=CARTESIAN_POINT('Ctrl Pts',(42.747579313366,45.8260615798695,45.662227756641));
#27992=CARTESIAN_POINT('Ctrl Pts',(42.8256240675031,45.8218321386664,45.6738314285264));
#27993=CARTESIAN_POINT('Ctrl Pts',(42.9032049148108,45.8176026974633,45.689365091158));
#27994=CARTESIAN_POINT('Ctrl Pts',(42.9798969335152,45.8133732562601,45.7087754393339));
#27995=CARTESIAN_POINT('Ctrl Pts',(43.0564994371497,45.8091487516688,45.7281631317146));
#27996=CARTESIAN_POINT('Ctrl Pts',(43.1322147211502,45.8049242470775,45.7514184033096));
#27997=CARTESIAN_POINT('Ctrl Pts',(43.206626859008,45.8006997424861,45.7784366875493));
#27998=CARTESIAN_POINT('Ctrl Pts',(43.2809914377693,45.7964779379062,45.8054377035688));
#27999=CARTESIAN_POINT('Ctrl Pts',(43.3540540835199,45.7922561333263,45.8361967989557));
#28000=CARTESIAN_POINT('Ctrl Pts',(43.4254140506975,45.7880343287464,45.8705595886402));
#28001=CARTESIAN_POINT('Ctrl Pts',(43.4967506918237,45.7838139041844,45.9049111458616));
#28002=CARTESIAN_POINT('Ctrl Pts',(43.5663853370023,45.7795934796223,45.9428638548478));
#28003=CARTESIAN_POINT('Ctrl Pts',(43.6339386382233,45.7753730550603,45.9842158156193));
#28004=CARTESIAN_POINT('Ctrl Pts',(43.7014909509352,45.7711526922558,46.0255671712864));
#28005=CARTESIAN_POINT('Ctrl Pts',(43.7669615806392,45.7669323294514,46.0703174336924));
#28006=CARTESIAN_POINT('Ctrl Pts',(43.8299984406264,45.7627119666469,46.1182202836926));
#28007=CARTESIAN_POINT('Ctrl Pts',(43.8930983699963,45.7584873813022,46.1661710612574));
#28008=CARTESIAN_POINT('Ctrl Pts',(43.9537592908116,45.7542627959576,46.2172804427092));
#28009=CARTESIAN_POINT('Ctrl Pts',(44.0116611256183,45.7500382106129,46.2712609054369));
#28010=CARTESIAN_POINT('Ctrl Pts',(44.0695907699354,45.7458115962539,46.3252672942902));
#28011=CARTESIAN_POINT('Ctrl Pts',(44.1247583611697,45.741584981895,46.3821471740817));
#28012=CARTESIAN_POINT('Ctrl Pts',(44.1768815691912,45.737358367536,46.4415769733578));
#28013=CARTESIAN_POINT('Ctrl Pts',(44.2291000594114,45.733124026847,46.501115411418));
#28014=CARTESIAN_POINT('Ctrl Pts',(44.2782627537765,45.728889686158,46.5632127143961));
#28015=CARTESIAN_POINT('Ctrl Pts',(44.3241285495196,45.7246553454689,46.6275132912033));
#28016=CARTESIAN_POINT('Ctrl Pts',(44.3678631671639,45.7206177556265,46.6888261082035));
#28017=CARTESIAN_POINT('Ctrl Pts',(44.408600301503,45.716580165784,46.7521416755179));
#28018=CARTESIAN_POINT('Ctrl Pts',(44.4461700576661,45.7125425759415,46.8171312262086));
#28019=CARTESIAN_POINT('Ctrl Pts',(44.4855806562007,45.70830715233,46.8853051339683));
#28020=CARTESIAN_POINT('Ctrl Pts',(44.5216553535162,45.7040717287186,46.955580438681));
#28021=CARTESIAN_POINT('Ctrl Pts',(44.554164114165,45.6998363051072,47.0275970947473));
#28022=CARTESIAN_POINT('Ctrl Pts',(44.586625737438,45.6956070228173,47.0995093273874));
#28023=CARTESIAN_POINT('Ctrl Pts',(44.6155315003955,45.6913777405275,47.173157473115));
#28024=CARTESIAN_POINT('Ctrl Pts',(44.6406963388631,45.6871484582376,47.2481553631864));
#28025=CARTESIAN_POINT('Ctrl Pts',(44.6658317809674,45.6829241163935,47.3230656443018));
#28026=CARTESIAN_POINT('Ctrl Pts',(44.6872348339817,45.6786997745494,47.3993220938773));
#28027=CARTESIAN_POINT('Ctrl Pts',(44.704768410672,45.6744754327053,47.4765183727499));
#28028=CARTESIAN_POINT('Ctrl Pts',(44.7222907712953,45.6702537931336,47.553665269876));
#28029=CARTESIAN_POINT('Ctrl Pts',(44.7359484647868,45.666032153562,47.631750346571));
#28030=CARTESIAN_POINT('Ctrl Pts',(44.7456545142861,45.6618105139903,47.7103530761266));
#28031=CARTESIAN_POINT('Ctrl Pts',(44.7553573862834,45.657590256471,47.7889300732429));
#28032=CARTESIAN_POINT('Ctrl Pts',(44.7611111255918,45.6533699989517,47.8680239212373));
#28033=CARTESIAN_POINT('Ctrl Pts',(44.762880292075,45.6491497414323,47.9472063808419));
#28034=CARTESIAN_POINT('Ctrl Pts',(44.7646494319101,45.6449295474805,48.0263876477634));
#28035=CARTESIAN_POINT('Ctrl Pts',(44.7624341090695,45.6407093535286,48.1056570543583));
#28036=CARTESIAN_POINT('Ctrl Pts',(44.7562509892401,45.6364891595768,48.1845852556551));
#28037=CARTESIAN_POINT('Ctrl Pts',(44.7500616853169,45.6322647447663,48.2635923975843));
#28038=CARTESIAN_POINT('Ctrl Pts',(44.7398966937245,45.6280403299558,48.3422571834517));
#28039=CARTESIAN_POINT('Ctrl Pts',(44.7258246503668,45.6238159151453,48.4201548960159));
#28040=CARTESIAN_POINT('Ctrl Pts',(44.7117458521016,45.6195894725177,48.4980900012906));
#28041=CARTESIAN_POINT('Ctrl Pts',(44.6937563726085,45.61536302989,48.575256841995));
#28042=CARTESIAN_POINT('Ctrl Pts',(44.6719755873081,45.6111365872623,48.6512429435902));
#28043=CARTESIAN_POINT('Ctrl Pts',(44.6501549847554,45.606902418314,48.7273679546755));
#28044=CARTESIAN_POINT('Ctrl Pts',(44.6245293791978,45.6026682493656,48.8023074681743));
#28045=CARTESIAN_POINT('Ctrl Pts',(44.5952673796896,45.5984340804172,48.8756663591636));
#28046=CARTESIAN_POINT('Ctrl Pts',(44.5673536082888,45.5943949981233,48.9456452856793));
#28047=CARTESIAN_POINT('Ctrl Pts',(44.5361313352964,45.5903559158295,49.014185724706));
#28048=CARTESIAN_POINT('Ctrl Pts',(44.5017853702595,45.5863168335356,49.0809665574213));
#28049=CARTESIAN_POINT('Ctrl Pts',(44.4657689987264,45.5820813115931,49.1509952574382));
#28050=CARTESIAN_POINT('Ctrl Pts',(44.4261804483698,45.5778457896507,49.2193550564107));
#28051=CARTESIAN_POINT('Ctrl Pts',(44.3831981053932,45.5736102677082,49.2856576977037));
#28052=CARTESIAN_POINT('Ctrl Pts',(44.3402780710023,45.5693808857144,49.3518642245573));
#28053=CARTESIAN_POINT('Ctrl Pts',(44.2939742669022,45.5651515037207,49.4160191252013));
#28054=CARTESIAN_POINT('Ctrl Pts',(44.2445113775134,45.560922121727,49.4777578350743));
#28055=CARTESIAN_POINT('Ctrl Pts',(44.1951062482349,45.5566976785788,49.5394244497921));
#28056=CARTESIAN_POINT('Ctrl Pts',(44.1425496563542,45.5524732354305,49.5986801161953));
#28057=CARTESIAN_POINT('Ctrl Pts',(44.0871092040993,45.5482487922823,49.6551897094724));
#28058=CARTESIAN_POINT('Ctrl Pts',(44.0317042035504,45.5440270504778,49.7116631673753));
#28059=CARTESIAN_POINT('Ctrl Pts',(43.9734193305794,45.5398053086733,49.7653937032946));
#28060=CARTESIAN_POINT('Ctrl Pts',(43.9125612275284,45.5355835668688,49.8160806628225));
#28061=CARTESIAN_POINT('Ctrl Pts',(43.8517230359666,45.5313632063293,49.8667510386451));
#28062=CARTESIAN_POINT('Ctrl Pts',(43.7883136464435,45.5271428457898,49.9143795152516));
#28063=CARTESIAN_POINT('Ctrl Pts',(43.7226740674798,45.5229224852502,49.9587046107355));
#28064=CARTESIAN_POINT('Ctrl Pts',(43.6570354671272,45.5187021876314,50.0030290453829));
#28065=CARTESIAN_POINT('Ctrl Pts',(43.5891671331395,45.5144818900127,50.0440499352498));
#28066=CARTESIAN_POINT('Ctrl Pts',(43.5194391916917,45.5102615923939,50.081549023445));
#28067=CARTESIAN_POINT('Ctrl Pts',(43.4496415081877,45.5060370736232,50.1190856183191));
#28068=CARTESIAN_POINT('Ctrl Pts',(43.3779809160197,45.5018125548525,50.1530931520212));
#28069=CARTESIAN_POINT('Ctrl Pts',(43.3048517638537,45.4975880360818,50.1833995800931));
#28070=CARTESIAN_POINT('Ctrl Pts',(43.231687503134,45.4933614891631,50.2137205579695));
#28071=CARTESIAN_POINT('Ctrl Pts',(43.1570537205715,45.4891349422444,50.2403367326149));
#28072=CARTESIAN_POINT('Ctrl Pts',(43.0813619174185,45.4849083953257,50.2631253563141));
#28073=CARTESIAN_POINT('Ctrl Pts',(43.0055317583089,45.4806741227627,50.2859556350103));
#28074=CARTESIAN_POINT('Ctrl Pts',(42.928640170997,45.4764398501998,50.3049442696378));
#28075=CARTESIAN_POINT('Ctrl Pts',(42.8511106996711,45.4722055776368,50.3200193054245));
#28076=CARTESIAN_POINT('Ctrl Pts',(42.7771720069113,45.4681674154678,50.3343961407145));
#28077=CARTESIAN_POINT('Ctrl Pts',(42.7026535677558,45.4641292532988,50.3452138526462));
#28078=CARTESIAN_POINT('Ctrl Pts',(42.6279251674152,45.4600910911298,50.3524541566115));
#28079=CARTESIAN_POINT('Ctrl Pts',(42.549544776891,45.4558555832591,50.3600482955162));
#28080=CARTESIAN_POINT('Ctrl Pts',(42.4706354580106,45.4516200753884,50.3637352971135));
#28081=CARTESIAN_POINT('Ctrl Pts',(42.3916202483146,45.4473845675177,50.3634551446266));
#28082=CARTESIAN_POINT('Ctrl Pts',(42.3127195816137,45.4431551995757,50.3631753982577));
#28083=CARTESIAN_POINT('Ctrl Pts',(42.2337137943035,45.4389258316337,50.3589399197566));
#28084=CARTESIAN_POINT('Ctrl Pts',(42.1550310453491,45.4346964636918,50.3507404476371));
#28085=CARTESIAN_POINT('Ctrl Pts',(42.0764401763512,45.4304720344962,50.3425505502612));
#28086=CARTESIAN_POINT('Ctrl Pts',(41.9981720604984,45.4262476053006,50.3304059060715));
#28087=CARTESIAN_POINT('Ctrl Pts',(41.9206533154213,45.4220231761051,50.3143502753221));
#28088=CARTESIAN_POINT('Ctrl Pts',(41.8431841390787,45.4178014481866,50.2983049112159));
#28089=CARTESIAN_POINT('Ctrl Pts',(41.7664638407974,45.4135797202681,50.2783536191345));
#28090=CARTESIAN_POINT('Ctrl Pts',(41.6909111680883,45.4093579923496,50.254591641375));
#28091=CARTESIAN_POINT('Ctrl Pts',(41.6153832131594,45.4051376456098,50.230837437574));
#28092=CARTESIAN_POINT('Ctrl Pts',(41.5410225726666,45.40091729887,50.2032751643405));
#28093=CARTESIAN_POINT('Ctrl Pts',(41.468233640797,45.3966969521302,50.1720501588954));
#28094=CARTESIAN_POINT('Ctrl Pts',(41.3954457923024,45.3924766682052,50.1408256181967));
#28095=CARTESIAN_POINT('Ctrl Pts',(41.3242300367412,45.3882563842802,50.1059386399121));
#28096=CARTESIAN_POINT('Ctrl Pts',(41.2549701672457,45.3840361003551,50.0675824343911));
#28097=CARTESIAN_POINT('Ctrl Pts',(41.1856410192716,45.3798115950122,50.0291878623589));
#28098=CARTESIAN_POINT('Ctrl Pts',(41.1182720771132,45.3755870896693,49.9873173589389));
#28099=CARTESIAN_POINT('Ctrl Pts',(41.0532213720964,45.3713625843265,49.9422095068046));
#28100=CARTESIAN_POINT('Ctrl Pts',(40.9881394349135,45.3671360507127,49.8970799974734));
#28101=CARTESIAN_POINT('Ctrl Pts',(40.9253783244348,45.3629095170989,49.8487103299414));
#28102=CARTESIAN_POINT('Ctrl Pts',(40.8652638913551,45.3586829834851,49.7973801817427));
#28103=CARTESIAN_POINT('Ctrl Pts',(40.8050395703519,45.3544487238564,49.7459562031092));
#28104=CARTESIAN_POINT('Ctrl Pts',(40.747471936393,45.3502144642278,49.6915612531637));
#28105=CARTESIAN_POINT('Ctrl Pts',(40.6928506369372,45.3459802045991,49.6345126163766));
#28106=CARTESIAN_POINT('Ctrl Pts',(40.6407573763549,45.3419419193074,49.5801043629731));
#28107=CARTESIAN_POINT('Ctrl Pts',(40.5913439603892,45.3379036340156,49.5232829229293));
#28108=CARTESIAN_POINT('Ctrl Pts',(40.5448258364757,45.3338653487239,49.4643494336707));
#28109=CARTESIAN_POINT('Ctrl Pts',(40.4960866490667,45.3296342506682,49.4026020944407));
#28110=CARTESIAN_POINT('Ctrl Pts',(40.4503371423291,45.3254031526125,49.338296520154));
#28111=CARTESIAN_POINT('Ctrl Pts',(40.4078575312895,45.3211720545568,49.2717542314694));
#28112=CARTESIAN_POINT('Ctrl Pts',(40.3654379737318,45.31694693801,49.2053060137055));
#28113=CARTESIAN_POINT('Ctrl Pts',(40.3262793873813,45.3127218214632,49.136627749403));
#28114=CARTESIAN_POINT('Ctrl Pts',(40.2906215083225,45.3084967049163,49.0660735526915));
#28115=CARTESIAN_POINT('Ctrl Pts',(40.2550028702488,45.3042762380498,48.9955969998628));
#28116=CARTESIAN_POINT('Ctrl Pts',(40.2228775010959,45.3000557711832,48.9232490303305));
#28117=CARTESIAN_POINT('Ctrl Pts',(40.1944407853412,45.2958353043166,48.8494109673965));
#28118=CARTESIAN_POINT('Ctrl Pts',(40.1660249639791,45.2916179385146,48.7756271583185));
#28119=CARTESIAN_POINT('Ctrl Pts',(40.1412925829797,45.2874005727126,48.7003558668539));
#28120=CARTESIAN_POINT('Ctrl Pts',(40.1203915607568,45.2831832069106,48.6239998434545));
#28121=CARTESIAN_POINT('Ctrl Pts',(40.0994998459173,45.2789677191335,48.5476778219702));
#28122=CARTESIAN_POINT('Ctrl Pts',(40.082436222452,45.2747522313564,48.4702724813342));
#28123=CARTESIAN_POINT('Ctrl Pts',(40.0692987721116,45.2705367435793,48.3922017685062));
#28124=CARTESIAN_POINT('Ctrl Pts',(40.0561590716584,45.2663205337958,48.3141176841405));
#28125=CARTESIAN_POINT('Ctrl Pts',(40.0469469719495,45.2621043240124,48.2353684624106));
#28126=CARTESIAN_POINT('Ctrl Pts',(40.0417092274347,45.2578881142289,48.1563811783223));
#28127=CARTESIAN_POINT('Ctrl Pts',(40.0382158055873,45.255076026062,48.103698978355));
#28128=CARTESIAN_POINT('Ctrl Pts',(40.0364893083885,45.2522639378952,48.0509110511116));
#28129=CARTESIAN_POINT('Ctrl Pts',(40.0365307281518,45.2494518497283,47.9981447562687));
#28130=CARTESIAN_POINT('',(40.0365300816234,44.4557018497661,47.9993788486445));
#28131=CARTESIAN_POINT('Ctrl Pts',(40.0365307281522,45.2494518497012,47.9981447557607));
#28132=CARTESIAN_POINT('Ctrl Pts',(40.0366033020995,45.2445246297871,47.9056899238653));
#28133=CARTESIAN_POINT('Ctrl Pts',(40.0421048202983,45.239597409873,47.8134622725509));
#28134=CARTESIAN_POINT('Ctrl Pts',(40.0529320912302,45.2346701899588,47.7220383614186));
#28135=CARTESIAN_POINT('Ctrl Pts',(40.0638750024599,45.2296903450405,47.6296380003228));
#28136=CARTESIAN_POINT('Ctrl Pts',(40.0802579395256,45.2247105001222,47.5380587616016));
#28137=CARTESIAN_POINT('Ctrl Pts',(40.1019249589366,45.2197306552039,47.4478754247985));
#28138=CARTESIAN_POINT('Ctrl Pts',(40.1194607788405,45.2157003055753,47.3748871322));
#28139=CARTESIAN_POINT('Ctrl Pts',(40.140456810413,45.2116699559466,47.3028128097879));
#28140=CARTESIAN_POINT('Ctrl Pts',(40.1648076914569,45.207639606318,47.231946756579));
#28141=CARTESIAN_POINT('Ctrl Pts',(40.1903980876707,45.2034041027364,47.1574734602552));
#28142=CARTESIAN_POINT('Ctrl Pts',(40.2197632084637,45.1991685991548,47.084138962129));
#28143=CARTESIAN_POINT('Ctrl Pts',(40.2527822542417,45.1949330955732,47.0123531029762));
#28144=CARTESIAN_POINT('Ctrl Pts',(40.2857534331853,45.1907037320887,46.9406713098784));
#28145=CARTESIAN_POINT('Ctrl Pts',(40.3223678237371,45.1864743686043,46.8705341203382));
#28146=CARTESIAN_POINT('Ctrl Pts',(40.3624554064291,45.1822450051198,46.8023345750545));
#28147=CARTESIAN_POINT('Ctrl Pts',(40.4024961755055,45.178020580616,46.734214672071));
#28148=CARTESIAN_POINT('Ctrl Pts',(40.4460018402179,45.1737961561122,46.6680283193652));
#28149=CARTESIAN_POINT('Ctrl Pts',(40.4927556815083,45.1695717316084,46.6041455840664));
#28150=CARTESIAN_POINT('Ctrl Pts',(40.5394796248446,45.1653500085223,46.5403037002365));
#28151=CARTESIAN_POINT('Ctrl Pts',(40.5894473456508,45.1611282854361,46.4787628877371));
#28152=CARTESIAN_POINT('Ctrl Pts',(40.6423985406384,45.1569065623499,46.4198647048592));
#28153=CARTESIAN_POINT('Ctrl Pts',(40.6953324104342,45.1526862205765,46.360985792978));
#28154=CARTESIAN_POINT('Ctrl Pts',(40.7512475025109,45.1484658788031,46.304748142587));
#28155=CARTESIAN_POINT('Ctrl Pts',(40.8098438798882,45.1442455370297,46.2514594787163));
#28156=CARTESIAN_POINT('Ctrl Pts',(40.8684393833551,45.1400252581988,46.1981716095965));
#28157=CARTESIAN_POINT('Ctrl Pts',(40.9297157445013,45.1358049793678,46.1478329543665));
#28158=CARTESIAN_POINT('Ctrl Pts',(40.9933380050967,45.1315847005369,46.1007126407532));
#28159=CARTESIAN_POINT('Ctrl Pts',(41.0570239026048,45.1273602004552,46.0535451959746));
#28160=CARTESIAN_POINT('Ctrl Pts',(41.1230600087996,45.1231357003735,46.0096028033464));
#28161=CARTESIAN_POINT('Ctrl Pts',(41.1910807598299,45.1189112002919,45.9691123340651));
#28162=CARTESIAN_POINT('Ctrl Pts',(41.2591341674404,45.114684672039,45.928602425418));
#28163=CARTESIAN_POINT('Ctrl Pts',(41.3291737025875,45.1104581437862,45.8915479613691));
#28164=CARTESIAN_POINT('Ctrl Pts',(41.4008097497902,45.1062316155333,45.8581294892581));
#28165=CARTESIAN_POINT('Ctrl Pts',(41.4725767445262,45.1019973613733,45.8246499296548));
#28166=CARTESIAN_POINT('Ctrl Pts',(41.5459456469414,45.0977631072133,45.7948198203616));
#28167=CARTESIAN_POINT('Ctrl Pts',(41.6205076318713,45.0935288530533,45.7687711706485));
#28168=CARTESIAN_POINT('Ctrl Pts',(41.6916195367968,45.0894905233396,45.7439278258319));
#28169=CARTESIAN_POINT('Ctrl Pts',(41.7638162025467,45.0854521936259,45.7225238010962));
#28170=CARTESIAN_POINT('Ctrl Pts',(41.8367342512713,45.0814138639122,45.7046302831114));
#28171=CARTESIAN_POINT('Ctrl Pts',(41.9132125189615,45.077178363014,45.68586311528));
#28172=CARTESIAN_POINT('Ctrl Pts',(41.9907751193135,45.0729428621159,45.6708866715058));
#28173=CARTESIAN_POINT('Ctrl Pts',(42.069012013743,45.0687073612177,45.6598210765299));
#28174=CARTESIAN_POINT('Ctrl Pts',(42.1471354899157,45.0644780004294,45.6487715230969));
#28175=CARTESIAN_POINT('Ctrl Pts',(42.2259308582106,45.0602486396411,45.6416216250712));
#28176=CARTESIAN_POINT('Ctrl Pts',(42.3049755817985,45.0560192788528,45.6384410232125));
#28177=CARTESIAN_POINT('Ctrl Pts',(42.3839279980922,45.0517948570513,45.6352641356151));
#28178=CARTESIAN_POINT('Ctrl Pts',(42.4631287244875,45.0475704352499,45.636047351779));
#28179=CARTESIAN_POINT('Ctrl Pts',(42.5421492814504,45.0433460134484,45.6408086082975));
#28180=CARTESIAN_POINT('Ctrl Pts',(42.6211193065925,45.0391242930672,45.6455668201024));
#28181=CARTESIAN_POINT('Ctrl Pts',(42.6999089237416,45.0349025726859,45.6542979950814));
#28182=CARTESIAN_POINT('Ctrl Pts',(42.7780900513668,45.0306808523046,45.6669679912274));
#28183=CARTESIAN_POINT('Ctrl Pts',(42.8562455987824,45.0264605132348,45.6796338418569));
#28184=CARTESIAN_POINT('Ctrl Pts',(42.93379258905,45.022240174165,45.6962358795983));
#28185=CARTESIAN_POINT('Ctrl Pts',(43.0103099538483,45.0180198350952,45.7166883258885));
#28186=CARTESIAN_POINT('Ctrl Pts',(43.0868261775518,45.0137995589629,45.7371404671738));
#28187=CARTESIAN_POINT('Ctrl Pts',(43.1623123532194,45.0095792828305,45.7614427803804));
#28188=CARTESIAN_POINT('Ctrl Pts',(43.2363609277338,45.0053590066982,45.7894591522751));
#28189=CARTESIAN_POINT('Ctrl Pts',(43.3104835684002,45.0011345092879,45.8175035471921));
#28190=CARTESIAN_POINT('Ctrl Pts',(43.3831652954117,44.9969100118777,45.8492692553728));
#28191=CARTESIAN_POINT('Ctrl Pts',(43.4540175371904,44.9926855144674,45.8845715629701));
#28192=CARTESIAN_POINT('Ctrl Pts',(43.5249037951369,44.9884589888755,45.9198908192084));
#28193=CARTESIAN_POINT('Ctrl Pts',(43.5939584085004,44.9842324632837,45.9587498268391));
#28194=CARTESIAN_POINT('Ctrl Pts',(43.660818753645,44.9800059376918,46.0009185831095));
#28195=CARTESIAN_POINT('Ctrl Pts',(43.7278013174142,44.975771686143,46.0431644225505));
#28196=CARTESIAN_POINT('Ctrl Pts',(43.7925812130381,44.9715374345943,46.0887318294391));
#28197=CARTESIAN_POINT('Ctrl Pts',(43.8548262464889,44.9673031830455,46.137348386459));
#28198=CARTESIAN_POINT('Ctrl Pts',(43.9141915126665,44.9632648291991,46.183715697843));
#28199=CARTESIAN_POINT('Ctrl Pts',(43.9712510336822,44.9592264753528,46.2328560001001));
#28200=CARTESIAN_POINT('Ctrl Pts',(44.0257483506338,44.9551881215064,46.2845021884854));
#28201=CARTESIAN_POINT('Ctrl Pts',(44.082906129461,44.9509526224233,46.3386696517316));
#28202=CARTESIAN_POINT('Ctrl Pts',(44.1374624215625,44.9467171233403,46.3957998168079));
#28203=CARTESIAN_POINT('Ctrl Pts',(44.189094371249,44.9424816242572,46.4556128167894));
#28204=CARTESIAN_POINT('Ctrl Pts',(44.2406514707316,44.9382522653252,46.5153391065988));
#28205=CARTESIAN_POINT('Ctrl Pts',(44.2892923423664,44.9340229063932,46.5777401556207));
#28206=CARTESIAN_POINT('Ctrl Pts',(44.3347298274189,44.9297935474612,46.6424982741095));
#28207=CARTESIAN_POINT('Ctrl Pts',(44.3801142506296,44.9255691275696,46.7071807681435));
#28208=CARTESIAN_POINT('Ctrl Pts',(44.4223024529642,44.921344707678,46.7742144795354));
#28209=CARTESIAN_POINT('Ctrl Pts',(44.4610475453567,44.9171202877864,46.8432487490047));
#28210=CARTESIAN_POINT('Ctrl Pts',(44.4997678608552,44.9128985693467,46.9122388721146));
#28211=CARTESIAN_POINT('Ctrl Pts',(44.5350492074518,44.908676850907,46.9832266059233));
#28212=CARTESIAN_POINT('Ctrl Pts',(44.566688710933,44.9044551324673,47.0558334517599));
#28213=CARTESIAN_POINT('Ctrl Pts',(44.598317862011,44.9002347953682,47.128416540734));
#28214=CARTESIAN_POINT('Ctrl Pts',(44.6263073487521,44.8960144582691,47.2026172598375));
#28215=CARTESIAN_POINT('Ctrl Pts',(44.6505015188027,44.89179412117,47.278035073728));
#28216=CARTESIAN_POINT('Ctrl Pts',(44.6746953278965,44.8875738470348,47.3534517624478));
#28217=CARTESIAN_POINT('Ctrl Pts',(44.6950937907522,44.8833535728996,47.4300850625351));
#28218=CARTESIAN_POINT('Ctrl Pts',(44.7115908994855,44.8791332987644,47.5075185746487));
#28219=CARTESIAN_POINT('Ctrl Pts',(44.7281045091421,44.8749088033792,47.5850295381794));
#28220=CARTESIAN_POINT('Ctrl Pts',(44.7407088713939,44.870684307994,47.6633418524846));
#28221=CARTESIAN_POINT('Ctrl Pts',(44.7493491216818,44.8664598126088,47.7420287896819));
#28222=CARTESIAN_POINT('Ctrl Pts',(44.7579935201187,44.8622332890606,47.8207535041575));
#28223=CARTESIAN_POINT('Ctrl Pts',(44.7626699875375,44.8580067655124,47.8998527306407));
#28224=CARTESIAN_POINT('Ctrl Pts',(44.7633757862348,44.8537802419642,47.9788970632581));
#28225=CARTESIAN_POINT('Ctrl Pts',(44.7640828751094,44.8495459924666,48.0580858863779));
#28226=CARTESIAN_POINT('Ctrl Pts',(44.7608048110432,44.845311742969,48.1372191449375));
#28227=CARTESIAN_POINT('Ctrl Pts',(44.7535909903321,44.8410774934714,48.2158700792777));
#28228=CARTESIAN_POINT('Ctrl Pts',(44.7467108837934,44.8370391220145,48.2908825905824));
#28229=CARTESIAN_POINT('Ctrl Pts',(44.7362511936526,44.8330007505575,48.3654560672734));
#28230=CARTESIAN_POINT('Ctrl Pts',(44.7222978216176,44.8289623791005,48.4392303138562));
#28231=CARTESIAN_POINT('Ctrl Pts',(44.7076633288885,44.8247268783501,48.516605780697));
#28232=CARTESIAN_POINT('Ctrl Pts',(44.6891297353807,44.8204913775997,48.5933961188597));
#28233=CARTESIAN_POINT('Ctrl Pts',(44.6667577552311,44.8162558768493,48.6691783917608));
#28234=CARTESIAN_POINT('Ctrl Pts',(44.6444182073185,44.8120265162244,48.7448508045328));
#28235=CARTESIAN_POINT('Ctrl Pts',(44.6182514545177,44.8077971555994,48.8195176077341));
#28236=CARTESIAN_POINT('Ctrl Pts',(44.5883693327607,44.8035677949744,48.892765425144));
#28237=CARTESIAN_POINT('Ctrl Pts',(44.5585221070795,44.7993433733592,48.9659277044048));
#28238=CARTESIAN_POINT('Ctrl Pts',(44.5249683107645,44.7951189517439,49.0376738584772));
#28239=CARTESIAN_POINT('Ctrl Pts',(44.4878692935888,44.7908945301286,49.1076065428613));
#28240=CARTESIAN_POINT('Ctrl Pts',(44.4507940004999,44.7866728099473,49.1774945066785));
#28241=CARTESIAN_POINT('Ctrl Pts',(44.4101782056166,44.782451089766,49.2455708890191));
#28242=CARTESIAN_POINT('Ctrl Pts',(44.3662304840665,44.7782293695847,49.3114603022691));
#28243=CARTESIAN_POINT('Ctrl Pts',(44.3222971419844,44.7740090307284,49.3773281568426));
#28244=CARTESIAN_POINT('Ctrl Pts',(44.2750342982299,44.7697886918722,49.4410100730306));
#28245=CARTESIAN_POINT('Ctrl Pts',(44.2246946079982,44.765568353016,49.5021584565026));
#28246=CARTESIAN_POINT('Ctrl Pts',(44.1743556686358,44.7613480771105,49.5633059278825));
#28247=CARTESIAN_POINT('Ctrl Pts',(44.1209402733613,44.7571278012051,49.6219195801549));
#28248=CARTESIAN_POINT('Ctrl Pts',(44.064741276658,44.7529075252996,49.6776849891118));
#28249=CARTESIAN_POINT('Ctrl Pts',(44.0084860678758,44.7486830281359,49.733506176459));
#28250=CARTESIAN_POINT('Ctrl Pts',(43.9494420297357,44.7444585309721,49.7864730980574));
#28251=CARTESIAN_POINT('Ctrl Pts',(43.8879383714039,44.7402340338083,49.8363087550311));
#28252=CARTESIAN_POINT('Ctrl Pts',(43.8264051853199,44.7360075084741,49.8861683379789));
#28253=CARTESIAN_POINT('Ctrl Pts',(43.7624104062164,44.7317809831398,49.9328933843703));
#28254=CARTESIAN_POINT('Ctrl Pts',(43.6963136956999,44.7275544578055,49.9762492867148));
#28255=CARTESIAN_POINT('Ctrl Pts',(43.6300961627024,44.7233202065304,50.0196844421363));
#28256=CARTESIAN_POINT('Ctrl Pts',(43.5617694265342,44.7190859552553,50.0597379090438));
#28257=CARTESIAN_POINT('Ctrl Pts',(43.4917191273015,44.7148517039801,50.0962203576876));
#28258=CARTESIAN_POINT('Ctrl Pts',(43.4249096700583,44.7108133482183,50.1310149641275));
#28259=CARTESIAN_POINT('Ctrl Pts',(43.3565329421062,44.7067749924565,50.1625615514277));
#28260=CARTESIAN_POINT('Ctrl Pts',(43.2869383457606,44.7027366366947,50.1907375040656));
#28261=CARTESIAN_POINT('Ctrl Pts',(43.2139462788801,44.6985011363925,50.220288950979));
#28262=CARTESIAN_POINT('Ctrl Pts',(43.1393369414077,44.6942656360903,50.2462445959887));
#28263=CARTESIAN_POINT('Ctrl Pts',(43.0634988806087,44.6900301357881,50.2684266962657));
#28264=CARTESIAN_POINT('Ctrl Pts',(42.9877707608884,44.6858007756148,50.2905766395492));
#28265=CARTESIAN_POINT('Ctrl Pts',(42.9108179017726,44.6815714154415,50.3089637707813));
#28266=CARTESIAN_POINT('Ctrl Pts',(42.833048466458,44.6773420552683,50.3234585140687));
#28267=CARTESIAN_POINT('Ctrl Pts',(42.7553698496655,44.6731176341079,50.3379363305113));
#28268=CARTESIAN_POINT('Ctrl Pts',(42.6768770106461,44.6688932129475,50.3485307062118));
#28269=CARTESIAN_POINT('Ctrl Pts',(42.5979914160436,44.664668791787,50.3551623808292));
#28270=CARTESIAN_POINT('Ctrl Pts',(42.5191562672544,44.6604470720623,50.3617898146188));
#28271=CARTESIAN_POINT('Ctrl Pts',(42.4399293278184,44.6562253523376,50.3644595377019));
#28272=CARTESIAN_POINT('Ctrl Pts',(42.3607391465437,44.6520036326129,50.3631438860734));
#28273=CARTESIAN_POINT('Ctrl Pts',(42.2815748759114,44.6477832942144,50.3618286649196));
#28274=CARTESIAN_POINT('Ctrl Pts',(42.2024478084901,44.6435629558158,50.3565306661472));
#28275=CARTESIAN_POINT('Ctrl Pts',(42.1237869651027,44.6393426174173,50.3472743342551));
#28276=CARTESIAN_POINT('Ctrl Pts',(42.0451272950326,44.63512234197,50.3380181404319));
#28277=CARTESIAN_POINT('Ctrl Pts',(41.9669343011522,44.6309020665227,50.3248037870308));
#28278=CARTESIAN_POINT('Ctrl Pts',(41.8896308547567,44.6266817910753,50.3077074720345));
#28279=CARTESIAN_POINT('Ctrl Pts',(41.8122500868648,44.6224572943672,50.2905940567312));
#28280=CARTESIAN_POINT('Ctrl Pts',(41.7357611032287,44.618232797659,50.2695910249086));
#28281=CARTESIAN_POINT('Ctrl Pts',(41.6605749669654,44.6140083009508,50.2448253966449));
#28282=CARTESIAN_POINT('Ctrl Pts',(41.5853527340113,44.6097817760715,50.2200478784601));
#28283=CARTESIAN_POINT('Ctrl Pts',(41.5114350329334,44.6055552511922,50.1915043345427));
#28284=CARTESIAN_POINT('Ctrl Pts',(41.4392137490155,44.6013287263129,50.1593703297071));
#28285=CARTESIAN_POINT('Ctrl Pts',(41.3668604469842,44.5970944754862,50.1271775849756));
#28286=CARTESIAN_POINT('Ctrl Pts',(41.2962101784068,44.5928602246595,50.0913814771134));
#28287=CARTESIAN_POINT('Ctrl Pts',(41.2276308028632,44.5886259738328,50.0522039144551));
#28288=CARTESIAN_POINT('Ctrl Pts',(41.1622241446536,44.5845876139848,50.0148388403353));
#28289=CARTESIAN_POINT('Ctrl Pts',(41.0987012852547,44.5805492541368,49.9743984905189));
#28290=CARTESIAN_POINT('Ctrl Pts',(41.0373543723427,44.5765108942888,49.9311103889541));
#28291=CARTESIAN_POINT('Ctrl Pts',(40.9734456513011,44.5723038950978,49.8860146037548));
#28292=CARTESIAN_POINT('Ctrl Pts',(40.9116484640583,44.5680968959068,49.837651354278));
#28293=CARTESIAN_POINT('Ctrl Pts',(40.8523197968065,44.5638898967158,49.7862464638294));
#28294=CARTESIAN_POINT('Ctrl Pts',(40.7930773333072,44.5596890102379,49.7349162639925));
#28295=CARTESIAN_POINT('Ctrl Pts',(40.7362966266365,44.5554881237599,49.6805535054133));
#28296=CARTESIAN_POINT('Ctrl Pts',(40.6823050293388,44.5512872372819,49.6234267549432));
#28297=CARTESIAN_POINT('Ctrl Pts',(40.62837581227,44.5470912043788,49.5663660069613));
#28298=CARTESIAN_POINT('Ctrl Pts',(40.5772296285932,44.5428951714757,49.5065479552999));
#28299=CARTESIAN_POINT('Ctrl Pts',(40.5291588834611,44.5386991385726,49.4442797366049));
#28300=CARTESIAN_POINT('Ctrl Pts',(40.4811179883224,44.5345057112367,49.3820501839615));
#28301=CARTESIAN_POINT('Ctrl Pts',(40.4361490329949,44.5303122839007,49.3173738591201));
#28302=CARTESIAN_POINT('Ctrl Pts',(40.3945049441187,44.5261188565648,49.2505918685708));
#28303=CARTESIAN_POINT('Ctrl Pts',(40.3528732643496,44.5219266787864,49.1838297777216));
#28304=CARTESIAN_POINT('Ctrl Pts',(40.3145647359826,44.5177345010081,49.1149636708361));
#28305=CARTESIAN_POINT('Ctrl Pts',(40.2797887364826,44.5135423232298,49.0443632696307));
#28306=CARTESIAN_POINT('Ctrl Pts',(40.2450118677341,44.5093500406653,48.9737611037231));
#28307=CARTESIAN_POINT('Ctrl Pts',(40.2137679116889,44.5051577581008,48.9014249857457));
#28308=CARTESIAN_POINT('Ctrl Pts',(40.1862193708099,44.5009654755363,48.8277474051441));
#28309=CARTESIAN_POINT('Ctrl Pts',(40.1586435762283,44.4967690455572,48.753996935496));
#28310=CARTESIAN_POINT('Ctrl Pts',(40.1347706618192,44.492572615578,48.6789028011075));
#28311=CARTESIAN_POINT('Ctrl Pts',(40.1147139350392,44.4883761855988,48.6028748146972));
#28312=CARTESIAN_POINT('Ctrl Pts',(40.0946464483958,44.4841775043543,48.5268060414345));
#28313=CARTESIAN_POINT('Ctrl Pts',(40.0783993219462,44.4799788231098,48.449802885319));
#28314=CARTESIAN_POINT('Ctrl Pts',(40.0660346410796,44.4757801418653,48.3722850309365));
#28315=CARTESIAN_POINT('Ctrl Pts',(40.0536493071805,44.4715744474597,48.2946376965637));
#28316=CARTESIAN_POINT('Ctrl Pts',(40.0451594155884,44.467368753054,48.2164744211785));
#28317=CARTESIAN_POINT('Ctrl Pts',(40.0405750864627,44.4631630586483,48.1382190952057));
#28318=CARTESIAN_POINT('Ctrl Pts',(40.037864108291,44.4606759890209,48.0919422082909));
#28319=CARTESIAN_POINT('Ctrl Pts',(40.0365179253812,44.4581889193935,48.0456331351725));
#28320=CARTESIAN_POINT('Ctrl Pts',(40.0365300816234,44.4557018497661,47.9993788486445));
#28321=CARTESIAN_POINT('',(40.0365310047746,43.6619518497613,48.0021793366867));
#28322=CARTESIAN_POINT('Ctrl Pts',(40.0365300816236,44.4557018497283,47.9993788479416));
#28323=CARTESIAN_POINT('Ctrl Pts',(40.0365389068377,44.4538962837798,47.9657991026046));
#28324=CARTESIAN_POINT('Ctrl Pts',(40.0372633394702,44.4520907178314,47.9322296454892));
#28325=CARTESIAN_POINT('Ctrl Pts',(40.0387022762554,44.450285151883,47.8986910628888));
#28326=CARTESIAN_POINT('Ctrl Pts',(40.0420777371408,44.4460496515486,47.8200161864904));
#28327=CARTESIAN_POINT('Ctrl Pts',(40.0493959105134,44.4418141512142,47.7413606516739));
#28328=CARTESIAN_POINT('Ctrl Pts',(40.0606574248334,44.4375786508797,47.6631517301321));
#28329=CARTESIAN_POINT('Ctrl Pts',(40.0719026135347,44.4333492906754,47.5850561866845));
#28330=CARTESIAN_POINT('Ctrl Pts',(40.0870797247141,44.4291199304711,47.507406431426));
#28331=CARTESIAN_POINT('Ctrl Pts',(40.1061374221056,44.4248905702667,47.4306276133884));
#28332=CARTESIAN_POINT('Ctrl Pts',(40.1251728640626,44.4206661490772,47.3539384570727));
#28333=CARTESIAN_POINT('Ctrl Pts',(40.1480797743804,44.4164417278876,47.2781186700249));
#28334=CARTESIAN_POINT('Ctrl Pts',(40.1747555143851,44.412217306698,47.203584643455));
#28335=CARTESIAN_POINT('Ctrl Pts',(40.2014141957622,44.4079955869454,47.1290982799758));
#28336=CARTESIAN_POINT('Ctrl Pts',(40.2318367655739,44.4037738671927,47.0558964857531));
#28337=CARTESIAN_POINT('Ctrl Pts',(40.2658706969478,44.39955214744,46.9843807018602));
#28338=CARTESIAN_POINT('Ctrl Pts',(40.2998934925749,44.3953318090147,46.9128883176051));
#28339=CARTESIAN_POINT('Ctrl Pts',(40.3375251019218,44.3911114705895,46.8430812717631));
#28340=CARTESIAN_POINT('Ctrl Pts',(40.3785653847968,44.3868911321642,46.775339827806));
#28341=CARTESIAN_POINT('Ctrl Pts',(40.419605055496,44.3826708566914,46.7075993943114));
#28342=CARTESIAN_POINT('Ctrl Pts',(40.4640530543128,44.3784505812186,46.6419249021921));
#28343=CARTESIAN_POINT('Ctrl Pts',(40.5116646964617,44.3742303057459,46.5786695590712));
#28344=CARTESIAN_POINT('Ctrl Pts',(40.5593239613443,44.3700058090144,46.5153509458712));
#28345=CARTESIAN_POINT('Ctrl Pts',(40.6101529078774,44.365781312283,46.454456691243));
#28346=CARTESIAN_POINT('Ctrl Pts',(40.6638655006203,44.3615568155516,46.3963081839195));
#28347=CARTESIAN_POINT('Ctrl Pts',(40.71760388064,44.3573302906503,46.338131759648));
#28348=CARTESIAN_POINT('Ctrl Pts',(40.7742283289578,44.3531037657489,46.2827040375186));
#28349=CARTESIAN_POINT('Ctrl Pts',(40.8334165876995,44.3488772408475,46.2303088254713));
#28350=CARTESIAN_POINT('Ctrl Pts',(40.8927130405837,44.3446429900011,46.1778178367419));
#28351=CARTESIAN_POINT('Ctrl Pts',(40.9545823011305,44.3404087391546,46.1283707287589));
#28352=CARTESIAN_POINT('Ctrl Pts',(41.0186699022907,44.3361744883081,46.082210229962));
#28353=CARTESIAN_POINT('Ctrl Pts',(41.0797925871386,44.3321361286977,46.0381852770958));
#28354=CARTESIAN_POINT('Ctrl Pts',(41.1429325758987,44.3280977690873,45.9971497222663));
#28355=CARTESIAN_POINT('Ctrl Pts',(41.2077616859249,44.3240594094768,45.9592750691601));
#28356=CARTESIAN_POINT('Ctrl Pts',(41.275755559475,44.3198239092118,45.919551488611));
#28357=CARTESIAN_POINT('Ctrl Pts',(41.3458661400769,44.3155884089467,45.8831543034111));
#28358=CARTESIAN_POINT('Ctrl Pts',(41.4177344202536,44.3113529086816,45.8503151924653));
#28359=CARTESIAN_POINT('Ctrl Pts',(41.4894985142388,44.3071235485474,45.8175236878055));
#28360=CARTESIAN_POINT('Ctrl Pts',(41.5630148244236,44.3028941884131,45.7882802077816));
#28361=CARTESIAN_POINT('Ctrl Pts',(41.6378980160727,44.2986648282789,45.7627715791645));
#28362=CARTESIAN_POINT('Ctrl Pts',(41.7126937596841,44.2944404071601,45.7372927393354));
#28363=CARTESIAN_POINT('Ctrl Pts',(41.7888527707718,44.2902159860414,45.7155402342941));
#28364=CARTESIAN_POINT('Ctrl Pts',(41.8659693260067,44.2859915649227,45.6976530061404));
#28365=CARTESIAN_POINT('Ctrl Pts',(41.9430365666652,44.2817698452413,45.6797772165303));
#28366=CARTESIAN_POINT('Ctrl Pts',(42.0210596801459,44.2775481255598,45.6657619036346));
#28367=CARTESIAN_POINT('Ctrl Pts',(42.0996185275127,44.2733264058784,45.6556959642814));
#28368=CARTESIAN_POINT('Ctrl Pts',(42.1781516707776,44.2691060675247,45.6456333184584));
#28369=CARTESIAN_POINT('Ctrl Pts',(42.2572197346683,44.264885729171,45.6395175398692));
#28370=CARTESIAN_POINT('Ctrl Pts',(42.3363946328045,44.2606653908173,45.6373860243019));
#28371=CARTESIAN_POINT('Ctrl Pts',(42.4155683499277,44.2564451154163,45.6352545405294));
#28372=CARTESIAN_POINT('Ctrl Pts',(42.4948484289113,44.2522248400153,45.6371072129401));
#28373=CARTESIAN_POINT('Ctrl Pts',(42.5738054398561,44.2480045646143,45.6429293370846));
#28374=CARTESIAN_POINT('Ctrl Pts',(42.6528414262107,44.2437800679545,45.64875728471));
#28375=CARTESIAN_POINT('Ctrl Pts',(42.731553229808,44.2395555712946,45.6585625807997));
#28376=CARTESIAN_POINT('Ctrl Pts',(42.8095158109758,44.2353310746348,45.6722785300941));
#28377=CARTESIAN_POINT('Ctrl Pts',(42.8875158217775,44.231104549805,45.6860010643803));
#28378=CARTESIAN_POINT('Ctrl Pts',(42.9647654353776,44.2268780249753,45.7036378874573));
#28379=CARTESIAN_POINT('Ctrl Pts',(43.0408516225767,44.2226515001455,45.7250715090929));
#28380=CARTESIAN_POINT('Ctrl Pts',(43.1170768927797,44.2184172493698,45.7465443106716));
#28381=CARTESIAN_POINT('Ctrl Pts',(43.1921340409633,44.2141829985941,45.7718276291732));
#28382=CARTESIAN_POINT('Ctrl Pts',(43.2656271620513,44.2099487478184,45.8007546618854));
#28383=CARTESIAN_POINT('Ctrl Pts',(43.3357202468722,44.2059103875694,45.8283434338343));
#28384=CARTESIAN_POINT('Ctrl Pts',(43.4043905078659,44.2018720273204,45.8592460549525));
#28385=CARTESIAN_POINT('Ctrl Pts',(43.4713161614431,44.1978336670714,45.8932792963634));
#28386=CARTESIAN_POINT('Ctrl Pts',(43.5415089141829,44.1935981668218,45.9289739331971));
#28387=CARTESIAN_POINT('Ctrl Pts',(43.6100491956043,44.1893626665722,45.968248331619));
#28388=CARTESIAN_POINT('Ctrl Pts',(43.6765479372573,44.1851271663226,46.0109258925862));
#28389=CARTESIAN_POINT('Ctrl Pts',(43.7429502768371,44.1808978062043,46.0535415846329));
#28390=CARTESIAN_POINT('Ctrl Pts',(43.8073165622004,44.1766684460859,46.0995503907936));
#28391=CARTESIAN_POINT('Ctrl Pts',(43.8692812039775,44.1724390859676,46.1487293054395));
#28392=CARTESIAN_POINT('Ctrl Pts',(43.931173483894,44.1682146648655,46.1978507893045));
#28393=CARTESIAN_POINT('Ctrl Pts',(43.9906693278038,44.1639902437633,46.2501347347698));
#28394=CARTESIAN_POINT('Ctrl Pts',(44.0474323886332,44.1597658226611,46.3053150836269));
#28395=CARTESIAN_POINT('Ctrl Pts',(44.1041591505548,44.1555441029967,46.3604601456908));
#28396=CARTESIAN_POINT('Ctrl Pts',(44.1581562623044,44.1513223833322,46.4184976086617));
#28397=CARTESIAN_POINT('Ctrl Pts',(44.2091216675651,44.1471006636677,46.4791222163348));
#28398=CARTESIAN_POINT('Ctrl Pts',(44.2600703971697,44.1428803253313,46.5397269879032));
#28399=CARTESIAN_POINT('Ctrl Pts',(44.3079890881949,44.1386599869949,46.6029168643068));
#28400=CARTESIAN_POINT('Ctrl Pts',(44.3526146986442,44.1344396486585,46.6683520436922));
#28401=CARTESIAN_POINT('Ctrl Pts',(44.3972396434315,44.1302193732751,46.7337862470079));
#28402=CARTESIAN_POINT('Ctrl Pts',(44.4385713419416,44.1259990978918,46.801465298217));
#28403=CARTESIAN_POINT('Ctrl Pts',(44.476389843107,44.1217788225084,46.8710200797436));
#28404=CARTESIAN_POINT('Ctrl Pts',(44.5142461715825,44.1175543258667,46.9406444322529));
#28405=CARTESIAN_POINT('Ctrl Pts',(44.548582058289,44.1133298292249,47.0121478496339));
#28406=CARTESIAN_POINT('Ctrl Pts',(44.5792236529652,44.1091053325832,47.0851367800284));
#28407=CARTESIAN_POINT('Ctrl Pts',(44.6098799585901,44.1048788077717,47.1581607522156));
#28408=CARTESIAN_POINT('Ctrl Pts',(44.6368382790136,44.1006522829603,47.2326712162209));
#28409=CARTESIAN_POINT('Ctrl Pts',(44.6599739815353,44.0964257581489,47.3082572416832));
#28410=CARTESIAN_POINT('Ctrl Pts',(44.6831519753458,44.0921915073917,47.3839814358669));
#28411=CARTESIAN_POINT('Ctrl Pts',(44.702493273436,44.0879572566346,47.4607846638789));
#28412=CARTESIAN_POINT('Ctrl Pts',(44.7179239802904,44.0837230058774,47.5382437195935));
#28413=CARTESIAN_POINT('Ctrl Pts',(44.7326408119428,44.0796846454734,47.6121192648726));
#28414=CARTESIAN_POINT('Ctrl Pts',(44.7438008675764,44.0756462850694,47.6865909396363));
#28415=CARTESIAN_POINT('Ctrl Pts',(44.7513841656328,44.0716079246653,47.7612889895468));
#28416=CARTESIAN_POINT('Ctrl Pts',(44.7593376561077,44.0673724243897,47.8396335599491));
#28417=CARTESIAN_POINT('Ctrl Pts',(44.7633864936398,44.0631369241141,47.9185249761328));
#28418=CARTESIAN_POINT('Ctrl Pts',(44.7634687202651,44.0589014238385,47.997540482027));
#28419=CARTESIAN_POINT('Ctrl Pts',(44.7635508276879,44.0546720636938,48.0764414405206));
#28420=CARTESIAN_POINT('Ctrl Pts',(44.7596777428528,44.050442703549,48.1554656661121));
#28421=CARTESIAN_POINT('Ctrl Pts',(44.75183923902,44.0462133434043,48.2341850437283));
#28422=CARTESIAN_POINT('Ctrl Pts',(44.7440098889341,44.0419889222752,48.3128124934352));
#28423=CARTESIAN_POINT('Ctrl Pts',(44.7322243683506,44.037764501146,48.3911353379879));
#28424=CARTESIAN_POINT('Ctrl Pts',(44.7165244787904,44.0335400800169,48.4687267648265));
#28425=CARTESIAN_POINT('Ctrl Pts',(44.7008346290126,44.0293183603252,48.546268573416));
#28426=CARTESIAN_POINT('Ctrl Pts',(44.6812354713363,44.0250966406335,48.623079433845));
#28427=CARTESIAN_POINT('Ctrl Pts',(44.6578203249055,44.0208749209417,48.698740167261));
#28428=CARTESIAN_POINT('Ctrl Pts',(44.6344128398059,44.0166545825778,48.7743761448232));
#28429=CARTESIAN_POINT('Ctrl Pts',(44.6071919838615,44.0124342442139,48.8488622945803));
#28430=CARTESIAN_POINT('Ctrl Pts',(44.5763012364911,44.0082139058499,48.9217935609165));
#28431=CARTESIAN_POINT('Ctrl Pts',(44.5454109499037,44.0039936304388,48.9947237393711));
#28432=CARTESIAN_POINT('Ctrl Pts',(44.5108510649889,43.9997733550277,49.0660986488462));
#28433=CARTESIAN_POINT('Ctrl Pts',(44.472813028337,43.9955530796166,49.135533614851));
#28434=CARTESIAN_POINT('Ctrl Pts',(44.4347369447869,43.9913285829469,49.2050380319977));
#28435=CARTESIAN_POINT('Ctrl Pts',(44.3931759858738,43.9871040862772,49.272598216875));
#28436=CARTESIAN_POINT('Ctrl Pts',(44.3483670882485,43.9828795896075,49.3378550483256));
#28437=CARTESIAN_POINT('Ctrl Pts',(44.3035366779883,43.978653064768,49.4031432094106));
#28438=CARTESIAN_POINT('Ctrl Pts',(44.2554555078394,43.9744265399285,49.4661254405331));
#28439=CARTESIAN_POINT('Ctrl Pts',(44.2044017565428,43.9702000150889,49.5264746122636));
#28440=CARTESIAN_POINT('Ctrl Pts',(44.1532546807014,43.9659657643038,49.5869341002556));
#28441=CARTESIAN_POINT('Ctrl Pts',(44.0991244873708,43.9617315135187,49.6447505675384));
#28442=CARTESIAN_POINT('Ctrl Pts',(44.0423271279393,43.9574972627335,49.6996329149951));
#28443=CARTESIAN_POINT('Ctrl Pts',(43.9881574046413,43.9534589025755,49.7519762211881));
#28444=CARTESIAN_POINT('Ctrl Pts',(43.9315621344702,43.9494205424176,49.80165068022));
#28445=CARTESIAN_POINT('Ctrl Pts',(43.8728414812907,43.9453821822596,49.8484394531305));
#28446=CARTESIAN_POINT('Ctrl Pts',(43.8112542695525,43.9411466819943,49.8975123075383));
#28447=CARTESIAN_POINT('Ctrl Pts',(43.7470947611614,43.9369111817289,49.9435970781654));
#28448=CARTESIAN_POINT('Ctrl Pts',(43.6806849871049,43.9326756814635,49.9864129491886));
#28449=CARTESIAN_POINT('Ctrl Pts',(43.6143714861415,43.9284463213291,50.0291667507891));
#28450=CARTESIAN_POINT('Ctrl Pts',(43.5458145887447,43.9242169611948,50.0686608111637));
#28451=CARTESIAN_POINT('Ctrl Pts',(43.4753688191252,43.9199876010604,50.1046549227257));
#28452=CARTESIAN_POINT('Ctrl Pts',(43.4050053155588,43.9157631799417,50.1406070006282));
#28453=CARTESIAN_POINT('Ctrl Pts',(43.3327577389102,43.9115387588231,50.1730670393305));
#28454=CARTESIAN_POINT('Ctrl Pts',(43.2590076647864,43.9073143377044,50.2018392931225));
#28455=CARTESIAN_POINT('Ctrl Pts',(43.1853047524407,43.9030926180232,50.2305931476022));
#28456=CARTESIAN_POINT('Ctrl Pts',(43.1101016857122,43.8988708983421,50.2556637277048));
#28457=CARTESIAN_POINT('Ctrl Pts',(43.0338014906415,43.8946491786609,50.2769027452574));
#28458=CARTESIAN_POINT('Ctrl Pts',(42.9575262606545,43.8904288403075,50.2981348134981));
#28459=CARTESIAN_POINT('Ctrl Pts',(42.8801550669499,43.8862085019542,50.3155376827934));
#28460=CARTESIAN_POINT('Ctrl Pts',(42.8021061938115,43.8819881636009,50.3290128917201));
#28461=CARTESIAN_POINT('Ctrl Pts',(42.7240584848924,43.8777678882004,50.3424878996433));
#28462=CARTESIAN_POINT('Ctrl Pts',(42.6453335793691,43.8735476127999,50.3520352851183));
#28463=CARTESIAN_POINT('Ctrl Pts',(42.5663585702586,43.8693273373994,50.3576079544745));
#28464=CARTESIAN_POINT('Ctrl Pts',(42.4873045677405,43.8651028407404,50.3631861977983));
#28465=CARTESIAN_POINT('Ctrl Pts',(42.4080004312113,43.8608783440813,50.3647817500414));
#28466=CARTESIAN_POINT('Ctrl Pts',(42.3288763723535,43.8566538474222,50.3623996000868));
#28467=CARTESIAN_POINT('Ctrl Pts',(42.2497143262418,43.8524273225933,50.3600163064683));
#28468=CARTESIAN_POINT('Ctrl Pts',(42.1707329985079,43.8482007977645,50.3536515440794));
#28469=CARTESIAN_POINT('Ctrl Pts',(42.0923580065131,43.8439742729356,50.3433622948113));
#28470=CARTESIAN_POINT('Ctrl Pts',(42.0138397476598,43.839740022161,50.3330542371404));
#28471=CARTESIAN_POINT('Ctrl Pts',(41.9359305022217,43.8355057713864,50.3188074422433));
#28472=CARTESIAN_POINT('Ctrl Pts',(41.8590460197369,43.8312715206118,50.3007301519599));
#28473=CARTESIAN_POINT('Ctrl Pts',(41.7857184690927,43.8272331603591,50.2834891772415));
#28474=CARTESIAN_POINT('Ctrl Pts',(41.7133232936402,43.8231948001064,50.2627644257604));
#28475=CARTESIAN_POINT('Ctrl Pts',(41.6422052471526,43.8191564398537,50.2386910357298));
#28476=CARTESIAN_POINT('Ctrl Pts',(41.567615441922,43.8149209395893,50.2134424587187));
#28477=CARTESIAN_POINT('Ctrl Pts',(41.4941471084168,43.810685439325,50.1844139801348));
#28478=CARTESIAN_POINT('Ctrl Pts',(41.4222106366493,43.8064499390606,50.151724518106));
#28479=CARTESIAN_POINT('Ctrl Pts',(41.350378449933,43.8022205789273,50.1190824454213));
#28480=CARTESIAN_POINT('Ctrl Pts',(41.2800741386975,43.7979912187939,50.0827901211133));
#28481=CARTESIAN_POINT('Ctrl Pts',(41.2116915188455,43.7937618586606,50.0430157597327));
#28482=CARTESIAN_POINT('Ctrl Pts',(41.1433887557167,43.7895374375431,50.0032878465604));
#28483=CARTESIAN_POINT('Ctrl Pts',(41.0770036280594,43.7853130164255,49.9600862115607));
#28484=CARTESIAN_POINT('Ctrl Pts',(41.0129071926658,43.781088595308,49.9136258737647));
#28485=CARTESIAN_POINT('Ctrl Pts',(40.9488517457316,43.776866875628,49.8671952464769));
#28486=CARTESIAN_POINT('Ctrl Pts',(40.8870824651688,43.772645155948,49.8175103271596));
#28487=CARTESIAN_POINT('Ctrl Pts',(40.827942099151,43.7684234362679,49.7648298493844));
#28488=CARTESIAN_POINT('Ctrl Pts',(40.7688210835978,43.7642030979158,49.7121666084272));
#28489=CARTESIAN_POINT('Ctrl Pts',(40.7123276247838,43.7599827595637,49.6565100671843));
#28490=CARTESIAN_POINT('Ctrl Pts',(40.6587708197668,43.7557624212116,49.5981587476857));
#28491=CARTESIAN_POINT('Ctrl Pts',(40.6052148136326,43.7515421458123,49.5398082985876));
#28492=CARTESIAN_POINT('Ctrl Pts',(40.5545956906101,43.7473218704131,49.4787634978217));
#28493=CARTESIAN_POINT('Ctrl Pts',(40.5071841114854,43.7431015950139,49.4153580653272));
#28494=CARTESIAN_POINT('Ctrl Pts',(40.4597251097368,43.7388770983561,49.3518892126294));
#28495=CARTESIAN_POINT('Ctrl Pts',(40.4154803425935,43.7346526016983,49.2860553882291));
#28496=CARTESIAN_POINT('Ctrl Pts',(40.3746783551241,43.7304281050406,49.2182211111687));
#28497=CARTESIAN_POINT('Ctrl Pts',(40.3338567787273,43.726201580213,49.1503542670495));
#28498=CARTESIAN_POINT('Ctrl Pts',(40.2964814964142,43.7219750553854,49.0804854714386));
#28499=CARTESIAN_POINT('Ctrl Pts',(40.2627348401853,43.7177485305579,49.0090035072002));
#28500=CARTESIAN_POINT('Ctrl Pts',(40.2289264962002,43.7135142797846,48.9373908763276));
#28501=CARTESIAN_POINT('Ctrl Pts',(40.1987602118412,43.7092800290114,48.8641596195118));
#28502=CARTESIAN_POINT('Ctrl Pts',(40.1723698696445,43.7050457782381,48.789717951697));
#28503=CARTESIAN_POINT('Ctrl Pts',(40.1472004323646,43.7010074179747,48.7187202027812));
#28504=CARTESIAN_POINT('Ctrl Pts',(40.1254653561815,43.6969690577113,48.6466219139841));
#28505=CARTESIAN_POINT('Ctrl Pts',(40.107237494923,43.6929306974479,48.573786141531));
#28506=CARTESIAN_POINT('Ctrl Pts',(40.0822668479016,43.6873984812843,48.4740072185593));
#28507=CARTESIAN_POINT('Ctrl Pts',(40.0637993296254,43.6818662651206,48.3725403527942));
#28508=CARTESIAN_POINT('Ctrl Pts',(40.0520163089416,43.676334048957,48.2701166922342));
#28509=CARTESIAN_POINT('Ctrl Pts',(40.0418054672349,43.6715399825584,48.1813591645122));
#28510=CARTESIAN_POINT('Ctrl Pts',(40.0366137200381,43.6667459161599,48.0918832185466));
#28511=CARTESIAN_POINT('Ctrl Pts',(40.0365310047746,43.6619518497613,48.0021793366867));
#28512=CARTESIAN_POINT('',(40.0365300407226,42.8682018496837,47.9995612592237));
#28513=CARTESIAN_POINT('Ctrl Pts',(40.0365310047741,43.6619518497283,48.0021793360685));
#28514=CARTESIAN_POINT('Ctrl Pts',(40.0364589799385,43.657777385097,47.9240690949938));
#28515=CARTESIAN_POINT('Ctrl Pts',(40.0402633944012,43.6536029204657,47.8458562414444));
#28516=CARTESIAN_POINT('Ctrl Pts',(40.047948045871,43.6494284558344,47.767961111066));
#28517=CARTESIAN_POINT('Ctrl Pts',(40.0556277589757,43.6452566738271,47.6901160382075));
#28518=CARTESIAN_POINT('Ctrl Pts',(40.0671827163339,43.6410848918198,47.6125887614653));
#28519=CARTESIAN_POINT('Ctrl Pts',(40.0825646803434,43.6369131098125,47.535797479425));
#28520=CARTESIAN_POINT('Ctrl Pts',(40.0979418366337,43.6327426317191,47.4590301989312));
#28521=CARTESIAN_POINT('Ctrl Pts',(40.1171435311434,43.6285721536257,47.3829989284983));
#28522=CARTESIAN_POINT('Ctrl Pts',(40.1400701839293,43.6244016755323,47.308112966349));
#28523=CARTESIAN_POINT('Ctrl Pts',(40.1629972380133,43.6202311244407,47.2332256934285));
#28524=CARTESIAN_POINT('Ctrl Pts',(40.1896492365983,43.6160605733491,47.1594842284149));
#28525=CARTESIAN_POINT('Ctrl Pts',(40.2198768503229,43.6118900222574,47.0872823584798));
#28526=CARTESIAN_POINT('Ctrl Pts',(40.2501347668174,43.6077152902453,47.0150081071564));
#28527=CARTESIAN_POINT('Ctrl Pts',(40.283975266881,43.6035405582332,46.9442769767219));
#28528=CARTESIAN_POINT('Ctrl Pts',(40.32120133412,43.5993658262211,46.875461629096));
#28529=CARTESIAN_POINT('Ctrl Pts',(40.3584475512711,43.5951888344891,46.806609032754));
#28530=CARTESIAN_POINT('Ctrl Pts',(40.3990827308522,43.5910118427571,46.7396746935101));
#28531=CARTESIAN_POINT('Ctrl Pts',(40.4428658481235,43.5868348510251,46.6750032632272));
#28532=CARTESIAN_POINT('Ctrl Pts',(40.4867236541362,43.5826507338467,46.6102215112487));
#28533=CARTESIAN_POINT('Ctrl Pts',(40.5337398262852,43.5784666166684,46.5477107572811));
#28534=CARTESIAN_POINT('Ctrl Pts',(40.5836327163485,43.57428249949,46.4877829746427));
#28535=CARTESIAN_POINT('Ctrl Pts',(40.6137518212058,43.5717566513406,46.4516060531041));
#28536=CARTESIAN_POINT('Ctrl Pts',(40.6449185295089,43.5692308031913,46.4163697355742));
#28537=CARTESIAN_POINT('Ctrl Pts',(40.6770647487152,43.566704955042,46.3821358027387));
#28538=CARTESIAN_POINT('Ctrl Pts',(40.7309695410664,43.562469454776,46.3247302015069));
#28539=CARTESIAN_POINT('Ctrl Pts',(40.7878489354429,43.5582339545099,46.2699124753785));
#28540=CARTESIAN_POINT('Ctrl Pts',(40.8474245481059,43.5539984542439,46.2180067600926));
#28541=CARTESIAN_POINT('Ctrl Pts',(40.9069137950403,43.5497690941088,46.1661762916185));
#28542=CARTESIAN_POINT('Ctrl Pts',(40.9690911474661,43.5455397339738,46.1172497565619));
#28543=CARTESIAN_POINT('Ctrl Pts',(41.033640235542,43.5413103738387,46.071515767508));
#28544=CARTESIAN_POINT('Ctrl Pts',(41.098113943666,43.5370859527194,46.0258351862713));
#28545=CARTESIAN_POINT('Ctrl Pts',(41.1649535025596,43.5328615316002,45.9833400122769));
#28546=CARTESIAN_POINT('Ctrl Pts',(41.2338093885432,43.5286371104809,45.9442787400404));
#28547=CARTESIAN_POINT('Ctrl Pts',(41.3026212424893,43.524415390799,45.9052424467491));
#28548=CARTESIAN_POINT('Ctrl Pts',(41.3734464572018,43.5201936711172,45.8696359277568));
#28549=CARTESIAN_POINT('Ctrl Pts',(41.4459074680793,43.5159719514354,45.8376637908426));
#28550=CARTESIAN_POINT('Ctrl Pts',(41.5183447700367,43.5117516130814,45.8057021150693));
#28551=CARTESIAN_POINT('Ctrl Pts',(41.592416376295,43.5075312747275,45.7773726494351));
#28552=CARTESIAN_POINT('Ctrl Pts',(41.6677224692794,43.5033109363735,45.7528328814034));
#28553=CARTESIAN_POINT('Ctrl Pts',(41.7430274389571,43.4990906609724,45.7282934794203));
#28554=CARTESIAN_POINT('Ctrl Pts',(41.8195664120887,43.4948703855714,45.7075438068233));
#28555=CARTESIAN_POINT('Ctrl Pts',(41.8969234796218,43.4906501101703,45.6906917798734));
#28556=CARTESIAN_POINT('Ctrl Pts',(41.9743579222437,43.4864256135106,45.6738228969707));
#28557=CARTESIAN_POINT('Ctrl Pts',(42.0526116342033,43.482201116851,45.66085954771));
#28558=CARTESIAN_POINT('Ctrl Pts',(42.1312581434926,43.4779766201913,45.6518585529272));
#28559=CARTESIAN_POINT('Ctrl Pts',(42.2099424107654,43.4737500953619,45.6428532367904));
#28560=CARTESIAN_POINT('Ctrl Pts',(42.2890193819993,43.4695235705324,45.6378140946676));
#28561=CARTESIAN_POINT('Ctrl Pts',(42.3680596681864,43.465297045703,45.636745833368));
#28562=CARTESIAN_POINT('Ctrl Pts',(42.4472444373668,43.4610627949278,45.6356756193225));
#28563=CARTESIAN_POINT('Ctrl Pts',(42.5263919172336,43.4568285441527,45.6385907732392));
#28564=CARTESIAN_POINT('Ctrl Pts',(42.6050751258938,43.4525942933775,45.6454438563416));
#28565=CARTESIAN_POINT('Ctrl Pts',(42.6801181875456,43.4485559331304,45.6519798930197));
#28566=CARTESIAN_POINT('Ctrl Pts',(42.75473863647,43.4445175728833,45.6620974688143));
#28567=CARTESIAN_POINT('Ctrl Pts',(42.8285758901674,43.4404792126362,45.6757123355171));
#28568=CARTESIAN_POINT('Ctrl Pts',(42.9060176458659,43.4362437123701,45.6899918371003));
#28569=CARTESIAN_POINT('Ctrl Pts',(42.9828921603495,43.4320082121041,45.7081730808793));
#28570=CARTESIAN_POINT('Ctrl Pts',(43.0587762231309,43.4277727118381,45.7301972929928));
#28571=CARTESIAN_POINT('Ctrl Pts',(43.1345502781076,43.423543351703,45.7521895769894));
#28572=CARTESIAN_POINT('Ctrl Pts',(43.2093362857701,43.419313991568,45.778013636414));
#28573=CARTESIAN_POINT('Ctrl Pts',(43.2827203614424,43.4150846314329,45.8075595323031));
#28574=CARTESIAN_POINT('Ctrl Pts',(43.3560187397288,43.4108602103136,45.8370709247114));
#28575=CARTESIAN_POINT('Ctrl Pts',(43.4279180062527,43.4066357891943,45.8702953422259));
#28576=CARTESIAN_POINT('Ctrl Pts',(43.498020080816,43.4024113680751,45.9070732590401));
#28577=CARTESIAN_POINT('Ctrl Pts',(43.5680773264276,43.3981896483933,45.9438276570717));
#28578=CARTESIAN_POINT('Ctrl Pts',(43.6363392466317,43.3939679287114,45.9841308267216));
#28579=CARTESIAN_POINT('Ctrl Pts',(43.7024295013073,43.3897462090296,46.0277759166301));
#28580=CARTESIAN_POINT('Ctrl Pts',(43.7684981315458,43.3855258706757,46.0714067260595));
#28581=CARTESIAN_POINT('Ctrl Pts',(43.8323961158317,43.3813055323218,46.1183770260475));
#28582=CARTESIAN_POINT('Ctrl Pts',(43.893774704883,43.3770851939678,46.1684357581696));
#28583=CARTESIAN_POINT('Ctrl Pts',(43.9551523783777,43.3728649185668,46.2184937435884));
#28584=CARTESIAN_POINT('Ctrl Pts',(44.0140103684607,43.3686446431657,46.2716397718904));
#28585=CARTESIAN_POINT('Ctrl Pts',(44.0700329112701,43.3644243677647,46.3275824336683));
#28586=CARTESIAN_POINT('Ctrl Pts',(44.1261114896733,43.360199871105,46.3835810511404));
#28587=CARTESIAN_POINT('Ctrl Pts',(44.1793486224083,43.3559753744454,46.4423815575808));
#28588=CARTESIAN_POINT('Ctrl Pts',(44.2294658038304,43.3517508777858,46.50365601765));
#28589=CARTESIAN_POINT('Ctrl Pts',(44.2796070463803,43.3475243529564,46.5649598954272));
#28590=CARTESIAN_POINT('Ctrl Pts',(44.3266250747688,43.343297828127,46.6287397146439));
#28591=CARTESIAN_POINT('Ctrl Pts',(44.3702836346383,43.3390713032976,46.6946368934368));
#28592=CARTESIAN_POINT('Ctrl Pts',(44.4140220008917,43.3348370525225,46.7606545300633));
#28593=CARTESIAN_POINT('Ctrl Pts',(44.4543883876324,43.3306028017473,46.8287968554796));
#28594=CARTESIAN_POINT('Ctrl Pts',(44.4911916986327,43.3263685509722,46.8986791019554));
#28595=CARTESIAN_POINT('Ctrl Pts',(44.5262923660251,43.3223301907249,46.9653283632178));
#28596=CARTESIAN_POINT('Ctrl Pts',(44.5581522286103,43.3182918304776,47.0335597774958));
#28597=CARTESIAN_POINT('Ctrl Pts',(44.5866470694326,43.3142534702303,47.1030245072234));
#28598=CARTESIAN_POINT('Ctrl Pts',(44.6165329385733,43.3100179699639,47.1758802861161));
#28599=CARTESIAN_POINT('Ctrl Pts',(44.6428304603488,43.3057824696975,47.250369808548));
#28600=CARTESIAN_POINT('Ctrl Pts',(44.6653601119542,43.3015469694311,47.326105346462));
#28601=CARTESIAN_POINT('Ctrl Pts',(44.687857102716,43.2973176092956,47.4017310918857));
#28602=CARTESIAN_POINT('Ctrl Pts',(44.7065969376097,43.2930882491602,47.4785988196821));
#28603=CARTESIAN_POINT('Ctrl Pts',(44.7214481703021,43.2888588890248,47.556300965179));
#28604=CARTESIAN_POINT('Ctrl Pts',(44.7362820598338,43.2846344679051,47.6339123706798));
#28605=CARTESIAN_POINT('Ctrl Pts',(44.747236283483,43.2804100467855,47.7123557989017));
#28606=CARTESIAN_POINT('Ctrl Pts',(44.7542296489309,43.2761856256658,47.791210151122));
#28607=CARTESIAN_POINT('Ctrl Pts',(44.7612185422539,43.2719639059836,47.8700140774744));
#28608=CARTESIAN_POINT('Ctrl Pts',(44.7642515632779,43.2677421863014,47.9492279400133));
#28609=CARTESIAN_POINT('Ctrl Pts',(44.7632990829994,43.2635204666192,48.028423321309));
#28610=CARTESIAN_POINT('Ctrl Pts',(44.7623469143682,43.2593001282649,48.1075927902289));
#28611=CARTESIAN_POINT('Ctrl Pts',(44.7574118394623,43.2550797899105,48.1867433209506));
#28612=CARTESIAN_POINT('Ctrl Pts',(44.7485163350697,43.2508594515562,48.2654457850688));
#28613=CARTESIAN_POINT('Ctrl Pts',(44.7396209633673,43.2466391761548,48.344147075218));
#28614=CARTESIAN_POINT('Ctrl Pts',(44.7267653336476,43.2424189007533,48.4223998458172));
#28615=CARTESIAN_POINT('Ctrl Pts',(44.7100237038394,43.2381986253519,48.4997808805869));
#28616=CARTESIAN_POINT('Ctrl Pts',(44.6932653285012,43.2339741286918,48.5772393144182));
#28617=CARTESIAN_POINT('Ctrl Pts',(44.6726132879773,43.2297496320318,48.6538238107783));
#28618=CARTESIAN_POINT('Ctrl Pts',(44.6481927159089,43.2255251353718,48.7291227283758));
#28619=CARTESIAN_POINT('Ctrl Pts',(44.6237604195877,43.221298610542,48.8044577967868));
#28620=CARTESIAN_POINT('Ctrl Pts',(44.595556154744,43.2170720857122,48.8785056176767));
#28621=CARTESIAN_POINT('Ctrl Pts',(44.5637536871924,43.2128455608824,48.9508735047636));
#28622=CARTESIAN_POINT('Ctrl Pts',(44.5318930857963,43.2086113101068,49.0233736779219));
#28623=CARTESIAN_POINT('Ctrl Pts',(44.4964213492767,43.2043770593313,49.0941873602226));
#28624=CARTESIAN_POINT('Ctrl Pts',(44.4575586966613,43.2001428085558,49.1629456783073));
#28625=CARTESIAN_POINT('Ctrl Pts',(44.4204939596841,43.196104448312,49.2285230077814));
#28626=CARTESIAN_POINT('Ctrl Pts',(44.380345339802,43.1920660880683,49.292230660774));
#28627=CARTESIAN_POINT('Ctrl Pts',(44.3373390188821,43.1880277278245,49.3537754491853));
#28628=CARTESIAN_POINT('Ctrl Pts',(44.2922332648856,43.1837922275583,49.4183246602425));
#28629=CARTESIAN_POINT('Ctrl Pts',(44.2438122213345,43.1795567272921,49.480739811804));
#28630=CARTESIAN_POINT('Ctrl Pts',(44.1923048580973,43.1753212270259,49.5406601625734));
#28631=CARTESIAN_POINT('Ctrl Pts',(44.1408721641878,43.1710918668906,49.6004936478535));
#28632=CARTESIAN_POINT('Ctrl Pts',(44.0863623388966,43.1668625067554,49.6578391614924));
#28633=CARTESIAN_POINT('Ctrl Pts',(44.0290470442044,43.1626331466202,49.7123656644154));
#28634=CARTESIAN_POINT('Ctrl Pts',(43.9717986818932,43.1584087255008,49.7668284916881));
#28635=CARTESIAN_POINT('Ctrl Pts',(43.9117516988982,43.1541843043813,49.8184785282764));
#28636=CARTESIAN_POINT('Ctrl Pts',(43.8492163267107,43.1499598832618,49.8670196783364));
#28637=CARTESIAN_POINT('Ctrl Pts',(43.7867209447117,43.1457381635798,49.9155297872484));
#28638=CARTESIAN_POINT('Ctrl Pts',(43.7217407016284,43.1415164438979,49.960934668518));
#28639=CARTESIAN_POINT('Ctrl Pts',(43.6546198795043,43.1372947242159,50.0029776331384));
#28640=CARTESIAN_POINT('Ctrl Pts',(43.5875210190141,43.1330743858617,50.0450068414881));
#28641=CARTESIAN_POINT('Ctrl Pts',(43.5182833676833,43.1288540475076,50.0836760684711));
#28642=CARTESIAN_POINT('Ctrl Pts',(43.4472799942956,43.1246337091535,50.1187720628818));
#28643=CARTESIAN_POINT('Ctrl Pts',(43.3762776800328,43.1204134337522,50.1538675337815));
#28644=CARTESIAN_POINT('Ctrl Pts',(43.3035101174174,43.116193158351,50.1853896712794));
#28645=CARTESIAN_POINT('Ctrl Pts',(43.2293734161261,43.1119728829497,50.2131719719722));
#28646=CARTESIAN_POINT('Ctrl Pts',(43.1551625608627,43.1077483862899,50.2409820614379));
#28647=CARTESIAN_POINT('Ctrl Pts',(43.0795802718135,43.1035238896301,50.2650446764673));
#28648=CARTESIAN_POINT('Ctrl Pts',(43.0030404470927,43.0992993929703,50.2852423635296));
#28649=CARTESIAN_POINT('Ctrl Pts',(42.9264638758024,43.0950728681406,50.3054497474486));
#28650=CARTESIAN_POINT('Ctrl Pts',(42.8489293129374,43.090846343311,50.3217884100212));
#28651=CARTESIAN_POINT('Ctrl Pts',(42.7708610245089,43.0866198184814,50.3341920532382));
#28652=CARTESIAN_POINT('Ctrl Pts',(42.6926500298663,43.0823855677061,50.3466183698991));
#28653=CARTESIAN_POINT('Ctrl Pts',(42.6139038280005,43.0781513169308,50.3550952433692));
#28654=CARTESIAN_POINT('Ctrl Pts',(42.5350517883784,43.0739170661555,50.3596083266839));
#28655=CARTESIAN_POINT('Ctrl Pts',(42.4598477064768,43.0698787059099,50.3639126197478));
#28656=CARTESIAN_POINT('Ctrl Pts',(42.3845477205658,43.0658403456642,50.3646118016675));
#28657=CARTESIAN_POINT('Ctrl Pts',(42.3095207725316,43.0618019854186,50.3617374854748));
#28658=CARTESIAN_POINT('Ctrl Pts',(42.2308312453366,43.0575664851523,50.3587228542237));
#28659=CARTESIAN_POINT('Ctrl Pts',(42.1521429786395,43.0533309848861,50.3517654633841));
#28660=CARTESIAN_POINT('Ctrl Pts',(42.0738832367456,43.0490954846199,50.3408627250705));
#28661=CARTESIAN_POINT('Ctrl Pts',(41.9957369466373,43.0448661244846,50.3299757922668));
#28662=CARTESIAN_POINT('Ctrl Pts',(41.918018408619,43.0406367643494,50.3151549341235));
#28663=CARTESIAN_POINT('Ctrl Pts',(41.8411530026631,43.0364074042142,50.2964495366691));
#28664=CARTESIAN_POINT('Ctrl Pts',(41.7643773595648,43.0321829830947,50.2777659832406));
#28665=CARTESIAN_POINT('Ctrl Pts',(41.6884533224055,43.0279585619752,50.2552070154485));
#28666=CARTESIAN_POINT('Ctrl Pts',(41.6137977486969,43.0237341408558,50.2288733613523));
#28667=CARTESIAN_POINT('Ctrl Pts',(41.5391899158165,43.0195124211738,50.2025565471302));
#28668=CARTESIAN_POINT('Ctrl Pts',(41.4658493778377,43.0152907014918,50.1724699932682));
#28669=CARTESIAN_POINT('Ctrl Pts',(41.3941782710748,43.0110689818097,50.1387643840596));
#28670=CARTESIAN_POINT('Ctrl Pts',(41.3225306147789,43.0068486434556,50.1050698031764));
#28671=CARTESIAN_POINT('Ctrl Pts',(41.2525517294732,43.0026283051015,50.0677587178443));
#28672=CARTESIAN_POINT('Ctrl Pts',(41.1846227924436,42.9984079667474,50.0270295222942));
#28673=CARTESIAN_POINT('Ctrl Pts',(41.1166948686789,42.9941876913461,49.9863009342829));
#28674=CARTESIAN_POINT('Ctrl Pts',(41.0508172342608,42.9899674159448,49.9421545799041));
#28675=CARTESIAN_POINT('Ctrl Pts',(40.9873442151886,42.9857471405436,49.8948335215894));
#28676=CARTESIAN_POINT('Ctrl Pts',(40.9238077083106,42.9815226438837,49.8474651311925));
#28677=CARTESIAN_POINT('Ctrl Pts',(40.8626809986058,42.9772981472239,49.7969159747142));
#28678=CARTESIAN_POINT('Ctrl Pts',(40.8042867831472,42.9730736505641,49.7434706107248));
#28679=CARTESIAN_POINT('Ctrl Pts',(40.7458645327784,42.9688471257345,49.6899995877559));
#28680=CARTESIAN_POINT('Ctrl Pts',(40.6901777203547,42.9646206009049,49.6336299216627));
#28681=CARTESIAN_POINT('Ctrl Pts',(40.6375116286636,42.9603940760752,49.5746825654093));
#28682=CARTESIAN_POINT('Ctrl Pts',(40.5847492651227,42.9561598252999,49.5156274553649));
#28683=CARTESIAN_POINT('Ctrl Pts',(40.5350189515994,42.9519255745246,49.453985605871));
#28684=CARTESIAN_POINT('Ctrl Pts',(40.488565039521,42.9476913237493,49.3901103671143));
#28685=CARTESIAN_POINT('Ctrl Pts',(40.4442602399847,42.9436529635038,49.329190209439));
#28686=CARTESIAN_POINT('Ctrl Pts',(40.4029355568504,42.9396146032582,49.2662390593534));
#28687=CARTESIAN_POINT('Ctrl Pts',(40.3647639970915,42.9355762430127,49.2015843097199));
#28688=CARTESIAN_POINT('Ctrl Pts',(40.3232516974056,42.9311844491795,49.1312710356526));
#28689=CARTESIAN_POINT('Ctrl Pts',(40.2853206180267,42.9267926553463,49.0586920893796));
#28690=CARTESIAN_POINT('Ctrl Pts',(40.2512151199357,42.9224008615132,48.9842326859574));
#28691=CARTESIAN_POINT('Ctrl Pts',(40.2161405322847,42.9178842771978,48.907657558252));
#28692=CARTESIAN_POINT('Ctrl Pts',(40.1851125221882,42.9133676928824,48.8290938244295));
#28693=CARTESIAN_POINT('Ctrl Pts',(40.1583484050748,42.9088511085669,48.7489917008013));
#28694=CARTESIAN_POINT('Ctrl Pts',(40.1324271131578,42.9044767553981,48.6714120623272));
#28695=CARTESIAN_POINT('Ctrl Pts',(40.1105053531251,42.9001024022292,48.5923899091533));
#28696=CARTESIAN_POINT('Ctrl Pts',(40.0927330828449,42.8957280490603,48.5123571155957));
#28697=CARTESIAN_POINT('Ctrl Pts',(40.0740940202823,42.8911403491716,48.4284209485972));
#28698=CARTESIAN_POINT('Ctrl Pts',(40.0600197140069,42.886552649283,48.3433734694791));
#28699=CARTESIAN_POINT('Ctrl Pts',(40.050624681986,42.8819649493943,48.2577325280336));
#28700=CARTESIAN_POINT('Ctrl Pts',(40.0412296499651,42.8773772495056,48.1720915865882));
#28701=CARTESIAN_POINT('Ctrl Pts',(40.0365140211838,42.872789549617,48.085857708865));
#28702=CARTESIAN_POINT('Ctrl Pts',(40.0365300407225,42.8682018497283,47.9995612600632));
#28703=CARTESIAN_POINT('',(40.0365308527828,42.0744518497637,47.9979922519359));
#28704=CARTESIAN_POINT('Ctrl Pts',(40.0365300407226,42.8682018496837,47.9995612592237));
#28705=CARTESIAN_POINT('Ctrl Pts',(40.0365457119377,42.8637139118291,47.9151413737289));
#28706=CARTESIAN_POINT('Ctrl Pts',(40.0410886773983,42.8592259739746,47.830834979817));
#28707=CARTESIAN_POINT('Ctrl Pts',(40.0500971862548,42.8547380361201,47.7471221503326));
#28708=CARTESIAN_POINT('Ctrl Pts',(40.0591375370619,42.8502342349637,47.6631134250652));
#28709=CARTESIAN_POINT('Ctrl Pts',(40.0726749541952,42.8457304338073,47.5797028312392));
#28710=CARTESIAN_POINT('Ctrl Pts',(40.0905962313369,42.8412266326509,47.4973622833642));
#28711=CARTESIAN_POINT('Ctrl Pts',(40.1085512889131,42.8367143421241,47.4148665289462));
#28712=CARTESIAN_POINT('Ctrl Pts',(40.1309065954803,42.8322020515973,47.3334452030884));
#28713=CARTESIAN_POINT('Ctrl Pts',(40.1574993385981,42.8276897610705,47.253554272226));
#28714=CARTESIAN_POINT('Ctrl Pts',(40.1841701190507,42.8231642290693,47.1734288986327));
#28715=CARTESIAN_POINT('Ctrl Pts',(40.2151030608842,42.8186386970682,47.0948432455739));
#28716=CARTESIAN_POINT('Ctrl Pts',(40.2500872145016,42.814113165067,47.0182335024811));
#28717=CARTESIAN_POINT('Ctrl Pts',(40.2623596416297,42.812525610247,46.9913588351764));
#28718=CARTESIAN_POINT('Ctrl Pts',(40.2751302065365,42.8109380554269,46.9647270873352));
#28719=CARTESIAN_POINT('Ctrl Pts',(40.2883885151456,42.8093505006069,46.9383562848436));
#28720=CARTESIAN_POINT('Ctrl Pts',(40.3237608808337,42.8051150003407,46.8680005783414));
#28721=CARTESIAN_POINT('Ctrl Pts',(40.3627205485394,42.8008795000744,46.7992809094294));
#28722=CARTESIAN_POINT('Ctrl Pts',(40.4050927052958,42.7966439998082,46.7325871523312));
#28723=CARTESIAN_POINT('Ctrl Pts',(40.4474034358743,42.7924146396729,46.6659900800113));
#28724=CARTESIAN_POINT('Ctrl Pts',(40.4931165820223,42.7881852795377,46.601413480092));
#28725=CARTESIAN_POINT('Ctrl Pts',(40.5420108170025,42.7839559194024,46.5392239607783));
#28726=CARTESIAN_POINT('Ctrl Pts',(40.5908479536534,42.7797314982829,46.4771070659295));
#28727=CARTESIAN_POINT('Ctrl Pts',(40.6428585084515,42.7755070771634,46.4173720792295));
#28728=CARTESIAN_POINT('Ctrl Pts',(40.697777968431,42.771282656044,46.3603565643284));
#28729=CARTESIAN_POINT('Ctrl Pts',(40.7526623084538,42.7670609363619,46.3033775097715));
#28730=CARTESIAN_POINT('Ctrl Pts',(40.8104515368487,42.7628392166799,46.2491148124934));
#28731=CARTESIAN_POINT('Ctrl Pts',(40.8708417858123,42.7586174969979,46.1978719255052));
#28732=CARTESIAN_POINT('Ctrl Pts',(40.9312122753554,42.7543971586437,46.1466458049614));
#28733=CARTESIAN_POINT('Ctrl Pts',(40.9941817379733,42.7501768202896,46.0984378361704));
#28734=CARTESIAN_POINT('Ctrl Pts',(41.0594115816624,42.7459564819354,46.0535126166555));
#28735=CARTESIAN_POINT('Ctrl Pts',(41.1246404523477,42.7417362065341,46.0085880672698));
#28736=CARTESIAN_POINT('Ctrl Pts',(41.1921292497807,42.7375159311329,45.966946434947));
#28737=CARTESIAN_POINT('Ctrl Pts',(41.2615098689342,42.7332956557316,45.9288093611727));
#28738=CARTESIAN_POINT('Ctrl Pts',(41.3309598848699,42.7290711590718,45.8906341414402));
#28739=CARTESIAN_POINT('Ctrl Pts',(41.4023050902673,42.7248466624119,45.8559707093128));
#28740=CARTESIAN_POINT('Ctrl Pts',(41.4751527346609,42.7206221657521,45.8249947180076));
#28741=CARTESIAN_POINT('Ctrl Pts',(41.548035353018,42.7163956409224,45.79400385521));
#28742=CARTESIAN_POINT('Ctrl Pts',(41.6224214061022,42.7121691160928,45.7667041218784));
#28743=CARTESIAN_POINT('Ctrl Pts',(41.6979005394215,42.7079425912632,45.7432220338821));
#28744=CARTESIAN_POINT('Ctrl Pts',(41.7735176460661,42.7037083404878,45.7196970214162));
#28745=CARTESIAN_POINT('Ctrl Pts',(41.85023136984,42.6994740897125,45.7000037160322));
#28746=CARTESIAN_POINT('Ctrl Pts',(41.9276188479409,42.6952398389372,45.6842179532436));
#28747=CARTESIAN_POINT('Ctrl Pts',(42.0014261238054,42.6912014786918,45.6691624923672));
#28748=CARTESIAN_POINT('Ctrl Pts',(42.0758458337977,42.6871631184464,45.6576610360458));
#28749=CARTESIAN_POINT('Ctrl Pts',(42.1505083191468,42.683124758201,45.6497352612769));
#28750=CARTESIAN_POINT('Ctrl Pts',(42.2288155917424,42.6788892579347,45.6414225751608));
#28751=CARTESIAN_POINT('Ctrl Pts',(42.3076876106676,42.6746537576685,45.6370119931367));
#28752=CARTESIAN_POINT('Ctrl Pts',(42.3867019084308,42.6704182574022,45.6365674112299));
#28753=CARTESIAN_POINT('Ctrl Pts',(42.4656016605423,42.666188897267,45.6361234738257));
#28754=CARTESIAN_POINT('Ctrl Pts',(42.5446428165234,42.6619595371317,45.6396341217822));
#28755=CARTESIAN_POINT('Ctrl Pts',(42.6233973127031,42.6577301769965,45.6471115450203));
#28756=CARTESIAN_POINT('Ctrl Pts',(42.7020598399593,42.653505755877,45.6545802361783));
#28757=CARTESIAN_POINT('Ctrl Pts',(42.78043590782,42.6492813347575,45.6660064531012));
#28758=CARTESIAN_POINT('Ctrl Pts',(42.8580985165179,42.645056913638,45.681350352023));
#28759=CARTESIAN_POINT('Ctrl Pts',(42.9357114614455,42.640835193956,45.6966844388113));
#28760=CARTESIAN_POINT('Ctrl Pts',(43.0126113935494,42.636613474274,45.7159311444201));
#28761=CARTESIAN_POINT('Ctrl Pts',(43.0883787104353,42.6323917545919,45.7389990729946));
#28762=CARTESIAN_POINT('Ctrl Pts',(43.1641212365924,42.6281714162378,45.7620594538455));
#28763=CARTESIAN_POINT('Ctrl Pts',(43.2387314347309,42.6239510778836,45.7889384384078));
#28764=CARTESIAN_POINT('Ctrl Pts',(43.3118035955149,42.6197307395295,45.8194944063117));
#28765=CARTESIAN_POINT('Ctrl Pts',(43.3848746663147,42.6155104641282,45.8500499184261));
#28766=CARTESIAN_POINT('Ctrl Pts',(43.4564073128616,42.6112901887269,45.8842821225544));
#28767=CARTESIAN_POINT('Ctrl Pts',(43.5260159867585,42.6070699133256,45.9220013381948));
#28768=CARTESIAN_POINT('Ctrl Pts',(43.5956942855454,42.6028454166658,45.9597582818379));
#28769=CARTESIAN_POINT('Ctrl Pts',(43.6634443537622,42.598620920006,46.0010089802159));
#28770=CARTESIAN_POINT('Ctrl Pts',(43.7289059874642,42.5943964233461,46.0455181460597));
#28771=CARTESIAN_POINT('Ctrl Pts',(43.7943990491254,42.5901698985165,46.0900486806377));
#28772=CARTESIAN_POINT('Ctrl Pts',(43.8576011127006,42.5859433736868,46.137840515644));
#28773=CARTESIAN_POINT('Ctrl Pts',(43.9181837765053,42.5817168488572,46.1886169754423));
#28774=CARTESIAN_POINT('Ctrl Pts',(43.9788771833885,42.5774825980819,46.2394862529068));
#28775=CARTESIAN_POINT('Ctrl Pts',(44.036941277607,42.5732483473065,46.2933507370757));
#28776=CARTESIAN_POINT('Ctrl Pts',(44.0920835141889,42.5690140965312,46.3498958148316));
#28777=CARTESIAN_POINT('Ctrl Pts',(44.144674687425,42.5649757362859,46.4038249291412));
#28778=CARTESIAN_POINT('Ctrl Pts',(44.194608164733,42.5609373760405,46.4601918039581));
#28779=CARTESIAN_POINT('Ctrl Pts',(44.2416657329005,42.5568990157952,46.5186972729519));
#28780=CARTESIAN_POINT('Ctrl Pts',(44.2910205032515,42.5526635155289,46.5800587945713));
#28781=CARTESIAN_POINT('Ctrl Pts',(44.3373990175007,42.5484280152627,46.6440062888083));
#28782=CARTESIAN_POINT('Ctrl Pts',(44.3805189859801,42.5441925149964,46.710219015851));
#28783=CARTESIAN_POINT('Ctrl Pts',(44.423576444192,42.5399631548612,46.7763357554562));
#28784=CARTESIAN_POINT('Ctrl Pts',(44.4633844834144,42.5357337947259,46.844710816708));
#28785=CARTESIAN_POINT('Ctrl Pts',(44.4997012727788,42.5315044345906,46.9149907806884));
#28786=CARTESIAN_POINT('Ctrl Pts',(44.5359756516626,42.5272800134711,46.9851886722418));
#28787=CARTESIAN_POINT('Ctrl Pts',(44.5687666682094,42.5230555923516,47.057286631161));
#28788=CARTESIAN_POINT('Ctrl Pts',(44.5978768289048,42.5188311712321,47.1309039835189));
#28789=CARTESIAN_POINT('Ctrl Pts',(44.6269683742027,42.5146094515501,47.2044742589714));
#28790=CARTESIAN_POINT('Ctrl Pts',(44.65238356339,42.5103877318681,47.27956156411));
#28791=CARTESIAN_POINT('Ctrl Pts',(44.6739722616212,42.506166012186,47.3557635571646));
#28792=CARTESIAN_POINT('Ctrl Pts',(44.6955538961266,42.5019456738319,47.4319406172664));
#28793=CARTESIAN_POINT('Ctrl Pts',(44.7133113979149,42.4977253354777,47.5092311898326));
#28794=CARTESIAN_POINT('Ctrl Pts',(44.7271443883942,42.4935049971236,47.5872174465103));
#28795=CARTESIAN_POINT('Ctrl Pts',(44.740977172533,42.4892847217223,47.6652025399025));
#28796=CARTESIAN_POINT('Ctrl Pts',(44.7508854810686,42.485064446321,47.7438828344079));
#28797=CARTESIAN_POINT('Ctrl Pts',(44.7568202622255,42.4808441709197,47.8228314574665));
#28798=CARTESIAN_POINT('Ctrl Pts',(44.7627609795461,42.4766196742598,47.9018590475401));
#28799=CARTESIAN_POINT('Ctrl Pts',(44.7647201947495,42.4723951776,47.9811550331627));
#28800=CARTESIAN_POINT('Ctrl Pts',(44.7627009237643,42.4681706809401,48.060289184297));
#28801=CARTESIAN_POINT('Ctrl Pts',(44.7606806833325,42.4639441561105,48.1394613275303));
#28802=CARTESIAN_POINT('Ctrl Pts',(44.7546781872409,42.4597176312808,48.2184710128488));
#28803=CARTESIAN_POINT('Ctrl Pts',(44.7447484649486,42.4554911064512,48.296892366054));
#28804=CARTESIAN_POINT('Ctrl Pts',(44.7348005914569,42.4512568556758,48.3754570708638));
#28805=CARTESIAN_POINT('Ctrl Pts',(44.7209112292878,42.4470226049005,48.4534308312628));
#28806=CARTESIAN_POINT('Ctrl Pts',(44.703186712563,42.4427883541251,48.5303974056998));
#28807=CARTESIAN_POINT('Ctrl Pts',(44.6862821909592,42.4387499938799,48.603803250302));
#28808=CARTESIAN_POINT('Ctrl Pts',(44.6658896534714,42.4347116336346,48.6762927057238));
#28809=CARTESIAN_POINT('Ctrl Pts',(44.6421426558893,42.4306732733893,48.7475204020907));
#28810=CARTESIAN_POINT('Ctrl Pts',(44.6172364047199,42.426437773123,48.8222252101321));
#28811=CARTESIAN_POINT('Ctrl Pts',(44.5885451487791,42.4222022728568,48.8958258924366));
#28812=CARTESIAN_POINT('Ctrl Pts',(44.5561859229428,42.4179667725905,48.9679115179619));
#28813=CARTESIAN_POINT('Ctrl Pts',(44.5238736077129,42.4137374124553,49.039892642211));
#28814=CARTESIAN_POINT('Ctrl Pts',(44.4879040725767,42.40950805232,49.1103626466809));
#28815=CARTESIAN_POINT('Ctrl Pts',(44.4484437243221,42.4052786921848,49.1789269481972));
#28816=CARTESIAN_POINT('Ctrl Pts',(44.4090294575729,42.4010542710653,49.2474111808247));
#28817=CARTESIAN_POINT('Ctrl Pts',(44.3661327114626,42.3968298499458,49.3139937282349));
#28818=CARTESIAN_POINT('Ctrl Pts',(44.3199668011377,42.3926054288263,49.3783025514846));
#28819=CARTESIAN_POINT('Ctrl Pts',(44.2738304130399,42.3883837091443,49.4425702504574));
#28820=CARTESIAN_POINT('Ctrl Pts',(44.2244292830312,42.3841619894622,49.5045667309079));
#28821=CARTESIAN_POINT('Ctrl Pts',(44.172020570159,42.3799402697802,49.5639480617441));
#28822=CARTESIAN_POINT('Ctrl Pts',(44.1196290051843,42.3757199314261,49.6233099632733));
#28823=CARTESIAN_POINT('Ctrl Pts',(44.0642321217211,42.3714995930719,49.680058062624));
#28824=CARTESIAN_POINT('Ctrl Pts',(44.006127021177,42.3672792547178,49.7338818970003));
#28825=CARTESIAN_POINT('Ctrl Pts',(43.9480227873603,42.3630589793165,49.7877049285108));
#28826=CARTESIAN_POINT('Ctrl Pts',(43.8872107619944,42.3588387039152,49.8386034637785));
#28827=CARTESIAN_POINT('Ctrl Pts',(43.8240234202902,42.3546184285139,49.8863053144613));
#28828=CARTESIAN_POINT('Ctrl Pts',(43.7607728765241,42.3503939318541,49.9340548781075));
#28829=CARTESIAN_POINT('Ctrl Pts',(43.6951426458085,42.3461694351942,49.9786010864343));
#28830=CARTESIAN_POINT('Ctrl Pts',(43.6274961952718,42.3419449385344,50.0197137251337));
#28831=CARTESIAN_POINT('Ctrl Pts',(43.5598172678509,42.3377184137047,50.0608461019034));
#28832=CARTESIAN_POINT('Ctrl Pts',(43.4901206056763,42.3334918888751,50.0985414015462));
#28833=CARTESIAN_POINT('Ctrl Pts',(43.4187941513704,42.3292653640454,50.1326155110646));
#28834=CARTESIAN_POINT('Ctrl Pts',(43.3473373146972,42.3250311132701,50.166751906913));
#28835=CARTESIAN_POINT('Ctrl Pts',(43.2742451670299,42.3207968624948,50.1972537042632));
#28836=CARTESIAN_POINT('Ctrl Pts',(43.1999253050504,42.3165626117194,50.2239851499594));
#28837=CARTESIAN_POINT('Ctrl Pts',(43.1290437271798,42.3125242514741,50.2494799100308));
#28838=CARTESIAN_POINT('Ctrl Pts',(43.0570458714223,42.3084858912288,50.2715453921));
#28839=CARTESIAN_POINT('Ctrl Pts',(42.9842944560811,42.3044475309835,50.2901070781719));
#28840=CARTESIAN_POINT('Ctrl Pts',(42.9079915459072,42.3002120307172,50.3095748872636));
#28841=CARTESIAN_POINT('Ctrl Pts',(42.8305695810991,42.295976530451,50.3252620784841));
#28842=CARTESIAN_POINT('Ctrl Pts',(42.7524374810683,42.2917410301847,50.3370447712524));
#28843=CARTESIAN_POINT('Ctrl Pts',(42.6744186477825,42.2875116700495,50.3488103828562));
#28844=CARTESIAN_POINT('Ctrl Pts',(42.5956921837992,42.2832823099142,50.3566826669339));
#28845=CARTESIAN_POINT('Ctrl Pts',(42.5166799692987,42.2790529497789,50.3605881101252));
#28846=CARTESIAN_POINT('Ctrl Pts',(42.4377600246832,42.2748285286594,50.3644889925686));
#28847=CARTESIAN_POINT('Ctrl Pts',(42.3585554590132,42.27060410754,50.3644322166106));
#28848=CARTESIAN_POINT('Ctrl Pts',(42.2794945691606,42.2663796864205,50.3603959163747));
#28849=CARTESIAN_POINT('Ctrl Pts',(42.2004842372526,42.2621579667384,50.3563621972764));
#28850=CARTESIAN_POINT('Ctrl Pts',(42.1216178662786,42.2579362470564,50.3483540287107));
#28851=CARTESIAN_POINT('Ctrl Pts',(42.0433238327958,42.2537145273744,50.33640162486));
#28852=CARTESIAN_POINT('Ctrl Pts',(41.9650554167722,42.2494941890202,50.3244531317827));
#28853=CARTESIAN_POINT('Ctrl Pts',(41.8873594300161,42.245273850666,50.3085630367748));
#28854=CARTESIAN_POINT('Ctrl Pts',(41.8106577097856,42.2410535123119,50.2888132527283));
#28855=CARTESIAN_POINT('Ctrl Pts',(41.7339571336798,42.2368332369106,50.2690637632804));
#28856=CARTESIAN_POINT('Ctrl Pts',(41.6582512488118,42.2326129615093,50.2454548175639));
#28857=CARTESIAN_POINT('Ctrl Pts',(41.583948839476,42.228392686108,50.2181187849859));
#28858=CARTESIAN_POINT('Ctrl Pts',(41.5095721104213,42.2241681894482,50.1907554100071));
#28859=CARTESIAN_POINT('Ctrl Pts',(41.4366021027103,42.2199436927883,50.1596576635497));
#28860=CARTESIAN_POINT('Ctrl Pts',(41.3654290656604,42.2157191961285,50.1250066876882));
#28861=CARTESIAN_POINT('Ctrl Pts',(41.2942218586215,42.2114926712988,50.0903390759839));
#28862=CARTESIAN_POINT('Ctrl Pts',(41.2248137525836,42.2072661464692,50.0521150632474));
#28863=CARTESIAN_POINT('Ctrl Pts',(41.157569465402,42.2030396216395,50.0105613165478));
#28864=CARTESIAN_POINT('Ctrl Pts',(41.0902022579178,42.1988053708642,49.9689316109924));
#28865=CARTESIAN_POINT('Ctrl Pts',(41.0250071604507,42.1945711200888,49.9239602761392));
#28866=CARTESIAN_POINT('Ctrl Pts',(40.9623188515509,42.1903368693135,49.8759166709356));
#28867=CARTESIAN_POINT('Ctrl Pts',(40.9025307124117,42.1862985090682,49.8300957227703));
#28868=CARTESIAN_POINT('Ctrl Pts',(40.8450227954835,42.1822601488229,49.7814807433587));
#28869=CARTESIAN_POINT('Ctrl Pts',(40.7900540000068,42.1782217885776,49.7303364753729));
#28870=CARTESIAN_POINT('Ctrl Pts',(40.7312006102975,42.173898041127,49.6755778889956));
#28871=CARTESIAN_POINT('Ctrl Pts',(40.675011657768,42.1695742936764,49.617689584426));
#28872=CARTESIAN_POINT('Ctrl Pts',(40.6218435444555,42.1652505462258,49.5569682271985));
#28873=CARTESIAN_POINT('Ctrl Pts',(40.5706245486074,42.1610853052774,49.4984728857247));
#28874=CARTESIAN_POINT('Ctrl Pts',(40.5222091535806,42.156920064329,49.4373489697679));
#28875=CARTESIAN_POINT('Ctrl Pts',(40.4768817937906,42.1527548233806,49.3739020364808));
#28876=CARTESIAN_POINT('Ctrl Pts',(40.4315970956775,42.148593502717,49.3105148188396));
#28877=CARTESIAN_POINT('Ctrl Pts',(40.3893949493629,42.1444321820535,49.2448093115539));
#28878=CARTESIAN_POINT('Ctrl Pts',(40.3505201270085,42.1402708613899,49.1771247559638));
#28879=CARTESIAN_POINT('Ctrl Pts',(40.3116689089882,42.1361120674313,49.1094812976384));
#28880=CARTESIAN_POINT('Ctrl Pts',(40.2761412472426,42.1319532734726,49.0398615943417));
#28881=CARTESIAN_POINT('Ctrl Pts',(40.244138143138,42.127794479514,48.9686331065101));
#28882=CARTESIAN_POINT('Ctrl Pts',(40.2121437854714,42.1236368221524,48.8974240854012));
#28883=CARTESIAN_POINT('Ctrl Pts',(40.1836722700636,42.1194791647908,48.8246075950335));
#28884=CARTESIAN_POINT('Ctrl Pts',(40.1588774918835,42.1153215074292,48.7505733438604));
#28885=CARTESIAN_POINT('Ctrl Pts',(40.134070501267,42.1111618022522,48.6765026278083));
#28886=CARTESIAN_POINT('Ctrl Pts',(40.1129440199525,42.1070020970753,48.6012134126361));
#28887=CARTESIAN_POINT('Ctrl Pts',(40.095602460452,42.1028423918984,48.5251118172591));
#28888=CARTESIAN_POINT('Ctrl Pts',(40.0782556616417,42.0986814299727,48.4489872297263));
#28889=CARTESIAN_POINT('Ctrl Pts',(40.0646961483959,42.094520468047,48.3720502501643));
#28890=CARTESIAN_POINT('Ctrl Pts',(40.054977006387,42.0903595061213,48.2947161351649));
#28891=CARTESIAN_POINT('Ctrl Pts',(40.0452468055504,42.086193809687,48.2172940263222));
#28892=CARTESIAN_POINT('Ctrl Pts',(40.0393657308817,42.0820281132527,48.1394743631729));
#28893=CARTESIAN_POINT('Ctrl Pts',(40.0373348542212,42.0778624168184,48.0616753583057));
#28894=CARTESIAN_POINT('Ctrl Pts',(40.0367806098798,42.0767255611335,48.0404433164714));
#28895=CARTESIAN_POINT('Ctrl Pts',(40.0365128260987,42.0755887054486,48.0192127986881));
#28896=CARTESIAN_POINT('Ctrl Pts',(40.0365308527828,42.0744518497637,47.9979922519359));
#28897=CARTESIAN_POINT('',(40.0365304529153,41.2807018496994,48.001463182638));
#28898=CARTESIAN_POINT('Ctrl Pts',(40.0365308527833,42.0744518497283,47.997992251275));
#28899=CARTESIAN_POINT('Ctrl Pts',(40.0366334841975,42.067979385482,47.8771772419789));
#28900=CARTESIAN_POINT('Ctrl Pts',(40.0460029002097,42.0615069212358,47.7567426871142));
#28901=CARTESIAN_POINT('Ctrl Pts',(40.0644473300431,42.0550344569895,47.6378064512486));
#28902=CARTESIAN_POINT('Ctrl Pts',(40.0673334927678,42.0540216533836,47.6191954487035));
#28903=CARTESIAN_POINT('Ctrl Pts',(40.0704417825611,42.0530088497776,47.600621068999));
#28904=CARTESIAN_POINT('Ctrl Pts',(40.0737713756649,42.0519960461717,47.5820875352133));
#28905=CARTESIAN_POINT('Ctrl Pts',(40.0876955880151,42.0477605459054,47.5045811096588));
#28906=CARTESIAN_POINT('Ctrl Pts',(40.1055241028375,42.0435250456392,47.4276240264088));
#28907=CARTESIAN_POINT('Ctrl Pts',(40.1272000876839,42.0392895453729,47.351639761031));
#28908=CARTESIAN_POINT('Ctrl Pts',(40.1488446492325,42.0350601852377,47.2757656487196));
#28909=CARTESIAN_POINT('Ctrl Pts',(40.17432547699,42.0308308251024,47.2008620012471));
#28910=CARTESIAN_POINT('Ctrl Pts',(40.2035345311768,42.0266014649672,47.1273432031048));
#28911=CARTESIAN_POINT('Ctrl Pts',(40.2327094752443,42.0223770438477,47.0539102596762));
#28912=CARTESIAN_POINT('Ctrl Pts',(40.2656038215422,42.0181526227282,46.9818593857877));
#28913=CARTESIAN_POINT('Ctrl Pts',(40.3020598714922,42.0139282016087,46.9115893890187));
#28914=CARTESIAN_POINT('Ctrl Pts',(40.3384926084873,42.0097064819267,46.8413643285845));
#28915=CARTESIAN_POINT('Ctrl Pts',(40.3784823129429,42.0054847622447,46.7729183004168));
#28916=CARTESIAN_POINT('Ctrl Pts',(40.4218238615273,42.0012630425626,46.7066285892764));
#28917=CARTESIAN_POINT('Ctrl Pts',(40.4651512289501,41.9970427042085,46.6403605678342));
#28918=CARTESIAN_POINT('Ctrl Pts',(40.5118280061515,41.9928223658544,46.5762478549964));
#28919=CARTESIAN_POINT('Ctrl Pts',(40.5616047366716,41.9886020275002,46.5146403477031));
#28920=CARTESIAN_POINT('Ctrl Pts',(40.6113807246949,41.9843817520989,46.4530337593808));
#28921=CARTESIAN_POINT('Ctrl Pts',(40.6642562781117,41.9801614766977,46.3939326665623));
#28922=CARTESIAN_POINT('Ctrl Pts',(40.7199414386359,41.9759412012964,46.3376541661594));
#28923=CARTESIAN_POINT('Ctrl Pts',(40.775682297293,41.9717167046366,46.2813193741454));
#28924=CARTESIAN_POINT('Ctrl Pts',(40.8342380460026,41.9674922079767,46.2278131487776));
#28925=CARTESIAN_POINT('Ctrl Pts',(40.8952820300687,41.9632677113169,46.1774154966461));
#28926=CARTESIAN_POINT('Ctrl Pts',(40.9563553211919,41.9590411864873,46.1269936487335));
#28927=CARTESIAN_POINT('Ctrl Pts',(41.0199188504245,41.9548146616576,46.0796836277557));
#28928=CARTESIAN_POINT('Ctrl Pts',(41.0856151231092,41.950588136828,46.0357233300014));
#28929=CARTESIAN_POINT('Ctrl Pts',(41.1514314863779,41.9463538860527,45.9916826742967));
#28930=CARTESIAN_POINT('Ctrl Pts',(41.2193879796092,41.9421196352774,45.9510042190667));
#28931=CARTESIAN_POINT('Ctrl Pts',(41.2891007154644,41.937885384502,45.9138808230309));
#28932=CARTESIAN_POINT('Ctrl Pts',(41.3555883081961,41.9338470242567,45.8784748788205));
#28933=CARTESIAN_POINT('Ctrl Pts',(41.4236728992671,41.9298086640113,45.8463024497626));
#28934=CARTESIAN_POINT('Ctrl Pts',(41.4930062244249,41.9257703037659,45.8174893512361));
#28935=CARTESIAN_POINT('Ctrl Pts',(41.5657241840231,41.9215348034997,45.7872696880397));
#28936=CARTESIAN_POINT('Ctrl Pts',(41.640092325734,41.9172993032334,45.7606308423139));
#28937=CARTESIAN_POINT('Ctrl Pts',(41.715723748849,41.9130638029672,45.7377541130526));
#28938=CARTESIAN_POINT('Ctrl Pts',(41.7912455304067,41.9088344428319,45.7149105477873));
#28939=CARTESIAN_POINT('Ctrl Pts',(41.868026511167,41.9046050826967,45.6958184032925));
#28940=CARTESIAN_POINT('Ctrl Pts',(41.945659733541,41.9003757225614,45.6806109935645));
#28941=CARTESIAN_POINT('Ctrl Pts',(42.0232022964068,41.8961513014419,45.6654213429381));
#28942=CARTESIAN_POINT('Ctrl Pts',(42.1015946649512,41.8919268803224,45.6541075018368));
#28943=CARTESIAN_POINT('Ctrl Pts',(42.1804161172182,41.8877024592029,45.6467525928364));
#28944=CARTESIAN_POINT('Ctrl Pts',(42.2591871646564,41.8834807395209,45.6394023871612));
#28945=CARTESIAN_POINT('Ctrl Pts',(42.3383862851507,41.8792590198389,45.636006132267));
#28946=CARTESIAN_POINT('Ctrl Pts',(42.417585201652,41.8750373001569,45.6365954215195));
#28947=CARTESIAN_POINT('Ctrl Pts',(42.4967582046205,41.8708169618027,45.6371845179591));
#28948=CARTESIAN_POINT('Ctrl Pts',(42.5759305347451,41.8665966234485,45.6417565656403));
#28949=CARTESIAN_POINT('Ctrl Pts',(42.654672965057,41.8623762850944,45.6502910559456));
#28950=CARTESIAN_POINT('Ctrl Pts',(42.7334142208038,41.8581560096931,45.6588254189458));
#28951=CARTESIAN_POINT('Ctrl Pts',(42.8117251230099,41.8539357342918,45.6713220551797));
#28952=CARTESIAN_POINT('Ctrl Pts',(42.8891821193075,41.8497154588905,45.6877086483209));
#28953=CARTESIAN_POINT('Ctrl Pts',(42.9667165906458,41.8454909622307,45.7041116318728));
#28954=CARTESIAN_POINT('Ctrl Pts',(43.0433949896083,41.8412664655708,45.7244122474451));
#28955=CARTESIAN_POINT('Ctrl Pts',(43.1188051053835,41.837041968911,45.7484872504526));
#28956=CARTESIAN_POINT('Ctrl Pts',(43.1942514253581,41.8328154440813,45.7725738118061));
#28957=CARTESIAN_POINT('Ctrl Pts',(43.2684278091661,41.8285889192517,45.8004382051894));
#28958=CARTESIAN_POINT('Ctrl Pts',(43.3409407777844,41.824362394422,45.8319084674298));
#28959=CARTESIAN_POINT('Ctrl Pts',(43.4135862976784,41.8201281436467,45.8634362562546));
#28960=CARTESIAN_POINT('Ctrl Pts',(43.4845619047036,41.8158938928714,45.8985828762858));
#28961=CARTESIAN_POINT('Ctrl Pts',(43.5534977194812,41.811659642096,45.9371298024229));
#28962=CARTESIAN_POINT('Ctrl Pts',(43.6192443340884,41.8076212818507,45.973893419495));
#28963=CARTESIAN_POINT('Ctrl Pts',(43.683135434209,41.8035829216054,46.0137494611703));
#28964=CARTESIAN_POINT('Ctrl Pts',(43.7448767975816,41.7995445613601,46.0564730924871));
#28965=CARTESIAN_POINT('Ctrl Pts',(43.809632179746,41.7953090610938,46.1012823568481));
#28966=CARTESIAN_POINT('Ctrl Pts',(43.8722687283955,41.7910735608276,46.1494166624567));
#28967=CARTESIAN_POINT('Ctrl Pts',(43.9324246559972,41.7868380605613,46.2006486961708));
#28968=CARTESIAN_POINT('Ctrl Pts',(43.9924933765981,41.782608700426,46.2518064596976));
#28969=CARTESIAN_POINT('Ctrl Pts',(44.0500882630937,41.7783793402908,46.3060527318044));
#28970=CARTESIAN_POINT('Ctrl Pts',(44.1048770340794,41.7741499801555,46.3631173714745));
#28971=CARTESIAN_POINT('Ctrl Pts',(44.1596018231399,41.769925559036,46.4201153714766));
#28972=CARTESIAN_POINT('Ctrl Pts',(44.2115266852493,41.7657011379165,46.4799248618724));
#28973=CARTESIAN_POINT('Ctrl Pts',(44.2603541049907,41.761476716797,46.5422369722948));
#28974=CARTESIAN_POINT('Ctrl Pts',(44.3091503005201,41.757254997115,46.6045092353004));
#28975=CARTESIAN_POINT('Ctrl Pts',(44.3548526963495,41.7530332774329,46.6692805734822));
#28976=CARTESIAN_POINT('Ctrl Pts',(44.3972030273329,41.7488115577509,46.7362078855633));
#28977=CARTESIAN_POINT('Ctrl Pts',(44.4395395014766,41.7445912193968,46.803113299326));
#28978=CARTESIAN_POINT('Ctrl Pts',(44.4785258378359,41.7403708810426,46.8721728899318));
#28979=CARTESIAN_POINT('Ctrl Pts',(44.5139470765968,41.7361505426884,46.9430145704656));
#28980=CARTESIAN_POINT('Ctrl Pts',(44.5493677869951,41.7319302672871,47.0138551942863));
#28981=CARTESIAN_POINT('Ctrl Pts',(44.581223296794,41.7277099918859,47.086477434798));
#28982=CARTESIAN_POINT('Ctrl Pts',(44.6093452878274,41.7234897164846,47.160485950055));
#28983=CARTESIAN_POINT('Ctrl Pts',(44.6374954074031,41.7192652198247,47.2345684910684));
#28984=CARTESIAN_POINT('Ctrl Pts',(44.6619043811873,41.7150407231649,47.310039636938));
#28985=CARTESIAN_POINT('Ctrl Pts',(44.6824528587946,41.710816226505,47.3864860325305));
#28986=CARTESIAN_POINT('Ctrl Pts',(44.7030112016723,41.7065897016754,47.4629691298375));
#28987=CARTESIAN_POINT('Ctrl Pts',(44.7197052571245,41.7023631768457,47.5404279501617));
#28988=CARTESIAN_POINT('Ctrl Pts',(44.7324667822032,41.6981366520161,47.6184385359883));
#28989=CARTESIAN_POINT('Ctrl Pts',(44.7452516349219,41.6939024012407,47.6965917225504));
#28990=CARTESIAN_POINT('Ctrl Pts',(44.7540895403785,41.6896681504654,47.775298222405));
#28991=CARTESIAN_POINT('Ctrl Pts',(44.7589641827196,41.6854338996901,47.8541287363938));
#28992=CARTESIAN_POINT('Ctrl Pts',(44.763613307886,41.6813955394448,47.929312288502));
#28993=CARTESIAN_POINT('Ctrl Pts',(44.7646577996222,41.6773571791995,48.0046082762408));
#28994=CARTESIAN_POINT('Ctrl Pts',(44.7621275787021,41.6733188189542,48.0796476166296));
#28995=CARTESIAN_POINT('Ctrl Pts',(44.7594738403704,41.669083318688,48.1583501411424));
#28996=CARTESIAN_POINT('Ctrl Pts',(44.7528773781285,41.6648478184217,48.2370694862173));
#28997=CARTESIAN_POINT('Ctrl Pts',(44.7423336447328,41.6606123181555,48.3153784039098));
#28998=CARTESIAN_POINT('Ctrl Pts',(44.7318051964039,41.6563829580202,48.3935737985277));
#28999=CARTESIAN_POINT('Ctrl Pts',(44.717340902479,41.652153597885,48.4713594860876));
#29000=CARTESIAN_POINT('Ctrl Pts',(44.6989881977231,41.6479242377497,48.5483098646112));
#29001=CARTESIAN_POINT('Ctrl Pts',(44.6806569251213,41.6436998166302,48.6251703810468));
#29002=CARTESIAN_POINT('Ctrl Pts',(44.6584463735388,41.6394753955107,48.7011970727075));
#29003=CARTESIAN_POINT('Ctrl Pts',(44.6324553583148,41.6352509743912,48.7759726245376));
#29004=CARTESIAN_POINT('Ctrl Pts',(44.6064809638537,41.6310292547092,48.8507003588158));
#29005=CARTESIAN_POINT('Ctrl Pts',(44.5767310577221,41.6268075350272,48.9241780991155));
#29006=CARTESIAN_POINT('Ctrl Pts',(44.5433544784777,41.6225858153452,48.9960030223297));
#29007=CARTESIAN_POINT('Ctrl Pts',(44.5099888199012,41.618365476991,49.0678044447489));
#29008=CARTESIAN_POINT('Ctrl Pts',(44.4729990421105,41.6141451386369,49.1379536986034));
#29009=CARTESIAN_POINT('Ctrl Pts',(44.4325817892143,41.6099248002827,49.206068700802));
#29010=CARTESIAN_POINT('Ctrl Pts',(44.392165139204,41.6057045248814,49.2741826869601));
#29011=CARTESIAN_POINT('Ctrl Pts',(44.3483213563709,41.6014842494801,49.3402620788186));
#29012=CARTESIAN_POINT('Ctrl Pts',(44.3012918756923,41.5972639740789,49.4039514394474));
#29013=CARTESIAN_POINT('Ctrl Pts',(44.254215354577,41.593039477419,49.467704504274));
#29014=CARTESIAN_POINT('Ctrl Pts',(44.2039470497711,41.5888149807592,49.5290623838984));
#29015=CARTESIAN_POINT('Ctrl Pts',(44.1507700370006,41.5845904840993,49.5877010796875));
#29016=CARTESIAN_POINT('Ctrl Pts',(44.0975674940853,41.5803639592697,49.6463679277611));
#29017=CARTESIAN_POINT('Ctrl Pts',(44.0414537941184,41.57613743444,49.7023126595011));
#29018=CARTESIAN_POINT('Ctrl Pts',(43.9827485784147,41.5719109096104,49.7552485232657));
#29019=CARTESIAN_POINT('Ctrl Pts',(43.9239360515447,41.5676766588351,49.8082811520146));
#29020=CARTESIAN_POINT('Ctrl Pts',(43.862522907789,41.5634424080597,49.8582936251212));
#29021=CARTESIAN_POINT('Ctrl Pts',(43.7988613730507,41.5592081572844,49.9050399733041));
#29022=CARTESIAN_POINT('Ctrl Pts',(43.7381450327382,41.5551697970391,49.9496236798754));
#29023=CARTESIAN_POINT('Ctrl Pts',(43.6753840548971,41.5511314367937,49.9912366152817));
#29024=CARTESIAN_POINT('Ctrl Pts',(43.610905035557,41.5470930765484,50.0297042729824));
#29025=CARTESIAN_POINT('Ctrl Pts',(43.5432783536882,41.5428575762821,50.0700498005072));
#29026=CARTESIAN_POINT('Ctrl Pts',(43.4735045451748,41.5386220760159,50.1070884863463));
#29027=CARTESIAN_POINT('Ctrl Pts',(43.4019404775094,41.5343865757496,50.1405853686383));
#29028=CARTESIAN_POINT('Ctrl Pts',(43.3304801550268,41.5301572156144,50.1740336910832));
#29029=CARTESIAN_POINT('Ctrl Pts',(43.2572351487088,41.5259278554791,50.2039502088852));
#29030=CARTESIAN_POINT('Ctrl Pts',(43.1825890635681,41.5216984953438,50.2301445689649));
#29031=CARTESIAN_POINT('Ctrl Pts',(43.1080301495786,41.5174740742243,50.2563083394629));
#29032=CARTESIAN_POINT('Ctrl Pts',(43.0320738487144,41.5132496531048,50.2787584353536));
#29033=CARTESIAN_POINT('Ctrl Pts',(42.9551245929073,41.5090252319853,50.2973521992175));
#29034=CARTESIAN_POINT('Ctrl Pts',(42.8782245446948,41.5048035123033,50.3159340727209));
#29035=CARTESIAN_POINT('Ctrl Pts',(42.8003332568198,41.5005817926213,50.3306643988401));
#29036=CARTESIAN_POINT('Ctrl Pts',(42.7218700352141,41.4963600729392,50.341450431107));
#29037=CARTESIAN_POINT('Ctrl Pts',(42.6434324864251,41.4921397345851,50.3522329342322));
#29038=CARTESIAN_POINT('Ctrl Pts',(42.5644238401186,41.4879193962309,50.3590736422496));
#29039=CARTESIAN_POINT('Ctrl Pts',(42.4852718216873,41.4836990578767,50.3619312346735));
#29040=CARTESIAN_POINT('Ctrl Pts',(42.4061209839307,41.4794787824755,50.3647887844719));
#29041=CARTESIAN_POINT('Ctrl Pts',(42.3268272473944,41.4752585070742,50.3636633211789));
#29042=CARTESIAN_POINT('Ctrl Pts',(42.2478201587803,41.4710382316729,50.3585656100322));
#29043=CARTESIAN_POINT('Ctrl Pts',(42.1687340446719,41.466813735013,50.3534627999867));
#29044=CARTESIAN_POINT('Ctrl Pts',(42.0899356207309,41.4625892383532,50.344379835466));
#29045=CARTESIAN_POINT('Ctrl Pts',(42.0118505204597,41.4583647416933,50.3313795105972));
#29046=CARTESIAN_POINT('Ctrl Pts',(41.933727931736,41.4541382168637,50.3183729443065));
#29047=CARTESIAN_POINT('Ctrl Pts',(41.8563198080603,41.449911692034,50.3014453714602));
#29048=CARTESIAN_POINT('Ctrl Pts',(41.7800402388424,41.4456851672044,50.2807104891777));
#29049=CARTESIAN_POINT('Ctrl Pts',(41.7036212331292,41.441450916429,50.2599377042256));
#29050=CARTESIAN_POINT('Ctrl Pts',(41.6283353514743,41.4372166656537,50.2353438489837));
#29051=CARTESIAN_POINT('Ctrl Pts',(41.5545800121627,41.4329824148784,50.2070920880347));
#29052=CARTESIAN_POINT('Ctrl Pts',(41.4842368402638,41.4289440546331,50.180147347553));
#29053=CARTESIAN_POINT('Ctrl Pts',(41.4152860387921,41.4249056943878,50.1498758476075));
#29054=CARTESIAN_POINT('Ctrl Pts',(41.3480510583184,41.4208673341425,50.1164578580721));
#29055=CARTESIAN_POINT('Ctrl Pts',(41.2775338779776,41.4166318338763,50.0814085075986));
#29056=CARTESIAN_POINT('Ctrl Pts',(41.2086362670648,41.41239633361,50.0427643901465));
#29057=CARTESIAN_POINT('Ctrl Pts',(41.1417488973762,41.4081608333438,50.0006985289258));
#29058=CARTESIAN_POINT('Ctrl Pts',(41.074958493143,41.4039314732085,49.9586936498518));
#29059=CARTESIAN_POINT('Ctrl Pts',(41.0101729369737,41.3997021130732,49.9132771253288));
#29060=CARTESIAN_POINT('Ctrl Pts',(40.9477598481979,41.395472752938,49.8646685985434));
#29061=CARTESIAN_POINT('Ctrl Pts',(40.8854196449697,41.3912483318185,49.8161168364393));
#29062=CARTESIAN_POINT('Ctrl Pts',(40.8254467719094,41.387023910699,49.7643807663975));
#29063=CARTESIAN_POINT('Ctrl Pts',(40.768180002144,41.3827994895795,49.7097233505738));
#29064=CARTESIAN_POINT('Ctrl Pts',(40.7109498533955,41.3785777698975,49.6551008871344));
#29065=CARTESIAN_POINT('Ctrl Pts',(40.656422711875,41.3743560502155,49.5975611089631));
#29066=CARTESIAN_POINT('Ctrl Pts',(40.604903420906,41.3701343305334,49.5374064890669));
#29067=CARTESIAN_POINT('Ctrl Pts',(40.5534009868196,41.3659139921793,49.4772715514945));
#29068=CARTESIAN_POINT('Ctrl Pts',(40.5049047541546,41.3616936538251,49.4145238272755));
#29069=CARTESIAN_POINT('Ctrl Pts',(40.4596808703964,41.357473315471,49.349500691439));
#29070=CARTESIAN_POINT('Ctrl Pts',(40.4144576612224,41.3532530400697,49.284478525523));
#29071=CARTESIAN_POINT('Ctrl Pts',(40.3725069708237,41.3490327646684,49.2171814015387));
#29072=CARTESIAN_POINT('Ctrl Pts',(40.3340521264432,41.3448124892671,49.14797640422));
#29073=CARTESIAN_POINT('Ctrl Pts',(40.2955588182598,41.3405879926073,49.078702185782));
#29074=CARTESIAN_POINT('Ctrl Pts',(40.260568569631,41.3363634959474,49.0075166931521));
#29075=CARTESIAN_POINT('Ctrl Pts',(40.2292588330358,41.3321389992876,48.9348118671405));
#29076=CARTESIAN_POINT('Ctrl Pts',(40.1979340647179,41.3279124744579,48.862072135732));
#29077=CARTESIAN_POINT('Ctrl Pts',(40.1702934924723,41.3236859496283,48.7878120583056));
#29078=CARTESIAN_POINT('Ctrl Pts',(40.146465512677,41.3194594247987,48.7124414048508));
#29079=CARTESIAN_POINT('Ctrl Pts',(40.1225939761335,41.3152251740233,48.6369329763684));
#29080=CARTESIAN_POINT('Ctrl Pts',(40.1025490774193,41.310990923248,48.5603103705151));
#29081=CARTESIAN_POINT('Ctrl Pts',(40.086408590451,41.3067566724726,48.4829960978735));
#29082=CARTESIAN_POINT('Ctrl Pts',(40.0710148161161,41.3027183122273,48.4092586407416));
#29083=CARTESIAN_POINT('Ctrl Pts',(40.0591722004117,41.298679951982,48.3348924576612));
#29084=CARTESIAN_POINT('Ctrl Pts',(40.0509041153203,41.2946415917366,48.260267104108));
#29085=CARTESIAN_POINT('Ctrl Pts',(40.0413907678166,41.2899950110672,48.1744023708484));
#29086=CARTESIAN_POINT('Ctrl Pts',(40.0365840304864,41.2853484303977,48.0880066583314));
#29087=CARTESIAN_POINT('Ctrl Pts',(40.0365304529157,41.2807018497283,48.0014631831762));
#29088=CARTESIAN_POINT('',(40.0365303286314,40.4869518497552,48.0012463629995));
#29089=CARTESIAN_POINT('Ctrl Pts',(40.0365304529153,41.2807018496994,48.001463182638));
#29090=CARTESIAN_POINT('Ctrl Pts',(40.0364822936043,41.2765251727226,47.9236717558034));
#29091=CARTESIAN_POINT('Ctrl Pts',(40.0402790029724,41.2723484957457,47.8457269396662));
#29092=CARTESIAN_POINT('Ctrl Pts',(40.0479396135873,41.2681718187689,47.7680466004383));
#29093=CARTESIAN_POINT('Ctrl Pts',(40.0555893910889,41.2640010481639,47.6904761114504));
#29094=CARTESIAN_POINT('Ctrl Pts',(40.0670921711881,41.2598302775589,47.6131698334982));
#29095=CARTESIAN_POINT('Ctrl Pts',(40.0824149681851,41.2556595069539,47.5365455133376));
#29096=CARTESIAN_POINT('Ctrl Pts',(40.0977257549111,41.2514920054705,47.4599812526333));
#29097=CARTESIAN_POINT('Ctrl Pts',(40.1168505270377,41.247324503987,47.3840983613117));
#29098=CARTESIAN_POINT('Ctrl Pts',(40.1397046532171,41.2431570025036,47.3093080381158));
#29099=CARTESIAN_POINT('Ctrl Pts',(40.1625484484906,41.2389913848841,47.2345515228978));
#29100=CARTESIAN_POINT('Ctrl Pts',(40.189118112592,41.2348257672647,47.1608870572169));
#29101=CARTESIAN_POINT('Ctrl Pts',(40.2192786277662,41.2306601496452,47.0887125933151));
#29102=CARTESIAN_POINT('Ctrl Pts',(40.2494355147339,41.2264950331353,47.0165468117537));
#29103=CARTESIAN_POINT('Ctrl Pts',(40.2831822079519,41.2223299166253,46.9458711212109));
#29104=CARTESIAN_POINT('Ctrl Pts',(40.3203354515176,41.2181648001154,46.877063756625));
#29105=CARTESIAN_POINT('Ctrl Pts',(40.3575222543888,41.2139959213924,46.8081942406048));
#29106=CARTESIAN_POINT('Ctrl Pts',(40.3981215253446,41.2098270426694,46.7411968482197));
#29107=CARTESIAN_POINT('Ctrl Pts',(40.4419042788426,41.2056581639465,46.6764246951212));
#29108=CARTESIAN_POINT('Ctrl Pts',(40.4857054624514,41.2014875303568,46.6116252765389));
#29109=CARTESIAN_POINT('Ctrl Pts',(40.5326925062317,41.197316896767,46.549053348847));
#29110=CARTESIAN_POINT('Ctrl Pts',(40.582594966076,41.1931462631773,46.489030316794));
#29111=CARTESIAN_POINT('Ctrl Pts',(40.6325876920064,41.1889680855353,46.4288987120534));
#29112=CARTESIAN_POINT('Ctrl Pts',(40.6855060416132,41.1847899078932,46.3713255699776));
#29113=CARTESIAN_POINT('Ctrl Pts',(40.7410416825391,41.1806117302511,46.3165963817827));
#29114=CARTESIAN_POINT('Ctrl Pts',(40.7950768881226,41.176546436611,46.2633458405765));
#29115=CARTESIAN_POINT('Ctrl Pts',(40.8515893741545,41.1724811429709,46.2127877225138));
#29116=CARTESIAN_POINT('Ctrl Pts',(40.9102671796561,41.1684158493309,46.1651467184294));
#29117=CARTESIAN_POINT('Ctrl Pts',(40.9714017206828,41.1641803490646,46.1155110700979));
#29118=CARTESIAN_POINT('Ctrl Pts',(41.0351358559068,41.1599448487984,46.0688397875959));
#29119=CARTESIAN_POINT('Ctrl Pts',(41.1011501434374,41.1557093485321,46.0254166284993));
#29120=CARTESIAN_POINT('Ctrl Pts',(41.1670687312047,41.1514799883969,45.9820564192004));
#29121=CARTESIAN_POINT('Ctrl Pts',(41.2352605183376,41.1472506282616,45.9419352383165));
#29122=CARTESIAN_POINT('Ctrl Pts',(41.3053731986432,41.1430212681263,45.9052965349121));
#29123=CARTESIAN_POINT('Ctrl Pts',(41.3754040018746,41.1387968470069,45.868700617917));
#29124=CARTESIAN_POINT('Ctrl Pts',(41.4473508267955,41.1345724258874,45.8355793131379));
#29125=CARTESIAN_POINT('Ctrl Pts',(41.5208339091645,41.1303480047679,45.8061318577396));
#29126=CARTESIAN_POINT('Ctrl Pts',(41.5942700004913,41.1261262850858,45.7767032334325));
#29127=CARTESIAN_POINT('Ctrl Pts',(41.6692399649032,41.1219045654038,45.7509439696526));
#29128=CARTESIAN_POINT('Ctrl Pts',(41.745342153362,41.1176828457218,45.7290060447603));
#29129=CARTESIAN_POINT('Ctrl Pts',(41.8214194415237,41.1134625073676,45.7070752978593));
#29130=CARTESIAN_POINT('Ctrl Pts',(41.8986277674785,41.1092421690135,45.6889635370223));
#29131=CARTESIAN_POINT('Ctrl Pts',(41.976549767592,41.1050218306593,45.6747730558989));
#29132=CARTESIAN_POINT('Ctrl Pts',(42.0544706053783,41.100801555258,45.6605827864486));
#29133=CARTESIAN_POINT('Ctrl Pts',(42.1331046341663,41.0965812798567,45.6503137632214));
#29134=CARTESIAN_POINT('Ctrl Pts',(42.2120252108304,41.0923610044555,45.6440169950663));
#29135=CARTESIAN_POINT('Ctrl Pts',(42.2910247264567,41.0881365077956,45.637713928676));
#29136=CARTESIAN_POINT('Ctrl Pts',(42.3703108935256,41.0839120111358,45.6353910917051));
#29137=CARTESIAN_POINT('Ctrl Pts',(42.4494534726929,41.0796875144759,45.6370474412425));
#29138=CARTESIAN_POINT('Ctrl Pts',(42.5286340480055,41.0754609896463,45.638704585989));
#29139=CARTESIAN_POINT('Ctrl Pts',(42.6076704292831,41.0712344648166,45.6443446895344));
#29140=CARTESIAN_POINT('Ctrl Pts',(42.6861364944463,41.067007939987,45.653914676009));
#29141=CARTESIAN_POINT('Ctrl Pts',(42.7647459929461,41.0627736892116,45.663502156098));
#29142=CARTESIAN_POINT('Ctrl Pts',(42.8427826284677,41.0585394384363,45.6770337934225));
#29143=CARTESIAN_POINT('Ctrl Pts',(42.9198296762005,41.054305187661,45.6944051638154));
#29144=CARTESIAN_POINT('Ctrl Pts',(42.9933122711371,41.0502668274156,45.7109728768119));
#29145=CARTESIAN_POINT('Ctrl Pts',(43.0658944821732,41.0462284671703,45.7310327714717));
#29146=CARTESIAN_POINT('Ctrl Pts',(43.1372303305945,41.042190106925,45.7544528772365));
#29147=CARTESIAN_POINT('Ctrl Pts',(43.212048570332,41.0379546066587,45.7790162787599));
#29148=CARTESIAN_POINT('Ctrl Pts',(43.285780053544,41.0337191063925,45.8073697086495));
#29149=CARTESIAN_POINT('Ctrl Pts',(43.3580133168007,41.0294836061262,45.8393980177431));
#29150=CARTESIAN_POINT('Ctrl Pts',(43.4301418647534,41.0252542459909,45.8713798959546));
#29151=CARTESIAN_POINT('Ctrl Pts',(43.5007760804111,41.0210248858557,45.9070258854392));
#29152=CARTESIAN_POINT('Ctrl Pts',(43.569520621626,41.0167955257204,45.9461713906726));
#29153=CARTESIAN_POINT('Ctrl Pts',(43.6381848834693,41.0125711046009,45.9852711820719));
#29154=CARTESIAN_POINT('Ctrl Pts',(43.7049634503462,41.0083466834814,46.0278621371252));
#29155=CARTESIAN_POINT('Ctrl Pts',(43.7694833089865,41.0041222623619,46.0737326490574));
#29156=CARTESIAN_POINT('Ctrl Pts',(43.8339619083968,40.9999005426799,46.1195738276643));
#29157=CARTESIAN_POINT('Ctrl Pts',(43.8961842849022,40.9956788229979,46.1686901294023));
#29158=CARTESIAN_POINT('Ctrl Pts',(43.955805331725,40.9914571033158,46.220825975157));
#29159=CARTESIAN_POINT('Ctrl Pts',(44.0154068708067,40.9872367649617,46.2729447622951));
#29160=CARTESIAN_POINT('Ctrl Pts',(44.0724084172434,40.9830164266075,46.3280808229195));
#29161=CARTESIAN_POINT('Ctrl Pts',(44.1264981490303,40.9787960882534,46.3859384824937));
#29162=CARTESIAN_POINT('Ctrl Pts',(44.1805870739854,40.9745758128521,46.4437952790316));
#29163=CARTESIAN_POINT('Ctrl Pts',(44.2317639510734,40.9703555374508,46.5043732500526));
#29164=CARTESIAN_POINT('Ctrl Pts',(44.2797550701209,40.9661352620495,46.5673411720669));
#29165=CARTESIAN_POINT('Ctrl Pts',(44.3277941914675,40.9619107653896,46.6303720766722));
#29166=CARTESIAN_POINT('Ctrl Pts',(44.3726409041523,40.9576862687298,46.695797333427));
#29167=CARTESIAN_POINT('Ctrl Pts',(44.4140633294692,40.95346177207,46.7632545347617));
#29168=CARTESIAN_POINT('Ctrl Pts',(44.4555056415842,40.9492352472403,46.8307441221224));
#29169=CARTESIAN_POINT('Ctrl Pts',(44.4935201658159,40.9450087224107,46.9002671850647));
#29170=CARTESIAN_POINT('Ctrl Pts',(44.5279210120423,40.940782197581,46.9714366293666));
#29171=CARTESIAN_POINT('Ctrl Pts',(44.5623847418624,40.9365479468057,47.0427361690267));
#29172=CARTESIAN_POINT('Ctrl Pts',(44.5932214107531,40.9323136960303,47.1156876703405));
#29173=CARTESIAN_POINT('Ctrl Pts',(44.6202933977941,40.928079445255,47.1898841634607));
#29174=CARTESIAN_POINT('Ctrl Pts',(44.6461129446345,40.9240410850097,47.2606480799255));
#29175=CARTESIAN_POINT('Ctrl Pts',(44.6685083686557,40.9200027247644,47.3325439888181));
#29176=CARTESIAN_POINT('Ctrl Pts',(44.6874034892614,40.9159643645191,47.4052095173804));
#29177=CARTESIAN_POINT('Ctrl Pts',(44.7072210101102,40.9117288642529,47.4814223480537));
#29178=CARTESIAN_POINT('Ctrl Pts',(44.7232630846991,40.9074933639866,47.5587715590777));
#29179=CARTESIAN_POINT('Ctrl Pts',(44.7354039584918,40.9032578637204,47.6368488034428));
#29180=CARTESIAN_POINT('Ctrl Pts',(44.7475272318712,40.8990285035851,47.7148128605861));
#29181=CARTESIAN_POINT('Ctrl Pts',(44.7557604637776,40.8947991434498,47.7935023953432));
#29182=CARTESIAN_POINT('Ctrl Pts',(44.7600282069293,40.8905697833146,47.8724958690938));
#29183=CARTESIAN_POINT('Ctrl Pts',(44.7642909662418,40.8863453621951,47.9513970948447));
#29184=CARTESIAN_POINT('Ctrl Pts',(44.7645974140084,40.8821209410756,48.0306010880284));
#29185=CARTESIAN_POINT('Ctrl Pts',(44.7609237204617,40.8778965199561,48.1096796565512));
#29186=CARTESIAN_POINT('Ctrl Pts',(44.7572523761726,40.8736748002741,48.188707655824));
#29187=CARTESIAN_POINT('Ctrl Pts',(44.7496059640198,40.8694530805921,48.2676099220498));
#29188=CARTESIAN_POINT('Ctrl Pts',(44.738012733382,40.86523136091,48.3459579446169));
#29189=CARTESIAN_POINT('Ctrl Pts',(44.7264232959977,40.8610110225559,48.42428033206));
#29190=CARTESIAN_POINT('Ctrl Pts',(44.7108896730341,40.8567906842017,48.5020483719928));
#29191=CARTESIAN_POINT('Ctrl Pts',(44.6914918420243,40.8525703458476,48.5788398559498));
#29192=CARTESIAN_POINT('Ctrl Pts',(44.6720943003632,40.8483500704463,48.655630194443));
#29193=CARTESIAN_POINT('Ctrl Pts',(44.6488327814757,40.844129795045,48.7314435511853));
#29194=CARTESIAN_POINT('Ctrl Pts',(44.6218377787388,40.8399095196437,48.8058705391496));
#29195=CARTESIAN_POINT('Ctrl Pts',(44.5948157747103,40.8356850229839,48.8803719714405));
#29196=CARTESIAN_POINT('Ctrl Pts',(44.5640529874069,40.831460526324,48.9534838225824));
#29197=CARTESIAN_POINT('Ctrl Pts',(44.5297287673595,40.8272360296642,49.0248150166647));
#29198=CARTESIAN_POINT('Ctrl Pts',(44.4953880683438,40.8230095048345,49.0961804566666));
#29199=CARTESIAN_POINT('Ctrl Pts',(44.4574827552199,40.8187829800049,49.1657631238361));
#29200=CARTESIAN_POINT('Ctrl Pts',(44.4162378201187,40.8145564551753,49.2331972646835));
#29201=CARTESIAN_POINT('Ctrl Pts',(44.3749174906589,40.8103222043999,49.3007546728797));
#29202=CARTESIAN_POINT('Ctrl Pts',(44.33024560599,40.8060879536246,49.3661553182307));
#29203=CARTESIAN_POINT('Ctrl Pts',(44.282489987429,40.8018537028492,49.4290632904563));
#29204=CARTESIAN_POINT('Ctrl Pts',(44.2369437026859,40.7978153426039,49.4890609305651));
#29205=CARTESIAN_POINT('Ctrl Pts',(44.1885929592367,40.7937769823586,49.5467911855493));
#29206=CARTESIAN_POINT('Ctrl Pts',(44.1377013096872,40.7897386221133,49.6019939448111));
#29207=CARTESIAN_POINT('Ctrl Pts',(44.0843252901836,40.785503121847,49.6598915288174));
#29208=CARTESIAN_POINT('Ctrl Pts',(44.0279510586162,40.7812676215808,49.715228628654));
#29209=CARTESIAN_POINT('Ctrl Pts',(43.9688540141472,40.7770321213145,49.7676785689696));
#29210=CARTESIAN_POINT('Ctrl Pts',(43.9098426416343,40.7728027611793,49.8200524735201));
#29211=CARTESIAN_POINT('Ctrl Pts',(43.848116642757,40.768573401044,49.8695472212268));
#29212=CARTESIAN_POINT('Ctrl Pts',(43.7839897269887,40.7643440409087,49.9158713100023));
#29213=CARTESIAN_POINT('Ctrl Pts',(43.7199376981628,40.7601196197892,49.9621413018462));
#29214=CARTESIAN_POINT('Ctrl Pts',(43.6534907025532,40.7558951986697,50.0052477192448));
#29215=CARTESIAN_POINT('Ctrl Pts',(43.5849959700272,40.7516707775502,50.0449388724163));
#29216=CARTESIAN_POINT('Ctrl Pts',(43.516545038588,40.7474490578682,50.0846046438456));
#29217=CARTESIAN_POINT('Ctrl Pts',(43.4460493742868,40.7432273381862,50.120859251127));
#29218=CARTESIAN_POINT('Ctrl Pts',(43.3738846492484,40.7390056185041,50.153494632187));
#29219=CARTESIAN_POINT('Ctrl Pts',(43.3017435361867,40.73478528015,50.1861193350957));
#29220=CARTESIAN_POINT('Ctrl Pts',(43.2279348741094,40.7305649417958,50.2151269699477));
#29221=CARTESIAN_POINT('Ctrl Pts',(43.1528570193506,40.7263446034417,50.2403563889066));
#29222=CARTESIAN_POINT('Ctrl Pts',(43.0777802844939,40.7221243280404,50.2655854315298));
#29223=CARTESIAN_POINT('Ctrl Pts',(43.001434839916,40.7179040526391,50.2870362220449));
#29224=CARTESIAN_POINT('Ctrl Pts',(42.9242355874031,40.7136837772378,50.3045970341472));
#29225=CARTESIAN_POINT('Ctrl Pts',(42.8469591176534,40.7094592805779,50.3221754111526));
#29226=CARTESIAN_POINT('Ctrl Pts',(42.7688275927359,40.7052347839181,50.335855932858));
#29227=CARTESIAN_POINT('Ctrl Pts',(42.6902669455783,40.7010102872582,50.3455778693543));
#29228=CARTESIAN_POINT('Ctrl Pts',(42.6116685816595,40.6967837624286,50.3553044733269));
#29229=CARTESIAN_POINT('Ctrl Pts',(42.5326411538339,40.6925572375989,50.3610686718588));
#29230=CARTESIAN_POINT('Ctrl Pts',(42.4536139898798,40.6883307127693,50.3628618201218));
#29231=CARTESIAN_POINT('Ctrl Pts',(42.3744423669193,40.684096461994,50.3646582461997));
#29232=CARTESIAN_POINT('Ctrl Pts',(42.2952714792004,40.6798622112186,50.3624691299369));
#29233=CARTESIAN_POINT('Ctrl Pts',(42.2165287257499,40.6756279604433,50.3563379919751));
#29234=CARTESIAN_POINT('Ctrl Pts',(42.1414288740851,40.671589600198,50.3504905008563));
#29235=CARTESIAN_POINT('Ctrl Pts',(42.0667187686555,40.6675512399527,50.3410577451993));
#29236=CARTESIAN_POINT('Ctrl Pts',(41.9927597494912,40.6635128797074,50.3281206625228));
#29237=CARTESIAN_POINT('Ctrl Pts',(41.9151902840809,40.6592773794411,50.3145520322391));
#29238=CARTESIAN_POINT('Ctrl Pts',(41.8381522505117,40.6550418791749,50.2970766213165));
#29239=CARTESIAN_POINT('Ctrl Pts',(41.7620693805254,40.6508063789087,50.2757493195949));
#29240=CARTESIAN_POINT('Ctrl Pts',(41.6860968065511,40.6465770187734,50.2544529356913));
#29241=CARTESIAN_POINT('Ctrl Pts',(41.6110770945306,40.6423476586382,50.2293158754767));
#29242=CARTESIAN_POINT('Ctrl Pts',(41.5374251200559,40.6381182985029,50.2004442772744));
#29243=CARTESIAN_POINT('Ctrl Pts',(41.4638591558172,40.6338938773834,50.1716063951128));
#29244=CARTESIAN_POINT('Ctrl Pts',(41.3916581898303,40.6296694562639,50.1390428118174));
#29245=CARTESIAN_POINT('Ctrl Pts',(41.3212217486689,40.6254450351445,50.1029093954222));
#29246=CARTESIAN_POINT('Ctrl Pts',(41.2508303502802,40.6212233154624,50.0667990856638));
#29247=CARTESIAN_POINT('Ctrl Pts',(41.1822016536031,40.6170015957804,50.0271236874078));
#29248=CARTESIAN_POINT('Ctrl Pts',(41.1157138801031,40.6127798760984,49.9840865916437));
#29249=CARTESIAN_POINT('Ctrl Pts',(41.0492478611065,40.6085595377442,49.9410635774256));
#29250=CARTESIAN_POINT('Ctrl Pts',(40.9849217680386,40.6043391993901,49.8946813046486));
#29251=CARTESIAN_POINT('Ctrl Pts',(40.923086638139,40.6001188610359,49.8451876225621));
#29252=CARTESIAN_POINT('Ctrl Pts',(40.8612524306058,40.5958985856347,49.7956946787502));
#29253=CARTESIAN_POINT('Ctrl Pts',(40.8019094779762,40.5916783102334,49.74309071222));
#29254=CARTESIAN_POINT('Ctrl Pts',(40.7453762035434,40.5874580348321,49.6876642240385));
#29255=CARTESIAN_POINT('Ctrl Pts',(40.6887863826662,40.5832335381722,49.6321822964567));
#29256=CARTESIAN_POINT('Ctrl Pts',(40.6350121899266,40.5790090415124,49.5738725369367));
#29257=CARTESIAN_POINT('Ctrl Pts',(40.5843351269717,40.5747845448525,49.5130603126614));
#29258=CARTESIAN_POINT('Ctrl Pts',(40.5336337340914,40.5705580200229,49.4522188925963));
#29259=CARTESIAN_POINT('Ctrl Pts',(40.4860327154755,40.5663314951933,49.388872990123));
#29260=CARTESIAN_POINT('Ctrl Pts',(40.4417716043412,40.5621049703636,49.3233790051742));
#29261=CARTESIAN_POINT('Ctrl Pts',(40.3974295853797,40.5578707195883,49.2577652994165));
#29262=CARTESIAN_POINT('Ctrl Pts',(40.3564399171461,40.553636468813,49.1899960675313));
#29263=CARTESIAN_POINT('Ctrl Pts',(40.3189972167955,40.5494022180376,49.1204543083924));
#29264=CARTESIAN_POINT('Ctrl Pts',(40.2832867403507,40.5453638577923,49.0541297824259));
#29265=CARTESIAN_POINT('Ctrl Pts',(40.2508024214045,40.5413254975469,48.9861934463802));
#29266=CARTESIAN_POINT('Ctrl Pts',(40.221671671113,40.5372871373016,48.9169929838709));
#29267=CARTESIAN_POINT('Ctrl Pts',(40.1876925816392,40.5325766577317,48.8362752308537));
#29268=CARTESIAN_POINT('Ctrl Pts',(40.1581660688896,40.5278661781618,48.7535772427311));
#29269=CARTESIAN_POINT('Ctrl Pts',(40.1333014726962,40.5231556985919,48.6693789862394));
#29270=CARTESIAN_POINT('Ctrl Pts',(40.1085164075483,40.5184602858006,48.585450043406));
#29271=CARTESIAN_POINT('Ctrl Pts',(40.0883636356809,40.5137648730092,48.5000306604509));
#29272=CARTESIAN_POINT('Ctrl Pts',(40.073004121357,40.5090694602179,48.4136189329304));
#29273=CARTESIAN_POINT('Ctrl Pts',(40.0577283968686,40.5043996620298,48.3276786021146));
#29274=CARTESIAN_POINT('Ctrl Pts',(40.0471938971035,40.4997298638417,48.2407569881186));
#29275=CARTESIAN_POINT('Ctrl Pts',(40.0415110131285,40.4950600656537,48.1533627715776));
#29276=CARTESIAN_POINT('Ctrl Pts',(40.0382219309356,40.4923573270208,48.1027816295633));
#29277=CARTESIAN_POINT('Ctrl Pts',(40.0365571157034,40.489654588388,48.052042505279));
#29278=CARTESIAN_POINT('Ctrl Pts',(40.0365303286314,40.4869518497552,48.0012463629995));
#29279=CARTESIAN_POINT('',(40.0365308224644,39.6932018496801,47.9980282648923));
#29280=CARTESIAN_POINT('Ctrl Pts',(40.0365303286311,40.4869518497283,48.0012463624935));
#29281=CARTESIAN_POINT('Ctrl Pts',(40.0364879504104,40.4826760072291,47.9208847983668));
#29282=CARTESIAN_POINT('Ctrl Pts',(40.0405485387724,40.4784001647298,47.8405250305544));
#29283=CARTESIAN_POINT('Ctrl Pts',(40.0486851230954,40.4741243222306,47.760607455114));
#29284=CARTESIAN_POINT('Ctrl Pts',(40.0568243739978,40.4698470784217,47.6806636885162));
#29285=CARTESIAN_POINT('Ctrl Pts',(40.0690422298306,40.4655698346129,47.6011628519446));
#29286=CARTESIAN_POINT('Ctrl Pts',(40.0852600030886,40.4612925908041,47.5225388103745));
#29287=CARTESIAN_POINT('Ctrl Pts',(40.1015009109304,40.4570092455254,47.4438026119476));
#29288=CARTESIAN_POINT('Ctrl Pts',(40.1217530396299,40.4527259002467,47.365946150112));
#29289=CARTESIAN_POINT('Ctrl Pts',(40.1458868702053,40.448442554968,47.2893915009043));
#29290=CARTESIAN_POINT('Ctrl Pts',(40.1700380349793,40.4441561331632,47.2127818660826));
#29291=CARTESIAN_POINT('Ctrl Pts',(40.1980762971258,40.4398697113585,47.1374763301334));
#29292=CARTESIAN_POINT('Ctrl Pts',(40.2298235847538,40.4355832895538,47.0638778030572));
#29293=CARTESIAN_POINT('Ctrl Pts',(40.2616371863975,40.4312879142332,46.9901255427255));
#29294=CARTESIAN_POINT('Ctrl Pts',(40.297175095069,40.4269925389126,46.9180878228388));
#29295=CARTESIAN_POINT('Ctrl Pts',(40.3362127465961,40.422697163592,46.8481438398883));
#29296=CARTESIAN_POINT('Ctrl Pts',(40.371462524921,40.4188185740266,46.7849866109636));
#29297=CARTESIAN_POINT('Ctrl Pts',(40.4095651002173,40.4149399844611,46.7235363621325));
#29298=CARTESIAN_POINT('Ctrl Pts',(40.4503260771266,40.4110613948956,46.6640501374051));
#29299=CARTESIAN_POINT('Ctrl Pts',(40.4948379094919,40.4068258946294,46.5990899459699));
#29300=CARTESIAN_POINT('Ctrl Pts',(40.5426844648708,40.4025903943631,46.5362333175087));
#29301=CARTESIAN_POINT('Ctrl Pts',(40.5936400916276,40.3983548940969,46.4758430781823));
#29302=CARTESIAN_POINT('Ctrl Pts',(40.6445218488996,40.3941255339616,46.4155403855344));
#29303=CARTESIAN_POINT('Ctrl Pts',(40.6985034269968,40.3898961738264,46.3576973374298));
#29304=CARTESIAN_POINT('Ctrl Pts',(40.755316211548,40.3856668136911,46.3026474506151));
#29305=CARTESIAN_POINT('Ctrl Pts',(40.8120626505459,40.3814423925716,46.2476618506548));
#29306=CARTESIAN_POINT('Ctrl Pts',(40.8716333905205,40.3772179714521,46.1954632550286));
#29307=CARTESIAN_POINT('Ctrl Pts',(40.9337209287244,40.3729935503327,46.1463505924692));
#29308=CARTESIAN_POINT('Ctrl Pts',(40.9957687631211,40.3687718306506,46.0972693365293));
#29309=CARTESIAN_POINT('Ctrl Pts',(41.0603298342292,40.3645501109686,46.051270387283));
#29310=CARTESIAN_POINT('Ctrl Pts',(41.127062228754,40.3603283912866,46.0086135805838));
#29311=CARTESIAN_POINT('Ctrl Pts',(41.1937727887366,40.3561080529324,45.9659707310018));
#29312=CARTESIAN_POINT('Ctrl Pts',(41.2626528662615,40.3518877145782,45.9266681051667));
#29313=CARTESIAN_POINT('Ctrl Pts',(41.3333313641073,40.3476673762241,45.8909223669806));
#29314=CARTESIAN_POINT('Ctrl Pts',(41.404008807674,40.3434471008228,45.8551771619974));
#29315=CARTESIAN_POINT('Ctrl Pts',(41.4764841988021,40.3392268254215,45.8229889498333));
#29316=CARTESIAN_POINT('Ctrl Pts',(41.5503629715907,40.3350065500202,45.7945278598777));
#29317=CARTESIAN_POINT('Ctrl Pts',(41.624315640363,40.3307820533604,45.7660383022018));
#29318=CARTESIAN_POINT('Ctrl Pts',(41.699674055859,40.3265575567006,45.7412834829944));
#29319=CARTESIAN_POINT('Ctrl Pts',(41.7760254146192,40.3223330600407,45.7203846469856));
#29320=CARTESIAN_POINT('Ctrl Pts',(41.852413429467,40.3181065352111,45.6994757775004));
#29321=CARTESIAN_POINT('Ctrl Pts',(41.9297948782545,40.3138800103814,45.682426680252));
#29322=CARTESIAN_POINT('Ctrl Pts',(42.0077461208794,40.3096534855518,45.6693075416918));
#29323=CARTESIAN_POINT('Ctrl Pts',(42.0858398557624,40.3054192347765,45.6561644217861));
#29324=CARTESIAN_POINT('Ctrl Pts',(42.1645049983709,40.3011849840011,45.6469656702076));
#29325=CARTESIAN_POINT('Ctrl Pts',(42.2433123288832,40.2969507332258,45.6417295713553));
#29326=CARTESIAN_POINT('Ctrl Pts',(42.3184737700608,40.2929123729805,45.6367357118586));
#29327=CARTESIAN_POINT('Ctrl Pts',(42.3937641761254,40.2888740127351,45.6353459322716));
#29328=CARTESIAN_POINT('Ctrl Pts',(42.4688143307643,40.2848356524898,45.6375320047075));
#29329=CARTESIAN_POINT('Ctrl Pts',(42.547528197444,40.2806001522236,45.6398247943107));
#29330=CARTESIAN_POINT('Ctrl Pts',(42.6262769653922,40.2763646519573,45.6460601892281));
#29331=CARTESIAN_POINT('Ctrl Pts',(42.7046334120102,40.2721291516911,45.6562446959661));
#29332=CARTESIAN_POINT('Ctrl Pts',(42.7828762666518,40.2678997915558,45.6664144384021));
#29333=CARTESIAN_POINT('Ctrl Pts',(42.8607274678836,40.2636704314206,45.6805218639176));
#29334=CARTESIAN_POINT('Ctrl Pts',(42.9377612006724,40.2594410712853,45.6985214900088));
#29335=CARTESIAN_POINT('Ctrl Pts',(43.0147049740326,40.2552166501658,45.7165000962686));
#29336=CARTESIAN_POINT('Ctrl Pts',(43.0908327213179,40.2509922290463,45.7383617645431));
#29337=CARTESIAN_POINT('Ctrl Pts',(43.1657266787048,40.2467678079268,45.7640095942917));
#29338=CARTESIAN_POINT('Ctrl Pts',(43.2405727428216,40.2425460882448,45.7896410227379));
#29339=CARTESIAN_POINT('Ctrl Pts',(43.3141861401709,40.2383243685628,45.8190536554844));
#29340=CARTESIAN_POINT('Ctrl Pts',(43.3861633693248,40.2341026488807,45.8521005028396));
#29341=CARTESIAN_POINT('Ctrl Pts',(43.45811704785,40.2298823105266,45.8851365374136));
#29342=CARTESIAN_POINT('Ctrl Pts',(43.5284351949817,40.2256619721724,45.9218042297505));
#29343=CARTESIAN_POINT('Ctrl Pts',(43.5967348298591,40.2214416338183,45.9619086899989));
#29344=CARTESIAN_POINT('Ctrl Pts',(43.6650334459419,40.217221358417,46.0020125520272));
#29345=CARTESIAN_POINT('Ctrl Pts',(43.7313132055605,40.2130010830157,46.0455528412591));
#29346=CARTESIAN_POINT('Ctrl Pts',(43.7952175683292,40.2087808076144,46.0922897552496));
#29347=CARTESIAN_POINT('Ctrl Pts',(43.8591858503478,40.2045563109546,46.1390734170419));
#29348=CARTESIAN_POINT('Ctrl Pts',(43.9207736095071,40.2003318142947,46.1890598130093));
#29349=CARTESIAN_POINT('Ctrl Pts',(43.9796555524277,40.1961073176349,46.2419673562234));
#29350=CARTESIAN_POINT('Ctrl Pts',(44.0385657644152,40.1918807928052,46.2949003002105));
#29351=CARTESIAN_POINT('Ctrl Pts',(44.0947672389277,40.1876542679756,46.3507568539537));
#29352=CARTESIAN_POINT('Ctrl Pts',(44.1479717615001,40.1834277431459,46.4092186945095));
#29353=CARTESIAN_POINT('Ctrl Pts',(44.2012735401561,40.1791934923706,46.4677874013498));
#29354=CARTESIAN_POINT('Ctrl Pts',(44.2515671210607,40.1749592415953,46.5289705478201));
#29355=CARTESIAN_POINT('Ctrl Pts',(44.2986049222509,40.1707249908199,46.5924170397079));
#29356=CARTESIAN_POINT('Ctrl Pts',(44.3434665982432,40.1666866305746,46.6529282857674));
#29357=CARTESIAN_POINT('Ctrl Pts',(44.385366910784,40.1626482703293,46.7154977714741));
#29358=CARTESIAN_POINT('Ctrl Pts',(44.4241298574355,40.158609910084,46.7797997045));
#29359=CARTESIAN_POINT('Ctrl Pts',(44.4647850889873,40.1543744098177,46.8472406552591));
#29360=CARTESIAN_POINT('Ctrl Pts',(44.5021433601042,40.1501389095515,46.916843874885));
#29361=CARTESIAN_POINT('Ctrl Pts',(44.5359680748416,40.1459034092852,46.9882535771461));
#29362=CARTESIAN_POINT('Ctrl Pts',(44.569743754479,40.14167404915,47.0595597580053));
#29363=CARTESIAN_POINT('Ctrl Pts',(44.5999958509682,40.1374446890147,47.1326668003879));
#29364=CARTESIAN_POINT('Ctrl Pts',(44.6265322540626,40.1332153288794,47.2071919762523));
#29365=CARTESIAN_POINT('Ctrl Pts',(44.65303766814,40.1289909077599,47.2816301221625));
#29366=CARTESIAN_POINT('Ctrl Pts',(44.6758358549175,40.1247664866405,47.3574826707428));
#29367=CARTESIAN_POINT('Ctrl Pts',(44.6947823037968,40.120542065521,47.4343458485249));
#29368=CARTESIAN_POINT('Ctrl Pts',(44.7137166367802,40.1163203458389,47.5111598737575));
#29369=CARTESIAN_POINT('Ctrl Pts',(44.7288040085917,40.1120986261569,47.5889827909877));
#29370=CARTESIAN_POINT('Ctrl Pts',(44.739949750849,40.1078769064749,47.6673957240175));
#29371=CARTESIAN_POINT('Ctrl Pts',(44.7510918462691,40.1036565681207,47.7457830006848));
#29372=CARTESIAN_POINT('Ctrl Pts',(44.7582948070186,40.0994362297666,47.8247594454883));
#29373=CARTESIAN_POINT('Ctrl Pts',(44.7615153515461,40.0952158914124,47.903897527024));
#29374=CARTESIAN_POINT('Ctrl Pts',(44.7647358480343,40.0909956160111,47.9830344280927));
#29375=CARTESIAN_POINT('Ctrl Pts',(44.7639740286308,40.0867753406098,48.0623324920834));
#29376=CARTESIAN_POINT('Ctrl Pts',(44.759238688608,40.0825550652085,48.141362127443));
#29377=CARTESIAN_POINT('Ctrl Pts',(44.754498612142,40.0783305685487,48.220470810849));
#29378=CARTESIAN_POINT('Ctrl Pts',(44.7457771037386,40.0741060718888,48.2993100596483));
#29379=CARTESIAN_POINT('Ctrl Pts',(44.733135004958,40.069881575229,48.3774539568475));
#29380=CARTESIAN_POINT('Ctrl Pts',(44.7204868367387,40.0656550503993,48.4556353707275));
#29381=CARTESIAN_POINT('Ctrl Pts',(44.7039144267388,40.0614285255697,48.5331203083622));
#29382=CARTESIAN_POINT('Ctrl Pts',(44.683529571915,40.05720200074,48.6094941632941));
#29383=CARTESIAN_POINT('Ctrl Pts',(44.6631074542601,40.0529677499647,48.6860076270723));
#29384=CARTESIAN_POINT('Ctrl Pts',(44.6388591101169,40.0487334991894,48.761405501701));
#29385=CARTESIAN_POINT('Ctrl Pts',(44.6109458798371,40.044499248414,48.8352896248197));
#29386=CARTESIAN_POINT('Ctrl Pts',(44.5843240084693,40.0404608881687,48.9057556225588));
#29387=CARTESIAN_POINT('Ctrl Pts',(44.554369027367,40.0364225279234,48.9748445206523));
#29388=CARTESIAN_POINT('Ctrl Pts',(44.5212597212008,40.0323841676781,49.0422320452333));
#29389=CARTESIAN_POINT('Ctrl Pts',(44.4865341230461,40.0281486674118,49.1129092164035));
#29390=CARTESIAN_POINT('Ctrl Pts',(44.4482063685516,40.0239131671456,49.1819833203683));
#29391=CARTESIAN_POINT('Ctrl Pts',(44.4064476875312,40.0196776668794,49.2490628959746));
#29392=CARTESIAN_POINT('Ctrl Pts',(44.3647495433436,40.0154483067441,49.3160452274883));
#29393=CARTESIAN_POINT('Ctrl Pts',(44.3196305955762,40.0112189466088,49.3810383774373));
#29394=CARTESIAN_POINT('Ctrl Pts',(44.2713087992454,40.0069895864736,49.4436737230991));
#29395=CARTESIAN_POINT('Ctrl Pts',(44.2230434327543,40.0027651653541,49.5062359236632));
#29396=CARTESIAN_POINT('Ctrl Pts',(44.1715829355024,39.9985407442346,49.5664454218263));
#29397=CARTESIAN_POINT('Ctrl Pts',(44.1171887133054,39.9943163231151,49.6239622421093));
#29398=CARTESIAN_POINT('Ctrl Pts',(44.0628292751853,39.9900946034331,49.6814422814729));
#29399=CARTESIAN_POINT('Ctrl Pts',(44.0055401573259,39.985872883751,49.7362327205046));
#29400=CARTESIAN_POINT('Ctrl Pts',(43.9456224315768,39.981651164069,49.7880273319797));
#29401=CARTESIAN_POINT('Ctrl Pts',(43.8857243106408,39.9774308257149,49.8398049964887));
#29402=CARTESIAN_POINT('Ctrl Pts',(43.8231996444346,39.9732104873607,49.8885884731295));
#29403=CARTESIAN_POINT('Ctrl Pts',(43.7583845839174,39.9689901490066,49.9341100700518));
#29404=CARTESIAN_POINT('Ctrl Pts',(43.6935704902169,39.9647698736053,49.9796309879491));
#29405=CARTESIAN_POINT('Ctrl Pts',(43.626466454971,39.960549598204,50.0218898541813));
#29406=CARTESIAN_POINT('Ctrl Pts',(43.5574385349003,39.9563293228027,50.060661660445));
#29407=CARTESIAN_POINT('Ctrl Pts',(43.4883415708289,39.9521048261428,50.0994722475472));
#29408=CARTESIAN_POINT('Ctrl Pts',(43.4173172880305,39.947880329483,50.1347885768163));
#29409=CARTESIAN_POINT('Ctrl Pts',(43.344756809417,39.9436558328232,50.1664314002433));
#29410=CARTESIAN_POINT('Ctrl Pts',(43.2721614947074,39.9394293079935,50.1980894153071));
#29411=CARTESIAN_POINT('Ctrl Pts',(43.1980289546627,39.9352027831639,50.2260702451727));
#29412=CARTESIAN_POINT('Ctrl Pts',(43.1227683661523,39.9309762583342,50.2502436156536));
#29413=CARTESIAN_POINT('Ctrl Pts',(43.0473702038093,39.9267420075589,50.2744611742452));
#29414=CARTESIAN_POINT('Ctrl Pts',(42.9708403272855,39.9225077567836,50.2948572447362));
#29415=CARTESIAN_POINT('Ctrl Pts',(42.8936008860584,39.9182735060082,50.3113521164423));
#29416=CARTESIAN_POINT('Ctrl Pts',(42.8199347983912,39.9142351457629,50.3270838804978));
#29417=CARTESIAN_POINT('Ctrl Pts',(42.7456237061773,39.9101967855176,50.3392674065297));
#29418=CARTESIAN_POINT('Ctrl Pts',(42.6710370538251,39.9061584252723,50.347877628062));
#29419=CARTESIAN_POINT('Ctrl Pts',(42.5928093161525,39.9019229250061,50.3569081734757));
#29420=CARTESIAN_POINT('Ctrl Pts',(42.5139810670693,39.8976874247398,50.362041958593));
#29421=CARTESIAN_POINT('Ctrl Pts',(42.4349741702642,39.8934519244736,50.3632112153412));
#29422=CARTESIAN_POINT('Ctrl Pts',(42.3560818083822,39.8892225643383,50.3643787770382));
#29423=CARTESIAN_POINT('Ctrl Pts',(42.2770117784023,39.8849932042031,50.3615932166178));
#29424=CARTESIAN_POINT('Ctrl Pts',(42.198192014189,39.8807638440678,50.3548384186103));
#29425=CARTESIAN_POINT('Ctrl Pts',(42.1194642951185,39.8765394229483,50.3480915088064));
#29426=CARTESIAN_POINT('Ctrl Pts',(42.0409867262507,39.8723150018288,50.3373846123811));
#29427=CARTESIAN_POINT('Ctrl Pts',(41.9631866548269,39.8680905807093,50.3227536551212));
#29428=CARTESIAN_POINT('Ctrl Pts',(41.8854363350783,39.8638688610273,50.3081320540819));
#29429=CARTESIAN_POINT('Ctrl Pts',(41.8083631128912,39.8596471413453,50.2895914592671));
#29430=CARTESIAN_POINT('Ctrl Pts',(41.7323874112646,39.8554254216633,50.2672194142301));
#29431=CARTESIAN_POINT('Ctrl Pts',(41.6564365685492,39.8512050833091,50.2448546892266));
#29432=CARTESIAN_POINT('Ctrl Pts',(41.5815829832299,39.846984744955,50.2186611357793));
#29433=CARTESIAN_POINT('Ctrl Pts',(41.5082336464741,39.8427644066008,50.1887766472665));
#29434=CARTESIAN_POINT('Ctrl Pts',(41.4348854038371,39.8385441311995,50.1588926045271));
#29435=CARTESIAN_POINT('Ctrl Pts',(41.3630417993178,39.8343238557983,50.1253179144891));
#29436=CARTESIAN_POINT('Ctrl Pts',(41.2930901047849,39.830103580397,50.0882387135514));
#29437=CARTESIAN_POINT('Ctrl Pts',(41.2230684422614,39.8258790837371,50.0511224247748));
#29438=CARTESIAN_POINT('Ctrl Pts',(41.1549428856186,39.8216545870773,50.0104948431069));
#29439=CARTESIAN_POINT('Ctrl Pts',(41.0890757816296,39.8174300904174,49.9665879422467));
#29440=CARTESIAN_POINT('Ctrl Pts',(41.0231770550162,39.8132035655878,49.9226599617981));
#29441=CARTESIAN_POINT('Ctrl Pts',(40.9595393185366,39.8089770407581,49.8754498058017));
#29442=CARTESIAN_POINT('Ctrl Pts',(40.8984934976422,39.8047505159285,49.8252311262625));
#29443=CARTESIAN_POINT('Ctrl Pts',(40.8373360870338,39.8005162651532,49.7749206486607));
#29444=CARTESIAN_POINT('Ctrl Pts',(40.7787804074337,39.7962820143778,49.7215909751311));
#29445=CARTESIAN_POINT('Ctrl Pts',(40.7231218770389,39.7920477636025,49.6655540224305));
#29446=CARTESIAN_POINT('Ctrl Pts',(40.6700382954596,39.7880094033571,49.6121095256205));
#29447=CARTESIAN_POINT('Ctrl Pts',(40.6195899396743,39.7839710431118,49.556202995311));
#29448=CARTESIAN_POINT('Ctrl Pts',(40.5719977575736,39.7799326828665,49.4981315838684));
#29449=CARTESIAN_POINT('Ctrl Pts',(40.5222903575728,39.7757148391114,49.4374792088401));
#29450=CARTESIAN_POINT('Ctrl Pts',(40.4755045721295,39.7714969953564,49.3742277636628));
#29451=CARTESIAN_POINT('Ctrl Pts',(40.4319254715984,39.7672791516013,49.3086913660436));
#29452=CARTESIAN_POINT('Ctrl Pts',(40.3884068159339,39.7630671580589,49.2432458683916));
#29453=CARTESIAN_POINT('Ctrl Pts',(40.3480862789779,39.7588551645164,49.1755220970716));
#29454=CARTESIAN_POINT('Ctrl Pts',(40.3112091156363,39.754643170974,49.1058675699644));
#29455=CARTESIAN_POINT('Ctrl Pts',(40.2743713555646,39.750435677949,49.0362874687588));
#29456=CARTESIAN_POINT('Ctrl Pts',(40.2409698857243,39.7462281849241,48.9647811226784));
#29457=CARTESIAN_POINT('Ctrl Pts',(40.2112061406572,39.7420206918991,48.8917241065504));
#29458=CARTESIAN_POINT('Ctrl Pts',(40.181461551302,39.7378159067835,48.8187141093428));
#29459=CARTESIAN_POINT('Ctrl Pts',(40.1553502204571,39.733611121668,48.7441558588768));
#29460=CARTESIAN_POINT('Ctrl Pts',(40.1330265412458,39.7294063365524,48.6684472890242));
#29461=CARTESIAN_POINT('Ctrl Pts',(40.1107120521572,39.7252032824459,48.5927698865721));
#29462=CARTESIAN_POINT('Ctrl Pts',(40.0921822489825,39.7210002283394,48.5159435595929));
#29463=CARTESIAN_POINT('Ctrl Pts',(40.0775419483511,39.7167971742329,48.438382298036));
#29464=CARTESIAN_POINT('Ctrl Pts',(40.0628968075301,39.7125927305662,48.3607953941631));
#29465=CARTESIAN_POINT('Ctrl Pts',(40.0521438325292,39.7083882868995,48.2824735346466));
#29466=CARTESIAN_POINT('Ctrl Pts',(40.0453366784163,39.7041838432328,48.2038408273345));
#29467=CARTESIAN_POINT('Ctrl Pts',(40.0394099234416,39.7005231787313,48.1353780334109));
#29468=CARTESIAN_POINT('Ctrl Pts',(40.0364735495153,39.6968625142298,48.0666799369991));
#29469=CARTESIAN_POINT('Ctrl Pts',(40.0365308224637,39.6932018497283,47.9980282657969));
#29470=CARTESIAN_POINT('',(40.0365300273278,38.8994518497758,47.9996405879596));
#29471=CARTESIAN_POINT('Ctrl Pts',(40.0365308224644,39.6932018496801,47.9980282648923));
#29472=CARTESIAN_POINT('Ctrl Pts',(40.036609302553,39.6881857094131,47.9039561607262));
#29473=CARTESIAN_POINT('Ctrl Pts',(40.0423081124997,39.6831695691462,47.8101261109713));
#29474=CARTESIAN_POINT('Ctrl Pts',(40.0535177843081,39.6781534288793,47.717136689651));
#29475=CARTESIAN_POINT('Ctrl Pts',(40.064867614996,39.6730745698628,47.6229845854869));
#29476=CARTESIAN_POINT('Ctrl Pts',(40.0818668921383,39.6679957108462,47.529694318329));
#29477=CARTESIAN_POINT('Ctrl Pts',(40.1043529074695,39.6629168518297,47.4378657923091));
#29478=CARTESIAN_POINT('Ctrl Pts',(40.117944819063,39.6598468813734,47.3823590611679));
#29479=CARTESIAN_POINT('Ctrl Pts',(40.1335404969883,39.656776910917,47.3273859930675));
#29480=CARTESIAN_POINT('Ctrl Pts',(40.1510956352582,39.6537069404606,47.273075245197));
#29481=CARTESIAN_POINT('Ctrl Pts',(40.175315670556,39.6494714401943,47.1981451472256));
#29482=CARTESIAN_POINT('Ctrl Pts',(40.2033306781086,39.6452359399281,47.1242844137133));
#29483=CARTESIAN_POINT('Ctrl Pts',(40.2350273968893,39.6410004396618,47.0519050318242));
#29484=CARTESIAN_POINT('Ctrl Pts',(40.2666781654886,39.6367710795266,46.979630577065));
#29485=CARTESIAN_POINT('Ctrl Pts',(40.3019998596699,39.6325417193913,46.9088336356899));
#29486=CARTESIAN_POINT('Ctrl Pts',(40.3408296986338,39.6283123592561,46.8399103005063));
#29487=CARTESIAN_POINT('Ctrl Pts',(40.3796141923963,39.6240879381366,46.7710674534884));
#29488=CARTESIAN_POINT('Ctrl Pts',(40.4218984606851,39.6198635170171,46.704094271529));
#29489=CARTESIAN_POINT('Ctrl Pts',(40.4674726095466,39.6156390958976,46.6393647343806));
#29490=CARTESIAN_POINT('Ctrl Pts',(40.5130176146013,39.6114173762155,46.5746765905477));
#29491=CARTESIAN_POINT('Ctrl Pts',(40.5618480551299,39.6071956565335,46.5122296265529));
#29492=CARTESIAN_POINT('Ctrl Pts',(40.613709937326,39.6029739368515,46.4523701176017));
#29493=CARTESIAN_POINT('Ctrl Pts',(40.6655548505453,39.5987535984973,46.3925301944152));
#29494=CARTESIAN_POINT('Ctrl Pts',(40.7204289287941,39.5945332601431,46.3352763996614));
#29495=CARTESIAN_POINT('Ctrl Pts',(40.7780379306252,39.590312921789,46.2809219079957));
#29496=CARTESIAN_POINT('Ctrl Pts',(40.8356460731289,39.5860926463877,46.2265682271113));
#29497=CARTESIAN_POINT('Ctrl Pts',(40.8959887158222,39.5818723709864,46.1751140844765));
#29498=CARTESIAN_POINT('Ctrl Pts',(40.9587358939018,39.5776520955851,46.1268347063399));
#29499=CARTESIAN_POINT('Ctrl Pts',(41.0215458337771,39.5734275989253,46.0785070375779));
#29500=CARTESIAN_POINT('Ctrl Pts',(41.0867647406477,39.5692031022654,46.0333607636821));
#29501=CARTESIAN_POINT('Ctrl Pts',(41.1540312741243,39.5649786056056,45.9916294228804));
#29502=CARTESIAN_POINT('Ctrl Pts',(41.2213301020876,39.5607520807759,45.9498780469712));
#29503=CARTESIAN_POINT('Ctrl Pts',(41.2906781036953,39.5565255559463,45.9115450976135));
#29504=CARTESIAN_POINT('Ctrl Pts',(41.3616890412668,39.5522990311166,45.8768182381448));
#29505=CARTESIAN_POINT('Ctrl Pts',(41.4328297844515,39.5480647803413,45.8420278991413));
#29506=CARTESIAN_POINT('Ctrl Pts',(41.5056391052079,39.5438305295659,45.8108570072194));
#29507=CARTESIAN_POINT('Ctrl Pts',(41.579710669082,39.5395962787906,45.78344504817));
#29508=CARTESIAN_POINT('Ctrl Pts',(41.6503554359434,39.5355579185453,45.7573012575576));
#29509=CARTESIAN_POINT('Ctrl Pts',(41.7221478859671,39.5315195583,45.7345763625703));
#29510=CARTESIAN_POINT('Ctrl Pts',(41.7947259995611,39.5274811980547,45.7153482048039));
#29511=CARTESIAN_POINT('Ctrl Pts',(41.8708471479427,39.5232456977884,45.6951813889697));
#29512=CARTESIAN_POINT('Ctrl Pts',(41.9481219784927,39.5190101975222,45.6787847683847));
#29513=CARTESIAN_POINT('Ctrl Pts',(42.0261427251915,39.5147746972559,45.6662859688958));
#29514=CARTESIAN_POINT('Ctrl Pts',(42.1040503665722,39.5105453371207,45.6538052886988));
#29515=CARTESIAN_POINT('Ctrl Pts',(42.1827013172257,39.5063159769854,45.6452112821123));
#29516=CARTESIAN_POINT('Ctrl Pts',(42.261674388957,39.5020866168502,45.6405813287529));
#29517=CARTESIAN_POINT('Ctrl Pts',(42.340555236514,39.4978621957307,45.6359567822191));
#29518=CARTESIAN_POINT('Ctrl Pts',(42.4197569915148,39.4936377746112,45.6352871171725));
#29519=CARTESIAN_POINT('Ctrl Pts',(42.4988515756488,39.4894133534917,45.6385981267705));
#29520=CARTESIAN_POINT('Ctrl Pts',(42.5778955802913,39.4851916338097,45.6419070190404));
#29521=CARTESIAN_POINT('Ctrl Pts',(42.6568320824179,39.4809699141276,45.6491915139728));
#29522=CARTESIAN_POINT('Ctrl Pts',(42.7352324463743,39.4767481944456,45.6604253275867));
#29523=CARTESIAN_POINT('Ctrl Pts',(42.8136071580807,39.4725278560914,45.6716554655468));
#29524=CARTESIAN_POINT('Ctrl Pts',(42.8914456156923,39.4683075177373,45.6868322897868));
#29525=CARTESIAN_POINT('Ctrl Pts',(42.9683252484153,39.4640871793831,45.7058777598145));
#29526=CARTESIAN_POINT('Ctrl Pts',(43.0452037343597,39.4598669039819,45.7249229457496));
#29527=CARTESIAN_POINT('Ctrl Pts',(43.1211229685864,39.4556466285806,45.7478365486077));
#29528=CARTESIAN_POINT('Ctrl Pts',(43.1956729699453,39.4514263531793,45.7744899537862));
#29529=CARTESIAN_POINT('Ctrl Pts',(43.2702975386727,39.4472018565194,45.8011700185791));
#29530=CARTESIAN_POINT('Ctrl Pts',(43.3435496956695,39.4429773598596,45.8315971997728));
#29531=CARTESIAN_POINT('Ctrl Pts',(43.4150375466559,39.4387528631998,45.8655939421519));
#29532=CARTESIAN_POINT('Ctrl Pts',(43.4865597187727,39.4345263383701,45.8996070062781));
#29533=CARTESIAN_POINT('Ctrl Pts',(43.5563154837181,39.4302998135405,45.9371928226232));
#29534=CARTESIAN_POINT('Ctrl Pts',(43.6239380600601,39.4260732887108,45.978128078726));
#29535=CARTESIAN_POINT('Ctrl Pts',(43.6916842482046,39.4218390379355,46.0191381631046));
#29536=CARTESIAN_POINT('Ctrl Pts',(43.7572890660339,39.4176047871602,46.0635096581189));
#29537=CARTESIAN_POINT('Ctrl Pts',(43.8204153786014,39.4133705363848,46.1109762857146));
#29538=CARTESIAN_POINT('Ctrl Pts',(43.8806212579013,39.4093321761395,46.1562469491759));
#29539=CARTESIAN_POINT('Ctrl Pts',(43.9385726368473,39.4052938158942,46.2043324398239));
#29540=CARTESIAN_POINT('Ctrl Pts',(43.9940081989544,39.4012554556489,46.2549704006619));
#29541=CARTESIAN_POINT('Ctrl Pts',(44.0521499505075,39.3970199553827,46.3080803471707));
#29542=CARTESIAN_POINT('Ctrl Pts',(44.1077449942743,39.3927844551164,46.3642002163054));
#29543=CARTESIAN_POINT('Ctrl Pts',(44.1604653953895,39.3885489548502,46.4230561098961));
#29544=CARTESIAN_POINT('Ctrl Pts',(44.2131093686571,39.3843195947149,46.4818266811225));
#29545=CARTESIAN_POINT('Ctrl Pts',(44.2628866643237,39.3800902345796,46.5433250536541));
#29546=CARTESIAN_POINT('Ctrl Pts',(44.3095043447309,39.3758608744444,46.6072388581118));
#29547=CARTESIAN_POINT('Ctrl Pts',(44.3560675853526,39.3716364533249,46.671078024497));
#29548=CARTESIAN_POINT('Ctrl Pts',(44.3994782678398,39.3674120322054,46.7373266402747));
#29549=CARTESIAN_POINT('Ctrl Pts',(44.4394831127008,39.3631876110859,46.8056386334496));
#29550=CARTESIAN_POINT('Ctrl Pts',(44.4794623752197,39.3589658914038,46.8739069423962));
#29551=CARTESIAN_POINT('Ctrl Pts',(44.5160398863722,39.3547441717218,46.9442356059145));
#29552=CARTESIAN_POINT('Ctrl Pts',(44.549005863483,39.3505224520398,47.0162499099793));
#29553=CARTESIAN_POINT('Ctrl Pts',(44.5819610542729,39.3463021136856,47.0882406512845));
#29554=CARTESIAN_POINT('Ctrl Pts',(44.6113068622305,39.3420817753315,47.1619155115332));
#29555=CARTESIAN_POINT('Ctrl Pts',(44.636880314397,39.3378614369773,47.2368768775859));
#29556=CARTESIAN_POINT('Ctrl Pts',(44.662453385096,39.333641161576,47.3118371254739));
#29557=CARTESIAN_POINT('Ctrl Pts',(44.6842540615746,39.3294208861747,47.3880833963766));
#29558=CARTESIAN_POINT('Ctrl Pts',(44.7021687160105,39.3252006107735,47.4652013052347));
#29559=CARTESIAN_POINT('Ctrl Pts',(44.7201012892742,39.3209761141136,47.5423963499672));
#29560=CARTESIAN_POINT('Ctrl Pts',(44.7341399694105,39.3167516174537,47.6204643159974));
#29561=CARTESIAN_POINT('Ctrl Pts',(44.744222073869,39.3125271207939,47.6989795533768));
#29562=CARTESIAN_POINT('Ctrl Pts',(44.7543090187195,39.3083005959643,47.7775324857163));
#29563=CARTESIAN_POINT('Ctrl Pts',(44.7604355674331,39.3040740711346,47.8565326485915));
#29564=CARTESIAN_POINT('Ctrl Pts',(44.7625911064243,39.299847546305,47.9355507583827));
#29565=CARTESIAN_POINT('Ctrl Pts',(44.7647505856684,39.2956132955296,48.0147133106296));
#29566=CARTESIAN_POINT('Ctrl Pts',(44.7629245611091,39.2913790447543,48.0938934048865));
#29567=CARTESIAN_POINT('Ctrl Pts',(44.7571545929269,39.2871447939789,48.1726634470399));
#29568=CARTESIAN_POINT('Ctrl Pts',(44.751651562672,39.2831064337336,48.2477893249418));
#29569=CARTESIAN_POINT('Ctrl Pts',(44.7425615182468,39.2790680734883,48.322541902322));
#29570=CARTESIAN_POINT('Ctrl Pts',(44.7299637392547,39.275029713243,48.3965594717799));
#29571=CARTESIAN_POINT('Ctrl Pts',(44.7167509763921,39.2707942129767,48.4741903457243));
#29572=CARTESIAN_POINT('Ctrl Pts',(44.6996290368853,39.2665587127105,48.5513077094673));
#29573=CARTESIAN_POINT('Ctrl Pts',(44.6786508668115,39.2623232124442,48.6274875840041));
#29574=CARTESIAN_POINT('Ctrl Pts',(44.6577031084255,39.258093852309,48.7035570219033));
#29575=CARTESIAN_POINT('Ctrl Pts',(44.6329103443977,39.2538644921737,48.7786912207728));
#29576=CARTESIAN_POINT('Ctrl Pts',(44.6043768093628,39.2496351320385,48.8524748226449));
#29577=CARTESIAN_POINT('Ctrl Pts',(44.5758765955811,39.245410710919,48.9261722605674));
#29578=CARTESIAN_POINT('Ctrl Pts',(44.5436444601154,39.2411862897995,48.9985218002329));
#29579=CARTESIAN_POINT('Ctrl Pts',(44.5078344371775,39.23696186868,49.0691232044758));
#29580=CARTESIAN_POINT('Ctrl Pts',(44.4720473140723,39.232740148998,49.1396794604553));
#29581=CARTESIAN_POINT('Ctrl Pts',(44.4326870564077,39.2285184293159,49.2084893823486));
#29582=CARTESIAN_POINT('Ctrl Pts',(44.389955318554,39.2242967096339,49.2751738199394));
#29583=CARTESIAN_POINT('Ctrl Pts',(44.3472375623345,39.2200763712797,49.3418364386792));
#29584=CARTESIAN_POINT('Ctrl Pts',(44.3011507694226,39.2158560329256,49.4063745591698));
#29585=CARTESIAN_POINT('Ctrl Pts',(44.2519411766446,39.2116356945714,49.4684360112542));
#29586=CARTESIAN_POINT('Ctrl Pts',(44.2027323179038,39.2074154191702,49.5304965375961));
#29587=CARTESIAN_POINT('Ctrl Pts',(44.1504010445462,39.2031951437689,49.5900801020268));
#29588=CARTESIAN_POINT('Ctrl Pts',(44.0952343943522,39.1989748683676,49.6468669615683));
#29589=CARTESIAN_POINT('Ctrl Pts',(44.0400125646563,39.1947503717077,49.7037106211985));
#29590=CARTESIAN_POINT('Ctrl Pts',(43.9819500206073,39.1905258750479,49.7577516504136));
#29591=CARTESIAN_POINT('Ctrl Pts',(43.9213708350321,39.1863013783881,49.8087070584298));
#29592=CARTESIAN_POINT('Ctrl Pts',(43.8607625655483,39.1820748535584,49.8596869300041));
#29593=CARTESIAN_POINT('Ctrl Pts',(43.7976356220278,39.1778483287288,49.9075779451866));
#29594=CARTESIAN_POINT('Ctrl Pts',(43.7323453021837,39.1736218038991,49.9521389388692));
#29595=CARTESIAN_POINT('Ctrl Pts',(43.6669356338237,39.1693875531238,49.9967813885543));
#29596=CARTESIAN_POINT('Ctrl Pts',(43.5993550885029,39.1651533023485,50.0380814077597));
#29597=CARTESIAN_POINT('Ctrl Pts',(43.5299857685759,39.1609190515731,50.0758426249877));
#29598=CARTESIAN_POINT('Ctrl Pts',(43.4638257042102,39.1568806913278,50.111856882659));
#29599=CARTESIAN_POINT('Ctrl Pts',(43.3960390519226,39.1528423310825,50.1446524083331));
#29600=CARTESIAN_POINT('Ctrl Pts',(43.3269729073796,39.1488039708372,50.1741001977564));
#29601=CARTESIAN_POINT('Ctrl Pts',(43.2545351713106,39.144568470571,50.2049855354594));
#29602=CARTESIAN_POINT('Ctrl Pts',(43.180414480439,39.1403329703047,50.2323053412393));
#29603=CARTESIAN_POINT('Ctrl Pts',(43.1049960563844,39.1360974700385,50.2558747751997));
#29604=CARTESIAN_POINT('Ctrl Pts',(43.0296869651061,39.1318681099032,50.2794100409622));
#29605=CARTESIAN_POINT('Ctrl Pts',(42.9530843207721,39.1276387497679,50.2992055927087));
#29606=CARTESIAN_POINT('Ctrl Pts',(42.8755938411415,39.1234093896327,50.3151243895671));
#29607=CARTESIAN_POINT('Ctrl Pts',(42.7981938543251,39.1191849685132,50.3310245965712));
#29608=CARTESIAN_POINT('Ctrl Pts',(42.7199085499042,39.1149605473937,50.3430569512118));
#29609=CARTESIAN_POINT('Ctrl Pts',(42.6411578697656,39.1107361262742,50.3511344756841));
#29610=CARTESIAN_POINT('Ctrl Pts',(42.5624575491984,39.1065144065922,50.359206834732));
#29611=CARTESIAN_POINT('Ctrl Pts',(42.4832929092245,39.1022926869101,50.3633293354524));
#29612=CARTESIAN_POINT('Ctrl Pts',(42.4040919191154,39.0980709672281,50.3634664577899));
#29613=CARTESIAN_POINT('Ctrl Pts',(42.3249168432175,39.0938506288739,50.3636035352616));
#29614=CARTESIAN_POINT('Ctrl Pts',(42.2457059097968,39.0896302905198,50.3597578228464));
#29615=CARTESIAN_POINT('Ctrl Pts',(42.1668885158669,39.0854099521656,50.3519458915684));
#29616=CARTESIAN_POINT('Ctrl Pts',(42.0880722976202,39.0811896767643,50.3441340768174));
#29617=CARTESIAN_POINT('Ctrl Pts',(42.0096500741269,39.076969401363,50.3323562084255));
#29618=CARTESIAN_POINT('Ctrl Pts',(41.9320460432017,39.0727491259617,50.3166807149922));
#29619=CARTESIAN_POINT('Ctrl Pts',(41.8543643901669,39.0685246293019,50.3009895424137));
#29620=CARTESIAN_POINT('Ctrl Pts',(41.7775030256827,39.0643001326421,50.2813930501334));
#29621=CARTESIAN_POINT('Ctrl Pts',(41.701875273582,39.0600756359822,50.2580106968887));
#29622=CARTESIAN_POINT('Ctrl Pts',(41.6262112127954,39.0558491111526,50.2346171178374));
#29623=CARTESIAN_POINT('Ctrl Pts',(41.5517823857096,39.0516225863229,50.2074342182114));
#29624=CARTESIAN_POINT('Ctrl Pts',(41.4789838319879,39.0473960614933,50.1766303450886));
#29625=CARTESIAN_POINT('Ctrl Pts',(41.4060522049507,39.0431618107179,50.1457701635183));
#29626=CARTESIAN_POINT('Ctrl Pts',(41.3347572297971,39.0389275599426,50.1112759870524));
#29627=CARTESIAN_POINT('Ctrl Pts',(41.26547077459,39.0346933091672,50.0733629391861));
#29628=CARTESIAN_POINT('Ctrl Pts',(41.1993897413464,39.0306549489219,50.037203875067));
#29629=CARTESIAN_POINT('Ctrl Pts',(41.1351357818285,39.0266165886766,49.9979354982365));
#29630=CARTESIAN_POINT('Ctrl Pts',(41.0730051680361,39.0225782284313,49.9557799356883));
#29631=CARTESIAN_POINT('Ctrl Pts',(41.0081093410906,39.0183601351013,49.9117481786377));
#29632=CARTESIAN_POINT('Ctrl Pts',(40.9452791040872,39.0141420417714,49.8643957276567));
#29633=CARTESIAN_POINT('Ctrl Pts',(40.8848766116523,39.0099239484414,49.8139436482377));
#29634=CARTESIAN_POINT('Ctrl Pts',(40.8245618272495,39.0057119800353,49.7635648282558));
#29635=CARTESIAN_POINT('Ctrl Pts',(40.7666681488711,39.0015000116292,49.7100956167142));
#29636=CARTESIAN_POINT('Ctrl Pts',(40.7115287850674,38.9972880432231,49.6538002894074));
#29637=CARTESIAN_POINT('Ctrl Pts',(40.6564533472651,38.9930809579763,49.5975702282721));
#29638=CARTESIAN_POINT('Ctrl Pts',(40.6041262095551,38.9888738727295,49.5385208975658));
#29639=CARTESIAN_POINT('Ctrl Pts',(40.5548462813506,38.9846667874827,49.4769557188536));
#29640=CARTESIAN_POINT('Ctrl Pts',(40.5055972915353,38.9804623434824,49.415429191323));
#29641=CARTESIAN_POINT('Ctrl Pts',(40.4593920102545,38.9762578994822,49.3513903188447));
#29642=CARTESIAN_POINT('Ctrl Pts',(40.4164904665994,38.9720534554819,49.2851771752599));
#29643=CARTESIAN_POINT('Ctrl Pts',(40.3736021703791,38.9678503097589,49.2189844774265));
#29644=CARTESIAN_POINT('Ctrl Pts',(40.3340158437539,38.9636471640359,49.150619238736));
#29645=CARTESIAN_POINT('Ctrl Pts',(40.2979484921268,38.9594440183129,49.0804489340769));
#29646=CARTESIAN_POINT('Ctrl Pts',(40.2618807714525,38.9552408295826,49.0102779114236));
#29647=CARTESIAN_POINT('Ctrl Pts',(40.229332312171,38.9510376408523,48.9383022082623));
#29648=CARTESIAN_POINT('Ctrl Pts',(40.2004736799548,38.946834452122,48.8649129484107));
#29649=CARTESIAN_POINT('Ctrl Pts',(40.1715861759055,38.9426270582803,48.7914502657284));
#29650=CARTESIAN_POINT('Ctrl Pts',(40.146396043925,38.9384196644386,48.7165716442099));
#29651=CARTESIAN_POINT('Ctrl Pts',(40.1250250095019,38.9342122705969,48.6406865329537));
#29652=CARTESIAN_POINT('Ctrl Pts',(40.1036429612815,38.9300027084286,48.5647623134718));
#29653=CARTESIAN_POINT('Ctrl Pts',(40.0860840344984,38.9257931462603,48.487831033692));
#29654=CARTESIAN_POINT('Ctrl Pts',(40.0724189301043,38.9215835840919,48.4103130560477));
#29655=CARTESIAN_POINT('Ctrl Pts',(40.0587299728202,38.9173666739941,48.3326597682189));
#29656=CARTESIAN_POINT('Ctrl Pts',(40.0489484706961,38.9131497638963,48.2544182077444));
#29657=CARTESIAN_POINT('Ctrl Pts',(40.043093244688,38.9089328537985,48.1760141689309));
#29658=CARTESIAN_POINT('Ctrl Pts',(40.0387050852656,38.9057725191242,48.1172547937692));
#29659=CARTESIAN_POINT('Ctrl Pts',(40.0365210911557,38.90261218445,48.0584042686917));
#29660=CARTESIAN_POINT('Ctrl Pts',(40.0365300273278,38.8994518497758,47.9996405879596));
#29661=CARTESIAN_POINT('',(40.0365309862254,38.105701849771,48.0021591264912));
#29662=CARTESIAN_POINT('Ctrl Pts',(40.036530027328,38.8994518497283,47.9996405870764));
#29663=CARTESIAN_POINT('Ctrl Pts',(40.0365329485919,38.898418728494,47.9804305942669));
#29664=CARTESIAN_POINT('Ctrl Pts',(40.0367700699565,38.8973856072597,47.9612226144579));
#29665=CARTESIAN_POINT('Ctrl Pts',(40.0372412719132,38.8963524860254,47.9420204022983));
#29666=CARTESIAN_POINT('Ctrl Pts',(40.0391730645693,38.8921169857592,47.8632968488409));
#29667=CARTESIAN_POINT('Ctrl Pts',(40.045047261029,38.8878814854929,47.7845203141424));
#29668=CARTESIAN_POINT('Ctrl Pts',(40.0548723269245,38.8836459852267,47.7061179864713));
#29669=CARTESIAN_POINT('Ctrl Pts',(40.0646831495931,38.8794166250914,47.6278293172895));
#29670=CARTESIAN_POINT('Ctrl Pts',(40.0784334100136,38.8751872649562,47.5499142396325));
#29671=CARTESIAN_POINT('Ctrl Pts',(40.0960795788996,38.8709579048209,47.4727987726337));
#29672=CARTESIAN_POINT('Ctrl Pts',(40.1137051407189,38.8667334837014,47.395773360512));
#29673=CARTESIAN_POINT('Ctrl Pts',(40.1352174659245,38.8625090625819,47.319546158604));
#29674=CARTESIAN_POINT('Ctrl Pts',(40.1605215708118,38.8582846414625,47.2445353707149));
#29675=CARTESIAN_POINT('Ctrl Pts',(40.1858094942024,38.8540629217804,47.1695725508068));
#29676=CARTESIAN_POINT('Ctrl Pts',(40.2148842350025,38.8498412020984,47.0958250445317));
#29677=CARTESIAN_POINT('Ctrl Pts',(40.247600655478,38.8456194824164,47.0236970231525));
#29678=CARTESIAN_POINT('Ctrl Pts',(40.2803063712865,38.8413991440622,46.9515926017407));
#29679=CARTESIAN_POINT('Ctrl Pts',(40.316651207031,38.837178805708,46.8811070401549));
#29680=CARTESIAN_POINT('Ctrl Pts',(40.3564420312162,38.8329584673539,46.8126242089717));
#29681=CARTESIAN_POINT('Ctrl Pts',(40.3962322618597,38.8287381919526,46.7441423993157));
#29682=CARTESIAN_POINT('Ctrl Pts',(40.439468141818,38.8245179165513,46.677663665831));
#29683=CARTESIAN_POINT('Ctrl Pts',(40.4859115062213,38.82029764115,46.6135456448609));
#29684=CARTESIAN_POINT('Ctrl Pts',(40.5324013248086,38.8160731444902,46.5493634909329));
#29685=CARTESIAN_POINT('Ctrl Pts',(40.5821047607004,38.8118486478303,46.4875471474579));
#29686=CARTESIAN_POINT('Ctrl Pts',(40.6347417216878,38.8076241511705,46.4284231957203));
#29687=CARTESIAN_POINT('Ctrl Pts',(40.6874039535424,38.8033976263408,46.3692708587281));
#29688=CARTESIAN_POINT('Ctrl Pts',(40.7430021863726,38.7991711015112,46.312813823386));
#29689=CARTESIAN_POINT('Ctrl Pts',(40.8012194223008,38.7949445766815,46.2593417609215));
#29690=CARTESIAN_POINT('Ctrl Pts',(40.8595430773846,38.7907103259062,46.2057719533195));
#29691=CARTESIAN_POINT('Ctrl Pts',(40.9204949398595,38.7864760751308,46.1551983223142));
#29692=CARTESIAN_POINT('Ctrl Pts',(40.9837250545877,38.7822418243555,46.1078700573435));
#29693=CARTESIAN_POINT('Ctrl Pts',(41.0440299338148,38.7782034641102,46.0627313553918));
#29694=CARTESIAN_POINT('Ctrl Pts',(41.106406611522,38.7741651038649,46.0205445468993));
#29695=CARTESIAN_POINT('Ctrl Pts',(41.1705301059344,38.7701267436196,45.9814871264997));
#29696=CARTESIAN_POINT('Ctrl Pts',(41.2377839072695,38.7658912433533,45.9405230459192));
#29697=CARTESIAN_POINT('Ctrl Pts',(41.3072150742202,38.7616557430871,45.9028459751863));
#29698=CARTESIAN_POINT('Ctrl Pts',(41.378468909298,38.7574202428208,45.8686941393528));
#29699=CARTESIAN_POINT('Ctrl Pts',(41.4496194489317,38.7531908826856,45.8345918128411));
#29700=CARTESIAN_POINT('Ctrl Pts',(41.5225869899038,38.7489615225503,45.8040047738802));
#29701=CARTESIAN_POINT('Ctrl Pts',(41.596989689193,38.7447321624151,45.777126885844));
#29702=CARTESIAN_POINT('Ctrl Pts',(41.6713055015552,38.7405077412956,45.7502803856084));
#29703=CARTESIAN_POINT('Ctrl Pts',(41.7470527026375,38.7362833201761,45.7271345874006));
#29704=CARTESIAN_POINT('Ctrl Pts',(41.8238281859263,38.7320588990566,45.7078358519585));
#29705=CARTESIAN_POINT('Ctrl Pts',(41.9005545727447,38.7278371793746,45.6885494576929));
#29706=CARTESIAN_POINT('Ctrl Pts',(41.9783074826781,38.7236154596925,45.6731053574836));
#29707=CARTESIAN_POINT('Ctrl Pts',(42.0566684780718,38.7193937400105,45.661600139636));
#29708=CARTESIAN_POINT('Ctrl Pts',(42.1350038340967,38.7151734016563,45.6500986862444));
#29709=CARTESIAN_POINT('Ctrl Pts',(42.2139464164861,38.7109530633022,45.6425336242445));
#29710=CARTESIAN_POINT('Ctrl Pts',(42.2930688968157,38.706732724948,45.6389501953428));
#29711=CARTESIAN_POINT('Ctrl Pts',(42.3721901969113,38.7025124495467,45.6353668198935));
#29712=CARTESIAN_POINT('Ctrl Pts',(42.4514909206817,38.6982921741455,45.635764979386));
#29713=CARTESIAN_POINT('Ctrl Pts',(42.5305414407572,38.6940718987442,45.6401378486986));
#29714=CARTESIAN_POINT('Ctrl Pts',(42.6096710297683,38.6898474020843,45.6445150918991));
#29715=CARTESIAN_POINT('Ctrl Pts',(42.6885494454001,38.6856229054245,45.6528749607679));
#29716=CARTESIAN_POINT('Ctrl Pts',(42.7667504961249,38.6813984087646,45.6651585675913));
#29717=CARTESIAN_POINT('Ctrl Pts',(42.8449890909696,38.677171883935,45.6774480717423));
#29718=CARTESIAN_POINT('Ctrl Pts',(42.9225492130191,38.6729453591054,45.6936649703704));
#29719=CARTESIAN_POINT('Ctrl Pts',(42.9990157474873,38.6687188342757,45.7136993690325));
#29720=CARTESIAN_POINT('Ctrl Pts',(43.075622060217,38.6644845835004,45.7337703899037));
#29721=CARTESIAN_POINT('Ctrl Pts',(43.1511303421672,38.660250332725,45.7576727129945));
#29722=CARTESIAN_POINT('Ctrl Pts',(43.2251416952759,38.6560160819497,45.7852468255769));
#29723=CARTESIAN_POINT('Ctrl Pts',(43.2957290369222,38.6519777217044,45.8115452679603));
#29724=CARTESIAN_POINT('Ctrl Pts',(43.3649545786653,38.6479393614591,45.8411831002522));
#29725=CARTESIAN_POINT('Ctrl Pts',(43.4324932301622,38.6439010012138,45.8739830267448));
#29726=CARTESIAN_POINT('Ctrl Pts',(43.5033289057883,38.6396655009475,45.9083841422852));
#29727=CARTESIAN_POINT('Ctrl Pts',(43.5725780501447,38.6354300006813,45.9463947277719));
#29728=CARTESIAN_POINT('Ctrl Pts',(43.6398484209544,38.631194500415,45.9878453503876));
#29729=CARTESIAN_POINT('Ctrl Pts',(43.7070212710787,38.6269651402798,46.0292358827573));
#29730=CARTESIAN_POINT('Ctrl Pts',(43.7722206479711,38.6227357801445,46.0740563048966));
#29731=CARTESIAN_POINT('Ctrl Pts',(43.8350769332684,38.6185064200093,46.1220903545429));
#29732=CARTESIAN_POINT('Ctrl Pts',(43.8978598154564,38.6142819988898,46.170068310378));
#29733=CARTESIAN_POINT('Ctrl Pts',(43.9583046724889,38.6100575777703,46.2212521526019));
#29734=CARTESIAN_POINT('Ctrl Pts',(44.0160703336841,38.6058331566508,46.2753820372366));
#29735=CARTESIAN_POINT('Ctrl Pts',(44.0737990548309,38.6016114369688,46.3294773068332));
#29736=CARTESIAN_POINT('Ctrl Pts',(44.1288516391055,38.5973897172867,46.386514559564));
#29737=CARTESIAN_POINT('Ctrl Pts',(44.1809204818222,38.5931679976047,46.4461941310684));
#29738=CARTESIAN_POINT('Ctrl Pts',(44.2329722878454,38.5889476592505,46.5058541756828));
#29739=CARTESIAN_POINT('Ctrl Pts',(44.2820419825228,38.5847273208964,46.5681544689535));
#29740=CARTESIAN_POINT('Ctrl Pts',(44.3278603352689,38.5805069825422,46.6327600910605));
#29741=CARTESIAN_POINT('Ctrl Pts',(44.3736780045635,38.5762867071409,46.6973647494748));
#29742=CARTESIAN_POINT('Ctrl Pts',(44.4162441579054,38.5720664317396,46.7642742847531));
#29743=CARTESIAN_POINT('Ctrl Pts',(44.4553321106632,38.5678461563383,46.8331236758864));
#29744=CARTESIAN_POINT('Ctrl Pts',(44.4944591604796,38.5636216596785,46.90204193245));
#29745=CARTESIAN_POINT('Ctrl Pts',(44.5301008276703,38.5593971630187,46.9729035117433));
#29746=CARTESIAN_POINT('Ctrl Pts',(44.5620760724659,38.5551726663588,47.045318116978));
#29747=CARTESIAN_POINT('Ctrl Pts',(44.5940666684929,38.5509461415292,47.1177674882754));
#29748=CARTESIAN_POINT('Ctrl Pts',(44.6223871675287,38.5467196166995,47.1917709318967));
#29749=CARTESIAN_POINT('Ctrl Pts',(44.646905420318,38.5424930918699,47.2669198726976));
#29750=CARTESIAN_POINT('Ctrl Pts',(44.6714684916514,38.5382588410945,47.3422061832428));
#29751=CARTESIAN_POINT('Ctrl Pts',(44.6922153049804,38.5340245903192,47.4186417209783));
#29752=CARTESIAN_POINT('Ctrl Pts',(44.7090642145296,38.5297903395438,47.4958047064096));
#29753=CARTESIAN_POINT('Ctrl Pts',(44.7251336374596,38.5257519792985,47.5693978753808));
#29754=CARTESIAN_POINT('Ctrl Pts',(44.737657817594,38.5217136190532,47.6436523139323));
#29755=CARTESIAN_POINT('Ctrl Pts',(44.7466099944902,38.5176752588079,47.7181986964925));
#29756=CARTESIAN_POINT('Ctrl Pts',(44.7559991884512,38.5134397585416,47.7963841985283));
#29757=CARTESIAN_POINT('Ctrl Pts',(44.7614944169681,38.5092042582754,47.8751880757596));
#29758=CARTESIAN_POINT('Ctrl Pts',(44.7630259780619,38.5049687580091,47.9541887797103));
#29759=CARTESIAN_POINT('Ctrl Pts',(44.7645553188783,38.5007393978739,48.0330749577161));
#29760=CARTESIAN_POINT('Ctrl Pts',(44.7621323939109,38.4965100377386,48.1121569305197));
#29761=CARTESIAN_POINT('Ctrl Pts',(44.7557391254035,38.4922806776033,48.1910068426604));
#29762=CARTESIAN_POINT('Ctrl Pts',(44.7493533229083,38.4880562564838,48.2697646744515));
#29763=CARTESIAN_POINT('Ctrl Pts',(44.7390064282714,38.4838318353643,48.3482905187185));
#29764=CARTESIAN_POINT('Ctrl Pts',(44.7247324071361,38.4796074142449,48.426156867962));
#29765=CARTESIAN_POINT('Ctrl Pts',(44.7104675139676,38.4753856945628,48.503973423147));
#29766=CARTESIAN_POINT('Ctrl Pts',(44.6922805631403,38.4711639748808,48.58113085995));
#29767=CARTESIAN_POINT('Ctrl Pts',(44.6702571692749,38.4669422551988,48.6572083583279));
#29768=CARTESIAN_POINT('Ctrl Pts',(44.6482409813659,38.4627219168446,48.7332609644872));
#29769=CARTESIAN_POINT('Ctrl Pts',(44.6223909733764,38.4585015784904,48.80823388336));
#29770=CARTESIAN_POINT('Ctrl Pts',(44.5928431708198,38.4542812401363,48.8817194956952));
#29771=CARTESIAN_POINT('Ctrl Pts',(44.5632958090143,38.450060964735,48.9552040118788));
#29772=CARTESIAN_POINT('Ctrl Pts',(44.530050938619,38.4458406893337,49.027200830655));
#29773=CARTESIAN_POINT('Ctrl Pts',(44.4932929180909,38.4416204139324,49.097321830627));
#29774=CARTESIAN_POINT('Ctrl Pts',(44.456498130979,38.4373959172726,49.1675129679343));
#29775=CARTESIAN_POINT('Ctrl Pts',(44.4161833925721,38.4331714206127,49.2358241216887));
#29776=CARTESIAN_POINT('Ctrl Pts',(44.3725790124487,38.4289469239529,49.3018918851222));
#29777=CARTESIAN_POINT('Ctrl Pts',(44.3289536979764,38.4247203991233,49.3679913675161));
#29778=CARTESIAN_POINT('Ctrl Pts',(44.2820358738255,38.4204938742936,49.4318449352347));
#29779=CARTESIAN_POINT('Ctrl Pts',(44.2320976715372,38.416267349464,49.4931204113694));
#29780=CARTESIAN_POINT('Ctrl Pts',(44.1820681838893,38.4120330986886,49.5545078970203));
#29781=CARTESIAN_POINT('Ctrl Pts',(44.1290076008186,38.4077988479133,49.6133075247097));
#29782=CARTESIAN_POINT('Ctrl Pts',(44.0732264810481,38.403564597138,49.6692224489323));
#29783=CARTESIAN_POINT('Ctrl Pts',(44.0200259814856,38.3995262368926,49.7225505627076));
#29784=CARTESIAN_POINT('Ctrl Pts',(43.9643513894669,38.3954878766473,49.7732547690044));
#29785=CARTESIAN_POINT('Ctrl Pts',(43.9064988409918,38.391449516402,49.8211127595485));
#29786=CARTESIAN_POINT('Ctrl Pts',(43.8458221134131,38.3872140161358,49.8713070263742));
#29787=CARTESIAN_POINT('Ctrl Pts',(43.7825187127748,38.3829785158695,49.9185608946895));
#29788=CARTESIAN_POINT('Ctrl Pts',(43.7169054649991,38.3787430156033,49.9625876890359));
#29789=CARTESIAN_POINT('Ctrl Pts',(43.6513873356063,38.374513655468,50.0065506585052));
#29790=CARTESIAN_POINT('Ctrl Pts',(43.583566395141,38.3702842953327,50.0472955848435));
#29791=CARTESIAN_POINT('Ctrl Pts',(43.5137927021419,38.3660549351975,50.0845757979876));
#29792=CARTESIAN_POINT('Ctrl Pts',(43.4441004903501,38.361830514078,50.1218124755719));
#29793=CARTESIAN_POINT('Ctrl Pts',(43.3724604694405,38.3576060929585,50.1555922602152));
#29794=CARTESIAN_POINT('Ctrl Pts',(43.2992505603425,38.353381671839,50.1857124400579));
#29795=CARTESIAN_POINT('Ctrl Pts',(43.2260874675976,38.349159952157,50.2158133586149));
#29796=CARTESIAN_POINT('Ctrl Pts',(43.1513569120975,38.344938232475,50.2422591391675));
#29797=CARTESIAN_POINT('Ctrl Pts',(43.0754591320902,38.3407165127929,50.2648941259529));
#29798=CARTESIAN_POINT('Ctrl Pts',(42.9995861854986,38.3364961744388,50.2875217066714));
#29799=CARTESIAN_POINT('Ctrl Pts',(42.9225472221832,38.3322758360846,50.3063408354675));
#29800=CARTESIAN_POINT('Ctrl Pts',(42.8447586500196,38.3280554977305,50.3212453950698));
#29801=CARTESIAN_POINT('Ctrl Pts',(42.7669712381927,38.3238352223292,50.3361497323476));
#29802=CARTESIAN_POINT('Ctrl Pts',(42.6884347009615,38.3196149469279,50.3471395294893));
#29803=CARTESIAN_POINT('Ctrl Pts',(42.60957519567,38.3153946715266,50.3541598667592));
#29804=CARTESIAN_POINT('Ctrl Pts',(42.5306368125019,38.3111701748668,50.3611872260019));
#29805=CARTESIAN_POINT('Ctrl Pts',(42.4513752845733,38.3069456782069,50.3642371523107));
#29806=CARTESIAN_POINT('Ctrl Pts',(42.3722208426973,38.3027211815471,50.3633067425367));
#29807=CARTESIAN_POINT('Ctrl Pts',(42.2930283989807,38.2984946567174,50.3623758860755));
#29808=CARTESIAN_POINT('Ctrl Pts',(42.2139436128266,38.2942681318878,50.3574609158405));
#29809=CARTESIAN_POINT('Ctrl Pts',(42.1353930751858,38.2900416070581,50.3486109972152));
#29810=CARTESIAN_POINT('Ctrl Pts',(42.0566989497956,38.2858073562828,50.3397449012355));
#29811=CARTESIAN_POINT('Ctrl Pts',(41.9785414887562,38.2815731055075,50.3269295598006));
#29812=CARTESIAN_POINT('Ctrl Pts',(41.9013383570951,38.2773388547321,50.3102655706207));
#29813=CARTESIAN_POINT('Ctrl Pts',(41.8277068991924,38.2733004944868,50.2943725130285));
#29814=CARTESIAN_POINT('Ctrl Pts',(41.7549437581605,38.2692621342415,50.2749791626272));
#29815=CARTESIAN_POINT('Ctrl Pts',(41.6833961085529,38.2652237739962,50.2522143112197));
#29816=CARTESIAN_POINT('Ctrl Pts',(41.6083557281623,38.2609882737299,50.2283381515063));
#29817=CARTESIAN_POINT('Ctrl Pts',(41.5343672976752,38.2567527734637,50.2006621554591));
#29818=CARTESIAN_POINT('Ctrl Pts',(41.4618433193258,38.2525172731974,50.169297693588));
#29819=CARTESIAN_POINT('Ctrl Pts',(41.389424477725,38.2482879130622,50.1379787002312));
#29820=CARTESIAN_POINT('Ctrl Pts',(41.3184662995248,38.2440585529269,50.1029820441847));
#29821=CARTESIAN_POINT('Ctrl Pts',(41.2493656198619,38.2398291927916,50.0644686880997));
#29822=CARTESIAN_POINT('Ctrl Pts',(41.1803456354663,38.2356047716721,50.0260003076297));
#29823=CARTESIAN_POINT('Ctrl Pts',(41.1131792469015,38.2313803505526,49.9840236153632));
#29824=CARTESIAN_POINT('Ctrl Pts',(41.0482413925371,38.2271559294332,49.938746788018));
#29825=CARTESIAN_POINT('Ctrl Pts',(40.9833450647032,38.2229342097511,49.893498914348));
#29826=CARTESIAN_POINT('Ctrl Pts',(40.9206748265075,38.2187124900691,49.8449553619555));
#29827=CARTESIAN_POINT('Ctrl Pts',(40.8605781143012,38.214490770387,49.7933685339973));
#29828=CARTESIAN_POINT('Ctrl Pts',(40.8005010654714,38.2102704320329,49.7417985850194));
#29829=CARTESIAN_POINT('Ctrl Pts',(40.7429962264743,38.2060500936787,49.6871876431736));
#29830=CARTESIAN_POINT('Ctrl Pts',(40.6883781180301,38.2018297553246,49.6298285106298));
#29831=CARTESIAN_POINT('Ctrl Pts',(40.6337608242993,38.1976094799233,49.5724702336861));
#29832=CARTESIAN_POINT('Ctrl Pts',(40.5820304982221,38.193389204522,49.5123641883541));
#29833=CARTESIAN_POINT('Ctrl Pts',(40.533463876334,38.1891689291207,49.4498390738112));
#29834=CARTESIAN_POINT('Ctrl Pts',(40.4848486765098,38.1849444324608,49.3872514195879));
#29835=CARTESIAN_POINT('Ctrl Pts',(40.4394037908502,38.180719935801,49.3222402341853));
#29836=CARTESIAN_POINT('Ctrl Pts',(40.3973644121932,38.1764954391412,49.2551657832133));
#29837=CARTESIAN_POINT('Ctrl Pts',(40.3553048505404,38.1722689143115,49.1880591299729));
#29838=CARTESIAN_POINT('Ctrl Pts',(40.3166542822164,38.1680423894819,49.1188876481202));
#29839=CARTESIAN_POINT('Ctrl Pts',(40.2816021398275,38.1638158646522,49.0480367106721));
#29840=CARTESIAN_POINT('Ctrl Pts',(40.2464859232974,38.1595816138769,48.9770562600856));
#29841=CARTESIAN_POINT('Ctrl Pts',(40.2149814638827,38.1553473631015,48.9043906511003));
#29842=CARTESIAN_POINT('Ctrl Pts',(40.1872301093111,38.1511131123262,48.8304455742315));
#29843=CARTESIAN_POINT('Ctrl Pts',(40.1607626247427,38.1470747520809,48.7599214426659));
#29844=CARTESIAN_POINT('Ctrl Pts',(40.1377087367046,38.1430363918356,48.6882339613397));
#29845=CARTESIAN_POINT('Ctrl Pts',(40.1181479461546,38.1389980315903,48.6157447890655));
#29846=CARTESIAN_POINT('Ctrl Pts',(40.091268239247,38.1334486679537,48.516132879224));
#29847=CARTESIAN_POINT('Ctrl Pts',(40.0708982267616,38.1278993043172,48.4146948253093));
#29848=CARTESIAN_POINT('Ctrl Pts',(40.0572375947585,38.1223499406806,48.3121774391067));
#29849=CARTESIAN_POINT('Ctrl Pts',(40.0435769627555,38.1168005770441,48.2096600529041));
#29850=CARTESIAN_POINT('Ctrl Pts',(40.0366259066926,38.1112512134075,48.1060629894526));
#29851=CARTESIAN_POINT('Ctrl Pts',(40.0365309862254,38.105701849771,48.0021591264911));
#29852=CARTESIAN_POINT('',(40.036530095277,37.3119518496952,47.9993289049744));
#29853=CARTESIAN_POINT('Ctrl Pts',(40.0365309862246,38.1057018497283,48.0021591256915));
#29854=CARTESIAN_POINT('Ctrl Pts',(40.0364594804506,38.1015213847461,47.923885923739));
#29855=CARTESIAN_POINT('Ctrl Pts',(40.0402806015298,38.0973409197639,47.8455205042509));
#29856=CARTESIAN_POINT('Ctrl Pts',(40.0479951025618,38.0931604547817,47.7674846170108));
#29857=CARTESIAN_POINT('Ctrl Pts',(40.0557053122759,38.0889823152518,47.6894921385139));
#29858=CARTESIAN_POINT('Ctrl Pts',(40.0673045584702,38.0848041757218,47.6118293051813));
#29859=CARTESIAN_POINT('Ctrl Pts',(40.0827415695637,38.0806260361919,47.5349152685025));
#29860=CARTESIAN_POINT('Ctrl Pts',(40.09817505423,38.0764488511152,47.4580188020482));
#29861=CARTESIAN_POINT('Ctrl Pts',(40.1174444687557,38.0722716660385,47.3818712629778));
#29862=CARTESIAN_POINT('Ctrl Pts',(40.14044727168,38.0680944809618,47.3068824711193));
#29863=CARTESIAN_POINT('Ctrl Pts',(40.163452360777,38.0639168807284,47.2318862263725));
#29864=CARTESIAN_POINT('Ctrl Pts',(40.1901914315531,38.0597392804951,47.1580494154471));
#29865=CARTESIAN_POINT('Ctrl Pts',(40.2205123195484,38.0555616802617,47.0857659535656));
#29866=CARTESIAN_POINT('Ctrl Pts',(40.2508654090067,38.0513796433233,47.0134057250268));
#29867=CARTESIAN_POINT('Ctrl Pts',(40.2848077193831,38.0471976063848,46.9426025802068));
#29868=CARTESIAN_POINT('Ctrl Pts',(40.3221395781701,38.0430155694463,46.8737289365819));
#29869=CARTESIAN_POINT('Ctrl Pts',(40.3594942267784,38.0388309795175,46.8048132479564));
#29870=CARTESIAN_POINT('Ctrl Pts',(40.4002422894582,38.0346463895887,46.7378298124712));
#29871=CARTESIAN_POINT('Ctrl Pts',(40.4441403040548,38.0304617996599,46.6731227296102));
#29872=CARTESIAN_POINT('Ctrl Pts',(40.488111138022,38.0262702682053,46.608308308659));
#29873=CARTESIAN_POINT('Ctrl Pts',(40.5352420593665,38.0220787367506,46.5457781553767));
#29874=CARTESIAN_POINT('Ctrl Pts',(40.5852493227092,38.0178872052959,46.4858433303741));
#29875=CARTESIAN_POINT('Ctrl Pts',(40.605590571862,38.0161822332588,46.4614638877329));
#29876=CARTESIAN_POINT('Ctrl Pts',(40.626407314884,38.0144772612217,46.4375134349776));
#29877=CARTESIAN_POINT('Ctrl Pts',(40.6476788097917,38.0127722891846,46.4140110696329));
#29878=CARTESIAN_POINT('Ctrl Pts',(40.7005215663789,38.0085367889183,46.3556263732812));
#29879=CARTESIAN_POINT('Ctrl Pts',(40.7563858928542,38.0043012886521,46.2997745547736));
#29880=CARTESIAN_POINT('Ctrl Pts',(40.8149993977995,38.0000657883858,46.2467848015933));
#29881=CARTESIAN_POINT('Ctrl Pts',(40.8735279317674,37.9958364282506,46.1938718667355));
#29882=CARTESIAN_POINT('Ctrl Pts',(40.9347973846144,37.9916070681153,46.1438130699485));
#29883=CARTESIAN_POINT('Ctrl Pts',(40.9984967336247,37.98737770798,46.0969027783008));
#29884=CARTESIAN_POINT('Ctrl Pts',(41.062121695002,37.9831532868605,46.0500472681478));
#29885=CARTESIAN_POINT('Ctrl Pts',(41.1281705377089,37.9789288657411,46.0063332335187));
#29886=CARTESIAN_POINT('Ctrl Pts',(41.1962983549,37.9747044446216,45.9660155382886));
#29887=CARTESIAN_POINT('Ctrl Pts',(41.2643826056398,37.9704827249395,45.9257236254625));
#29888=CARTESIAN_POINT('Ctrl Pts',(41.334542789331,37.9662610052575,45.8888239796809));
#29889=CARTESIAN_POINT('Ctrl Pts',(41.406405157928,37.9620392855754,45.8555280998092));
#29890=CARTESIAN_POINT('Ctrl Pts',(41.478244013478,37.9578189472213,45.8222431142011));
#29891=CARTESIAN_POINT('Ctrl Pts',(41.5517835224818,37.9535986088671,45.7925597502938));
#29892=CARTESIAN_POINT('Ctrl Pts',(41.6266268233561,37.949378270513,45.7666428027412));
#29893=CARTESIAN_POINT('Ctrl Pts',(41.7014690078267,37.9451579951117,45.7407262417799));
#29894=CARTESIAN_POINT('Ctrl Pts',(41.77761450156,37.9409377197104,45.7185761378162));
#29895=CARTESIAN_POINT('Ctrl Pts',(41.8546494449382,37.9367174443091,45.7003080178003));
#29896=CARTESIAN_POINT('Ctrl Pts',(41.931761441206,37.9324929476493,45.6820216254086));
#29897=CARTESIAN_POINT('Ctrl Pts',(42.0097642065436,37.9282684509894,45.6676250820813));
#29898=CARTESIAN_POINT('Ctrl Pts',(42.088232382933,37.9240439543296,45.657183021692));
#29899=CARTESIAN_POINT('Ctrl Pts',(42.1667382316886,37.9198174294999,45.6467359480968));
#29900=CARTESIAN_POINT('Ctrl Pts',(42.2457094682034,37.9155909046703,45.6402471780457));
#29901=CARTESIAN_POINT('Ctrl Pts',(42.3247168620443,37.9113643798406,45.6377292936584));
#29902=CARTESIAN_POINT('Ctrl Pts',(42.4038686787525,37.9071301290653,45.6352068066629));
#29903=CARTESIAN_POINT('Ctrl Pts',(42.4830563143533,37.9028958782899,45.6366697011167));
#29904=CARTESIAN_POINT('Ctrl Pts',(42.5618519886392,37.8986616275146,45.6420783781742));
#29905=CARTESIAN_POINT('Ctrl Pts',(42.6370023128456,37.8946232672693,45.647236831834));
#29906=CARTESIAN_POINT('Ctrl Pts',(42.7117957900945,37.890584907024,45.6559839738596));
#29907=CARTESIAN_POINT('Ctrl Pts',(42.7858703532216,37.8865465467787,45.66824218423));
#29908=CARTESIAN_POINT('Ctrl Pts',(42.8635610030867,37.8823110465124,45.6810988018009));
#29909=CARTESIAN_POINT('Ctrl Pts',(42.9407560751894,37.8780755462462,45.6978669098096));
#29910=CARTESIAN_POINT('Ctrl Pts',(43.0170313521786,37.8738400459799,45.7184955070549));
#29911=CARTESIAN_POINT('Ctrl Pts',(43.0931960542268,37.8696106858446,45.739094199382));
#29912=CARTESIAN_POINT('Ctrl Pts',(43.1684431598382,37.8653813257094,45.7635421458197));
#29913=CARTESIAN_POINT('Ctrl Pts',(43.2423568374042,37.8611519655741,45.7917370176135));
#29914=CARTESIAN_POINT('Ctrl Pts',(43.3161841991192,37.8569275444546,45.8198989636427));
#29915=CARTESIAN_POINT('Ctrl Pts',(43.3886807909189,37.8527031233351,45.8517989734217));
#29916=CARTESIAN_POINT('Ctrl Pts',(43.459445673463,37.8484787022157,45.887284849801));
#29917=CARTESIAN_POINT('Ctrl Pts',(43.5301653032023,37.8442569825336,45.922748033633));
#29918=CARTESIAN_POINT('Ctrl Pts',(43.5991550032072,37.8400352628516,45.9617923229416));
#29919=CARTESIAN_POINT('Ctrl Pts',(43.6660347024841,37.8358135431696,46.0042178042166));
#29920=CARTESIAN_POINT('Ctrl Pts',(43.7328925190213,37.8315932048154,46.0466294040632));
#29921=CARTESIAN_POINT('Ctrl Pts',(43.797641309668,37.8273728664612,46.0924197478833));
#29922=CARTESIAN_POINT('Ctrl Pts',(43.8599277787561,37.8231525281071,46.1413442164521));
#29923=CARTESIAN_POINT('Ctrl Pts',(43.9222133187453,37.8189322527058,46.1902679552368));
#29924=CARTESIAN_POINT('Ctrl Pts',(43.9820362419074,37.8147119773045,46.2423254348709));
#29925=CARTESIAN_POINT('Ctrl Pts',(44.0390754923038,37.8104917019032,46.2972310868972));
#29926=CARTESIAN_POINT('Ctrl Pts',(44.0961717952384,37.8062672052434,46.3521916573664));
#29927=CARTESIAN_POINT('Ctrl Pts',(44.1504785244211,37.8020427085835,46.4100057648622));
#29928=CARTESIAN_POINT('Ctrl Pts',(44.2017112058828,37.7978182119237,46.4703506377289));
#29929=CARTESIAN_POINT('Ctrl Pts',(44.2529684840208,37.7935916870941,46.5307244820112));
#29930=CARTESIAN_POINT('Ctrl Pts',(44.3011484885996,37.7893651622644,46.5936311389899));
#29931=CARTESIAN_POINT('Ctrl Pts',(44.3460084276921,37.7851386374348,46.6587164206436));
#29932=CARTESIAN_POINT('Ctrl Pts',(44.3909503692494,37.7809043866594,46.7239206760101));
#29933=CARTESIAN_POINT('Ctrl Pts',(44.4325598708682,37.7766701358841,46.7913111135161));
#29934=CARTESIAN_POINT('Ctrl Pts',(44.4706388108378,37.7724358851088,46.8605065353622));
#29935=CARTESIAN_POINT('Ctrl Pts',(44.5069560923395,37.7683975248634,46.9265007467512));
#29936=CARTESIAN_POINT('Ctrl Pts',(44.540062135037,37.7643591646181,46.9941362896968));
#29937=CARTESIAN_POINT('Ctrl Pts',(44.5698263442917,37.7603208043728,47.0630666637813));
#29938=CARTESIAN_POINT('Ctrl Pts',(44.601043548445,37.7560853041066,47.1353620015057));
#29939=CARTESIAN_POINT('Ctrl Pts',(44.628702976007,37.7518498038403,47.2093566274597));
#29940=CARTESIAN_POINT('Ctrl Pts',(44.6526180224422,37.7476143035741,47.2846661717293));
#29941=CARTESIAN_POINT('Ctrl Pts',(44.6764983996511,37.7433849434388,47.3598665410639));
#29942=CARTESIAN_POINT('Ctrl Pts',(44.6966450342552,37.7391555833035,47.4363775997551));
#29943=CARTESIAN_POINT('Ctrl Pts',(44.7129190262478,37.7349262231683,47.513794262764));
#29944=CARTESIAN_POINT('Ctrl Pts',(44.7291740135917,37.7307018020488,47.5911205191612));
#29945=CARTESIAN_POINT('Ctrl Pts',(44.7415652492095,37.7264773809293,47.6693498213845));
#29946=CARTESIAN_POINT('Ctrl Pts',(44.7500038304048,37.7222529598098,47.7480626308332));
#29947=CARTESIAN_POINT('Ctrl Pts',(44.758437015287,37.7180312401278,47.826725104928));
#29948=CARTESIAN_POINT('Ctrl Pts',(44.7629225126911,37.7138095204457,47.9058700071481));
#29949=CARTESIAN_POINT('Ctrl Pts',(44.7634228403172,37.7095878007637,47.985069535613));
#29950=CARTESIAN_POINT('Ctrl Pts',(44.7639230042384,37.7053674624096,48.0642431503449));
#29951=CARTESIAN_POINT('Ctrl Pts',(44.760440584591,37.7011471240554,48.1434708868438));
#29952=CARTESIAN_POINT('Ctrl Pts',(44.7529901830593,37.6969267857013,48.2223232766187));
#29953=CARTESIAN_POINT('Ctrl Pts',(44.7455398926619,37.6927065103,48.3011744901884));
#29954=CARTESIAN_POINT('Ctrl Pts',(44.7341217835124,37.6884862348987,48.3796499010185));
#29955=CARTESIAN_POINT('Ctrl Pts',(44.7188023381678,37.6842659594974,48.457325001949));
#29956=CARTESIAN_POINT('Ctrl Pts',(44.7034675698091,37.6800414628376,48.5350777960756));
#29957=CARTESIAN_POINT('Ctrl Pts',(44.6842237610639,37.6758169661777,48.612028219629));
#29958=CARTESIAN_POINT('Ctrl Pts',(44.6611884739575,37.6715924695179,48.6877624052983));
#29959=CARTESIAN_POINT('Ctrl Pts',(44.6381421276701,37.6673659446882,48.7635329507519));
#29960=CARTESIAN_POINT('Ctrl Pts',(44.6113008360124,37.6631394198586,48.8380856528865));
#29961=CARTESIAN_POINT('Ctrl Pts',(44.580831132685,37.6589128950289,48.9110247041722));
#29962=CARTESIAN_POINT('Ctrl Pts',(44.5503057317613,37.6546786442536,48.9840970855984));
#29963=CARTESIAN_POINT('Ctrl Pts',(44.516138868655,37.6504443934783,49.0555494974379));
#29964=CARTESIAN_POINT('Ctrl Pts',(44.4785439592545,37.6462101427029,49.1250090890062));
#29965=CARTESIAN_POINT('Ctrl Pts',(44.4426883154572,37.6421717824576,49.191255248747));
#29966=CARTESIAN_POINT('Ctrl Pts',(44.4037150128913,37.6381334222123,49.2556886129284));
#29967=CARTESIAN_POINT('Ctrl Pts',(44.3618448175453,37.634095061967,49.3180118940172));
#29968=CARTESIAN_POINT('Ctrl Pts',(44.3179306512096,37.6298595617007,49.3833776012869));
#29969=CARTESIAN_POINT('Ctrl Pts',(44.2706626089232,37.6256240614345,49.4466704190592));
#29970=CARTESIAN_POINT('Ctrl Pts',(44.2202630051063,37.6213885611682,49.5075254668301));
#29971=CARTESIAN_POINT('Ctrl Pts',(44.1699364647174,37.6171592010329,49.568292294098));
#29972=CARTESIAN_POINT('Ctrl Pts',(44.1164876748209,37.6129298408977,49.6266280108294));
#29973=CARTESIAN_POINT('Ctrl Pts',(44.0601821795825,37.6087004807624,49.6821966506615));
#29974=CARTESIAN_POINT('Ctrl Pts',(44.0039424374888,37.6044760596429,49.7377003978432));
#29975=CARTESIAN_POINT('Ctrl Pts',(43.9448529517098,37.6002516385234,49.7904431614876));
#29976=CARTESIAN_POINT('Ctrl Pts',(43.8832184703814,37.5960272174039,49.8401232051196));
#29977=CARTESIAN_POINT('Ctrl Pts',(43.8216234031389,37.5918054977219,49.8897714793027));
#29978=CARTESIAN_POINT('Ctrl Pts',(43.7574869349752,37.5875837780398,49.9363606270291));
#29979=CARTESIAN_POINT('Ctrl Pts',(43.6911485816734,37.5833620583578,49.9796276874561));
#29980=CARTESIAN_POINT('Ctrl Pts',(43.6248319339853,37.5791417200037,50.0228805910937));
#29981=CARTESIAN_POINT('Ctrl Pts',(43.5563152245564,37.5749213816495,50.0628133095885));
#29982=CARTESIAN_POINT('Ctrl Pts',(43.4859675478282,37.5707010432953,50.0992057845681));
#29983=CARTESIAN_POINT('Ctrl Pts',(43.4156209204442,37.566480767894,50.1355977166977));
#29984=CARTESIAN_POINT('Ctrl Pts',(43.343443797536,37.5622604924928,50.1684492958105));
#29985=CARTESIAN_POINT('Ctrl Pts',(43.2698291680371,37.5580402170915,50.1975867808421));
#29986=CARTESIAN_POINT('Ctrl Pts',(43.1961409067595,37.5538157204316,50.2267534101466));
#29987=CARTESIAN_POINT('Ctrl Pts',(43.1210127040735,37.5495912237718,50.2521983511218));
#29988=CARTESIAN_POINT('Ctrl Pts',(43.0448562340585,37.5453667271119,50.2737965780377));
#29989=CARTESIAN_POINT('Ctrl Pts',(42.9686632015215,37.5411402022823,50.2954051742058));
#29990=CARTESIAN_POINT('Ctrl Pts',(42.8914413762488,37.5369136774526,50.3131632719361));
#29991=CARTESIAN_POINT('Ctrl Pts',(42.8136137367968,37.532687152623,50.3269968022395));
#29992=CARTESIAN_POINT('Ctrl Pts',(42.735643831029,37.5284529018477,50.3408556197726));
#29993=CARTESIAN_POINT('Ctrl Pts',(42.6570663651013,37.5242186510723,50.3507754756478));
#29994=CARTESIAN_POINT('Ctrl Pts',(42.5783103730831,37.519984400297,50.3567341495703));
#29995=CARTESIAN_POINT('Ctrl Pts',(42.5031978953109,37.5159460400517,50.3624171554101));
#29996=CARTESIAN_POINT('Ctrl Pts',(42.4279234026227,37.5119076798064,50.3644974157545));
#29997=CARTESIAN_POINT('Ctrl Pts',(42.3528563546987,37.5078693195611,50.3629997709707));
#29998=CARTESIAN_POINT('Ctrl Pts',(42.2741247700564,37.5036338192948,50.3614290158881));
#29999=CARTESIAN_POINT('Ctrl Pts',(42.1953221253149,37.4993983190286,50.3559161414232));
#30000=CARTESIAN_POINT('Ctrl Pts',(42.1168755654281,37.4951628187624,50.346450722996));
#30001=CARTESIAN_POINT('Ctrl Pts',(42.0385427281531,37.4909334586271,50.336999026421));
#30002=CARTESIAN_POINT('Ctrl Pts',(41.9605654126611,37.4867040984918,50.3236062202699));
#30003=CARTESIAN_POINT('Ctrl Pts',(41.8833698332261,37.4824747383566,50.3063138796962));
#30004=CARTESIAN_POINT('Ctrl Pts',(41.8062644022232,37.4782503172371,50.289041732991));
#30005=CARTESIAN_POINT('Ctrl Pts',(41.7299393487857,37.4740258961176,50.2678792032686));
#30006=CARTESIAN_POINT('Ctrl Pts',(41.6548133079061,37.4698014749981,50.2429193553996));
#30007=CARTESIAN_POINT('Ctrl Pts',(41.5797353087096,37.4655797553161,50.2179754688815));
#30008=CARTESIAN_POINT('Ctrl Pts',(41.5058552444528,37.461358035634,50.189239231483));
#30009=CARTESIAN_POINT('Ctrl Pts',(41.4335779477341,37.457136315952,50.1568539259287));
#30010=CARTESIAN_POINT('Ctrl Pts',(41.361324299825,37.4529159775978,50.1244792167022));
#30011=CARTESIAN_POINT('Ctrl Pts',(41.2906728061292,37.4486956392437,50.0884580018988));
#30012=CARTESIAN_POINT('Ctrl Pts',(41.2220082188658,37.4444753008895,50.0489816505963));
#30013=CARTESIAN_POINT('Ctrl Pts',(41.153344655841,37.4402550254882,50.0095058881447));
#30014=CARTESIAN_POINT('Ctrl Pts',(41.0866683465688,37.436034750087,49.9665753267307));
#30015=CARTESIAN_POINT('Ctrl Pts',(41.0223380158291,37.4318144746857,49.92042648864));
#30016=CARTESIAN_POINT('Ctrl Pts',(40.957943339772,37.4275899780258,49.8742314909603));
#30017=CARTESIAN_POINT('Ctrl Pts',(40.8958997120076,37.423365481366,49.8248120604304));
#30018=CARTESIAN_POINT('Ctrl Pts',(40.8365349948571,37.4191409847061,49.7724467886494));
#30019=CARTESIAN_POINT('Ctrl Pts',(40.7771417768612,37.4149144598765,49.7200563764384));
#30020=CARTESIAN_POINT('Ctrl Pts',(40.7204303680073,37.4106879350469,49.6647176337779));
#30021=CARTESIAN_POINT('Ctrl Pts',(40.666691890193,37.4064614102172,49.6067462268128));
#30022=CARTESIAN_POINT('Ctrl Pts',(40.6128551802427,37.4022271594419,49.5486688500592));
#30023=CARTESIAN_POINT('Ctrl Pts',(40.5620025627237,37.3979929086665,49.4879495534256));
#30024=CARTESIAN_POINT('Ctrl Pts',(40.5143848293078,37.3937586578912,49.4249371456156));
#30025=CARTESIAN_POINT('Ctrl Pts',(40.4689700506842,37.3897202976459,49.3648399014603));
#30026=CARTESIAN_POINT('Ctrl Pts',(40.4264976334479,37.3856819374006,49.3026573435625));
#30027=CARTESIAN_POINT('Ctrl Pts',(40.3871465606955,37.3816435771553,49.2387136363099));
#30028=CARTESIAN_POINT('Ctrl Pts',(40.3446380882119,37.3772811922606,49.1696392977945));
#30029=CARTESIAN_POINT('Ctrl Pts',(40.3056184800292,37.3729188073658,49.0982601812154));
#30030=CARTESIAN_POINT('Ctrl Pts',(40.2703369551552,37.3685564224711,49.0249515873066));
#30031=CARTESIAN_POINT('Ctrl Pts',(40.2351169695126,37.3642016465959,48.9517708607319));
#30032=CARTESIAN_POINT('Ctrl Pts',(40.2036222892192,37.3598468707208,48.8766677337123));
#30033=CARTESIAN_POINT('Ctrl Pts',(40.1760577304954,37.3554920948456,48.8000445130183));
#30034=CARTESIAN_POINT('Ctrl Pts',(40.1485459309493,37.3511456541082,48.7235679508708));
#30035=CARTESIAN_POINT('Ctrl Pts',(40.1249494227624,37.3467992133708,48.6455774906775));
#30036=CARTESIAN_POINT('Ctrl Pts',(40.1054254988952,37.3424527726335,48.5664965134752));
#30037=CARTESIAN_POINT('Ctrl Pts',(40.0859237581091,37.3381112703218,48.4875053880746));
#30038=CARTESIAN_POINT('Ctrl Pts',(40.0704855060544,37.3337697680101,48.4074266254418));
#30039=CARTESIAN_POINT('Ctrl Pts',(40.0592185511532,37.3294282656984,48.3266996321309));
#30040=CARTESIAN_POINT('Ctrl Pts',(40.0479640197821,37.3250915505528,48.246061652599));
#30041=CARTESIAN_POINT('Ctrl Pts',(40.040871690593,37.3207548354073,48.1647772909337));
#30042=CARTESIAN_POINT('Ctrl Pts',(40.0379982524025,37.3164181202617,48.0832957696788));
#30043=CARTESIAN_POINT('Ctrl Pts',(40.0370118258954,37.3149293634172,48.0553238673531));
#30044=CARTESIAN_POINT('Ctrl Pts',(40.0365221448597,37.3134406065728,48.027328798736));
#30045=CARTESIAN_POINT('Ctrl Pts',(40.0365300952768,37.3119518497283,47.9993289055974));
#30046=CARTESIAN_POINT('',(40.0365307594277,36.5182018497731,47.9981053315523));
#30047=CARTESIAN_POINT('Ctrl Pts',(40.036530095277,37.3119518496952,47.9993289049744));
#30048=CARTESIAN_POINT('Ctrl Pts',(40.0365552543786,37.307240681783,47.9107233018587));
#30049=CARTESIAN_POINT('Ctrl Pts',(40.0415680366451,37.3025295138709,47.8222574099801));
#30050=CARTESIAN_POINT('Ctrl Pts',(40.0514920247457,37.2978183459587,47.7344802623775));
#30051=CARTESIAN_POINT('Ctrl Pts',(40.0610728789532,37.293270072376,47.6497381158331));
#30052=CARTESIAN_POINT('Ctrl Pts',(40.0752307320124,37.2887217987933,47.5656381757661));
#30053=CARTESIAN_POINT('Ctrl Pts',(40.0938452749518,37.2841735252106,47.4826598555709));
#30054=CARTESIAN_POINT('Ctrl Pts',(40.1134598248503,37.2793809101337,47.3952237897344));
#30055=CARTESIAN_POINT('Ctrl Pts',(40.1380230555135,37.2745882950568,47.309033667321));
#30056=CARTESIAN_POINT('Ctrl Pts',(40.1673362679649,37.26979567998,47.2246271216022));
#30057=CARTESIAN_POINT('Ctrl Pts',(40.1966494804162,37.2650030649031,47.1402205758833));
#30058=CARTESIAN_POINT('Ctrl Pts',(40.2307124154202,37.2602104498262,47.0575979838451));
#30059=CARTESIAN_POINT('Ctrl Pts',(40.2692704858121,37.2554178347493,46.9772672987195));
#30060=CARTESIAN_POINT('Ctrl Pts',(40.3033463952669,37.2511823344831,46.9062746083447));
#30061=CARTESIAN_POINT('Ctrl Pts',(40.3410390123655,37.2469468342168,46.8368518799383));
#30062=CARTESIAN_POINT('Ctrl Pts',(40.3821807048506,37.2427113339506,46.7693921286524));
#30063=CARTESIAN_POINT('Ctrl Pts',(40.4232627549404,37.2384819738153,46.7020301725934));
#30064=CARTESIAN_POINT('Ctrl Pts',(40.4677837088575,37.23425261368,46.6366259399305));
#30065=CARTESIAN_POINT('Ctrl Pts',(40.515529001641,37.2300232535448,46.5735500368944));
#30066=CARTESIAN_POINT('Ctrl Pts',(40.5632185378215,37.2257988324253,46.5105477934356));
#30067=CARTESIAN_POINT('Ctrl Pts',(40.6141246485976,37.2215744113058,46.4498688487173));
#30068=CARTESIAN_POINT('Ctrl Pts',(40.6679890572934,37.2173499901863,46.3918555614484));
#30069=CARTESIAN_POINT('Ctrl Pts',(40.721819020718,37.2131282705043,46.3338793725801));
#30070=CARTESIAN_POINT('Ctrl Pts',(40.7786032088003,37.2089065508222,46.2785658008439));
#30071=CARTESIAN_POINT('Ctrl Pts',(40.8380433709711,37.2046848311402,46.2262238219176));
#30072=CARTESIAN_POINT('Ctrl Pts',(40.8974640845854,37.2004644927861,46.1738989690537));
#30073=CARTESIAN_POINT('Ctrl Pts',(40.9595386947168,37.1962441544319,46.124544088298));
#30074=CARTESIAN_POINT('Ctrl Pts',(41.0239335197275,37.1920238160778,46.0784299433093));
#30075=CARTESIAN_POINT('Ctrl Pts',(41.0883273841898,37.1878035406765,46.0323164861843));
#30076=CARTESIAN_POINT('Ctrl Pts',(41.1550410123622,37.1835832652752,45.9894439409183));
#30077=CARTESIAN_POINT('Ctrl Pts',(41.2237104266237,37.1793629898739,45.9500406637043));
#30078=CARTESIAN_POINT('Ctrl Pts',(41.2924485262967,37.175138493214,45.9105979740336));
#30079=CARTESIAN_POINT('Ctrl Pts',(41.363145911833,37.1709139965542,45.8746317184821));
#30080=CARTESIAN_POINT('Ctrl Pts',(41.4354131207765,37.1666894998944,45.8423247247721));
#30081=CARTESIAN_POINT('Ctrl Pts',(41.507715025018,37.1624629750647,45.8100022205589));
#30082=CARTESIAN_POINT('Ctrl Pts',(41.5815878158893,37.1582364502351,45.7813426479462));
#30083=CARTESIAN_POINT('Ctrl Pts',(41.6566235285636,37.1540099254054,45.7564800284787));
#30084=CARTESIAN_POINT('Ctrl Pts',(41.7317964040052,37.1497756746301,45.7315719609764));
#30085=CARTESIAN_POINT('Ctrl Pts',(41.8081359954775,37.1455414238548,45.7104748411244));
#30086=CARTESIAN_POINT('Ctrl Pts',(41.8852209023398,37.1413071730794,45.6932722480726));
#30087=CARTESIAN_POINT('Ctrl Pts',(41.9587396049162,37.1372688128341,45.6768655042157));
#30088=CARTESIAN_POINT('Ctrl Pts',(42.0329358281995,37.1332304525888,45.6640009333683));
#30089=CARTESIAN_POINT('Ctrl Pts',(42.1074403732221,37.1291920923435,45.6547069893765));
#30090=CARTESIAN_POINT('Ctrl Pts',(42.1855819953439,37.1249565920773,45.6449593443273));
#30091=CARTESIAN_POINT('Ctrl Pts',(42.2643598434414,37.120721091811,45.6391027879781));
#30092=CARTESIAN_POINT('Ctrl Pts',(42.3433526931166,37.1164855915448,45.637208954748));
#30093=CARTESIAN_POINT('Ctrl Pts',(42.4222310282329,37.1122562314095,45.6353178669751));
#30094=CARTESIAN_POINT('Ctrl Pts',(42.5013232807296,37.1080268712743,45.6373781055342));
#30095=CARTESIAN_POINT('Ctrl Pts',(42.5802016825473,37.103797511139,45.6434097100881));
#30096=CARTESIAN_POINT('Ctrl Pts',(42.6589879707454,37.0995730900195,45.6494342709783));
#30097=CARTESIAN_POINT('Ctrl Pts',(42.7375604389768,37.0953486689,45.6594209462268));
#30098=CARTESIAN_POINT('Ctrl Pts',(42.8154914284748,37.0911242477805,45.6733377310482));
#30099=CARTESIAN_POINT('Ctrl Pts',(42.8933725825779,37.0869025280985,45.6872456163487));
#30100=CARTESIAN_POINT('Ctrl Pts',(42.9706126113401,37.0826808084164,45.7050785407085));
#30101=CARTESIAN_POINT('Ctrl Pts',(43.0467903065244,37.0784590887344,45.7267528202402));
#30102=CARTESIAN_POINT('Ctrl Pts',(43.1229430767061,37.0742387503803,45.748420008044));
#30103=CARTESIAN_POINT('Ctrl Pts',(43.1980337524171,37.0700184120261,45.7739259269379));
#30104=CARTESIAN_POINT('Ctrl Pts',(43.2716540948951,37.0657980736719,45.8031364221344));
#30105=CARTESIAN_POINT('Ctrl Pts',(43.3452733392119,37.0615777982707,45.8323464816112));
#30106=CARTESIAN_POINT('Ctrl Pts',(43.4174218581185,37.0573575228694,45.8652608332087));
#30107=CARTESIAN_POINT('Ctrl Pts',(43.4877106888523,37.0531372474681,45.9016969002891));
#30108=CARTESIAN_POINT('Ctrl Pts',(43.5580698247914,37.0489127508082,45.9381694119248));
#30109=CARTESIAN_POINT('Ctrl Pts',(43.6265651390422,37.0446882541484,45.9781704592332));
#30110=CARTESIAN_POINT('Ctrl Pts',(43.6928321724845,37.0404637574885,46.0214714015994));
#30111=CARTESIAN_POINT('Ctrl Pts',(43.7591310205564,37.0362372326589,46.0647931326349));
#30112=CARTESIAN_POINT('Ctrl Pts',(43.8231990766439,37.0320107078292,46.1114176382367));
#30113=CARTESIAN_POINT('Ctrl Pts',(43.8847029193674,37.0277841829996,46.1610743130507));
#30114=CARTESIAN_POINT('Ctrl Pts',(43.9463191890535,37.0235499322242,46.2108217586015));
#30115=CARTESIAN_POINT('Ctrl Pts',(44.0053615282488,37.0193156814489,46.2636121353245));
#30116=CARTESIAN_POINT('Ctrl Pts',(44.0615316703824,37.0150814306736,46.3191362490624));
#30117=CARTESIAN_POINT('Ctrl Pts',(44.1151031948386,37.0110430704283,46.372091632546));
#30118=CARTESIAN_POINT('Ctrl Pts',(44.1660621853139,37.007004710183,46.4275331154113));
#30119=CARTESIAN_POINT('Ctrl Pts',(44.2141849778257,37.0029663499377,46.485165584253));
#30120=CARTESIAN_POINT('Ctrl Pts',(44.2646569734169,36.9987308496714,46.5456114886044));
#30121=CARTESIAN_POINT('Ctrl Pts',(44.3122006470405,36.9944953494052,46.6086975227285));
#30122=CARTESIAN_POINT('Ctrl Pts',(44.3565278733249,36.9902598491389,46.6741081786954));
#30123=CARTESIAN_POINT('Ctrl Pts',(44.4007908392012,36.9860304890037,46.7394240099732));
#30124=CARTESIAN_POINT('Ctrl Pts',(44.4418463562146,36.9818011288684,46.8070573856887));
#30125=CARTESIAN_POINT('Ctrl Pts',(44.479446151567,36.9775717687331,46.8766593821849));
#30126=CARTESIAN_POINT('Ctrl Pts',(44.5170020381539,36.9733473476137,46.9461800979797));
#30127=CARTESIAN_POINT('Ctrl Pts',(44.5511100005808,36.9691229264942,47.0176644553284));
#30128=CARTESIAN_POINT('Ctrl Pts',(44.5815655960173,36.9648985053747,47.090735466889));
#30129=CARTESIAN_POINT('Ctrl Pts',(44.6120017156763,36.9606767856926,47.1637597509189));
#30130=CARTESIAN_POINT('Ctrl Pts',(44.6387899239713,36.9564550660106,47.2383682432688));
#30131=CARTESIAN_POINT('Ctrl Pts',(44.6617727313293,36.9522333463286,47.3141614237189));
#30132=CARTESIAN_POINT('Ctrl Pts',(44.6847480188151,36.9480130079744,47.3899298049779));
#30133=CARTESIAN_POINT('Ctrl Pts',(44.7039202416452,36.9437926696203,47.4668816558271));
#30134=CARTESIAN_POINT('Ctrl Pts',(44.7191813740651,36.9395723312661,47.5446010594111));
#30135=CARTESIAN_POINT('Ctrl Pts',(44.7344422788416,36.9353520558648,47.6223193036901));
#30136=CARTESIAN_POINT('Ctrl Pts',(44.7457921200483,36.9311317804635,47.700804617132));
#30137=CARTESIAN_POINT('Ctrl Pts',(44.7531740242177,36.9269115050623,47.7796310987295));
#30138=CARTESIAN_POINT('Ctrl Pts',(44.7605633120109,36.9226870084024,47.8585364251721));
#30139=CARTESIAN_POINT('Ctrl Pts',(44.7639766905991,36.9184625117426,47.9377831330323));
#30140=CARTESIAN_POINT('Ctrl Pts',(44.7634092838742,36.9142380150827,48.0169410093344));
#30141=CARTESIAN_POINT('Ctrl Pts',(44.7628416047388,36.9100114902531,48.0961368891259));
#30142=CARTESIAN_POINT('Ctrl Pts',(44.7582893600182,36.9057849654234,48.1752433831794));
#30143=CARTESIAN_POINT('Ctrl Pts',(44.7497997582814,36.9015584405938,48.2538336795631));
#30144=CARTESIAN_POINT('Ctrl Pts',(44.7412946378373,36.8973241898184,48.3325676363738));
#30145=CARTESIAN_POINT('Ctrl Pts',(44.7288378523836,36.8930899390431,48.4107830452673));
#30146=CARTESIAN_POINT('Ctrl Pts',(44.7125280832083,36.8888556882678,48.4880617842782));
#30147=CARTESIAN_POINT('Ctrl Pts',(44.6969728582246,36.8848173280225,48.5617653516834));
#30148=CARTESIAN_POINT('Ctrl Pts',(44.6779133952358,36.8807789677771,48.634616663293));
#30149=CARTESIAN_POINT('Ctrl Pts',(44.6554768925876,36.8767406075318,48.7062679575795));
#30150=CARTESIAN_POINT('Ctrl Pts',(44.6319451105851,36.8725051072656,48.7814170422553));
#30151=CARTESIAN_POINT('Ctrl Pts',(44.6046087080825,36.8682696069993,48.8555316137063));
#30152=CARTESIAN_POINT('Ctrl Pts',(44.5735771627301,36.8640341067331,48.9281986633033));
#30153=CARTESIAN_POINT('Ctrl Pts',(44.5425906032687,36.8598047465978,49.0007603687438));
#30154=CARTESIAN_POINT('Ctrl Pts',(44.507919721353,36.8555753864625,49.0718782914855));
#30155=CARTESIAN_POINT('Ctrl Pts',(44.4697236581007,36.8513460263273,49.1411548624084));
#30156=CARTESIAN_POINT('Ctrl Pts',(44.4315721999312,36.8471216052078,49.2103505326594));
#30157=CARTESIAN_POINT('Ctrl Pts',(44.3899039664761,36.8428971840883,49.2777087152894));
#30158=CARTESIAN_POINT('Ctrl Pts',(44.3449254128398,36.8386727629688,49.3428535211965));
#30159=CARTESIAN_POINT('Ctrl Pts',(44.2999756221384,36.8344510432868,49.4079566682316));
#30160=CARTESIAN_POINT('Ctrl Pts',(44.2517199787753,36.8302293236047,49.470848862644));
#30161=CARTESIAN_POINT('Ctrl Pts',(44.2004092899499,36.8260076039227,49.5311815142438));
#30162=CARTESIAN_POINT('Ctrl Pts',(44.1491153897534,36.8217872655686,49.5914944252687));
#30163=CARTESIAN_POINT('Ctrl Pts',(44.0947687328041,36.8175669272144,49.6492490991557));
#30164=CARTESIAN_POINT('Ctrl Pts',(44.0376606758367,36.8133465888603,49.7041296757343));
#30165=CARTESIAN_POINT('Ctrl Pts',(43.9805534707242,36.809126313459,49.7590094336843));
#30166=CARTESIAN_POINT('Ctrl Pts',(43.9206852868116,36.8049060380577,49.8110148552911));
#30167=CARTESIAN_POINT('Ctrl Pts',(43.8583835507378,36.8006857626564,49.8598676995522));
#30168=CARTESIAN_POINT('Ctrl Pts',(43.796019498414,36.7964612659966,49.9087694080384));
#30169=CARTESIAN_POINT('Ctrl Pts',(43.7312174016947,36.7922367693367,49.9545119497349));
#30170=CARTESIAN_POINT('Ctrl Pts',(43.6643364438341,36.7880122726769,49.9968584821396));
#30171=CARTESIAN_POINT('Ctrl Pts',(43.5974233766006,36.7837857478472,50.0392253450038));
#30172=CARTESIAN_POINT('Ctrl Pts',(43.5284298692115,36.7795592230176,50.0781927194547));
#30173=CARTESIAN_POINT('Ctrl Pts',(43.4577404219148,36.7753326981879,50.1135694076012));
#30174=CARTESIAN_POINT('Ctrl Pts',(43.3869217566782,36.7710984474126,50.1490107631476));
#30175=CARTESIAN_POINT('Ctrl Pts',(43.3144013876554,36.7668641966373,50.1808481275017));
#30176=CARTESIAN_POINT('Ctrl Pts',(43.2405843528913,36.7626299458619,50.2089382939716));
#30177=CARTESIAN_POINT('Ctrl Pts',(43.1701823397762,36.7585915856166,50.2357289158727));
#30178=CARTESIAN_POINT('Ctrl Pts',(43.098601334768,36.7545532253713,50.2591113121279));
#30179=CARTESIAN_POINT('Ctrl Pts',(43.0262026282942,36.750514865126,50.2790043240892));
#30180=CARTESIAN_POINT('Ctrl Pts',(42.9502696451231,36.7462793648597,50.2998684502049));
#30181=CARTESIAN_POINT('Ctrl Pts',(42.873148449299,36.7420438645935,50.3169731208476));
#30182=CARTESIAN_POINT('Ctrl Pts',(42.7952456191475,36.7378083643272,50.3301869756405));
#30183=CARTESIAN_POINT('Ctrl Pts',(42.7174557233725,36.733579004192,50.3433816745383));
#30184=CARTESIAN_POINT('Ctrl Pts',(42.6388869022777,36.7293496440567,50.3526966806937));
#30185=CARTESIAN_POINT('Ctrl Pts',(42.5599596166417,36.7251202839215,50.358050754743));
#30186=CARTESIAN_POINT('Ctrl Pts',(42.4811245017114,36.720895862802,50.3633985763438));
#30187=CARTESIAN_POINT('Ctrl Pts',(42.4019322199432,36.7166714416825,50.3647946260616));
#30188=CARTESIAN_POINT('Ctrl Pts',(42.3228105950758,36.712447020563,50.3622091856285));
#30189=CARTESIAN_POINT('Ctrl Pts',(42.243739566992,36.7082253008809,50.3596253985356));
#30190=CARTESIAN_POINT('Ctrl Pts',(42.1647395739628,36.7040035811989,50.3530651900187));
#30191=CARTESIAN_POINT('Ctrl Pts',(42.0862394746819,36.6997818615169,50.3425509116457));
#30192=CARTESIAN_POINT('Ctrl Pts',(42.007765060284,36.6955615231627,50.3320400734978));
#30193=CARTESIAN_POINT('Ctrl Pts',(41.9297906796978,36.6913411848086,50.3175777967216));
#30194=CARTESIAN_POINT('Ctrl Pts',(41.8527396017054,36.6871208464544,50.2992382428445));
#30195=CARTESIAN_POINT('Ctrl Pts',(41.775689673049,36.6829005710531,50.2808989625301));
#30196=CARTESIAN_POINT('Ctrl Pts',(41.6995634758968,36.6786802956518,50.2586826300551));
#30197=CARTESIAN_POINT('Ctrl Pts',(41.6247721537662,36.6744600202505,50.232714094398));
#30198=CARTESIAN_POINT('Ctrl Pts',(41.5499060228899,36.6702355235907,50.2067195841557));
#30199=CARTESIAN_POINT('Ctrl Pts',(41.4763778786821,36.6660110269308,50.1769655278032));
#30200=CARTESIAN_POINT('Ctrl Pts',(41.4045812274179,36.661786530271,50.1436258787604));
#30201=CARTESIAN_POINT('Ctrl Pts',(41.3327501067692,36.6575600054413,50.1102702234393));
#30202=CARTESIAN_POINT('Ctrl Pts',(41.2626525508697,36.6533334806117,50.0733257652574));
#30203=CARTESIAN_POINT('Ctrl Pts',(41.1946573738737,36.649106955782,50.0330124432829));
#30204=CARTESIAN_POINT('Ctrl Pts',(41.1265379039738,36.6448727050067,49.9926254299073));
#30205=CARTESIAN_POINT('Ctrl Pts',(41.0605288845522,36.6406384542314,49.9488575073244));
#30206=CARTESIAN_POINT('Ctrl Pts',(40.9969698785914,36.636404203456,49.9019718502964));
#30207=CARTESIAN_POINT('Ctrl Pts',(40.9363513237343,36.6323658432107,49.8572552797712));
#30208=CARTESIAN_POINT('Ctrl Pts',(40.8779613577221,36.6283274829654,49.809703322906));
#30209=CARTESIAN_POINT('Ctrl Pts',(40.8220636923022,36.6242891227201,49.7595759289525));
#30210=CARTESIAN_POINT('Ctrl Pts',(40.7643098066972,36.6201166587381,49.7077839309448));
#30211=CARTESIAN_POINT('Ctrl Pts',(40.7089831080756,36.6159441947562,49.6530326374279));
#30212=CARTESIAN_POINT('Ctrl Pts',(40.6564092697084,36.6117717307743,49.5955819647205));
#30213=CARTESIAN_POINT('Ctrl Pts',(40.6039242673574,36.6076063171636,49.538228368602));
#30214=CARTESIAN_POINT('Ctrl Pts',(40.5541832096105,36.6034409035529,49.4781848075652));
#30215=CARTESIAN_POINT('Ctrl Pts',(40.5074774148454,36.5992754899422,49.4157502271163));
#30216=CARTESIAN_POINT('Ctrl Pts',(40.4608158950588,36.595114024955,49.3533748318224));
#30217=CARTESIAN_POINT('Ctrl Pts',(40.4171842214425,36.5909525599677,49.2886132972042));
#30218=CARTESIAN_POINT('Ctrl Pts',(40.3768348452745,36.5867910949805,49.2217991641856));
#30219=CARTESIAN_POINT('Ctrl Pts',(40.3365102421364,36.5826321849794,49.1550260525821));
#30220=CARTESIAN_POINT('Ctrl Pts',(40.2994641884032,36.5784732749783,49.0862032564411));
#30221=CARTESIAN_POINT('Ctrl Pts',(40.2659060323137,36.5743143649772,49.0156935453103));
#30222=CARTESIAN_POINT('Ctrl Pts',(40.2323572752878,36.5701566198154,48.9452035827395));
#30223=CARTESIAN_POINT('Ctrl Pts',(40.2022946835431,36.5659988746537,48.8730280809267));
#30224=CARTESIAN_POINT('Ctrl Pts',(40.1758810270027,36.5618411294919,48.7995531469849));
#30225=CARTESIAN_POINT('Ctrl Pts',(40.1494532345774,36.5576811592157,48.726038891217));
#30226=CARTESIAN_POINT('Ctrl Pts',(40.1266784446724,36.5535211889395,48.6512242699834));
#30227=CARTESIAN_POINT('Ctrl Pts',(40.1076703512129,36.5493612186634,48.5755130078388));
#30228=CARTESIAN_POINT('Ctrl Pts',(40.0886566805686,36.5452000278059,48.4997795311728));
#30229=CARTESIAN_POINT('Ctrl Pts',(40.0734120047945,36.5410388369485,48.4231493647047));
#30230=CARTESIAN_POINT('Ctrl Pts',(40.0619989009569,36.536877646091,48.3460365613242));
#30231=CARTESIAN_POINT('Ctrl Pts',(40.0505713886998,36.5327112019577,48.2688264072465));
#30232=CARTESIAN_POINT('Ctrl Pts',(40.0429851519426,36.5285447578243,48.1911328822445));
#30233=CARTESIAN_POINT('Ctrl Pts',(40.0392508194379,36.524378313691,48.1133743682477));
#30234=CARTESIAN_POINT('Ctrl Pts',(40.0374055232866,36.5223194923851,48.0749505036252));
#30235=CARTESIAN_POINT('Ctrl Pts',(40.0364999718189,36.5202606710791,48.0365107667864));
#30236=CARTESIAN_POINT('Ctrl Pts',(40.0365307594277,36.5182018497731,47.9981053315523));
#30237=CARTESIAN_POINT('',(40.0365305727061,35.7244518497007,48.0016453409487));
#30238=CARTESIAN_POINT('Ctrl Pts',(40.0365307594284,36.5182018497283,47.9981053307162));
#30239=CARTESIAN_POINT('Ctrl Pts',(40.0366311430135,36.5114890265903,47.8728837325548));
#30240=CARTESIAN_POINT('Ctrl Pts',(40.0466856383398,36.5047762034523,47.7480505508952));
#30241=CARTESIAN_POINT('Ctrl Pts',(40.0664971456614,36.4980633803143,47.624826880369));
#30242=CARTESIAN_POINT('Ctrl Pts',(40.0789973475601,36.4938278800481,47.5470780884537));
#30243=CARTESIAN_POINT('Ctrl Pts',(40.0954112714295,36.4895923797818,47.4698069314393));
#30244=CARTESIAN_POINT('Ctrl Pts',(40.1156898620174,36.4853568795156,47.3934378561022));
#30245=CARTESIAN_POINT('Ctrl Pts',(40.1359390550856,36.4811275193803,47.317179491684));
#30246=CARTESIAN_POINT('Ctrl Pts',(40.1600416697815,36.4768981592451,47.2418210618124));
#30247=CARTESIAN_POINT('Ctrl Pts',(40.187897285383,36.4726687991098,47.1677788629914));
#30248=CARTESIAN_POINT('Ctrl Pts',(40.2157203714007,36.4684443779903,47.0938231301076));
#30249=CARTESIAN_POINT('Ctrl Pts',(40.2472875846211,36.4642199568709,47.0211810108107));
#30250=CARTESIAN_POINT('Ctrl Pts',(40.2824485681572,36.4599955357514,46.9502541381837));
#30251=CARTESIAN_POINT('Ctrl Pts',(40.3175870669089,36.4557738160693,46.8793726219511));
#30252=CARTESIAN_POINT('Ctrl Pts',(40.3563145667419,36.4515520963873,46.81020459472));
#30253=CARTESIAN_POINT('Ctrl Pts',(40.3984328992107,36.4473303767053,46.7431310402679));
#30254=CARTESIAN_POINT('Ctrl Pts',(40.4405374507487,36.4431100383511,46.6760794319842));
#30255=CARTESIAN_POINT('Ctrl Pts',(40.4860303824847,36.438889699997,46.6111213328787));
#30256=CARTESIAN_POINT('Ctrl Pts',(40.53466869794,36.4346693616428,46.5486111567003));
#30257=CARTESIAN_POINT('Ctrl Pts',(40.5833062878795,36.4304490862415,46.4861019129577));
#30258=CARTESIAN_POINT('Ctrl Pts',(40.635088878997,36.4262288108403,46.4260408891683));
#30259=CARTESIAN_POINT('Ctrl Pts',(40.6897323781643,36.422008535439,46.3687504474789));
#30260=CARTESIAN_POINT('Ctrl Pts',(40.7444305335605,36.4177840387791,46.3114027020014));
#30261=CARTESIAN_POINT('Ctrl Pts',(40.8019949886455,36.4135595421193,46.2568314149466));
#30262=CARTESIAN_POINT('Ctrl Pts',(40.862104279723,36.4093350454594,46.2053225374866));
#30263=CARTESIAN_POINT('Ctrl Pts',(40.922242429114,36.4051085206298,46.1537889307491));
#30264=CARTESIAN_POINT('Ctrl Pts',(40.9849274765946,36.4008819958001,46.1053209500218));
#30265=CARTESIAN_POINT('Ctrl Pts',(41.0498063512841,36.3966554709705,46.0601630089445));
#30266=CARTESIAN_POINT('Ctrl Pts',(41.1148038223814,36.3924212201952,46.0149225206649));
#30267=CARTESIAN_POINT('Ctrl Pts',(41.1820027348204,36.3881869694198,45.9730044116997));
#30268=CARTESIAN_POINT('Ctrl Pts',(41.2510228033739,36.3839527186445,45.9346085498063));
#30269=CARTESIAN_POINT('Ctrl Pts',(41.3168497738978,36.3799143583991,45.897989008243));
#30270=CARTESIAN_POINT('Ctrl Pts',(41.3843327850954,36.3758759981537,45.8645731447572));
#30271=CARTESIAN_POINT('Ctrl Pts',(41.4531259390844,36.3718376379084,45.8344931416259));
#30272=CARTESIAN_POINT('Ctrl Pts',(41.5252773580597,36.3676021376421,45.8029447275344));
#30273=CARTESIAN_POINT('Ctrl Pts',(41.5991443629551,36.3633666373759,45.774946259881));
#30274=CARTESIAN_POINT('Ctrl Pts',(41.6743434436451,36.3591311371096,45.7506861039154));
#30275=CARTESIAN_POINT('Ctrl Pts',(41.7494335095372,36.3549017769743,45.7264611174755));
#30276=CARTESIAN_POINT('Ctrl Pts',(41.8258513735225,36.3506724168391,45.7059638237071));
#30277=CARTESIAN_POINT('Ctrl Pts',(41.9031925918014,36.3464430567038,45.6893349788299));
#30278=CARTESIAN_POINT('Ctrl Pts',(41.9804434915723,36.3422186355843,45.672725552996));
#30279=CARTESIAN_POINT('Ctrl Pts',(42.0586151463996,36.3379942144648,45.6599756969946));
#30280=CARTESIAN_POINT('Ctrl Pts',(42.1372884297915,36.3337697933454,45.6511762365434));
#30281=CARTESIAN_POINT('Ctrl Pts',(42.2159114031058,36.3295480736633,45.6423824031808));
#30282=CARTESIAN_POINT('Ctrl Pts',(42.2950349031182,36.3253263539813,45.6375340034249));
#30283=CARTESIAN_POINT('Ctrl Pts',(42.3742313043362,36.3211046342993,45.6366704810324));
#30284=CARTESIAN_POINT('Ctrl Pts',(42.4534017928445,36.3168842959451,45.6358072411805));
#30285=CARTESIAN_POINT('Ctrl Pts',(42.5326446662259,36.3126639575909,45.6389262948231));
#30286=CARTESIAN_POINT('Ctrl Pts',(42.6115303935436,36.3084436192368,45.6460150099231));
#30287=CARTESIAN_POINT('Ctrl Pts',(42.6904149441587,36.3042233438355,45.653103619284));
#30288=CARTESIAN_POINT('Ctrl Pts',(42.7689418919513,36.3000030684342,45.6641617290631));
#30289=CARTESIAN_POINT('Ctrl Pts',(42.8466864293436,36.2957827930329,45.6791248041439));
#30290=CARTESIAN_POINT('Ctrl Pts',(42.9245087293847,36.2915582963731,45.6941028457856));
#30291=CARTESIAN_POINT('Ctrl Pts',(43.0015465937044,36.2873337997132,45.7129935662894));
#30292=CARTESIAN_POINT('Ctrl Pts',(43.0773856202172,36.2831093030534,45.7356813028147));
#30293=CARTESIAN_POINT('Ctrl Pts',(43.1532610568484,36.2788827782238,45.758379931663));
#30294=CARTESIAN_POINT('Ctrl Pts',(43.2279360661542,36.2746562533941,45.7848790508678));
#30295=CARTESIAN_POINT('Ctrl Pts',(43.3010140810621,36.2704297285645,45.8150139436079));
#30296=CARTESIAN_POINT('Ctrl Pts',(43.3742256801313,36.2661954777891,45.8452039219217));
#30297=CARTESIAN_POINT('Ctrl Pts',(43.4458340259795,36.2619612270138,45.8790427531237));
#30298=CARTESIAN_POINT('Ctrl Pts',(43.5154652931418,36.2577269762384,45.9163187334201));
#30299=CARTESIAN_POINT('Ctrl Pts',(43.5818751861916,36.2536886159932,45.9518702028346));
#30300=CARTESIAN_POINT('Ctrl Pts',(43.6464865999726,36.2496502557479,45.9905476115089));
#30301=CARTESIAN_POINT('Ctrl Pts',(43.7090012376697,36.2456118955026,46.0321315591028));
#30302=CARTESIAN_POINT('Ctrl Pts',(43.7745676429749,36.2413763952364,46.0757455039735));
#30303=CARTESIAN_POINT('Ctrl Pts',(43.838076561073,36.2371408949701,46.1227227955636));
#30304=CARTESIAN_POINT('Ctrl Pts',(43.8991620957885,36.2329053947038,46.172842795091));
#30305=CARTESIAN_POINT('Ctrl Pts',(43.9601590758679,36.2286760345686,46.2228901365277));
#30306=CARTESIAN_POINT('Ctrl Pts',(44.0187392892554,36.2244466744333,46.2760708434371));
#30307=CARTESIAN_POINT('Ctrl Pts',(44.0745655553659,36.2202173142981,46.3321209151494));
#30308=CARTESIAN_POINT('Ctrl Pts',(44.130326627972,36.2159928931786,46.3881055319988));
#30309=CARTESIAN_POINT('Ctrl Pts',(44.1833398146736,36.2117684720591,46.4469525241243));
#30310=CARTESIAN_POINT('Ctrl Pts',(44.2333019846281,36.2075440509396,46.5083585303235));
#30311=CARTESIAN_POINT('Ctrl Pts',(44.2832322047192,36.2033223312575,46.5697252685423));
#30312=CARTESIAN_POINT('Ctrl Pts',(44.3301149850966,36.1991006115755,46.6336474097649));
#30313=CARTESIAN_POINT('Ctrl Pts',(44.3736858107019,36.1948788918935,46.6997866476867));
#30314=CARTESIAN_POINT('Ctrl Pts',(44.4172423801271,36.1906585535393,46.7659042451443));
#30315=CARTESIAN_POINT('Ctrl Pts',(44.4574888885549,36.1864382151852,46.8342371072001));
#30316=CARTESIAN_POINT('Ctrl Pts',(44.4942035873017,36.182217876831,46.904417152456));
#30317=CARTESIAN_POINT('Ctrl Pts',(44.5309177383921,36.1779976014297,46.9745961508681));
#30318=CARTESIAN_POINT('Ctrl Pts',(44.5640999681374,36.1737773260284,47.0466218612126));
#30319=CARTESIAN_POINT('Ctrl Pts',(44.5935747350978,36.1695570506271,47.1201020954449));
#30320=CARTESIAN_POINT('Ctrl Pts',(44.6230789836917,36.1653325539673,47.1936558270296));
#30321=CARTESIAN_POINT('Ctrl Pts',(44.6488681864982,36.1611080573074,47.2686665521205));
#30322=CARTESIAN_POINT('Ctrl Pts',(44.6708154312115,36.1568835606476,47.344723174321));
#30323=CARTESIAN_POINT('Ctrl Pts',(44.6927732127395,36.1526570358179,47.420816311107));
#30324=CARTESIAN_POINT('Ctrl Pts',(44.710885254245,36.1484305109883,47.4979558877583));
#30325=CARTESIAN_POINT('Ctrl Pts',(44.7250755477863,36.1442039861587,47.5757192698385));
#30326=CARTESIAN_POINT('Ctrl Pts',(44.7392917807084,36.1399697353833,47.653624800774));
#30327=CARTESIAN_POINT('Ctrl Pts',(44.7495718795936,36.135735484608,47.7321559491111));
#30328=CARTESIAN_POINT('Ctrl Pts',(44.7558916568792,36.1315012338326,47.810883787191));
#30329=CARTESIAN_POINT('Ctrl Pts',(44.7619190602389,36.1274628735873,47.8859694135201));
#30330=CARTESIAN_POINT('Ctrl Pts',(44.7643444989689,36.123424513342,47.9612335748426));
#30331=CARTESIAN_POINT('Ctrl Pts',(44.7631911188751,36.1193861530967,48.0363067014481));
#30332=CARTESIAN_POINT('Ctrl Pts',(44.7619814343997,36.1151506528304,48.1150446615137));
#30333=CARTESIAN_POINT('Ctrl Pts',(44.7568299978679,36.1109151525642,48.1938717590423));
#30334=CARTESIAN_POINT('Ctrl Pts',(44.747724425971,36.1066796522979,48.2723609013776));
#30335=CARTESIAN_POINT('Ctrl Pts',(44.7386320542631,36.1024502921627,48.3507362593697));
#30336=CARTESIAN_POINT('Ctrl Pts',(44.7255969840385,36.0982209320274,48.4287741727973));
#30337=CARTESIAN_POINT('Ctrl Pts',(44.708658835443,36.0939915718922,48.5060482412094));
#30338=CARTESIAN_POINT('Ctrl Pts',(44.6917404670933,36.0897671507727,48.5832320695306));
#30339=CARTESIAN_POINT('Ctrl Pts',(44.6709281779119,36.0855427296532,48.6596533693462));
#30340=CARTESIAN_POINT('Ctrl Pts',(44.6463131119784,36.0813183085337,48.7348930832808));
#30341=CARTESIAN_POINT('Ctrl Pts',(44.6217137869143,36.0770965888517,48.8100846828406));
#30342=CARTESIAN_POINT('Ctrl Pts',(44.5933166572539,36.0728748691697,48.8840957513468));
#30343=CARTESIAN_POINT('Ctrl Pts',(44.5612631476989,36.0686531494876,48.9565208033799));
#30344=CARTESIAN_POINT('Ctrl Pts',(44.5292201259095,36.0644328111335,49.0289221582586));
#30345=CARTESIAN_POINT('Ctrl Pts',(44.4935232895901,36.0602124727793,49.0997380982307));
#30346=CARTESIAN_POINT('Ctrl Pts',(44.4543622413764,36.0559921344252,49.1685829975261));
#30347=CARTESIAN_POINT('Ctrl Pts',(44.4152017773102,36.0517718590239,49.2374268698934));
#30348=CARTESIAN_POINT('Ctrl Pts',(44.37257743729,36.0475515836226,49.3042993527195));
#30349=CARTESIAN_POINT('Ctrl Pts',(44.3267240960435,36.0433313082214,49.3688406403324));
#30350=CARTESIAN_POINT('Ctrl Pts',(44.2808248907736,36.0391068115615,49.4334464842685));
#30351=CARTESIAN_POINT('Ctrl Pts',(44.2316905049191,36.0348823149017,49.4957160915161));
#30352=CARTESIAN_POINT('Ctrl Pts',(44.1795980236105,36.0306578182418,49.5553203256119));
#30353=CARTESIAN_POINT('Ctrl Pts',(44.1274805328378,36.0264312934122,49.6149531755447));
#30354=CARTESIAN_POINT('Ctrl Pts',(44.0724024441464,36.0222047685826,49.6719177652434));
#30355=CARTESIAN_POINT('Ctrl Pts',(44.0146780853099,36.0179782437529,49.7259215282625));
#30356=CARTESIAN_POINT('Ctrl Pts',(43.9568482082806,36.0137439929776,49.78002400835));
#30357=CARTESIAN_POINT('Ctrl Pts',(43.8963627544433,36.0095097422022,49.8311545429287));
#30358=CARTESIAN_POINT('Ctrl Pts',(43.8335693787318,36.0052754914269,49.8790607433669));
#30359=CARTESIAN_POINT('Ctrl Pts',(43.7736810335206,36.0012371311816,49.9247506435688));
#30360=CARTESIAN_POINT('Ctrl Pts',(43.7116939031599,35.9971987709362,49.9675077763346));
#30361=CARTESIAN_POINT('Ctrl Pts',(43.6479313278327,35.9931604106909,50.0071516738687));
#30362=CARTESIAN_POINT('Ctrl Pts',(43.5810560645158,35.9889249104246,50.0487308615488));
#30363=CARTESIAN_POINT('Ctrl Pts',(43.5119733797754,35.9846894101584,50.0870431477272));
#30364=CARTESIAN_POINT('Ctrl Pts',(43.4410357712582,35.9804539098921,50.1218470642016));
#30365=CARTESIAN_POINT('Ctrl Pts',(43.3702009997569,35.9762245497569,50.1566005260443));
#30366=CARTESIAN_POINT('Ctrl Pts',(43.297517062263,35.9719951896216,50.1878555131392));
#30367=CARTESIAN_POINT('Ctrl Pts',(43.2233640076852,35.9677658294863,50.2154146681262));
#30368=CARTESIAN_POINT('Ctrl Pts',(43.1492975485011,35.9635414083668,50.2429416397339));
#30369=CARTESIAN_POINT('Ctrl Pts',(43.073765819162,35.9593169872473,50.2667811932017));
#30370=CARTESIAN_POINT('Ctrl Pts',(42.9971705668534,35.9550925661278,50.2867832767851));
#30371=CARTESIAN_POINT('Ctrl Pts',(42.9206242957608,35.9508708464458,50.3067725694141));
#30372=CARTESIAN_POINT('Ctrl Pts',(42.8430163044532,35.9466491267638,50.322929144534));
#30373=CARTESIAN_POINT('Ctrl Pts',(42.764764127109,35.9424274070817,50.3351525801271));
#30374=CARTESIAN_POINT('Ctrl Pts',(42.6865375535287,35.9382070687276,50.3473720162666));
#30375=CARTESIAN_POINT('Ctrl Pts',(42.6076676758178,35.9339867303734,50.3556607958653));
#30376=CARTESIAN_POINT('Ctrl Pts',(42.5285813894844,35.9297663920192,50.3599697598017));
#30377=CARTESIAN_POINT('Ctrl Pts',(42.4494962828452,35.9255461166179,50.3642786594632));
#30378=CARTESIAN_POINT('Ctrl Pts',(42.3701952427293,35.9213258412166,50.3646078372648));
#30379=CARTESIAN_POINT('Ctrl Pts',(42.2911079410338,35.9171055658154,50.3609601776384));
#30380=CARTESIAN_POINT('Ctrl Pts',(42.2119415336124,35.9128810691555,50.3573088695025));
#30381=CARTESIAN_POINT('Ctrl Pts',(42.1329897616534,35.9086565724957,50.3496727995296));
#30382=CARTESIAN_POINT('Ctrl Pts',(42.0546793388577,35.9044320758358,50.3381069440657));
#30383=CARTESIAN_POINT('Ctrl Pts',(41.9763313194327,35.9002055510062,50.3265355358649));
#30384=CARTESIAN_POINT('Ctrl Pts',(41.8986257234762,35.8959790261765,50.3110306756431));
#30385=CARTESIAN_POINT('Ctrl Pts',(41.8219786562303,35.8917525013469,50.2916984459232));
#30386=CARTESIAN_POINT('Ctrl Pts',(41.7451914807151,35.8875182505715,50.2723308775354));
#30387=CARTESIAN_POINT('Ctrl Pts',(41.6694671503326,35.8832839997962,50.2491220972927));
#30388=CARTESIAN_POINT('Ctrl Pts',(41.5952060093662,35.8790497490208,50.2222279526502));
#30389=CARTESIAN_POINT('Ctrl Pts',(41.5243804358801,35.8750113887755,50.1965780206273));
#30390=CARTESIAN_POINT('Ctrl Pts',(41.4548859772165,35.8709730285303,50.1675763491656));
#30391=CARTESIAN_POINT('Ctrl Pts',(41.3870493361438,35.866934668285,50.1353972448922));
#30392=CARTESIAN_POINT('Ctrl Pts',(41.3159011240294,35.8626991680187,50.1016472581552));
#30393=CARTESIAN_POINT('Ctrl Pts',(41.2463062715651,35.8584636677525,50.0642734021379));
#30394=CARTESIAN_POINT('Ctrl Pts',(41.1786585585128,35.8542281674862,50.0234415050122));
#30395=CARTESIAN_POINT('Ctrl Pts',(41.1111089131723,35.849998807351,49.9826688011768));
#30396=CARTESIAN_POINT('Ctrl Pts',(41.0455012002203,35.8457694472157,49.9384482517782));
#30397=CARTESIAN_POINT('Ctrl Pts',(40.9822070059609,35.8415400870805,49.8909927199632));
#30398=CARTESIAN_POINT('Ctrl Pts',(40.9189867261978,35.837315665961,49.8435926063704));
#30399=CARTESIAN_POINT('Ctrl Pts',(40.8580749698998,35.8330912448415,49.7929652976213));
#30400=CARTESIAN_POINT('Ctrl Pts',(40.7998152766036,35.828866823722,49.7393674976579));
#30401=CARTESIAN_POINT('Ctrl Pts',(40.7415928392801,35.82464510404,49.6858039724745));
#30402=CARTESIAN_POINT('Ctrl Pts',(40.6860194433523,35.820423384358,49.6292740432384));
#30403=CARTESIAN_POINT('Ctrl Pts',(40.6334054289925,35.8162016646759,49.5700745404556));
#30404=CARTESIAN_POINT('Ctrl Pts',(40.5808086297038,35.8119813263218,49.5108944074863));
#30405=CARTESIAN_POINT('Ctrl Pts',(40.5311696008259,35.8077609879676,49.4490467859523));
#30406=CARTESIAN_POINT('Ctrl Pts',(40.4847606333963,35.8035406496135,49.384864112291));
#30407=CARTESIAN_POINT('Ctrl Pts',(40.4383523582283,35.7993203742122,49.3206823960135));
#30408=CARTESIAN_POINT('Ctrl Pts',(40.3951743226679,35.7951000988109,49.2541660779658));
#30409=CARTESIAN_POINT('Ctrl Pts',(40.3554565496667,35.7908798234096,49.185678084726));
#30410=CARTESIAN_POINT('Ctrl Pts',(40.3156990496398,35.7866553267498,49.1171215875377));
#30411=CARTESIAN_POINT('Ctrl Pts',(40.2794089621146,35.78243083009,49.0465898825571));
#30412=CARTESIAN_POINT('Ctrl Pts',(40.2467708989212,35.7782063334301,48.974471589718));
#30413=CARTESIAN_POINT('Ctrl Pts',(40.2141171662791,35.7739798086005,48.902318673075));
#30414=CARTESIAN_POINT('Ctrl Pts',(40.1851191228135,35.7697532837708,48.828578088533));
#30415=CARTESIAN_POINT('Ctrl Pts',(40.1599126595402,35.7655267589412,48.753657182021));
#30416=CARTESIAN_POINT('Ctrl Pts',(40.1346601196971,35.7612925081659,48.6785993226037));
#30417=CARTESIAN_POINT('Ctrl Pts',(40.1132131370043,35.7570582573905,48.6023572828514));
#30418=CARTESIAN_POINT('Ctrl Pts',(40.0956572222283,35.7528240066152,48.5253520756895));
#30419=CARTESIAN_POINT('Ctrl Pts',(40.0789135024857,35.7487856463698,48.4519093856397));
#30420=CARTESIAN_POINT('Ctrl Pts',(40.0657088114729,35.7447472861245,48.3777729380046));
#30421=CARTESIAN_POINT('Ctrl Pts',(40.0560732958414,35.7407089258792,48.3033117973838));
#30422=CARTESIAN_POINT('Ctrl Pts',(40.0431435172632,35.7352899004955,48.2033933189411));
#30423=CARTESIAN_POINT('Ctrl Pts',(40.0366008742664,35.7298708751119,48.1026308155814));
#30424=CARTESIAN_POINT('Ctrl Pts',(40.0365305727064,35.7244518497283,48.0016453414631));
#30425=CARTESIAN_POINT('',(40.0365302293311,34.930701849776,48.0010411697219));
#30426=CARTESIAN_POINT('Ctrl Pts',(40.0365305727061,35.7244518497007,48.0016453409487));
#30427=CARTESIAN_POINT('Ctrl Pts',(40.0364764503775,35.7202799598572,47.923900683194));
#30428=CARTESIAN_POINT('Ctrl Pts',(40.0402625742032,35.7161080700138,47.8460064445692));
#30429=CARTESIAN_POINT('Ctrl Pts',(40.0479067550704,35.7119361801703,47.7683800352804));
#30430=CARTESIAN_POINT('Ctrl Pts',(40.0555407043263,35.7077698743334,47.6908575276738));
#30431=CARTESIAN_POINT('Ctrl Pts',(40.0670224088016,35.7036035684964,47.613602615599));
#30432=CARTESIAN_POINT('Ctrl Pts',(40.0823176524898,35.6994372626595,47.537032423447));
#30433=CARTESIAN_POINT('Ctrl Pts',(40.0976016605286,35.6952740173263,47.4605184785728));
#30434=CARTESIAN_POINT('Ctrl Pts',(40.116693558554,35.6911107719931,47.3846887289259));
#30435=CARTESIAN_POINT('Ctrl Pts',(40.1395075048344,35.6869475266599,47.3099535376514));
#30436=CARTESIAN_POINT('Ctrl Pts',(40.1623122877722,35.6827859535163,47.2352483641628));
#30437=CARTESIAN_POINT('Ctrl Pts',(40.1888360119416,35.6786243803726,47.161637339074));
#30438=CARTESIAN_POINT('Ctrl Pts',(40.2189425039841,35.674462807229,47.0895173587745));
#30439=CARTESIAN_POINT('Ctrl Pts',(40.2490469258089,35.6703015202483,47.0174023376734));
#30440=CARTESIAN_POINT('Ctrl Pts',(40.2827334384652,35.6661402332677,46.9467786036397));
#30441=CARTESIAN_POINT('Ctrl Pts',(40.3198177222954,35.661978946287,46.8780231141313));
#30442=CARTESIAN_POINT('Ctrl Pts',(40.3569366995747,35.6578137662987,46.8092033018202));
#30443=CARTESIAN_POINT('Ctrl Pts',(40.3974595657716,35.6536485863105,46.7422556511874));
#30444=CARTESIAN_POINT('Ctrl Pts',(40.4411564144341,35.6494834063222,46.6775317591006));
#30445=CARTESIAN_POINT('Ctrl Pts',(40.4848737671885,35.6453162718857,46.6127774962969));
#30446=CARTESIAN_POINT('Ctrl Pts',(40.5317677753964,35.6411491374491,46.5502494556462));
#30447=CARTESIAN_POINT('Ctrl Pts',(40.58156725145,35.6369820030125,46.4902673150849));
#30448=CARTESIAN_POINT('Ctrl Pts',(40.6314538750544,35.6328075762189,46.4301802076233));
#30449=CARTESIAN_POINT('Ctrl Pts',(40.684255791651,35.6286331494253,46.3726482531046));
#30450=CARTESIAN_POINT('Ctrl Pts',(40.7396642417081,35.6244587226317,46.3179549320434));
#30451=CARTESIAN_POINT('Ctrl Pts',(40.7838003742899,35.6211335429122,46.2743884423254));
#30452=CARTESIAN_POINT('Ctrl Pts',(40.8295895906978,35.6178083631928,46.2326223958576));
#30453=CARTESIAN_POINT('Ctrl Pts',(40.8768618671674,35.6144831834733,46.1927809570473));
#30454=CARTESIAN_POINT('Ctrl Pts',(40.9370756770865,35.610247683207,46.1420322941396));
#30455=CARTESIAN_POINT('Ctrl Pts',(40.9999430179682,35.6060121829408,46.0941998150729));
#30456=CARTESIAN_POINT('Ctrl Pts',(41.0651497065104,35.6017766826745,46.0495730890724));
#30457=CARTESIAN_POINT('Ctrl Pts',(41.1302618660514,35.5975473225392,46.0050110576596));
#30458=CARTESIAN_POINT('Ctrl Pts',(41.1977062546563,35.5933179624039,45.9636458133875));
#30459=CARTESIAN_POINT('Ctrl Pts',(41.2671350908877,35.5890886022687,45.9257272265678));
#30460=CARTESIAN_POINT('Ctrl Pts',(41.3364828486331,35.5848641811492,45.8878529207959));
#30461=CARTESIAN_POINT('Ctrl Pts',(41.4078100390722,35.5806397600296,45.8534174978916));
#30462=CARTESIAN_POINT('Ctrl Pts',(41.4807406163786,35.5764153389101,45.8226271273564));
#30463=CARTESIAN_POINT('Ctrl Pts',(41.5536245559595,35.5721936192281,45.7918564466812));
#30464=CARTESIAN_POINT('Ctrl Pts',(41.6281094161086,35.567971899546,45.7647263740122));
#30465=CARTESIAN_POINT('Ctrl Pts',(41.7037964030363,35.563750179864,45.7413962294207));
#30466=CARTESIAN_POINT('Ctrl Pts',(41.779458625519,35.5595298415098,45.7180737183487));
#30467=CARTESIAN_POINT('Ctrl Pts',(41.8563217455693,35.5553095031556,45.6985488046853));
#30468=CARTESIAN_POINT('Ctrl Pts',(41.9339703460991,35.5510891648014,45.6829314203967));
#30469=CARTESIAN_POINT('Ctrl Pts',(42.01161778838,35.5468688894001,45.6673142690655));
#30470=CARTESIAN_POINT('Ctrl Pts',(42.0900502274505,35.5426486139988,45.6556046224865));
#30471=CARTESIAN_POINT('Ctrl Pts',(42.168842027597,35.5384283385975,45.6478613066627));
#30472=CARTESIAN_POINT('Ctrl Pts',(42.247712637899,35.5342038419376,45.6401102457192));
#30473=CARTESIAN_POINT('Ctrl Pts',(42.3269428590963,35.5299793452778,45.6363334866369));
#30474=CARTESIAN_POINT('Ctrl Pts',(42.4061025050981,35.5257548486179,45.6365378783802));
#30475=CARTESIAN_POINT('Ctrl Pts',(42.4853001554389,35.5215283237882,45.6367423682515));
#30476=CARTESIAN_POINT('Ctrl Pts',(42.5644266937462,35.5173017989586,45.6409317917222));
#30477=CARTESIAN_POINT('Ctrl Pts',(42.6430550960828,35.5130752741289,45.6490608980307));
#30478=CARTESIAN_POINT('Ctrl Pts',(42.721827228503,35.5088410233535,45.6572048640731));
#30479=CARTESIAN_POINT('Ctrl Pts',(42.8000989403447,35.5046067725782,45.669302831574));
#30480=CARTESIAN_POINT('Ctrl Pts',(42.8774516614981,35.5003725218028,45.6852580377432));
#30481=CARTESIAN_POINT('Ctrl Pts',(42.9512257883815,35.4963341615577,45.7004751029843));
#30482=CARTESIAN_POINT('Ctrl Pts',(43.0241637384678,35.4922958013126,45.7192002777303));
#30483=CARTESIAN_POINT('Ctrl Pts',(43.0959171705692,35.4882574410675,45.7413079597681));
#30484=CARTESIAN_POINT('Ctrl Pts',(43.1711733791099,35.4840219408013,45.7644948691752));
#30485=CARTESIAN_POINT('Ctrl Pts',(43.2454125328606,35.479786440535,45.7914911032359));
#30486=CARTESIAN_POINT('Ctrl Pts',(43.3182211254831,35.4755509402688,45.8221890794616));
#30487=CARTESIAN_POINT('Ctrl Pts',(43.3909241687566,35.4713215801336,45.8528425533656));
#30488=CARTESIAN_POINT('Ctrl Pts',(43.4622003403966,35.4670922199983,45.8871869320056));
#30489=CARTESIAN_POINT('Ctrl Pts',(43.5316513456607,35.4628628598631,45.925064899144));
#30490=CARTESIAN_POINT('Ctrl Pts',(43.6010212465498,35.4586384387436,45.96289863267));
#30491=CARTESIAN_POINT('Ctrl Pts',(43.668569806671,35.4544140176242,46.0042575310109));
#30492=CARTESIAN_POINT('Ctrl Pts',(43.7339201940952,35.4501895965047,46.0489368650182));
#30493=CARTESIAN_POINT('Ctrl Pts',(43.7992287911819,35.4459678768227,46.0935876274359));
#30494=CARTESIAN_POINT('Ctrl Pts',(43.8623416191588,35.4417461571407,46.1415543469306));
#30495=CARTESIAN_POINT('Ctrl Pts',(43.9229089413283,35.4375244374587,46.1925878175352));
#30496=CARTESIAN_POINT('Ctrl Pts',(43.9834564461398,35.4333040991045,46.2436045902155));
#30497=CARTESIAN_POINT('Ctrl Pts',(44.0414597403089,35.4290837607504,46.2976858193327));
#30498=CARTESIAN_POINT('Ctrl Pts',(44.0966016308579,35.4248634223963,46.3545415997144));
#30499=CARTESIAN_POINT('Ctrl Pts',(44.1517426988804,35.420643146995,46.4113965320044));
#30500=CARTESIAN_POINT('Ctrl Pts',(44.2040221223187,35.4164228715937,46.4710255954416));
#30501=CARTESIAN_POINT('Ctrl Pts',(44.2531601615548,35.4122025961925,46.5331026428117));
#30502=CARTESIAN_POINT('Ctrl Pts',(44.3023473502774,35.4079780995326,46.5952417816906));
#30503=CARTESIAN_POINT('Ctrl Pts',(44.3483865860238,35.4037536028728,46.6598334269079));
#30504=CARTESIAN_POINT('Ctrl Pts',(44.3910393816092,35.399529106213,46.7265194851191));
#30505=CARTESIAN_POINT('Ctrl Pts',(44.4337126546901,35.3953025813834,46.7932375591324));
#30506=CARTESIAN_POINT('Ctrl Pts',(44.4729960157661,35.3910760565538,46.8620516410921));
#30507=CARTESIAN_POINT('Ctrl Pts',(44.508696505682,35.3868495317241,46.9325781116051));
#30508=CARTESIAN_POINT('Ctrl Pts',(44.5444622548967,35.3826152809488,47.0032335021419));
#30509=CARTESIAN_POINT('Ctrl Pts',(44.5766318546358,35.3783810301735,47.0756071060647));
#30510=CARTESIAN_POINT('Ctrl Pts',(44.6050602422551,35.3741467793982,47.1492945463172));
#30511=CARTESIAN_POINT('Ctrl Pts',(44.6321734380714,35.3701084191527,47.2195729603982));
#30512=CARTESIAN_POINT('Ctrl Pts',(44.6558838508024,35.3660700589071,47.2910459837102));
#30513=CARTESIAN_POINT('Ctrl Pts',(44.6761086658167,35.3620316986616,47.3633527018089));
#30514=CARTESIAN_POINT('Ctrl Pts',(44.6973207925635,35.3577961983954,47.4391892060176));
#30515=CARTESIAN_POINT('Ctrl Pts',(44.7147789523769,35.3535606981292,47.5162311508201));
#30516=CARTESIAN_POINT('Ctrl Pts',(44.7283499217397,35.3493251978629,47.5940725645698));
#30517=CARTESIAN_POINT('Ctrl Pts',(44.7419012175044,35.3450958377277,47.6718011329772));
#30518=CARTESIAN_POINT('Ctrl Pts',(44.7515764333856,35.3408664775925,47.7503264103434));
#30519=CARTESIAN_POINT('Ctrl Pts',(44.7572924026886,35.3366371174573,47.8292283128655));
#30520=CARTESIAN_POINT('Ctrl Pts',(44.7630016969245,35.3324126963378,47.9080380743241));
#30521=CARTESIAN_POINT('Ctrl Pts',(44.7647608987576,35.3281882752184,47.9872231212413));
#30522=CARTESIAN_POINT('Ctrl Pts',(44.7625383282817,35.3239638540989,48.0663557706616));
#30523=CARTESIAN_POINT('Ctrl Pts',(44.7603171790975,35.3197421344169,48.1454378162483));
#30524=CARTESIAN_POINT('Ctrl Pts',(44.7541193245437,35.3155204147349,48.2244670629436));
#30525=CARTESIAN_POINT('Ctrl Pts',(44.743965149256,35.3112986950529,48.3030145540616));
#30526=CARTESIAN_POINT('Ctrl Pts',(44.7338142963693,35.3070783566988,48.3815363447903));
#30527=CARTESIAN_POINT('Ctrl Pts',(44.7197097533064,35.3028580183447,48.4595762278133));
#30528=CARTESIAN_POINT('Ctrl Pts',(44.7017237397524,35.2986376799906,48.536710598703));
#30529=CARTESIAN_POINT('Ctrl Pts',(44.6837379944876,35.2944174045893,48.6138438190142));
#30530=CARTESIAN_POINT('Ctrl Pts',(44.6618710017028,35.2901971291881,48.6900710972545));
#30531=CARTESIAN_POINT('Ctrl Pts',(44.6362457236063,35.2859768537868,48.7649807216868));
#30532=CARTESIAN_POINT('Ctrl Pts',(44.610594814262,35.281752357127,48.8399652731946));
#30533=CARTESIAN_POINT('Ctrl Pts',(44.5811782624854,35.2775278604672,48.913629092954));
#30534=CARTESIAN_POINT('Ctrl Pts',(44.5481682152923,35.2733033638074,48.9855778810971));
#30535=CARTESIAN_POINT('Ctrl Pts',(44.5151423200618,35.2690768389778,49.0575612116653));
#30536=CARTESIAN_POINT('Ctrl Pts',(44.478519709777,35.2648503141482,49.1278274535547));
#30537=CARTESIAN_POINT('Ctrl Pts',(44.4385186298535,35.2606237893186,49.1960067878737));
#30538=CARTESIAN_POINT('Ctrl Pts',(44.398444429297,35.2563895385433,49.2643107517302));
#30539=CARTESIAN_POINT('Ctrl Pts',(44.3549796767984,35.252155287768,49.3305197917651));
#30540=CARTESIAN_POINT('Ctrl Pts',(44.3083859871555,35.2479210369927,49.3942931416773));
#30541=CARTESIAN_POINT('Ctrl Pts',(44.2639478766286,35.2438826767471,49.4551161242269));
#30542=CARTESIAN_POINT('Ctrl Pts',(44.216664189521,35.2398443165014,49.5137235441245));
#30543=CARTESIAN_POINT('Ctrl Pts',(44.1667936629992,35.2358059562558,49.5698505002981));
#30544=CARTESIAN_POINT('Ctrl Pts',(44.1144886145335,35.2315704559894,49.6287173975946));
#30545=CARTESIAN_POINT('Ctrl Pts',(44.0591388925338,35.2273349557229,49.6850792364415));
#30546=CARTESIAN_POINT('Ctrl Pts',(44.0010138577604,35.2230994554565,49.7386043449156));
#30547=CARTESIAN_POINT('Ctrl Pts',(43.9429730858376,35.2188700953211,49.7920518589721));
#30548=CARTESIAN_POINT('Ctrl Pts',(43.8821653330907,35.2146407351856,49.8426704938245));
#30549=CARTESIAN_POINT('Ctrl Pts',(43.8188989093145,35.2104113750502,49.8901630421861));
#30550=CARTESIAN_POINT('Ctrl Pts',(43.7557063676045,35.2061869539305,49.9376001290976));
#30551=CARTESIAN_POINT('Ctrl Pts',(43.6900612339192,35.2019625328108,49.9819181036721));
#30552=CARTESIAN_POINT('Ctrl Pts',(43.6223060630681,35.1977381116912,50.0228589493801));
#30553=CARTESIAN_POINT('Ctrl Pts',(43.5545942203681,35.193516392009,50.063773614191));
#30554=CARTESIAN_POINT('Ctrl Pts',(43.4847754192573,35.1892946723268,50.1013151944229));
#30555=CARTESIAN_POINT('Ctrl Pts',(43.4132214522624,35.1850729526445,50.13526877221));
#30556=CARTESIAN_POINT('Ctrl Pts',(43.3416908974067,35.1808526142902,50.1692112405378));
#30557=CARTESIAN_POINT('Ctrl Pts',(43.2684267277205,35.1766322759359,50.1995678364937));
#30558=CARTESIAN_POINT('Ctrl Pts',(43.1938242766516,35.1724119375815,50.2261701324694));
#30559=CARTESIAN_POINT('Ctrl Pts',(43.1192229383935,35.1681916621801,50.2527720316307));
#30560=CARTESIAN_POINT('Ctrl Pts',(43.0432838009675,35.1639713867786,50.2756195857444));
#30561=CARTESIAN_POINT('Ctrl Pts',(42.9664196470083,35.1597511113771,50.2945934769329));
#30562=CARTESIAN_POINT('Ctrl Pts',(42.8894786109889,35.1555266147171,50.3135863464327));
#30563=CARTESIAN_POINT('Ctrl Pts',(42.8116111669309,35.1513021180571,50.3286977003229));
#30564=CARTESIAN_POINT('Ctrl Pts',(42.73324206216,35.1470776213971,50.3398590062026));
#30565=CARTESIAN_POINT('Ctrl Pts',(42.6548353325869,35.1428510965673,50.351025670596));
#30566=CARTESIAN_POINT('Ctrl Pts',(42.5759269305515,35.1386245717375,50.3582384663198));
#30567=CARTESIAN_POINT('Ctrl Pts',(42.4969459530339,35.1343980469076,50.3614808750211));
#30568=CARTESIAN_POINT('Ctrl Pts',(42.4178206009374,35.1301637961321,50.3647292107367));
#30569=CARTESIAN_POINT('Ctrl Pts',(42.3386228788274,35.1259295453566,50.3639926611499));
#30570=CARTESIAN_POINT('Ctrl Pts',(42.2597809121065,35.1216952945811,50.3593068999794));
#30571=CARTESIAN_POINT('Ctrl Pts',(42.184586437139,35.1176569343374,50.354837917714));
#30572=CARTESIAN_POINT('Ctrl Pts',(42.1097158798324,35.1136185740936,50.3467771251438));
#30573=CARTESIAN_POINT('Ctrl Pts',(42.0355320040277,35.1095802138499,50.3351988182619));
#30574=CARTESIAN_POINT('Ctrl Pts',(41.9577267051587,35.1053447135838,50.3230552949212));
#30575=CARTESIAN_POINT('Ctrl Pts',(41.8803810882845,35.1011092133178,50.3069959003845));
#30576=CARTESIAN_POINT('Ctrl Pts',(41.8039198206799,35.0968737130518,50.2870677429236));
#30577=CARTESIAN_POINT('Ctrl Pts',(41.7275693976435,35.0926443529168,50.2671684749656));
#30578=CARTESIAN_POINT('Ctrl Pts',(41.6521012283375,35.0884149927817,50.2434116989024));
#30579=CARTESIAN_POINT('Ctrl Pts',(41.5779320654063,35.0841856326467,50.2158959253117));
#30580=CARTESIAN_POINT('Ctrl Pts',(41.5038495166799,35.0799612115274,50.1884122844397));
#30581=CARTESIAN_POINT('Ctrl Pts',(41.4310633975859,35.0757367904082,50.1571785316532));
#30582=CARTESIAN_POINT('Ctrl Pts',(41.3599760265035,35.0715123692889,50.1223431804147));
#30583=CARTESIAN_POINT('Ctrl Pts',(41.2889341144513,35.0672906496071,50.0875301057248));
#30584=CARTESIAN_POINT('Ctrl Pts',(41.2195892146319,35.0630689299253,50.0491202098274));
#30585=CARTESIAN_POINT('Ctrl Pts',(41.1523232155949,35.0588472102435,50.007309911936));
#30586=CARTESIAN_POINT('Ctrl Pts',(41.0850792256931,35.0546268718895,49.9655132941879));
#30587=CARTESIAN_POINT('Ctrl Pts',(41.0199131842295,35.0504065335356,49.9203187312767));
#30588=CARTESIAN_POINT('Ctrl Pts',(40.9571806155803,35.0461861951817,49.8719675918249));
#30589=CARTESIAN_POINT('Ctrl Pts',(40.8944489826845,35.0419659197806,49.8236171736053));
#30590=CARTESIAN_POINT('Ctrl Pts',(40.8341511213803,35.0377456443796,49.7721105600202));
#30591=CARTESIAN_POINT('Ctrl Pts',(40.7766106932438,35.0335253689785,49.7177303628945));
#30592=CARTESIAN_POINT('Ctrl Pts',(40.7190127112742,35.0293008723189,49.6632957729029));
#30593=CARTESIAN_POINT('Ctrl Pts',(40.6641780140076,35.0250763756593,49.60598218084));
#30594=CARTESIAN_POINT('Ctrl Pts',(40.6123940238051,35.0208518789996,49.5461097356825));
#30595=CARTESIAN_POINT('Ctrl Pts',(40.5605851722442,35.0166253541702,49.4862085459205));
#30596=CARTESIAN_POINT('Ctrl Pts',(40.5118302346726,35.0123988293408,49.4237464262382));
#30597=CARTESIAN_POINT('Ctrl Pts',(40.4663752413027,35.0081723045113,49.3590753229505));
#30598=CARTESIAN_POINT('Ctrl Pts',(40.4208371577289,35.0039380537362,49.294286003054));
#30599=CARTESIAN_POINT('Ctrl Pts',(40.378611322974,34.9997038029611,49.2272800289112));
#30600=CARTESIAN_POINT('Ctrl Pts',(40.3398993466385,34.995469552186,49.1584367651796));
#30601=CARTESIAN_POINT('Ctrl Pts',(40.3029783151194,34.9914311919386,49.0927784198632));
#30602=CARTESIAN_POINT('Ctrl Pts',(40.2692533335794,34.9873928316913,49.025449359582));
#30603=CARTESIAN_POINT('Ctrl Pts',(40.238858169154,34.983354471444,48.9567948724086));
#30604=CARTESIAN_POINT('Ctrl Pts',(40.203843215612,34.9787023170925,48.8777055263148));
#30605=CARTESIAN_POINT('Ctrl Pts',(40.173132350658,34.9740501627411,48.7965988730332));
#30606=CARTESIAN_POINT('Ctrl Pts',(40.1469392857684,34.9693980083896,48.7139382738627));
#30607=CARTESIAN_POINT('Ctrl Pts',(40.1208200312477,34.9647589635093,48.6315106069341));
#30608=CARTESIAN_POINT('Ctrl Pts',(40.099193315503,34.960119918629,48.5475380103431));
#30609=CARTESIAN_POINT('Ctrl Pts',(40.0822249547242,34.9554808737487,48.4625032760932));
#30610=CARTESIAN_POINT('Ctrl Pts',(40.0653374664262,34.9508639389044,48.3778738237676));
#30611=CARTESIAN_POINT('Ctrl Pts',(40.053064163275,34.9462470040601,48.2921926237583));
#30612=CARTESIAN_POINT('Ctrl Pts',(40.0455206172929,34.9416300692159,48.2059545515576));
#30613=CARTESIAN_POINT('Ctrl Pts',(40.0395687950972,34.9379873294026,48.1379131193904));
#30614=CARTESIAN_POINT('Ctrl Pts',(40.0365603984321,34.9343445895893,48.0695254491627));
#30615=CARTESIAN_POINT('Ctrl Pts',(40.0365302293311,34.930701849776,48.0010411697218));
#30616=CARTESIAN_POINT('',(40.0365309009773,34.1369518496884,47.9979362983109));
#30617=CARTESIAN_POINT('Ctrl Pts',(40.0365302293307,34.9307018497283,48.0010411688257));
#30618=CARTESIAN_POINT('Ctrl Pts',(40.0364946440264,34.9264051318271,47.9202619629236));
#30619=CARTESIAN_POINT('Ctrl Pts',(40.0406047391561,34.9221084139259,47.8394991116311));
#30620=CARTESIAN_POINT('Ctrl Pts',(40.048829165374,34.9178116960247,47.7591968702359));
#30621=CARTESIAN_POINT('Ctrl Pts',(40.057057704256,34.913512829529,47.6788544733172));
#30622=CARTESIAN_POINT('Ctrl Pts',(40.0694046197622,34.9092139630333,47.5989735871373));
#30623=CARTESIAN_POINT('Ctrl Pts',(40.0857869235253,34.9049150965376,47.5199913776052));
#30624=CARTESIAN_POINT('Ctrl Pts',(40.1021952311961,34.9006094063784,47.4408837982761));
#30625=CARTESIAN_POINT('Ctrl Pts',(40.1226516265555,34.8963037162192,47.362678180888));
#30626=CARTESIAN_POINT('Ctrl Pts',(40.1470224109709,34.89199802606,47.2857994509714));
#30627=CARTESIAN_POINT('Ctrl Pts',(40.1714137197927,34.8876887097666,47.2088559758968));
#30628=CARTESIAN_POINT('Ctrl Pts',(40.1997258277564,34.8833793934732,47.1332420309795));
#30629=CARTESIAN_POINT('Ctrl Pts',(40.2317766603203,34.8790700771798,47.0593629870306));
#30630=CARTESIAN_POINT('Ctrl Pts',(40.2638943265441,34.8747517749302,46.9853298875857));
#30631=CARTESIAN_POINT('Ctrl Pts',(40.2997660943098,34.8704334726805,46.9130393157213));
#30632=CARTESIAN_POINT('Ctrl Pts',(40.3391636555107,34.8661151704309,46.8428725212268));
#30633=CARTESIAN_POINT('Ctrl Pts',(40.3664925959349,34.8631196899667,46.794199860076));
#30634=CARTESIAN_POINT('Ctrl Pts',(40.3955171271908,34.8601242095025,46.7465485590536));
#30635=CARTESIAN_POINT('Ctrl Pts',(40.4261493209387,34.8571287290383,46.7000369475754));
#30636=CARTESIAN_POINT('Ctrl Pts',(40.4694621271366,34.8528932287707,46.6342712231063));
#30637=CARTESIAN_POINT('Ctrl Pts',(40.5161476800916,34.8486577285031,46.5705475402857));
#30638=CARTESIAN_POINT('Ctrl Pts',(40.5659870212995,34.8444222282355,46.5092328032661));
#30639=CARTESIAN_POINT('Ctrl Pts',(40.6157541112821,34.840192868099,46.4480069531532));
#30640=CARTESIAN_POINT('Ctrl Pts',(40.6686656168081,34.8359635079624,46.3891834750637));
#30641=CARTESIAN_POINT('Ctrl Pts',(40.7244590862551,34.8317341478258,46.3331007567142));
#30642=CARTESIAN_POINT('Ctrl Pts',(40.7801874004975,34.827509726705,46.277083531352));
#30643=CARTESIAN_POINT('Ctrl Pts',(40.8387906614109,34.8232853055842,46.2238010364743));
#30644=CARTESIAN_POINT('Ctrl Pts',(40.8999669011061,34.8190608844634,46.1735577909162));
#30645=CARTESIAN_POINT('Ctrl Pts',(40.9611040197523,34.81483916478,46.1233466749641));
#30646=CARTESIAN_POINT('Ctrl Pts',(41.0248104897444,34.8106174450967,46.0761712478957));
#30647=CARTESIAN_POINT('Ctrl Pts',(41.090749221371,34.8063957254133,46.0322975734224));
#30648=CARTESIAN_POINT('Ctrl Pts',(41.1566663781384,34.8021753870578,45.98843825422));
#30649=CARTESIAN_POINT('Ctrl Pts',(41.2248139557738,34.7979550487023,45.9478788022596));
#30650=CARTESIAN_POINT('Ctrl Pts',(41.2948248936639,34.7937347103469,45.9108426518726));
#30651=CARTESIAN_POINT('Ctrl Pts',(41.3648347872325,34.7895144349443,45.873807053937));
#30652=CARTESIAN_POINT('Ctrl Pts',(41.436707570305,34.7852941595416,45.8402948713989));
#30653=CARTESIAN_POINT('Ctrl Pts',(41.5100518639737,34.781073884139,45.810483442382));
#30654=CARTESIAN_POINT('Ctrl Pts',(41.5834695190221,34.7768493874779,45.7806421949914));
#30655=CARTESIAN_POINT('Ctrl Pts',(41.658361189034,34.7726248908168,45.7545092727193));
#30656=CARTESIAN_POINT('Ctrl Pts',(41.7343163639405,34.7684003941556,45.7322134717786));
#30657=CARTESIAN_POINT('Ctrl Pts',(41.8103080047276,34.7641738693247,45.7099069666822));
#30658=CARTESIAN_POINT('Ctrl Pts',(41.887363710503,34.7599473444937,45.6914413623176));
#30659=CARTESIAN_POINT('Ctrl Pts',(41.9650611998378,34.7557208196628,45.6768946039808));
#30660=CARTESIAN_POINT('Ctrl Pts',(42.0429007175777,34.7514865688862,45.6623212546575));
#30661=CARTESIAN_POINT('Ctrl Pts',(42.1213838968034,34.7472523181096,45.651681128974));
#30662=CARTESIAN_POINT('Ctrl Pts',(42.2000819252879,34.743018067333,45.645000381252));
#30663=CARTESIAN_POINT('Ctrl Pts',(42.275139120872,34.7389797070994,45.6386287071697));
#30664=CARTESIAN_POINT('Ctrl Pts',(42.3503913677707,34.7349413468658,45.6358581410795));
#30665=CARTESIAN_POINT('Ctrl Pts',(42.4254689940191,34.7309029866323,45.636667232224));
#30666=CARTESIAN_POINT('Ctrl Pts',(42.5042116735762,34.7266674863681,45.6375158206505));
#30667=CARTESIAN_POINT('Ctrl Pts',(42.5830615660862,34.7224319861039,45.6423057109072));
#30668=CARTESIAN_POINT('Ctrl Pts',(42.6615916401724,34.7181964858398,45.651051244771));
#30669=CARTESIAN_POINT('Ctrl Pts',(42.7400078705775,34.7139671257066,45.6597841003866));
#30670=CARTESIAN_POINT('Ctrl Pts',(42.8181047407343,34.7097377655734,45.6724611605396));
#30671=CARTESIAN_POINT('Ctrl Pts',(42.8954556729822,34.7055084054402,45.6890447609247));
#30672=CARTESIAN_POINT('Ctrl Pts',(42.9727162753786,34.7012839843228,45.7056089951028));
#30673=CARTESIAN_POINT('Ctrl Pts',(43.0492322143667,34.6970595632054,45.726070606033));
#30674=CARTESIAN_POINT('Ctrl Pts',(43.1245840190017,34.692835142088,45.7503403723436));
#30675=CARTESIAN_POINT('Ctrl Pts',(43.1998876375823,34.688613422408,45.7745946185974));
#30676=CARTESIAN_POINT('Ctrl Pts',(43.2740281538242,34.684391702728,45.8026520432908));
#30677=CARTESIAN_POINT('Ctrl Pts',(43.3465994380146,34.680169983048,45.8343730827194));
#30678=CARTESIAN_POINT('Ctrl Pts',(43.4191469772041,34.6759496446959,45.8660837431651));
#30679=CARTESIAN_POINT('Ctrl Pts',(43.4901258741377,34.6717293063438,45.9014554502498));
#30680=CARTESIAN_POINT('Ctrl Pts',(43.5591496376044,34.6675089679917,45.9403003717674));
#30681=CARTESIAN_POINT('Ctrl Pts',(43.6281723714752,34.6632886925924,45.9791447138531));
#30682=CARTESIAN_POINT('Ctrl Pts',(43.6952396214777,34.6590684171932,46.0214619360348));
#30683=CARTESIAN_POINT('Ctrl Pts',(43.7599905086148,34.6548481417939,46.0670188160829));
#30684=CARTESIAN_POINT('Ctrl Pts',(43.8248061617241,34.650623645136,46.1126212636244));
#30685=CARTESIAN_POINT('Ctrl Pts',(43.8873004388834,34.6463991484782,46.161469571445));
#30686=CARTESIAN_POINT('Ctrl Pts',(43.94714293641,34.6421746518203,46.2132881667105));
#30687=CARTESIAN_POINT('Ctrl Pts',(44.0070141641634,34.6379481269926,46.2651316399483));
#30688=CARTESIAN_POINT('Ctrl Pts',(44.064230736708,34.6337216021649,46.3199479163091));
#30689=CARTESIAN_POINT('Ctrl Pts',(44.1184986492037,34.6294950773373,46.3774240130012));
#30690=CARTESIAN_POINT('Ctrl Pts',(44.1728657616248,34.6252608265638,46.4350051740719));
#30691=CARTESIAN_POINT('Ctrl Pts',(44.224273137964,34.6210265757904,46.4952555130286));
#30692=CARTESIAN_POINT('Ctrl Pts',(44.2724667979375,34.616792325017,46.5578285360188));
#30693=CARTESIAN_POINT('Ctrl Pts',(44.3184308590675,34.6127539647535,46.6175067230539));
#30694=CARTESIAN_POINT('Ctrl Pts',(44.361471808364,34.60871560449,46.6792971225263));
#30695=CARTESIAN_POINT('Ctrl Pts',(44.4014076971255,34.6046772442265,46.7428772252533));
#30696=CARTESIAN_POINT('Ctrl Pts',(44.4432931299291,34.600441743961,46.8095611079214));
#30697=CARTESIAN_POINT('Ctrl Pts',(44.4819218185688,34.5962062436954,46.8784673704397));
#30698=CARTESIAN_POINT('Ctrl Pts',(44.5170506808672,34.5919707434299,46.9492446262141));
#30699=CARTESIAN_POINT('Ctrl Pts',(44.5521286174653,34.5877413832954,47.0199192774328));
#30700=CARTESIAN_POINT('Ctrl Pts',(44.5837165961697,34.5835120231609,47.0924591188066));
#30701=CARTESIAN_POINT('Ctrl Pts',(44.6116155188343,34.5792826630264,47.1664850104819));
#30702=CARTESIAN_POINT('Ctrl Pts',(44.6394818613413,34.5750582419077,47.2404244552629));
#30703=CARTESIAN_POINT('Ctrl Pts',(44.6636675440464,34.570833820789,47.3158460648713));
#30704=CARTESIAN_POINT('Ctrl Pts',(44.6840206744163,34.5666093996702,47.3923487844667));
#30705=CARTESIAN_POINT('Ctrl Pts',(44.7043607893438,34.562387679989,47.4688025820186));
#30706=CARTESIAN_POINT('Ctrl Pts',(44.720873095994,34.5581659603078,47.546335665028));
#30707=CARTESIAN_POINT('Ctrl Pts',(44.7334552586409,34.5539442406265,47.6245309642312));
#30708=CARTESIAN_POINT('Ctrl Pts',(44.7460333044602,34.5497239022732,47.7027006782804));
#30709=CARTESIAN_POINT('Ctrl Pts',(44.7546836851917,34.5455035639199,47.78153171524));
#30710=CARTESIAN_POINT('Ctrl Pts',(44.7593552845364,34.5412832255665,47.8605974095289));
#30711=CARTESIAN_POINT('Ctrl Pts',(44.764026814197,34.5370629501661,47.9396619244302));
#30712=CARTESIAN_POINT('Ctrl Pts',(44.7647196540934,34.5328426747656,48.0189606210902));
#30713=CARTESIAN_POINT('Ctrl Pts',(44.7614347182004,34.5286223993652,48.0980638189019));
#30714=CARTESIAN_POINT('Ctrl Pts',(44.7581464966063,34.5243979027062,48.1772461383392));
#30715=CARTESIAN_POINT('Ctrl Pts',(44.7508725707835,34.5201734060472,48.2562320982361));
#30716=CARTESIAN_POINT('Ctrl Pts',(44.7396659596394,34.5159489093882,48.3345947372639));
#30717=CARTESIAN_POINT('Ctrl Pts',(44.7284539682306,34.5117223845594,48.4129949979896));
#30718=CARTESIAN_POINT('Ctrl Pts',(44.7133056200825,34.5074958597306,48.4907708803665));
#30719=CARTESIAN_POINT('Ctrl Pts',(44.6943250883908,34.5032693349019,48.5675057970456));
#30720=CARTESIAN_POINT('Ctrl Pts',(44.6753098609236,34.4990350841274,48.6443809825796));
#30721=CARTESIAN_POINT('Ctrl Pts',(44.6524485879072,34.4948008333529,48.7202109495185));
#30722=CARTESIAN_POINT('Ctrl Pts',(44.6258952792242,34.4905665825785,48.7945946430902));
#30723=CARTESIAN_POINT('Ctrl Pts',(44.6005704149039,34.4865282223258,48.8655370996341));
#30724=CARTESIAN_POINT('Ctrl Pts',(44.5718877420354,34.4824898620732,48.9351638260439));
#30725=CARTESIAN_POINT('Ctrl Pts',(44.5400200671921,34.4784515018206,49.0031473236345));
#30726=CARTESIAN_POINT('Ctrl Pts',(44.5065967128721,34.4742160015445,49.0744495613741));
#30727=CARTESIAN_POINT('Ctrl Pts',(44.4695424038322,34.4699805012685,49.1442150744385));
#30728=CARTESIAN_POINT('Ctrl Pts',(44.429021160673,34.4657450009925,49.212049326736));
#30729=CARTESIAN_POINT('Ctrl Pts',(44.3885586604541,34.4615156408474,49.2797852408997));
#30730=CARTESIAN_POINT('Ctrl Pts',(44.3446394454327,34.4572862807023,49.3455950545097));
#30731=CARTESIAN_POINT('Ctrl Pts',(44.2974746724665,34.4530569205573,49.4091062090021));
#30732=CARTESIAN_POINT('Ctrl Pts',(44.2503649781762,34.4488324994279,49.472543195634));
#30733=CARTESIAN_POINT('Ctrl Pts',(44.2000175360269,34.4446080782986,49.5336864826118));
#30734=CARTESIAN_POINT('Ctrl Pts',(44.1466874718296,34.4403836571693,49.5921913567953));
#30735=CARTESIAN_POINT('Ctrl Pts',(44.0933915112003,34.4361619374775,49.6506588182176));
#30736=CARTESIAN_POINT('Ctrl Pts',(44.0371170294983,34.4319402177856,49.7064908696767));
#30737=CARTESIAN_POINT('Ctrl Pts',(43.9781594309252,34.4277184980938,49.7593758130319));
#30738=CARTESIAN_POINT('Ctrl Pts',(43.9192211230161,34.4234981597298,49.812243452669));
#30739=CARTESIAN_POINT('Ctrl Pts',(43.8576017905845,34.4192778213659,49.8621655857811));
#30740=CARTESIAN_POINT('Ctrl Pts',(43.7936326178781,34.4150574830019,49.9088683996772));
#30741=CARTESIAN_POINT('Ctrl Pts',(43.729664399371,34.4108372075909,49.9555705169285));
#30742=CARTESIAN_POINT('Ctrl Pts',(43.6633467901245,34.4066169321798,49.9990531347413));
#30743=CARTESIAN_POINT('Ctrl Pts',(43.5950416580426,34.4023966567687,50.039084568242));
#30744=CARTESIAN_POINT('Ctrl Pts',(43.5266682049184,34.3981721600992,50.0791560425008));
#30745=CARTESIAN_POINT('Ctrl Pts',(43.456303663607,34.3939476634297,50.1157691987805));
#30746=CARTESIAN_POINT('Ctrl Pts',(43.3843358033486,34.3897231667602,50.1487376450247));
#30747=CARTESIAN_POINT('Ctrl Pts',(43.3123333915096,34.385496641921,50.1817219193332));
#30748=CARTESIAN_POINT('Ctrl Pts',(43.2387265638878,34.3812701170817,50.2110578237531));
#30749=CARTESIAN_POINT('Ctrl Pts',(43.1639220389498,34.3770435922425,50.2366076006548));
#30750=CARTESIAN_POINT('Ctrl Pts',(43.0889807738518,34.3728093414577,50.2622040816908));
#30751=CARTESIAN_POINT('Ctrl Pts',(43.0128378890165,34.368575090673,50.2840004760918));
#30752=CARTESIAN_POINT('Ctrl Pts',(42.9359140008011,34.3643408398882,50.3019093432725));
#30753=CARTESIAN_POINT('Ctrl Pts',(42.8625488693661,34.3603024797304,50.3189896862589));
#30754=CARTESIAN_POINT('Ctrl Pts',(42.7884737580912,34.3562641195726,50.3325342193753));
#30755=CARTESIAN_POINT('Ctrl Pts',(42.7140575894208,34.3522257594148,50.3425111038002));
#30756=CARTESIAN_POINT('Ctrl Pts',(42.6360086565505,34.3479902591667,50.3529750284639));
#30757=CARTESIAN_POINT('Ctrl Pts',(42.5572878366582,34.3437547589187,50.3595538633806));
#30758=CARTESIAN_POINT('Ctrl Pts',(42.4783156794139,34.3395192586706,50.3621721138092));
#30759=CARTESIAN_POINT('Ctrl Pts',(42.399458006731,34.3352898985536,50.3647865686058));
#30760=CARTESIAN_POINT('Ctrl Pts',(42.3203501853755,34.3310605384365,50.3634518252778));
#30761=CARTESIAN_POINT('Ctrl Pts',(42.2414197816143,34.3268311783194,50.3581439216547));
#30762=CARTESIAN_POINT('Ctrl Pts',(42.1625815521981,34.322606757218,50.3528422165623));
#30763=CARTESIAN_POINT('Ctrl Pts',(42.0839207945184,34.3183823361165,50.3435766027034));
#30764=CARTESIAN_POINT('Ctrl Pts',(42.0058654428886,34.3141579150151,50.3303751611684));
#30765=CARTESIAN_POINT('Ctrl Pts',(41.9278600061794,34.309936195351,50.3171821617055));
#30766=CARTESIAN_POINT('Ctrl Pts',(41.8504596686479,34.3057144756869,50.3000584081078));
#30767=CARTESIAN_POINT('Ctrl Pts',(41.7740863883335,34.3014927560229,50.2790837175564));
#30768=CARTESIAN_POINT('Ctrl Pts',(41.6977380970143,34.2972724176865,50.2581158898298));
#30769=CARTESIAN_POINT('Ctrl Pts',(41.6224166478823,34.2930520793503,50.2332997513138));
#30770=CARTESIAN_POINT('Ctrl Pts',(41.5485314929506,34.288831741014,50.2047657069183));
#30771=CARTESIAN_POINT('Ctrl Pts',(41.4746474401278,34.2846114656304,50.1762320881513));
#30772=CARTESIAN_POINT('Ctrl Pts',(41.4022000762725,34.2803911902468,50.1439808440776));
#30773=CARTESIAN_POINT('Ctrl Pts',(41.3315800223182,34.2761709148632,50.1081909762141));
#30774=CARTESIAN_POINT('Ctrl Pts',(41.2608893318526,34.2719464182208,50.0723653101422));
#30775=CARTESIAN_POINT('Ctrl Pts',(41.1920300220774,34.2677219215783,50.0329941624658));
#30776=CARTESIAN_POINT('Ctrl Pts',(41.1253686337984,34.2634974249359,49.9903028214809));
#30777=CARTESIAN_POINT('Ctrl Pts',(41.0586752415587,34.2592709001235,49.9475909844933));
#30778=CARTESIAN_POINT('Ctrl Pts',(40.9941822554756,34.2550443753111,49.9015560517779));
#30779=CARTESIAN_POINT('Ctrl Pts',(40.9322255648067,34.2508178504987,49.8524655592731));
#30780=CARTESIAN_POINT('Ctrl Pts',(40.870155619377,34.2465835997401,49.8032853309879));
#30781=CARTESIAN_POINT('Ctrl Pts',(40.8106315873747,34.2423493489816,49.7510386922827));
#30782=CARTESIAN_POINT('Ctrl Pts',(40.7539545586514,34.238115098223,49.6960320887045));
#30783=CARTESIAN_POINT('Ctrl Pts',(40.6998995955178,34.2340767378183,49.6435702713599));
#30784=CARTESIAN_POINT('Ctrl Pts',(40.6484342549836,34.2300383774136,49.5885984976851));
#30785=CARTESIAN_POINT('Ctrl Pts',(40.5997848983345,34.2260000170089,49.5314098173367));
#30786=CARTESIAN_POINT('Ctrl Pts',(40.5491120042058,34.2217936837019,49.4718424120461));
#30787=CARTESIAN_POINT('Ctrl Pts',(40.5012948400351,34.2175873503948,49.4096347864003));
#30788=CARTESIAN_POINT('Ctrl Pts',(40.4566233196973,34.2133810170877,49.3450938700907));
#30789=CARTESIAN_POINT('Ctrl Pts',(40.4120127572409,34.2091804236607,49.2806410250509));
#30790=CARTESIAN_POINT('Ctrl Pts',(40.3705395910079,34.2049798302336,49.213861593386));
#30791=CARTESIAN_POINT('Ctrl Pts',(40.3324545938023,34.2007792368066,49.1450966920792));
#30792=CARTESIAN_POINT('Ctrl Pts',(40.2944092730564,34.1965830195037,49.0764034291612));
#30793=CARTESIAN_POINT('Ctrl Pts',(40.2597453453305,34.1923868022008,49.0057292157322));
#30794=CARTESIAN_POINT('Ctrl Pts',(40.2286703096372,34.1881905848979,48.9334440618746));
#30795=CARTESIAN_POINT('Ctrl Pts',(40.197049657644,34.1839206903004,48.8598897233707));
#30796=CARTESIAN_POINT('Ctrl Pts',(40.1691454159207,34.179650795703,48.7846677500641));
#30797=CARTESIAN_POINT('Ctrl Pts',(40.1451269353427,34.1753809011055,48.7081934080342));
#30798=CARTESIAN_POINT('Ctrl Pts',(40.121545235019,34.1711886552853,48.6331097652391));
#30799=CARTESIAN_POINT('Ctrl Pts',(40.1017092685791,34.1669964094651,48.5568194022073));
#30800=CARTESIAN_POINT('Ctrl Pts',(40.0857297276285,34.1628041636449,48.4797327874113));
#30801=CARTESIAN_POINT('Ctrl Pts',(40.0693062270907,34.1584954446588,48.4005044751918));
#30802=CARTESIAN_POINT('Ctrl Pts',(40.0569567714156,34.1541867256727,48.3204355148518));
#30803=CARTESIAN_POINT('Ctrl Pts',(40.0487453046816,34.1498780066866,48.2399829132314));
#30804=CARTESIAN_POINT('Ctrl Pts',(40.0405338379475,34.1455692877005,48.1595303116111));
#30805=CARTESIAN_POINT('Ctrl Pts',(40.0364603855593,34.1412605687144,48.0786946135994));
#30806=CARTESIAN_POINT('Ctrl Pts',(40.0365309009766,34.1369518497283,47.9979362990588));
#30807=CARTESIAN_POINT('',(40.0365300017577,33.3432018497554,47.9999088486209));
#30808=CARTESIAN_POINT('Ctrl Pts',(40.0365309009773,34.1369518496884,47.9979362983109));
#30809=CARTESIAN_POINT('Ctrl Pts',(40.0366146349956,34.1318354334801,47.9020393157517));
#30810=CARTESIAN_POINT('Ctrl Pts',(40.0425386403499,34.1267190172719,47.8063991429868));
#30811=CARTESIAN_POINT('Ctrl Pts',(40.054186890387,34.1216026010636,47.711640336268));
#30812=CARTESIAN_POINT('Ctrl Pts',(40.066007939675,34.1164102839359,47.6154758033015));
#30813=CARTESIAN_POINT('Ctrl Pts',(40.0837242615162,34.1112179668082,47.5202189535493));
#30814=CARTESIAN_POINT('Ctrl Pts',(40.10716584825,34.1060256496804,47.4265002236539));
#30815=CARTESIAN_POINT('Ctrl Pts',(40.1165734754215,34.103941857988,47.388888824739));
#30816=CARTESIAN_POINT('Ctrl Pts',(40.1269026727228,34.1018580662955,47.3515249082308));
#30817=CARTESIAN_POINT('Ctrl Pts',(40.1381403134859,34.0997742746031,47.3144482518275));
#30818=CARTESIAN_POINT('Ctrl Pts',(40.1609818630579,34.095538774266,47.2390865008115));
#30819=CARTESIAN_POINT('Ctrl Pts',(40.1876373614446,34.0913032739288,47.1647243248294));
#30820=CARTESIAN_POINT('Ctrl Pts',(40.21800112357,34.0870677735917,47.0917757192421));
#30821=CARTESIAN_POINT('Ctrl Pts',(40.248320867881,34.0828384133853,47.0189328659713));
#30822=CARTESIAN_POINT('Ctrl Pts',(40.2823380216964,34.0786090531788,46.9474999433386));
#30823=CARTESIAN_POINT('Ctrl Pts',(40.3198970969558,34.0743796929724,46.8778759633413));
#30824=CARTESIAN_POINT('Ctrl Pts',(40.357412311004,34.0701552717816,46.8083332897146));
#30825=CARTESIAN_POINT('Ctrl Pts',(40.3984610053576,34.0659308505909,46.7405957717856));
#30826=CARTESIAN_POINT('Ctrl Pts',(40.4428401811182,34.0617064294001,46.6750411763929));
#30827=CARTESIAN_POINT('Ctrl Pts',(40.4871909772354,34.0574847096467,46.6095285019236));
#30828=CARTESIAN_POINT('Ctrl Pts',(40.5348677651948,34.0532629898934,46.546196366967));
#30829=CARTESIAN_POINT('Ctrl Pts',(40.5856229454918,34.0490412701401,46.4853956473804));
#30830=CARTESIAN_POINT('Ctrl Pts',(40.6363615189194,34.0448209317146,46.424614821519));
#30831=CARTESIAN_POINT('Ctrl Pts',(40.690176184096,34.0406005932892,46.366364126399));
#30832=CARTESIAN_POINT('Ctrl Pts',(40.7467784934986,34.0363802548638,46.3109620811417));
#30833=CARTESIAN_POINT('Ctrl Pts',(40.803379958588,34.0321599793915,46.2555608622936));
#30834=CARTESIAN_POINT('Ctrl Pts',(40.8627686488952,34.0279397039191,46.2030085361961));
#30835=CARTESIAN_POINT('Ctrl Pts',(40.9246197034793,34.0237194284467,46.1535863352059));
#30836=CARTESIAN_POINT('Ctrl Pts',(40.9865326235147,34.0194949317165,46.104114700511));
#30837=CARTESIAN_POINT('Ctrl Pts',(41.0509124603078,34.0152704349864,46.057779738888));
#30838=CARTESIAN_POINT('Ctrl Pts',(41.1174022179446,34.0110459382562,46.014821577196));
#30839=CARTESIAN_POINT('Ctrl Pts',(41.1839238971349,34.0068194133565,45.9718427914063));
#30840=CARTESIAN_POINT('Ctrl Pts',(41.252557108026,34.0025928884568,45.9322442700401));
#30841=CARTESIAN_POINT('Ctrl Pts',(41.3229191201371,33.9983663635571,45.8962207294648));
#30842=CARTESIAN_POINT('Ctrl Pts',(41.3934097516231,33.9941321127131,45.8601313390775));
#30843=CARTESIAN_POINT('Ctrl Pts',(41.4656350699925,33.989897861869,45.8276301809428));
#30844=CARTESIAN_POINT('Ctrl Pts',(41.5391913676716,33.985663611025,45.7988641706135));
#30845=CARTESIAN_POINT('Ctrl Pts',(41.6093446940789,33.9816252514158,45.7714289764053));
#30846=CARTESIAN_POINT('Ctrl Pts',(41.6807082215308,33.9775868918065,45.7473910500946));
#30847=CARTESIAN_POINT('Ctrl Pts',(41.7529214193359,33.9735485321973,45.7268348605203));
#30848=CARTESIAN_POINT('Ctrl Pts',(41.82865984706,33.9693130320853,45.70527517994));
#30849=CARTESIAN_POINT('Ctrl Pts',(41.9056209179429,33.9650775319733,45.6874638985284));
#30850=CARTESIAN_POINT('Ctrl Pts',(41.9833992755834,33.9608420318614,45.6735361001478));
#30851=CARTESIAN_POINT('Ctrl Pts',(42.061064879291,33.9566126718803,45.6596284926543));
#30852=CARTESIAN_POINT('Ctrl Pts',(42.1395449588451,33.9523833118992,45.6495932703991));
#30853=CARTESIAN_POINT('Ctrl Pts',(42.2184198162798,33.9481539519181,45.6435155256654));
#30854=CARTESIAN_POINT('Ctrl Pts',(42.2972025642471,33.9439295309519,45.6374448784764));
#30855=CARTESIAN_POINT('Ctrl Pts',(42.3763787084319,33.9397051099857,45.6353225608754));
#30856=CARTESIAN_POINT('Ctrl Pts',(42.4555207156813,33.9354806890195,45.6371822137477));
#30857=CARTESIAN_POINT('Ctrl Pts',(42.5346121131225,33.9312589694902,45.6390406774074));
#30858=CARTESIAN_POINT('Ctrl Pts',(42.6136689490017,33.9270372499608,45.6448760464962));
#30859=CARTESIAN_POINT('Ctrl Pts',(42.6922621776862,33.9228155304315,45.6546699037462));
#30860=CARTESIAN_POINT('Ctrl Pts',(42.7708296910304,33.9185951922292,45.6644605564914));
#30861=CARTESIAN_POINT('Ctrl Pts',(42.8489334329895,33.9143748540269,45.6782070675668));
#30862=CARTESIAN_POINT('Ctrl Pts',(42.9261494724226,33.9101545158247,45.6958391606554));
#30863=CARTESIAN_POINT('Ctrl Pts',(43.0033643600774,33.9059342405743,45.7134709907382));
#30864=CARTESIAN_POINT('Ctrl Pts',(43.0796911142504,33.9017139653239,45.7349881818388));
#30865=CARTESIAN_POINT('Ctrl Pts',(43.1547174636666,33.8974936900734,45.7602696611117));
#30866=CARTESIAN_POINT('Ctrl Pts',(43.2298188569599,33.8932691935618,45.7855764277702));
#30867=CARTESIAN_POINT('Ctrl Pts',(43.303616801326,33.8890446970502,45.8146548537638));
#30868=CARTESIAN_POINT('Ctrl Pts',(43.3757162116203,33.8848202005386,45.8473346021081));
#30869=CARTESIAN_POINT('Ctrl Pts',(43.4478502366745,33.8805936758561,45.8800300399238));
#30870=CARTESIAN_POINT('Ctrl Pts',(43.5182836853803,33.8763671511735,45.9163300291294));
#30871=CARTESIAN_POINT('Ctrl Pts',(43.586645741911,33.8721406264909,45.9560180225588));
#30872=CARTESIAN_POINT('Ctrl Pts',(43.6551327620544,33.8679063758588,45.9957785643475));
#30873=CARTESIAN_POINT('Ctrl Pts',(43.7215404292606,33.8636721252268,46.0389392293035));
#30874=CARTESIAN_POINT('Ctrl Pts',(43.7855267811018,33.8594378745947,46.0852399681031));
#30875=CARTESIAN_POINT('Ctrl Pts',(43.8465529339506,33.8553995129936,46.1293986969836));
#30876=CARTESIAN_POINT('Ctrl Pts',(43.9053765954837,33.8513611513925,46.1764131347739));
#30877=CARTESIAN_POINT('Ctrl Pts',(43.9617316806105,33.8473227897913,46.2260257615519));
#30878=CARTESIAN_POINT('Ctrl Pts',(44.0208378242783,33.8430872894733,46.2780603035899));
#30879=CARTESIAN_POINT('Ctrl Pts',(44.0774528983318,33.8388517891552,46.333150975109));
#30880=CARTESIAN_POINT('Ctrl Pts',(44.1312439990707,33.8346162888371,46.3910299391904));
#30881=CARTESIAN_POINT('Ctrl Pts',(44.1849571197706,33.8303869286515,46.4488249971272));
#30882=CARTESIAN_POINT('Ctrl Pts',(44.2358540800347,33.8261575684658,46.5093999797577));
#30883=CARTESIAN_POINT('Ctrl Pts',(44.2836362618204,33.8219282082801,46.5724479434868));
#30884=CARTESIAN_POINT('Ctrl Pts',(44.331362643899,33.8177037871125,46.6354222802323));
#30885=CARTESIAN_POINT('Ctrl Pts',(44.3759811937051,33.8134793659449,46.7008634871008));
#30886=CARTESIAN_POINT('Ctrl Pts',(44.4172323264973,33.8092549447773,46.7684301961179));
#30887=CARTESIAN_POINT('Ctrl Pts',(44.4584570799563,33.8050332250486,46.8359536974794));
#30888=CARTESIAN_POINT('Ctrl Pts',(44.4963184465296,33.8008115053199,46.9055996037187));
#30889=CARTESIAN_POINT('Ctrl Pts',(44.5305998056052,33.7965897855912,46.9769971118051));
#30890=CARTESIAN_POINT('Ctrl Pts',(44.564869947961,33.7923694471918,47.0483712589203));
#30891=CARTESIAN_POINT('Ctrl Pts',(44.5955622057589,33.7881491087924,47.1214954470759));
#30892=CARTESIAN_POINT('Ctrl Pts',(44.6225063401989,33.7839287703931,47.1959751193679));
#30893=CARTESIAN_POINT('Ctrl Pts',(44.6494500727158,33.7797084949481,47.2704536806535));
#30894=CARTESIAN_POINT('Ctrl Pts',(44.672645634599,33.7754882195031,47.3462872440715));
#30895=CARTESIAN_POINT('Ctrl Pts',(44.6919718162422,33.7712679440581,47.4230635785016));
#30896=CARTESIAN_POINT('Ctrl Pts',(44.7113173285569,33.7670434473573,47.4999167071025));
#30897=CARTESIAN_POINT('Ctrl Pts',(44.7267856144159,33.7628189506564,47.5777140342167));
#30898=CARTESIAN_POINT('Ctrl Pts',(44.7383061942865,33.7585944539556,47.6560311312614));
#30899=CARTESIAN_POINT('Ctrl Pts',(44.7498323051536,33.7543679290863,47.7343858281133));
#30900=CARTESIAN_POINT('Ctrl Pts',(44.7574068894699,33.7501414042171,47.8132603241657));
#30901=CARTESIAN_POINT('Ctrl Pts',(44.7610114612567,33.7459148793478,47.8922256026953));
#30902=CARTESIAN_POINT('Ctrl Pts',(44.7646226220774,33.7416806285357,47.9713352270527));
#30903=CARTESIAN_POINT('Ctrl Pts',(44.764249271304,33.7374463777236,48.050535494908));
#30904=CARTESIAN_POINT('Ctrl Pts',(44.7599251189361,33.7332121269114,48.129398121757));
#30905=CARTESIAN_POINT('Ctrl Pts',(44.7558010166928,33.7291737670695,48.2046122929127));
#30906=CARTESIAN_POINT('Ctrl Pts',(44.7480836571655,33.7251354072275,48.2795190215198));
#30907=CARTESIAN_POINT('Ctrl Pts',(44.7368456719384,33.7210970473855,48.3537552069477));
#30908=CARTESIAN_POINT('Ctrl Pts',(44.725059081124,33.7168615466212,48.431615385938));
#30909=CARTESIAN_POINT('Ctrl Pts',(44.70935455133,33.7126260458568,48.5090338451429));
#30910=CARTESIAN_POINT('Ctrl Pts',(44.6897772429322,33.7083905450925,48.5855857056399));
#30911=CARTESIAN_POINT('Ctrl Pts',(44.6702283154024,33.7041611844565,48.6620265902968));
#30912=CARTESIAN_POINT('Ctrl Pts',(44.6468178735759,33.6999318238206,48.7376029201498));
#30913=CARTESIAN_POINT('Ctrl Pts',(44.6196425158882,33.6957024631847,48.8118974951072));
#30914=CARTESIAN_POINT('Ctrl Pts',(44.5924988933709,33.6914780415631,48.8861053094407));
#30915=CARTESIAN_POINT('Ctrl Pts',(44.5615992523267,33.6872536199415,48.9590339048458));
#30916=CARTESIAN_POINT('Ctrl Pts',(44.5270902597421,33.6830291983198,49.0302802860436));
#30917=CARTESIAN_POINT('Ctrl Pts',(44.4926033349979,33.678807478135,49.1014811065443));
#30918=CARTESIAN_POINT('Ctrl Pts',(44.4545118438668,33.6745857579502,49.1710014266907));
#30919=CARTESIAN_POINT('Ctrl Pts',(44.4130104522693,33.6703640377653,49.2384584611341));
#30920=CARTESIAN_POINT('Ctrl Pts',(44.3715226397408,33.6661436989083,49.3058934239387));
#30921=CARTESIAN_POINT('Ctrl Pts',(44.3266273879185,33.6619233600514,49.3712660421081));
#30922=CARTESIAN_POINT('Ctrl Pts',(44.2785644325601,33.6577030211944,49.4342196880604));
#30923=CARTESIAN_POINT('Ctrl Pts',(44.2305021941429,33.653482745291,49.4971723949515));
#30924=CARTESIAN_POINT('Ctrl Pts',(44.1792726319915,33.6492624693877,49.5577058291042));
#30925=CARTESIAN_POINT('Ctrl Pts',(44.1251568707502,33.6450421934843,49.6154950362671));
#30926=CARTESIAN_POINT('Ctrl Pts',(44.0709869812064,33.6408176963269,49.6733420460295));
#30927=CARTESIAN_POINT('Ctrl Pts',(44.0139254472705,33.6365931991696,49.7284390021823));
#30928=CARTESIAN_POINT('Ctrl Pts',(43.9542910965313,33.6323687020123,49.7804970171678));
#30929=CARTESIAN_POINT('Ctrl Pts',(43.8946281155237,33.6281421766868,49.8325800250463));
#30930=CARTESIAN_POINT('Ctrl Pts',(43.8323902262042,33.6239156513614,49.8816208943922));
#30931=CARTESIAN_POINT('Ctrl Pts',(43.7679282429864,33.619689126036,49.9273719835414));
#30932=CARTESIAN_POINT('Ctrl Pts',(43.7033484255725,33.6154548747737,49.9732067040425));
#30933=CARTESIAN_POINT('Ctrl Pts',(43.6365367872811,33.6112206235114,50.0157393750479));
#30934=CARTESIAN_POINT('Ctrl Pts',(43.5678717642886,33.6069863722491,50.0547666493005));
#30935=CARTESIAN_POINT('Ctrl Pts',(43.5023834940629,33.6029480164926,50.091988346331));
#30936=CARTESIAN_POINT('Ctrl Pts',(43.4352098736056,33.5989096607361,50.1260216957278));
#30937=CARTESIAN_POINT('Ctrl Pts',(43.3666955727028,33.5948713049797,50.1567313487351));
#30938=CARTESIAN_POINT('Ctrl Pts',(43.2948365613139,33.5906358059894,50.1889401763247));
#30939=CARTESIAN_POINT('Ctrl Pts',(43.221229477731,33.5864003069991,50.2176149438563));
#30940=CARTESIAN_POINT('Ctrl Pts',(43.1462560880774,33.5821648080087,50.242563776553));
#30941=CARTESIAN_POINT('Ctrl Pts',(43.0713913860735,33.5779354491494,50.2674764413506));
#30942=CARTESIAN_POINT('Ctrl Pts',(42.995164752915,33.57370609029,50.2886737506457));
#30943=CARTESIAN_POINT('Ctrl Pts',(42.9179793241891,33.5694767314307,50.3060112446848));
#30944=CARTESIAN_POINT('Ctrl Pts',(42.8408840319596,33.5652523115811,50.3233284921437));
#30945=CARTESIAN_POINT('Ctrl Pts',(42.7628326247246,33.5610278917316,50.3367947791789));
#30946=CARTESIAN_POINT('Ctrl Pts',(42.6842433781053,33.556803471882,50.3463154397701));
#30947=CARTESIAN_POINT('Ctrl Pts',(42.6057043877616,33.5525817534658,50.3558300120862));
#30948=CARTESIAN_POINT('Ctrl Pts',(42.5266287053627,33.5483600350495,50.3614039095781));
#30949=CARTESIAN_POINT('Ctrl Pts',(42.4474435764409,33.5441383166333,50.3629937680736));
#30950=CARTESIAN_POINT('Ctrl Pts',(42.3682843564389,33.5399179795391,50.3645831063765));
#30951=CARTESIAN_POINT('Ctrl Pts',(42.2890162299233,33.5356976424449,50.3621909846959));
#30952=CARTESIAN_POINT('Ctrl Pts',(42.2100688254176,33.5314773053507,50.355826094987));
#30953=CARTESIAN_POINT('Ctrl Pts',(42.1311225983941,33.5272570312019,50.3494613002089));
#30954=CARTESIAN_POINT('Ctrl Pts',(42.0524975515986,33.523036757053,50.3391238942317));
#30955=CARTESIAN_POINT('Ctrl Pts',(41.9746190664326,33.5188164829042,50.3248745132281));
#30956=CARTESIAN_POINT('Ctrl Pts',(41.8966626842367,33.5145919874762,50.3106108794502));
#30957=CARTESIAN_POINT('Ctrl Pts',(41.8194548181666,33.5103674920483,50.2924275387982));
#30958=CARTESIAN_POINT('Ctrl Pts',(41.7434109134956,33.5061429966203,50.2704363484545));
#30959=CARTESIAN_POINT('Ctrl Pts',(41.6673305001692,33.5019164730134,50.248434600147));
#30960=CARTESIAN_POINT('Ctrl Pts',(41.5924156058328,33.4976899494065,50.2226215133649));
#30961=CARTESIAN_POINT('Ctrl Pts',(41.5190642913965,33.4934634257996,50.1931581607826));
#30962=CARTESIAN_POINT('Ctrl Pts',(41.4455788926556,33.4892291762169,50.1636409499542));
#30963=CARTESIAN_POINT('Ctrl Pts',(41.3736632124349,33.4849949266342,50.1304603370704));
#30964=CARTESIAN_POINT('Ctrl Pts',(41.3036930019361,33.4807606770515,50.093824588378));
#30965=CARTESIAN_POINT('Ctrl Pts',(41.2369596415406,33.4767223055589,50.0588836241673));
#30966=CARTESIAN_POINT('Ctrl Pts',(41.1719960242722,33.4726839340663,50.0208003394924));
#30967=CARTESIAN_POINT('Ctrl Pts',(41.1091024491847,33.4686455625738,49.9797913915863));
#30968=CARTESIAN_POINT('Ctrl Pts',(41.0432115943436,33.4644147369379,49.9368281059103));
#30969=CARTESIAN_POINT('Ctrl Pts',(40.9793413080481,33.4601839113021,49.8904892083675));
#30970=CARTESIAN_POINT('Ctrl Pts',(40.9178590231447,33.4559530856662,49.8409911910779));
#30971=CARTESIAN_POINT('Ctrl Pts',(40.8564659153205,33.4517283966382,49.7915649682672));
#30972=CARTESIAN_POINT('Ctrl Pts',(40.7974542944261,33.4475037076102,49.7389890170494));
#30973=CARTESIAN_POINT('Ctrl Pts',(40.7411633225029,33.4432790185822,49.683523483142));
#30974=CARTESIAN_POINT('Ctrl Pts',(40.684937948313,33.4390592527242,49.6281225850575));
#30975=CARTESIAN_POINT('Ctrl Pts',(40.631427256575,33.4348394868662,49.569839123921));
#30976=CARTESIAN_POINT('Ctrl Pts',(40.58093675295,33.4306197210082,49.5089729434724));
#30977=CARTESIAN_POINT('Ctrl Pts',(40.5304783742662,33.4264026400061,49.4481454895631));
#30978=CARTESIAN_POINT('Ctrl Pts',(40.4830366695324,33.4221855590041,49.3847389388626));
#30979=CARTESIAN_POINT('Ctrl Pts',(40.4388788661868,33.4179684780021,49.3190884501849));
#30980=CARTESIAN_POINT('Ctrl Pts',(40.3947352858967,33.4137527553053,49.2534591072724));
#30981=CARTESIAN_POINT('Ctrl Pts',(40.3538737691867,33.4095370326085,49.1855876516346));
#30982=CARTESIAN_POINT('Ctrl Pts',(40.3165190562355,33.4053213099118,49.1158394140154));
#30983=CARTESIAN_POINT('Ctrl Pts',(40.2791646398873,33.4011056206886,49.0460917302095));
#30984=CARTESIAN_POINT('Ctrl Pts',(40.2453171927927,33.3968899314654,48.9744677095271));
#30985=CARTESIAN_POINT('Ctrl Pts',(40.2151554674143,33.3926742422422,48.9013572040709));
#30986=CARTESIAN_POINT('Ctrl Pts',(40.1849635162688,33.3884543283787,48.8281734328751));
#30987=CARTESIAN_POINT('Ctrl Pts',(40.1584648442828,33.3842344145152,48.7535006374389));
#30988=CARTESIAN_POINT('Ctrl Pts',(40.1357897395433,33.3800145006517,48.6777479895525));
#30989=CARTESIAN_POINT('Ctrl Pts',(40.1131035277608,33.3757925197299,48.6019582354247));
#30990=CARTESIAN_POINT('Ctrl Pts',(40.0942447258862,33.371570538808,48.5250880328208));
#30991=CARTESIAN_POINT('Ctrl Pts',(40.0792928199903,33.3673485578862,48.4475585163433));
#30992=CARTESIAN_POINT('Ctrl Pts',(40.064313858222,33.3631189371773,48.3698887081383));
#30993=CARTESIAN_POINT('Ctrl Pts',(40.0532559831891,33.3588893164684,48.2915576693378));
#30994=CARTESIAN_POINT('Ctrl Pts',(40.0461469170547,33.3546596957595,48.2129932036679));
#30995=CARTESIAN_POINT('Ctrl Pts',(40.0397275404243,33.3508404137581,48.1420507077958));
#30996=CARTESIAN_POINT('Ctrl Pts',(40.036527263158,33.3470211317567,48.0709181788555));
#30997=CARTESIAN_POINT('Ctrl Pts',(40.0365300017577,33.3432018497554,47.9999088486209));
#30998=CARTESIAN_POINT('',(40.0365309427124,32.5494518497613,48.0021109581357));
#30999=CARTESIAN_POINT('Ctrl Pts',(40.0365300017577,33.3432018497283,47.999908848118));
#31000=CARTESIAN_POINT('Ctrl Pts',(40.0365301886757,33.3429411732082,47.995062265673));
#31001=CARTESIAN_POINT('Ctrl Pts',(40.0365452833311,33.3426804966881,47.9902157169632));
#31002=CARTESIAN_POINT('Ctrl Pts',(40.0365752852343,33.342419820168,47.9853692606322));
#31003=CARTESIAN_POINT('Ctrl Pts',(40.0370627597868,33.3381843165302,47.9066234518049));
#31004=CARTESIAN_POINT('Ctrl Pts',(40.0414910096202,33.3339488128924,47.8277523584294));
#31005=CARTESIAN_POINT('Ctrl Pts',(40.0498763342247,33.3297133092546,47.7491829422411));
#31006=CARTESIAN_POINT('Ctrl Pts',(40.0582495028227,33.3254839457262,47.6707274262747));
#31007=CARTESIAN_POINT('Ctrl Pts',(40.0705683051724,33.3212545821977,47.5925731817794));
#31008=CARTESIAN_POINT('Ctrl Pts',(40.0867970331473,33.3170252186692,47.5151469552082));
#31009=CARTESIAN_POINT('Ctrl Pts',(40.1030068094114,33.3128007941399,47.4378111460411));
#31010=CARTESIAN_POINT('Ctrl Pts',(40.1231173420964,33.3085763696107,47.3612021223331));
#31011=CARTESIAN_POINT('Ctrl Pts',(40.1470413339673,33.3043519450814,47.2857397602776));
#31012=CARTESIAN_POINT('Ctrl Pts',(40.1709500269587,33.300130221981,47.210325654784));
#31013=CARTESIAN_POINT('Ctrl Pts',(40.1986671975273,33.2959084988806,47.1360572017636));
#31014=CARTESIAN_POINT('Ctrl Pts',(40.2300551454641,33.2916867757802,47.0633411671409));
#31015=CARTESIAN_POINT('Ctrl Pts',(40.2614328234411,33.2874664340038,46.990648924795));
#31016=CARTESIAN_POINT('Ctrl Pts',(40.2964787080179,33.2832460922275,46.9195085228346));
#31017=CARTESIAN_POINT('Ctrl Pts',(40.335006740943,33.2790257504511,46.8503073102132));
#31018=CARTESIAN_POINT('Ctrl Pts',(40.3735341991558,33.2748054716284,46.7811071298479));
#31019=CARTESIAN_POINT('Ctrl Pts',(40.4155434729893,33.2705851928057,46.7138464907509));
#31020=CARTESIAN_POINT('Ctrl Pts',(40.4608029972008,33.2663649139831,46.6488873380674));
#31021=CARTESIAN_POINT('Ctrl Pts',(40.5061077911708,33.2621404139273,46.5838632115425));
#31022=CARTESIAN_POINT('Ctrl Pts',(40.5546690608197,33.2579159138715,46.5211455559961));
#31023=CARTESIAN_POINT('Ctrl Pts',(40.6062127509982,33.2536914138157,46.4610660357838));
#31024=CARTESIAN_POINT('Ctrl Pts',(40.6577811870465,33.2494648855984,46.4009576716919));
#31025=CARTESIAN_POINT('Ctrl Pts',(40.712334572453,33.2452383573811,46.343490306935));
#31026=CARTESIAN_POINT('Ctrl Pts',(40.7695612755813,33.2410118291638,46.2889593789697));
#31027=CARTESIAN_POINT('Ctrl Pts',(40.8268925863817,33.2367775750553,46.2343287710801));
#31028=CARTESIAN_POINT('Ctrl Pts',(40.8869066230888,33.2325433209469,46.1826456329205));
#31029=CARTESIAN_POINT('Ctrl Pts',(40.949258059808,33.2283090668384,46.1341655314932));
#31030=CARTESIAN_POINT('Ctrl Pts',(41.0087244148732,33.2242707371463,46.0879286670877));
#31031=CARTESIAN_POINT('Ctrl Pts',(41.0703163320914,33.2202324074542,46.0446051538659));
#31032=CARTESIAN_POINT('Ctrl Pts',(41.1337121478315,33.2161940777621,46.0043784135387));
#31033=CARTESIAN_POINT('Ctrl Pts',(41.2002030886068,33.2119585878129,45.9621877140823));
#31034=CARTESIAN_POINT('Ctrl Pts',(41.2689313141011,33.2077230978637,45.9232435152126));
#31035=CARTESIAN_POINT('Ctrl Pts',(41.3395465581916,33.2034876079144,45.887790507867));
#31036=CARTESIAN_POINT('Ctrl Pts',(41.4100594322341,33.1992582581027,45.8523888963088));
#31037=CARTESIAN_POINT('Ctrl Pts',(41.4824534765709,33.1950289082911,45.820468634562));
#31038=CARTESIAN_POINT('Ctrl Pts',(41.556350470286,33.1907995584794,45.7922305573468));
#31039=CARTESIAN_POINT('Ctrl Pts',(41.6301611680874,33.1865751476454,45.7640254561777));
#31040=CARTESIAN_POINT('Ctrl Pts',(41.7054708913532,33.1823507368114,45.7394941612978));
#31041=CARTESIAN_POINT('Ctrl Pts',(41.7818792878239,33.1781263259774,45.7187904028611));
#31042=CARTESIAN_POINT('Ctrl Pts',(41.8582388229468,33.1739046165535,45.6980998839842));
#31043=CARTESIAN_POINT('Ctrl Pts',(41.9356951850186,33.1696829071295,45.6812321659715));
#31044=CARTESIAN_POINT('Ctrl Pts',(42.0138317801886,33.1654611977055,45.668291496154));
#31045=CARTESIAN_POINT('Ctrl Pts',(42.0919428101117,33.1612408695683,45.6553550603503));
#31046=CARTESIAN_POINT('Ctrl Pts',(42.1707331685003,33.1570205414311,45.6463431980313));
#31047=CARTESIAN_POINT('Ctrl Pts',(42.2497764303575,33.1528002132939,45.6413089816545));
#31048=CARTESIAN_POINT('Ctrl Pts',(42.3288185141863,33.1485799480547,45.6362748403056));
#31049=CARTESIAN_POINT('Ctrl Pts',(42.4081130255018,33.1443596828155,45.6352182555618));
#31050=CARTESIAN_POINT('Ctrl Pts',(42.4872302856977,33.1401394175764,45.6381402839802));
#31051=CARTESIAN_POINT('Ctrl Pts',(42.5664266847193,33.1359149309216,45.6410652352235));
#31052=CARTESIAN_POINT('Ctrl Pts',(42.6454450082886,33.1316904442669,45.6479767322123));
#31053=CARTESIAN_POINT('Ctrl Pts',(42.7238580581001,33.1274659576121,45.6588237146461));
#31054=CARTESIAN_POINT('Ctrl Pts',(42.8023087551845,33.1232394427184,45.6696759048777));
#31055=CARTESIAN_POINT('Ctrl Pts',(42.8801531378612,33.1190129278247,45.6844672569032));
#31056=CARTESIAN_POINT('Ctrl Pts',(42.9569741471685,33.114786412931,45.7030955091067));
#31057=CARTESIAN_POINT('Ctrl Pts',(43.0339355873157,33.1105521718561,45.7217578142486));
#31058=CARTESIAN_POINT('Ctrl Pts',(43.1098694647127,33.1063179307812,45.7442709013296));
#31059=CARTESIAN_POINT('Ctrl Pts',(43.1843740243166,33.1020836897063,45.7704826013513));
#31060=CARTESIAN_POINT('Ctrl Pts',(43.2554335226878,33.0980452382563,45.7954822827788));
#31061=CARTESIAN_POINT('Ctrl Pts',(43.3251926467937,33.0940067868063,45.8238459238552));
#31062=CARTESIAN_POINT('Ctrl Pts',(43.3933230863742,33.0899683353563,45.8554022085771));
#31063=CARTESIAN_POINT('Ctrl Pts',(43.4647779751452,33.085732826222,45.8884982935094));
#31064=CARTESIAN_POINT('Ctrl Pts',(43.5347127990157,33.0814973170877,45.9252323543139));
#31065=CARTESIAN_POINT('Ctrl Pts',(43.6027322727976,33.0772618079534,45.9654421805043));
#31066=CARTESIAN_POINT('Ctrl Pts',(43.6706531389894,33.0730324390217,46.0055937146522));
#31067=CARTESIAN_POINT('Ctrl Pts',(43.7366637684668,33.0688030700899,46.0492107711841));
#31068=CARTESIAN_POINT('Ctrl Pts',(43.8003906372222,33.0645737011582,46.0960839030881));
#31069=CARTESIAN_POINT('Ctrl Pts',(43.8640430841429,33.0603492713895,46.1429022953736));
#31070=CARTESIAN_POINT('Ctrl Pts',(43.9254166941085,33.0561248416209,46.1929689300503));
#31071=CARTESIAN_POINT('Ctrl Pts',(43.9841655866422,33.0519004118522,46.2460302639445));
#31072=CARTESIAN_POINT('Ctrl Pts',(44.0428769091537,33.047678683614,46.2990576650205));
#31073=CARTESIAN_POINT('Ctrl Pts',(44.0989664983492,33.0434569553757,46.3550756504771));
#31074=CARTESIAN_POINT('Ctrl Pts',(44.1521213036876,33.0392352271375,46.4137902477717));
#31075=CARTESIAN_POINT('Ctrl Pts',(44.2052587157395,33.0350148803308,46.4724856325077));
#31076=CARTESIAN_POINT('Ctrl Pts',(44.2554629360496,33.0307945335242,46.5338755292781));
#31077=CARTESIAN_POINT('Ctrl Pts',(44.3024586350226,33.0265741867175,46.5976300121124));
#31078=CARTESIAN_POINT('Ctrl Pts',(44.3494536317073,33.0223539029784,46.6613835422206));
#31079=CARTESIAN_POINT('Ctrl Pts',(44.3932399249475,33.0181336192392,46.7275012095623));
#31080=CARTESIAN_POINT('Ctrl Pts',(44.4335841717754,33.0139133355,46.7956222115945));
#31081=CARTESIAN_POINT('Ctrl Pts',(44.4739687699017,33.0096888307395,46.8638113465352));
#31082=CARTESIAN_POINT('Ctrl Pts',(44.5109042047491,33.0054643259789,46.9340074139761));
#31083=CARTESIAN_POINT('Ctrl Pts',(44.5442023068821,33.0012398212184,47.0058235025604));
#31084=CARTESIAN_POINT('Ctrl Pts',(44.577516394402,32.9970132884041,47.0776740678228));
#31085=CARTESIAN_POINT('Ctrl Pts',(44.6071894946154,32.9927867555897,47.1511457677516));
#31086=CARTESIAN_POINT('Ctrl Pts',(44.6330819850572,32.9885602227754,47.2258325188222));
#31087=CARTESIAN_POINT('Ctrl Pts',(44.6590218042317,32.9843259643063,47.3006557893711));
#31088=CARTESIAN_POINT('Ctrl Pts',(44.6811670731451,32.9800917058371,47.3766980972965));
#31089=CARTESIAN_POINT('Ctrl Pts',(44.6994284220833,32.975857447368,47.453539230488));
#31090=CARTESIAN_POINT('Ctrl Pts',(44.7168445832576,32.9718191625621,47.5268239349756));
#31091=CARTESIAN_POINT('Ctrl Pts',(44.7307283585708,32.9677808777563,47.6008347990511));
#31092=CARTESIAN_POINT('Ctrl Pts',(44.7410462183001,32.9637425929504,47.6752030716234));
#31093=CARTESIAN_POINT('Ctrl Pts',(44.7518680209965,32.9595070709964,47.753203625398));
#31094=CARTESIAN_POINT('Ctrl Pts',(44.7588078116323,32.9552715490425,47.8318938707056));
#31095=CARTESIAN_POINT('Ctrl Pts',(44.7617881702188,32.9510360270885,47.9108536040287));
#31096=CARTESIAN_POINT('Ctrl Pts',(44.76476420838,32.9468066450858,47.9896988747386));
#31097=CARTESIAN_POINT('Ctrl Pts',(44.7637921950172,32.9425772630831,48.0688123926393));
#31098=CARTESIAN_POINT('Ctrl Pts',(44.7588462100641,32.9383478810803,48.1477667018179));
#31099=CARTESIAN_POINT('Ctrl Pts',(44.7539060007715,32.9341234379269,48.2266288123171));
#31100=CARTESIAN_POINT('Ctrl Pts',(44.7450010708078,32.9298989947735,48.3053316175483));
#31101=CARTESIAN_POINT('Ctrl Pts',(44.7321575411424,32.92567455162,48.3834470552665));
#31102=CARTESIAN_POINT('Ctrl Pts',(44.7193222243507,32.9214528098126,48.4615125415903));
#31103=CARTESIAN_POINT('Ctrl Pts',(44.7025533826062,32.9172310680052,48.5389909440019));
#31104=CARTESIAN_POINT('Ctrl Pts',(44.6819288998,32.9130093261978,48.615459939523));
#31105=CARTESIAN_POINT('Ctrl Pts',(44.6613111649013,32.9087889656577,48.6919039159582));
#31106=CARTESIAN_POINT('Ctrl Pts',(44.6368404159638,32.9045686051175,48.7673386884742));
#31107=CARTESIAN_POINT('Ctrl Pts',(44.6086451813714,32.9003482445774,48.8413542082292));
#31108=CARTESIAN_POINT('Ctrl Pts',(44.580450367153,32.8961279469603,48.9153686244573));
#31109=CARTESIAN_POINT('Ctrl Pts',(44.5485313459866,32.8919076493432,48.9879633918609));
#31110=CARTESIAN_POINT('Ctrl Pts',(44.513065328651,32.8876873517261,49.0587470697731));
#31111=CARTESIAN_POINT('Ctrl Pts',(44.477563838149,32.8834628329607,49.1296015456313));
#31112=CARTESIAN_POINT('Ctrl Pts',(44.4385084752291,32.8792383141953,49.198640892767));
#31113=CARTESIAN_POINT('Ctrl Pts',(44.3961228473338,32.8750137954299,49.2654975382244));
#31114=CARTESIAN_POINT('Ctrl Pts',(44.3537168705543,32.8707872485184,49.3323862808385));
#31115=CARTESIAN_POINT('Ctrl Pts',(44.3079777150414,32.8665607016069,49.3970898504622));
#31116=CARTESIAN_POINT('Ctrl Pts',(44.2591713759898,32.8623341546955,49.4592711316271));
#31117=CARTESIAN_POINT('Ctrl Pts',(44.2102758245718,32.8580998821431,49.5215660730121));
#31118=CARTESIAN_POINT('Ctrl Pts',(44.1583021953996,32.8538656095907,49.5813291580854));
#31119=CARTESIAN_POINT('Ctrl Pts',(44.103555552443,32.8496313370383,49.6382578919818));
#31120=CARTESIAN_POINT('Ctrl Pts',(44.0513445009608,32.8455931748737,49.6925499708338));
#31121=CARTESIAN_POINT('Ctrl Pts',(43.9966118976582,32.8415550127092,49.7442642130799));
#31122=CARTESIAN_POINT('Ctrl Pts',(43.9396497050753,32.8375168505446,49.7931729494283));
#31123=CARTESIAN_POINT('Ctrl Pts',(43.8799050192773,32.8332814319488,49.8444707831917));
#31124=CARTESIAN_POINT('Ctrl Pts',(43.8174802415135,32.829046013353,49.8928770260256));
#31125=CARTESIAN_POINT('Ctrl Pts',(43.7526868699549,32.8248105947572,49.9380992422349));
#31126=CARTESIAN_POINT('Ctrl Pts',(43.6879874316164,32.8205813163961,49.9832558982135));
#31127=CARTESIAN_POINT('Ctrl Pts',(43.6209266001007,32.8163520380349,50.0252374277449));
#31128=CARTESIAN_POINT('Ctrl Pts',(43.5518498352913,32.8121227596738,50.0637907834467));
#31129=CARTESIAN_POINT('Ctrl Pts',(43.4828537357243,32.8078984201046,50.1022991179927));
#31130=CARTESIAN_POINT('Ctrl Pts',(43.4118467886812,32.8036740805353,50.1373870064232));
#31131=CARTESIAN_POINT('Ctrl Pts',(43.339203118874,32.799449740966,50.168844840554));
#31132=CARTESIAN_POINT('Ctrl Pts',(43.2666059012847,32.7952281026637,50.2002825588759));
#31133=CARTESIAN_POINT('Ctrl Pts',(43.1923744677768,32.7910064643614,50.2280946440591));
#31134=CARTESIAN_POINT('Ctrl Pts',(43.1169061203529,32.786784826059,50.2521181264535));
#31135=CARTESIAN_POINT('Ctrl Pts',(43.0414624613174,32.7825645688052,50.27613374991));
#31136=CARTESIAN_POINT('Ctrl Pts',(42.9647831387621,32.7783443115513,50.2963630893206));
#31137=CARTESIAN_POINT('Ctrl Pts',(42.8872825306362,32.7741240542975,50.3126924084791));
#31138=CARTESIAN_POINT('Ctrl Pts',(42.8097830714399,32.769903859608,50.329021485559));
#31139=CARTESIAN_POINT('Ctrl Pts',(42.7314628104373,32.7656836649185,50.3414505618484));
#31140=CARTESIAN_POINT('Ctrl Pts',(42.6527468126245,32.761463470229,50.3499169112137));
#31141=CARTESIAN_POINT('Ctrl Pts',(42.5739520570758,32.7572390531072,50.3583917314175));
#31142=CARTESIAN_POINT('Ctrl Pts',(42.4947612415589,32.7530146359853,50.3628958541422));
#31143=CARTESIAN_POINT('Ctrl Pts',(42.4156044580236,32.7487902188635,50.3634184863857));
#31144=CARTESIAN_POINT('Ctrl Pts',(42.3364096612673,32.7445637730626,50.3639413696114));
#31145=CARTESIAN_POINT('Ctrl Pts',(42.257249398617,32.7403373272618,50.3604789739278));
#31146=CARTESIAN_POINT('Ctrl Pts',(42.1785510773987,32.736110881461,50.3530726328736));
#31147=CARTESIAN_POINT('Ctrl Pts',(42.0997088620007,32.7318767079102,50.3456527498613));
#31148=CARTESIAN_POINT('Ctrl Pts',(42.0213307415196,32.7276425343593,50.3342745793876));
#31149=CARTESIAN_POINT('Ctrl Pts',(41.9438361418862,32.7234083608085,50.3190310423646));
#31150=CARTESIAN_POINT('Ctrl Pts',(41.8699121019261,32.7193692765852,50.3044898505222));
#31151=CARTESIAN_POINT('Ctrl Pts',(41.7967922975485,32.715330192362,50.2864317634616));
#31152=CARTESIAN_POINT('Ctrl Pts',(41.7248263995385,32.7112911081387,50.2649792604216));
#31153=CARTESIAN_POINT('Ctrl Pts',(41.6493592792177,32.7070555179009,50.2424830688521));
#31154=CARTESIAN_POINT('Ctrl Pts',(41.5748742971278,32.7028199276631,50.2161682479835));
#31155=CARTESIAN_POINT('Ctrl Pts',(41.5017859410379,32.6985843374253,50.1861385924005));
#31156=CARTESIAN_POINT('Ctrl Pts',(41.4288035460196,32.6943548878056,50.156152472815));
#31157=CARTESIAN_POINT('Ctrl Pts',(41.3572141865826,32.6901254381859,50.1224623903211));
#31158=CARTESIAN_POINT('Ctrl Pts',(41.287417594974,32.6858959885662,50.0852220104648));
#31159=CARTESIAN_POINT('Ctrl Pts',(41.21770252839,32.6816714791015,50.0480251287623));
#31160=CARTESIAN_POINT('Ctrl Pts',(41.1497764803467,32.6774469696368,50.0072864101184));
#31161=CARTESIAN_POINT('Ctrl Pts',(41.0840181554684,32.6732224601722,49.9632071275755));
#31162=CARTESIAN_POINT('Ctrl Pts',(41.0183018922523,32.6690006528732,49.9191560399098));
#31163=CARTESIAN_POINT('Ctrl Pts',(40.954750988961,32.6647788455742,49.8717688899777));
#31164=CARTESIAN_POINT('Ctrl Pts',(40.8937174639057,32.6605570382752,49.821291674158));
#31165=CARTESIAN_POINT('Ctrl Pts',(40.8327039204864,32.6563366131448,49.7708309839667));
#31166=CARTESIAN_POINT('Ctrl Pts',(40.7742064801868,32.6521161880143,49.7172825355787));
#31167=CARTESIAN_POINT('Ctrl Pts',(40.7185449923322,32.6478957628839,49.6609333213855));
#31168=CARTESIAN_POINT('Ctrl Pts',(40.6628843473165,32.6436754016601,49.604584960445));
#31169=CARTESIAN_POINT('Ctrl Pts',(40.61005989826,32.6394550404363,49.5454362528354));
#31170=CARTESIAN_POINT('Ctrl Pts',(40.5603543753744,32.6352346792125,49.4838107752324));
#31171=CARTESIAN_POINT('Ctrl Pts',(40.5105991610115,32.63101009882,49.4221236895657));
#31172=CARTESIAN_POINT('Ctrl Pts',(40.4639693968664,32.6267855184275,49.3579552538229));
#31173=CARTESIAN_POINT('Ctrl Pts',(40.4207068556936,32.622560938035,49.2916613680844));
#31174=CARTESIAN_POINT('Ctrl Pts',(40.3774235549587,32.6183343304746,49.2253356711762));
#31175=CARTESIAN_POINT('Ctrl Pts',(40.3375109327348,32.6141077229141,49.1568828985045));
#31176=CARTESIAN_POINT('Ctrl Pts',(40.3011654703015,32.6098811153537,49.0866848935387));
#31177=CARTESIAN_POINT('Ctrl Pts',(40.2647535939065,32.605646784525,49.0163586159551));
#31178=CARTESIAN_POINT('Ctrl Pts',(40.2319220973869,32.6014124536964,48.9442811618195));
#31179=CARTESIAN_POINT('Ctrl Pts',(40.202819758277,32.5971781228678,48.8708555714251));
#31180=CARTESIAN_POINT('Ctrl Pts',(40.1750696382883,32.5931405371561,48.8008416479397));
#31181=CARTESIAN_POINT('Ctrl Pts',(40.1507099100065,32.5891029514445,48.7296024347614));
#31182=CARTESIAN_POINT('Ctrl Pts',(40.1298266558031,32.5850653657328,48.6574978541392));
#31183=CARTESIAN_POINT('Ctrl Pts',(40.1025025412974,32.579782498741,48.5631546163417));
#31184=CARTESIAN_POINT('Ctrl Pts',(40.0810445127194,32.5744996317493,48.4670411181778));
#31185=CARTESIAN_POINT('Ctrl Pts',(40.0656409106017,32.5692167647575,48.3698081700603));
#31186=CARTESIAN_POINT('Ctrl Pts',(40.0504879803225,32.5640198689543,48.2741575506527));
#31187=CARTESIAN_POINT('Ctrl Pts',(40.0411940473043,32.558822973151,48.1774235249491));
#31188=CARTESIAN_POINT('Ctrl Pts',(40.0378927055361,32.5536260773478,48.0802469335257));
#31189=CARTESIAN_POINT('Ctrl Pts',(40.0370088091741,32.5522346681523,48.0542290166743));
#31190=CARTESIAN_POINT('Ctrl Pts',(40.0365542261138,32.5508432589568,48.0281794990929));
#31191=CARTESIAN_POINT('Ctrl Pts',(40.0365309427124,32.5494518497613,48.0021109581356));
#31192=CARTESIAN_POINT('',(40.036530204639,31.7557018496867,47.9990164777473));
#31193=CARTESIAN_POINT('Ctrl Pts',(40.0365309427119,32.5494518497283,48.0021109575178));
#31194=CARTESIAN_POINT('Ctrl Pts',(40.0364608572083,32.5452635594843,47.923641865808));
#31195=CARTESIAN_POINT('Ctrl Pts',(40.0403028998604,32.5410752692403,47.845091734552));
#31196=CARTESIAN_POINT('Ctrl Pts',(40.0480545536977,32.5368869789963,47.7668840234603));
#31197=CARTESIAN_POINT('Ctrl Pts',(40.0558026175344,32.5327006284628,47.6887125324764));
#31198=CARTESIAN_POINT('Ctrl Pts',(40.0674566527063,32.5285142779294,47.6108836216765));
#31199=CARTESIAN_POINT('Ctrl Pts',(40.0829621346619,32.5243279273959,47.5338176628296));
#31200=CARTESIAN_POINT('Ctrl Pts',(40.0984654725121,32.520142155753,47.4567623607004));
#31201=CARTESIAN_POINT('Ctrl Pts',(40.1178191046942,32.5159563841101,47.3804702691739));
#31202=CARTESIAN_POINT('Ctrl Pts',(40.1409173179971,32.5117706124672,47.3053519763402));
#31203=CARTESIAN_POINT('Ctrl Pts',(40.1640198407705,32.5075840598782,47.2302196685665));
#31204=CARTESIAN_POINT('Ctrl Pts',(40.1908681884987,32.5033975072892,47.1562620499446));
#31205=CARTESIAN_POINT('Ctrl Pts',(40.2213071605378,32.4992109547002,47.0838733972993));
#31206=CARTESIAN_POINT('Ctrl Pts',(40.2517803805662,32.4950196916694,47.0114032975602));
#31207=CARTESIAN_POINT('Ctrl Pts',(40.285852097053,32.4908284286385,46.9405061254933));
#31208=CARTESIAN_POINT('Ctrl Pts',(40.3233197885971,32.4866371656076,46.8715542811161));
#31209=CARTESIAN_POINT('Ctrl Pts',(40.3608130679852,32.4824430402337,46.8025553473943));
#31210=CARTESIAN_POINT('Ctrl Pts',(40.4017066855213,32.4782489148598,46.7355047899506));
#31211=CARTESIAN_POINT('Ctrl Pts',(40.4457545542511,32.474054789486,46.6707463828638));
#31212=CARTESIAN_POINT('Ctrl Pts',(40.4898735926267,32.4698538875205,46.6058833434071));
#31213=CARTESIAN_POINT('Ctrl Pts',(40.5371567570249,32.465652985555,46.5433202181791));
#31214=CARTESIAN_POINT('Ctrl Pts',(40.5873180183348,32.4614520835895,46.483367389825));
#31215=CARTESIAN_POINT('Ctrl Pts',(40.5977161267224,32.460581263502,46.4709395522649));
#31216=CARTESIAN_POINT('Ctrl Pts',(40.608237786181,32.4597104434145,46.4586237507235));
#31217=CARTESIAN_POINT('Ctrl Pts',(40.6188802620662,32.458839623327,46.4464225413444));
#31218=CARTESIAN_POINT('Ctrl Pts',(40.6706354675536,32.4546047560784,46.3870870910772));
#31219=CARTESIAN_POINT('Ctrl Pts',(40.7254574787414,32.4503698888297,46.3302277192351));
#31220=CARTESIAN_POINT('Ctrl Pts',(40.7830801107519,32.4461350215811,46.2761785148532));
#31221=CARTESIAN_POINT('Ctrl Pts',(40.8406191793464,32.4419062956689,46.2222076917599));
#31222=CARTESIAN_POINT('Ctrl Pts',(40.9009504640461,32.4376775697568,46.1710392619322));
#31223=CARTESIAN_POINT('Ctrl Pts',(40.9637685103185,32.4334488438446,46.1229732157087));
#31224=CARTESIAN_POINT('Ctrl Pts',(41.0265132040005,32.4292250558129,46.0749632961749));
#31225=CARTESIAN_POINT('Ctrl Pts',(41.0917385180085,32.4250012677811,46.0300488452585));
#31226=CARTESIAN_POINT('Ctrl Pts',(41.1591043888966,32.4207774797494,45.9884909835538));
#31227=CARTESIAN_POINT('Ctrl Pts',(41.226427189383,32.4165563921985,45.9469596918878));
#31228=CARTESIAN_POINT('Ctrl Pts',(41.295887431959,32.4123353046477,45.9087809758935));
#31229=CARTESIAN_POINT('Ctrl Pts',(41.3671154168577,32.4081142170968,45.8741731305661));
#31230=CARTESIAN_POINT('Ctrl Pts',(41.4383201232241,32.4038945090701,45.8395765956787));
#31231=CARTESIAN_POINT('Ctrl Pts',(41.5112910027688,32.3996748010433,45.8085488191928));
#31232=CARTESIAN_POINT('Ctrl Pts',(41.5856343863434,32.3954550930166,45.7812618252273));
#31233=CARTESIAN_POINT('Ctrl Pts',(41.6599767075322,32.3912354452905,45.7539752211999));
#31234=CARTESIAN_POINT('Ctrl Pts',(41.7356910525477,32.3870157975645,45.7304294539531));
#31235=CARTESIAN_POINT('Ctrl Pts',(41.812365852117,32.3827961498385,45.7107476003853));
#31236=CARTESIAN_POINT('Ctrl Pts',(41.8891175111503,32.378572272302,45.6910460175619));
#31237=CARTESIAN_POINT('Ctrl Pts',(41.9668310921309,32.3743483947656,45.6752162026539));
#31238=CARTESIAN_POINT('Ctrl Pts',(42.04508259513,32.3701245172292,45.6633305589749));
#31239=CARTESIAN_POINT('Ctrl Pts',(42.1233717394494,32.365898607881,45.6514391979448));
#31240=CARTESIAN_POINT('Ctrl Pts',(42.202198853473,32.3616726985328,45.6434958347941));
#31241=CARTESIAN_POINT('Ctrl Pts',(42.2811351138128,32.3574467891846,45.6395209003824));
#31242=CARTESIAN_POINT('Ctrl Pts',(42.3602159403493,32.3532131403813,45.6355386861584));
#31243=CARTESIAN_POINT('Ctrl Pts',(42.4394058418959,32.348979491578,45.6355394235851));
#31244=CARTESIAN_POINT('Ctrl Pts',(42.5182764905371,32.3447458427747,45.6394913445009));
#31245=CARTESIAN_POINT('Ctrl Pts',(42.5936138449197,32.3407018554902,45.6432662249115));
#31246=CARTESIAN_POINT('Ctrl Pts',(42.6686595840971,32.3366578682057,45.6506457692674));
#31247=CARTESIAN_POINT('Ctrl Pts',(42.743048710163,32.3326138809212,45.6615586337572));
#31248=CARTESIAN_POINT('Ctrl Pts',(42.8209763868576,32.3283775287777,45.6729906026584));
#31249=CARTESIAN_POINT('Ctrl Pts',(42.8984798686474,32.3241411766341,45.6883438939023));
#31250=CARTESIAN_POINT('Ctrl Pts',(42.9751339462279,32.3199048244906,45.7075752171998));
#31251=CARTESIAN_POINT('Ctrl Pts',(43.0516768649382,32.3156746156356,45.7267786524549));
#31252=CARTESIAN_POINT('Ctrl Pts',(43.1273723743003,32.3114444067807,45.749848838815));
#31253=CARTESIAN_POINT('Ctrl Pts',(43.2018027161336,32.3072141979257,45.7766910144335));
#31254=CARTESIAN_POINT('Ctrl Pts',(43.27614600427,32.3029889367213,45.8035017954545));
#31255=CARTESIAN_POINT('Ctrl Pts',(43.3492266264,32.2987636755168,45.8340756403681));
#31256=CARTESIAN_POINT('Ctrl Pts',(43.4206408061468,32.2945384143124,45.8682676561707));
#31257=CARTESIAN_POINT('Ctrl Pts',(43.4920092323684,32.2903158601417,45.902437765886));
#31258=CARTESIAN_POINT('Ctrl Pts',(43.5617129132941,32.286093305971,45.9402212434752));
#31259=CARTESIAN_POINT('Ctrl Pts',(43.6293680649197,32.2818707518003,45.9814251062059));
#31260=CARTESIAN_POINT('Ctrl Pts',(43.697000977395,32.2776495856395,46.0226154246778));
#31261=CARTESIAN_POINT('Ctrl Pts',(43.7625862973116,32.2734284194786,46.0672236518772));
#31262=CARTESIAN_POINT('Ctrl Pts',(43.8257661917328,32.2692072533178,46.115011616107));
#31263=CARTESIAN_POINT('Ctrl Pts',(43.8889450275653,32.2649861578832,46.1627987796421));
#31264=CARTESIAN_POINT('Ctrl Pts',(43.9497181446446,32.2607650624487,46.2137652902326));
#31265=CARTESIAN_POINT('Ctrl Pts',(44.007759191331,32.2565439670141,46.2676314411793));
#31266=CARTESIAN_POINT('Ctrl Pts',(44.0658580353617,32.2523186682076,46.3215512321039));
#31267=CARTESIAN_POINT('Ctrl Pts',(44.1212190295284,32.2480933694012,46.3783761115966));
#31268=CARTESIAN_POINT('Ctrl Pts',(44.1735517137177,32.2438680705947,46.4377885035409));
#31269=CARTESIAN_POINT('Ctrl Pts',(44.2259094134132,32.2396407520564,46.497229295157));
#31270=CARTESIAN_POINT('Ctrl Pts',(44.27523562692,32.2354134335181,46.5592596955544));
#31271=CARTESIAN_POINT('Ctrl Pts',(44.3212809875985,32.2311861149798,46.6235299467142));
#31272=CARTESIAN_POINT('Ctrl Pts',(44.3674102436011,32.2269510942049,46.6879172992166));
#31273=CARTESIAN_POINT('Ctrl Pts',(44.4102464473705,32.2227160734301,46.7545522617234));
#31274=CARTESIAN_POINT('Ctrl Pts',(44.4495843956108,32.2184810526553,46.8230572460104));
#31275=CARTESIAN_POINT('Ctrl Pts',(44.4870269849002,32.2144500812753,46.8882615615802));
#31276=CARTESIAN_POINT('Ctrl Pts',(44.5213005112486,32.2104191098953,46.9551595267172));
#31277=CARTESIAN_POINT('Ctrl Pts',(44.5522687182219,32.2063881385153,47.0234090900159));
#31278=CARTESIAN_POINT('Ctrl Pts',(44.584813386975,32.2021519672565,47.0951329528803));
#31279=CARTESIAN_POINT('Ctrl Pts',(44.6138305078913,32.1979157959978,47.1686212744498));
#31280=CARTESIAN_POINT('Ctrl Pts',(44.6391265225361,32.193679624739,47.2434929894737));
#31281=CARTESIAN_POINT('Ctrl Pts',(44.6643859409941,32.1894495820233,47.3182563862778));
#31282=CARTESIAN_POINT('Ctrl Pts',(44.6859347948584,32.1852195393076,47.3943987613566));
#31283=CARTESIAN_POINT('Ctrl Pts',(44.7036268507566,32.180989496592,47.4715174805413));
#31284=CARTESIAN_POINT('Ctrl Pts',(44.721298308255,32.1767643788048,47.5485464124106));
#31285=CARTESIAN_POINT('Ctrl Pts',(44.7351217866846,32.1725392610176,47.6265489745438));
#31286=CARTESIAN_POINT('Ctrl Pts',(44.7450007815637,32.1683141432305,47.7051071798673));
#31287=CARTESIAN_POINT('Ctrl Pts',(44.7548734793124,32.1640917186442,47.7836153101311));
#31288=CARTESIAN_POINT('Ctrl Pts',(44.7608066255724,32.1598692940578,47.8626779163478));
#31289=CARTESIAN_POINT('Ctrl Pts',(44.7627549789776,32.1556468694715,47.941867821161));
#31290=CARTESIAN_POINT('Ctrl Pts',(44.7647026983203,32.15142581901,48.0210319548058));
#31291=CARTESIAN_POINT('Ctrl Pts',(44.7626681883074,32.1472047685486,48.1003228361092));
#31292=CARTESIAN_POINT('Ctrl Pts',(44.756658253001,32.1429837180871,48.1793106786063));
#31293=CARTESIAN_POINT('Ctrl Pts',(44.7506483985321,32.1387627244014,48.258297458667));
#31294=CARTESIAN_POINT('Ctrl Pts',(44.7406632619964,32.1345417307157,48.3369807403088));
#31295=CARTESIAN_POINT('Ctrl Pts',(44.7267616098647,32.13032073703,48.4149347560278));
#31296=CARTESIAN_POINT('Ctrl Pts',(44.7128460402428,32.1260955175417,48.4929668145752));
#31297=CARTESIAN_POINT('Ctrl Pts',(44.6950062049653,32.1218702980534,48.5702676857593));
#31298=CARTESIAN_POINT('Ctrl Pts',(44.6733521350314,32.117645078565,48.6464213107936));
#31299=CARTESIAN_POINT('Ctrl Pts',(44.6516876520385,32.1134178272434,48.7226115567583));
#31300=CARTESIAN_POINT('Ctrl Pts',(44.626205431482,32.1091905759218,48.7976530126676));
#31301=CARTESIAN_POINT('Ctrl Pts',(44.5970647971759,32.1049633246002,48.8711467832177));
#31302=CARTESIAN_POINT('Ctrl Pts',(44.5678709214925,32.1007283498818,48.9447748305144));
#31303=CARTESIAN_POINT('Ctrl Pts',(44.5350054708115,32.0964933751634,49.0168491140407));
#31304=CARTESIAN_POINT('Ctrl Pts',(44.4986750622441,32.0922584004449,49.0869928353098));
#31305=CARTESIAN_POINT('Ctrl Pts',(44.4640858923939,32.0882263989998,49.1537747181615));
#31306=CARTESIAN_POINT('Ctrl Pts',(44.4263564860087,32.0841943975546,49.2188065591027));
#31307=CARTESIAN_POINT('Ctrl Pts',(44.3857010299083,32.0801623961095,49.2817885397839));
#31308=CARTESIAN_POINT('Ctrl Pts',(44.3430420096339,32.0759316913556,49.347874370531));
#31309=CARTESIAN_POINT('Ctrl Pts',(44.2969980803195,32.0717009866017,49.4119556142401));
#31310=CARTESIAN_POINT('Ctrl Pts',(44.2477839303533,32.0674702818478,49.4736637973528));
#31311=CARTESIAN_POINT('Ctrl Pts',(44.1986413466439,32.0632457293022,49.5352822456293));
#31312=CARTESIAN_POINT('Ctrl Pts',(44.1463379872993,32.0590211767567,49.594534120947));
#31313=CARTESIAN_POINT('Ctrl Pts',(44.0911323333135,32.0547966242111,49.6510790023865));
#31314=CARTESIAN_POINT('Ctrl Pts',(44.035991168931,32.0505770066622,49.7075578297769));
#31315=CARTESIAN_POINT('Ctrl Pts',(43.9779547736778,32.0463573891133,49.7613356118631));
#31316=CARTESIAN_POINT('Ctrl Pts',(43.9173214936809,32.0421377715644,49.8121053848256));
#31317=CARTESIAN_POINT('Ctrl Pts',(43.8567269689845,32.0379208510912,49.8628427069985));
#31318=CARTESIAN_POINT('Ctrl Pts',(43.793539213529,32.033703930618,49.9105755345289));
#31319=CARTESIAN_POINT('Ctrl Pts',(43.728092079237,32.0294870101448,49.9550350047935));
#31320=CARTESIAN_POINT('Ctrl Pts',(43.6626662169804,32.0252714602814,49.9994800245641));
#31321=CARTESIAN_POINT('Ctrl Pts',(43.5949828228806,32.021055910418,50.0406535353018));
#31322=CARTESIAN_POINT('Ctrl Pts',(43.5254061330093,32.0168403605545,50.0783290106922));
#31323=CARTESIAN_POINT('Ctrl Pts',(43.4558302002533,32.0126248565636,50.1160040761081));
#31324=CARTESIAN_POINT('Ctrl Pts',(43.3843614270841,32.0084093525727,50.1501809589749));
#31325=CARTESIAN_POINT('Ctrl Pts',(43.3113888010036,32.0041938485818,50.1806789984556));
#31326=CARTESIAN_POINT('Ctrl Pts',(43.2383420628195,31.9999740632612,50.2112080122068));
#31327=CARTESIAN_POINT('Ctrl Pts',(43.1637888559236,31.9957542779406,50.2380505371248));
#31328=CARTESIAN_POINT('Ctrl Pts',(43.0881377505087,31.99153449262,50.261074275035));
#31329=CARTESIAN_POINT('Ctrl Pts',(43.0124498389637,31.9873126542697,50.2841092145618));
#31330=CARTESIAN_POINT('Ctrl Pts',(42.9356634220074,31.9830908159194,50.3033215519959));
#31331=CARTESIAN_POINT('Ctrl Pts',(42.8581992873437,31.9788689775691,50.3186297362834));
#31332=CARTESIAN_POINT('Ctrl Pts',(42.7805915934368,31.9746393151604,50.3339662902334));
#31333=CARTESIAN_POINT('Ctrl Pts',(42.7023041389721,31.9704096527516,50.3453841654492));
#31334=CARTESIAN_POINT('Ctrl Pts',(42.6237647000761,31.9661799903429,50.3528535440821));
#31335=CARTESIAN_POINT('Ctrl Pts',(42.5479836489396,31.9620988781298,50.3600605902758));
#31336=CARTESIAN_POINT('Ctrl Pts',(42.4719684048579,31.9580177659167,50.3635919372317));
#31337=CARTESIAN_POINT('Ctrl Pts',(42.396101149199,31.9539366537036,50.3634667841674));
#31338=CARTESIAN_POINT('Ctrl Pts',(42.31722052377,31.949693443889,50.3633366601514));
#31339=CARTESIAN_POINT('Ctrl Pts',(42.23819890299,31.9454502340745,50.3592530261779));
#31340=CARTESIAN_POINT('Ctrl Pts',(42.1594644392978,31.9412070242599,50.3511982232338));
#31341=CARTESIAN_POINT('Ctrl Pts',(42.0808442658474,31.9369699738507,50.3431551125694));
#31342=CARTESIAN_POINT('Ctrl Pts',(42.0025108828749,31.9327329234415,50.3311523285694));
#31343=CARTESIAN_POINT('Ctrl Pts',(41.9248923818167,31.9284958730323,50.3152242206845));
#31344=CARTESIAN_POINT('Ctrl Pts',(41.8473655468738,31.9242638265068,50.2993149236212));
#31345=CARTESIAN_POINT('Ctrl Pts',(41.7705523715381,31.9200317799812,50.2794896094482));
#31346=CARTESIAN_POINT('Ctrl Pts',(41.6948742435766,31.9157997334557,50.2558342378216));
#31347=CARTESIAN_POINT('Ctrl Pts',(41.619245190707,31.9115704312908,50.232194206024));
#31348=CARTESIAN_POINT('Ctrl Pts',(41.5447501691425,31.9073411291258,50.2047291860695));
#31349=CARTESIAN_POINT('Ctrl Pts',(41.471797652959,31.9031118269609,50.1735755896328));
#31350=CARTESIAN_POINT('Ctrl Pts',(41.3988698801052,31.8988839592498,50.142432559572));
#31351=CARTESIAN_POINT('Ctrl Pts',(41.3274840032654,31.8946560915387,50.107603620975));
#31352=CARTESIAN_POINT('Ctrl Pts',(41.258029291252,31.8904282238276,50.0692736264838));
#31353=CARTESIAN_POINT('Ctrl Pts',(41.1885766545262,31.886200482444,50.0309447772823));
#31354=CARTESIAN_POINT('Ctrl Pts',(41.121055476621,31.8819727410605,49.9891153071296));
#31355=CARTESIAN_POINT('Ctrl Pts',(41.0558298434275,31.8777449996769,49.9440156972308));
#31356=CARTESIAN_POINT('Ctrl Pts',(40.9905414240873,31.8735131886726,49.8988726744806));
#31357=CARTESIAN_POINT('Ctrl Pts',(40.9275533492749,31.8692813776682,49.8504534899445));
#31358=CARTESIAN_POINT('Ctrl Pts',(40.867199632914,31.8650495666639,49.7990312603068));
#31359=CARTESIAN_POINT('Ctrl Pts',(40.8068180043334,31.8608157985433,49.7475852490586));
#31360=CARTESIAN_POINT('Ctrl Pts',(40.7490735025845,31.8565820304227,49.6931337464098));
#31361=CARTESIAN_POINT('Ctrl Pts',(40.6942641376324,31.8523482623022,49.6359876554342));
#31362=CARTESIAN_POINT('Ctrl Pts',(40.6393574214939,31.8481069742559,49.5787400628309));
#31363=CARTESIAN_POINT('Ctrl Pts',(40.5873965671617,31.8438656862097,49.5187886719602));
#31364=CARTESIAN_POINT('Ctrl Pts',(40.5386399076417,31.8396243981635,49.4564783031257));
#31365=CARTESIAN_POINT('Ctrl Pts',(40.4929885381772,31.8356532358749,49.3981364540914));
#31366=CARTESIAN_POINT('Ctrl Pts',(40.4501459827415,31.8316820735863,49.337727110732));
#31367=CARTESIAN_POINT('Ctrl Pts',(40.4102885577865,31.8277109112977,49.2755543177868));
#31368=CARTESIAN_POINT('Ctrl Pts',(40.3669097120312,31.8233888950967,49.2078885315904));
#31369=CARTESIAN_POINT('Ctrl Pts',(40.3269112702481,31.8190668788957,49.1378906414038));
#31370=CARTESIAN_POINT('Ctrl Pts',(40.2905461636704,31.8147448626947,49.065924459469));
#31371=CARTESIAN_POINT('Ctrl Pts',(40.2542398387595,31.8104298327324,48.9940746058644));
#31372=CARTESIAN_POINT('Ctrl Pts',(40.2215553756603,31.8061148027702,48.9202631763286));
#31373=CARTESIAN_POINT('Ctrl Pts',(40.1927018902877,31.8017997728079,48.8448819419069));
#31374=CARTESIAN_POINT('Ctrl Pts',(40.1638961493857,31.7974918830167,48.7696254424033));
#31375=CARTESIAN_POINT('Ctrl Pts',(40.1389089291594,31.7931839932255,48.692804719184));
#31376=CARTESIAN_POINT('Ctrl Pts',(40.1179022731241,31.7888761034343,48.614833640823));
#31377=CARTESIAN_POINT('Ctrl Pts',(40.0969160724432,31.784572408476,48.5369384872566));
#31378=CARTESIAN_POINT('Ctrl Pts',(40.0799028481842,31.7802687135178,48.4578956312762));
#31379=CARTESIAN_POINT('Ctrl Pts',(40.0669753931644,31.7759650185595,48.3781357227233));
#31380=CARTESIAN_POINT('Ctrl Pts',(40.0540580840903,31.7716647013005,48.2984384127022));
#31381=CARTESIAN_POINT('Ctrl Pts',(40.0452202372997,31.7673643840415,48.2180256065206));
#31382=CARTESIAN_POINT('Ctrl Pts',(40.0405236688884,31.7630640667825,48.1373385736929));
#31383=CARTESIAN_POINT('Ctrl Pts',(40.0378434669426,31.7606099944311,48.0912927113866));
#31384=CARTESIAN_POINT('Ctrl Pts',(40.036511003673,31.7581559220797,48.0451577207413));
#31385=CARTESIAN_POINT('Ctrl Pts',(40.0365302046386,31.7557018497283,47.9990164785296));
#31386=CARTESIAN_POINT('',(40.2639804386337,31.6997437308952,46.9881764997223));
#31387=CARTESIAN_POINT('Ctrl Pts',(40.036530204639,31.7557018496867,47.9990164777473));
#31388=CARTESIAN_POINT('Ctrl Pts',(40.0365663398342,31.7510834198396,47.912181185345));
#31389=CARTESIAN_POINT('Ctrl Pts',(40.0413922398844,31.7464649899924,47.8254998942774));
#31390=CARTESIAN_POINT('Ctrl Pts',(40.0509321358632,31.7418465601453,47.7394801148097));
#31391=CARTESIAN_POINT('Ctrl Pts',(40.0605002169713,31.737214485386,47.6532061943516));
#31392=CARTESIAN_POINT('Ctrl Pts',(40.0748100619829,31.7325824106267,47.5675980002164));
#31393=CARTESIAN_POINT('Ctrl Pts',(40.0937349511213,31.7279503358674,47.483151893473));
#31394=CARTESIAN_POINT('Ctrl Pts',(40.1127460894233,31.7232971506768,47.3983209281438));
#31395=CARTESIAN_POINT('Ctrl Pts',(40.1364142967733,31.7186439654861,47.3146629597844));
#31396=CARTESIAN_POINT('Ctrl Pts',(40.1645624236317,31.7139907802954,47.2326609073814));
#31397=CARTESIAN_POINT('Ctrl Pts',(40.1897788092404,31.7098222431609,47.1591997003714));
#31398=CARTESIAN_POINT('Ctrl Pts',(40.2185897699603,31.7056537060265,47.0870672898386));
#31399=CARTESIAN_POINT('Ctrl Pts',(40.2508364890358,31.701485168892,47.0165943644456));
#31400=CARTESIAN_POINT('Ctrl Pts',(40.2551818317863,31.700923445928,47.0070979249863));
#31401=CARTESIAN_POINT('Ctrl Pts',(40.2595901732973,31.700361722964,46.9976301622621));
#31402=CARTESIAN_POINT('Ctrl Pts',(40.2640612763241,31.6998,46.9881916141869));
#31403=CARTESIAN_POINT('',(40.03653,31.6998,48.));
#31404=CARTESIAN_POINT('Origin',(42.4,31.6998,48.));
#31405=CARTESIAN_POINT('',(40.3450946017473,31.6998,49.167627614067));
#31406=CARTESIAN_POINT('Origin',(42.4,31.6998,48.));
#31407=CARTESIAN_POINT('',(40.0365309987239,32.4282731502717,48.0021727647993));
#31408=CARTESIAN_POINT('Ctrl Pts',(40.3450946017473,31.6998,49.167627614067));
#31409=CARTESIAN_POINT('Ctrl Pts',(40.733984951581,31.7418752474686,49.8520349281576));
#31410=CARTESIAN_POINT('Ctrl Pts',(42.2432941503802,31.8260257424058,50.7894931656538));
#31411=CARTESIAN_POINT('Ctrl Pts',(44.6658134148021,31.9522514848118,49.6394916517794));
#31412=CARTESIAN_POINT('Ctrl Pts',(45.002413620778,32.0784772272174,46.9819641293264));
#31413=CARTESIAN_POINT('Ctrl Pts',(42.9528043529522,32.2047029696235,45.2602400010695));
#31414=CARTESIAN_POINT('Ctrl Pts',(40.5894215430047,32.3213015890215,45.9925773628642));
#31415=CARTESIAN_POINT('Ctrl Pts',(40.041973387172,32.3958249609508,47.3953266536232));
#31416=CARTESIAN_POINT('Ctrl Pts',(40.0363942808121,32.4282730854115,48.0021716774805));
#31417=CARTESIAN_POINT('',(40.0365301523602,33.2220231503183,47.9991513555514));
#31418=CARTESIAN_POINT('Ctrl Pts',(40.0365309987239,32.4282731502717,48.0021727647993));
#31419=CARTESIAN_POINT('Ctrl Pts',(40.0366288369523,32.433964126123,48.108598283094));
#31420=CARTESIAN_POINT('Ctrl Pts',(40.043918722001,32.4396551019744,48.2147058241217));
#31421=CARTESIAN_POINT('Ctrl Pts',(40.0582509534344,32.4453460778257,48.319690231019));
#31422=CARTESIAN_POINT('Ctrl Pts',(40.0681637458294,32.4492822033622,48.3923019966833));
#31423=CARTESIAN_POINT('Ctrl Pts',(40.0814443994366,32.4532183288986,48.4643771967112));
#31424=CARTESIAN_POINT('Ctrl Pts',(40.0980306723185,32.4571544544351,48.5356562846768));
#31425=CARTESIAN_POINT('Ctrl Pts',(40.115881679449,32.4613907168865,48.6123705360693));
#31426=CARTESIAN_POINT('Ctrl Pts',(40.1376054805314,32.4656269793378,48.6883366720028));
#31427=CARTESIAN_POINT('Ctrl Pts',(40.1631235815122,32.4698632417892,48.7631345420782));
#31428=CARTESIAN_POINT('Ctrl Pts',(40.1886047934042,32.4740933802793,48.8378242839952));
#31429=CARTESIAN_POINT('Ctrl Pts',(40.2178692624813,32.4783235187694,48.9113486735642));
#31430=CARTESIAN_POINT('Ctrl Pts',(40.2507878209739,32.4825536572596,48.9832992679881));
#31431=CARTESIAN_POINT('Ctrl Pts',(40.2836681061506,32.486778877508,49.0551662078426));
#31432=CARTESIAN_POINT('Ctrl Pts',(40.3201938439724,32.4910040977564,49.1254625643036));
#31433=CARTESIAN_POINT('Ctrl Pts',(40.3601870708306,32.4952293180048,49.1937979958491));
#31434=CARTESIAN_POINT('Ctrl Pts',(40.4001548439042,32.4994518491017,49.2620899351464));
#31435=CARTESIAN_POINT('Ctrl Pts',(40.4435854894103,32.5036743801987,49.3284230228211));
#31436=CARTESIAN_POINT('Ctrl Pts',(40.4902547835621,32.5078969112956,49.3924308417988));
#31437=CARTESIAN_POINT('Ctrl Pts',(40.5369089341258,32.5121180722353,49.4564178910594));
#31438=CARTESIAN_POINT('Ctrl Pts',(40.5867993703725,32.516339233175,49.5180807910649));
#31439=CARTESIAN_POINT('Ctrl Pts',(40.6396589950288,32.5205603941147,49.5770827458053));
#31440=CARTESIAN_POINT('Ctrl Pts',(40.6925179574176,32.5247815021683,49.6360839613222));
#31441=CARTESIAN_POINT('Ctrl Pts',(40.748345720209,32.5290026102219,49.6924239493138));
#31442=CARTESIAN_POINT('Ctrl Pts',(40.8068364142566,32.5332237182755,49.745800741769));
#31443=CARTESIAN_POINT('Ctrl Pts',(40.8653857410508,32.5374490576887,49.7992310406494));
#31444=CARTESIAN_POINT('Ctrl Pts',(40.9266029841594,32.5416743971019,49.8496918932931));
#31445=CARTESIAN_POINT('Ctrl Pts',(40.990147520111,32.5458997365151,49.8969202476253));
#31446=CARTESIAN_POINT('Ctrl Pts',(41.0537226611592,32.550127110988,49.9441713486551));
#31447=CARTESIAN_POINT('Ctrl Pts',(41.1196269373464,32.5543544854608,49.9881865889613));
#31448=CARTESIAN_POINT('Ctrl Pts',(41.1874910744808,32.5585818599337,50.0287465456376));
#31449=CARTESIAN_POINT('Ctrl Pts',(41.2554792674611,32.5628169620597,50.0693806460361));
#31450=CARTESIAN_POINT('Ctrl Pts',(41.3254340649262,32.5670520641858,50.1065466207299));
#31451=CARTESIAN_POINT('Ctrl Pts',(41.3969621315318,32.5712871663118,50.1400713715479));
#31452=CARTESIAN_POINT('Ctrl Pts',(41.4650432204419,32.5753181764882,50.1719805457984));
#31453=CARTESIAN_POINT('Ctrl Pts',(41.5345491053882,32.5793491866646,50.2005912390327));
#31454=CARTESIAN_POINT('Ctrl Pts',(41.6051276134198,32.583380196841,50.2257961114964));
#31455=CARTESIAN_POINT('Ctrl Pts',(41.679276065189,32.5876151002413,50.2522758759791));
#31456=CARTESIAN_POINT('Ctrl Pts',(41.7548904835065,32.5918500036415,50.2750968677632));
#31457=CARTESIAN_POINT('Ctrl Pts',(41.831575399182,32.5960849070417,50.2940976252298));
#31458=CARTESIAN_POINT('Ctrl Pts',(41.9081489701943,32.6003136614635,50.313070794051));
#31459=CARTESIAN_POINT('Ctrl Pts',(41.9857895001044,32.6045424158853,50.3282346316287));
#31460=CARTESIAN_POINT('Ctrl Pts',(42.0640839130019,32.6087711703071,50.3394766131329));
#31461=CARTESIAN_POINT('Ctrl Pts',(42.1422866868052,32.6129949752158,50.3507054365462));
#31462=CARTESIAN_POINT('Ctrl Pts',(42.2211413604342,32.6172187801245,50.3580214592381));
#31463=CARTESIAN_POINT('Ctrl Pts',(42.3002236499624,32.6214425850331,50.3613629794831));
#31464=CARTESIAN_POINT('Ctrl Pts',(42.3792552459753,32.6256636823884,50.3647023577389));
#31465=CARTESIAN_POINT('Ctrl Pts',(42.4585137004836,32.6298847797437,50.3640722704571));
#31466=CARTESIAN_POINT('Ctrl Pts',(42.5375697915496,32.634105877099,50.3594628611938));
#31467=CARTESIAN_POINT('Ctrl Pts',(42.6165999135277,32.6383255878686,50.3548549660727));
#31468=CARTESIAN_POINT('Ctrl Pts',(42.6954273357058,32.6425452986382,50.3462703718458));
#31469=CARTESIAN_POINT('Ctrl Pts',(42.7736245259,32.6467650094078,50.333751305205));
#31470=CARTESIAN_POINT('Ctrl Pts',(42.85182046785,32.650984652819,50.3212324384032));
#31471=CARTESIAN_POINT('Ctrl Pts',(42.9293857344215,32.6552042962303,50.3047792995598));
#31472=CARTESIAN_POINT('Ctrl Pts',(43.0059010863693,32.6594239396416,50.2844855688834));
#31473=CARTESIAN_POINT('Ctrl Pts',(43.0824929371117,32.6636478017831,50.2641715488677));
#31474=CARTESIAN_POINT('Ctrl Pts',(43.1580323214428,32.6678716639247,50.2400093872476));
#31475=CARTESIAN_POINT('Ctrl Pts',(43.2321139099739,32.6720955260663,50.2121430518228));
#31476=CARTESIAN_POINT('Ctrl Pts',(43.3062310277249,32.6763214139545,50.1842633518202));
#31477=CARTESIAN_POINT('Ctrl Pts',(43.3788885257198,32.6805473018427,50.1526761264666));
#31478=CARTESIAN_POINT('Ctrl Pts',(43.4497022551402,32.6847731897309,50.11757304867));
#31479=CARTESIAN_POINT('Ctrl Pts',(43.5206455067916,32.689006807002,50.082405765401));
#31480=CARTESIAN_POINT('Ctrl Pts',(43.5897378404033,32.6932404242731,50.0437100096986));
#31481=CARTESIAN_POINT('Ctrl Pts',(43.6566210405138,32.6974740415442,50.0017227583854));
#31482=CARTESIAN_POINT('Ctrl Pts',(43.7205081052318,32.7015180074451,49.9616163903057));
#31483=CARTESIAN_POINT('Ctrl Pts',(43.7823794542321,32.705561973346,49.9185073546962));
#31484=CARTESIAN_POINT('Ctrl Pts',(43.8419514606082,32.7096059392468,49.8726362236564));
#31485=CARTESIAN_POINT('Ctrl Pts',(43.9043469228363,32.7138415716684,49.8245909990908));
#31486=CARTESIAN_POINT('Ctrl Pts',(43.9644570313206,32.7180772040899,49.7733325933318));
#31487=CARTESIAN_POINT('Ctrl Pts',(44.0219320147086,32.7223128365114,49.7191064482933));
#31488=CARTESIAN_POINT('Ctrl Pts',(44.0793236902889,32.7265423295444,49.6649589019944));
#31489=CARTESIAN_POINT('Ctrl Pts',(44.1340874871881,32.7307718225775,49.6078524780488));
#31490=CARTESIAN_POINT('Ctrl Pts',(44.1859052814896,32.7350013156105,49.548073889208));
#31491=CARTESIAN_POINT('Ctrl Pts',(44.2376625711192,32.7392258701067,49.4883651004031));
#31492=CARTESIAN_POINT('Ctrl Pts',(44.2864803880359,32.7434504246028,49.4259906997908));
#31493=CARTESIAN_POINT('Ctrl Pts',(44.3320772999161,32.747674979099,49.3612743103611));
#31494=CARTESIAN_POINT('Ctrl Pts',(44.3776450568527,32.7518968323892,49.2965993009856));
#31495=CARTESIAN_POINT('Ctrl Pts',(44.4199957267821,32.7561186856795,49.2295856576005));
#31496=CARTESIAN_POINT('Ctrl Pts',(44.4588888182748,32.7603405389697,49.1605891929891));
#31497=CARTESIAN_POINT('Ctrl Pts',(44.4977691849325,32.7645610109764,49.0916153022743));
#31498=CARTESIAN_POINT('Ctrl Pts',(44.5331939891252,32.7687814829831,49.0206602870238));
#31499=CARTESIAN_POINT('Ctrl Pts',(44.5649674630409,32.7730019549899,48.9481067054264));
#31500=CARTESIAN_POINT('Ctrl Pts',(44.596740461947,32.777222363901,48.8755542084961));
#31501=CARTESIAN_POINT('Ctrl Pts',(44.6248620520384,32.7814427728122,48.8014036231594));
#31502=CARTESIAN_POINT('Ctrl Pts',(44.6491842294469,32.7856631817234,48.7260583605381));
#31503=CARTESIAN_POINT('Ctrl Pts',(44.6735307271568,32.7898878107179,48.650637758466));
#31504=CARTESIAN_POINT('Ctrl Pts',(44.6940700784421,32.7941124397125,48.5740205404645));
#31505=CARTESIAN_POINT('Ctrl Pts',(44.7107040998377,32.798337068707,48.4966256174355));
#31506=CARTESIAN_POINT('Ctrl Pts',(44.7273461052669,32.8025637254481,48.4191935462241));
#31507=CARTESIAN_POINT('Ctrl Pts',(44.7400789710655,32.8067903821892,48.3409834902103));
#31508=CARTESIAN_POINT('Ctrl Pts',(44.7488560940843,32.8110170389303,48.2624223507687));
#31509=CARTESIAN_POINT('Ctrl Pts',(44.7576492561023,32.815251419312,48.1837176515242));
#31510=CARTESIAN_POINT('Ctrl Pts',(44.7624722022754,32.8194857996937,48.1046610565485));
#31511=CARTESIAN_POINT('Ctrl Pts',(44.7633304609072,32.8237201800754,48.0256821620638));
#31512=CARTESIAN_POINT('Ctrl Pts',(44.7641487467668,32.8277573472679,47.9503816521985));
#31513=CARTESIAN_POINT('Ctrl Pts',(44.7613634749228,32.8317945144603,47.8751521212201));
#31514=CARTESIAN_POINT('Ctrl Pts',(44.7550232350933,32.8358316816527,47.8003603168944));
#31515=CARTESIAN_POINT('Ctrl Pts',(44.7483713953103,32.840067261073,47.7218927647446));
#31516=CARTESIAN_POINT('Ctrl Pts',(44.7377809076998,32.8443028404933,47.6436089492841));
#31517=CARTESIAN_POINT('Ctrl Pts',(44.7232689731068,32.8485384199136,47.5659358117754));
#31518=CARTESIAN_POINT('Ctrl Pts',(44.7087780695174,32.8527678610423,47.4883752398254));
#31519=CARTESIAN_POINT('Ctrl Pts',(44.6903770899501,32.856997302171,47.4114240458049));
#31520=CARTESIAN_POINT('Ctrl Pts',(44.6681350661798,32.8612267432998,47.3355048815335));
#31521=CARTESIAN_POINT('Ctrl Pts',(44.6459190033573,32.8654512478138,47.2596743303078));
#31522=CARTESIAN_POINT('Ctrl Pts',(44.6198709367108,32.8696757523279,47.1848738631517));
#31523=CARTESIAN_POINT('Ctrl Pts',(44.5901107904022,32.873900256842,47.1115152411751));
#31524=CARTESIAN_POINT('Ctrl Pts',(44.5603696647349,32.8781220613429,47.0382035049912));
#31525=CARTESIAN_POINT('Ctrl Pts',(44.5269213442865,32.8823438658438,46.9663322186796));
#31526=CARTESIAN_POINT('Ctrl Pts',(44.4899349742621,32.8865656703448,46.8962961247435));
#31527=CARTESIAN_POINT('Ctrl Pts',(44.4529606943075,32.8907860948262,46.82628292414));
#31528=CARTESIAN_POINT('Ctrl Pts',(44.412450880239,32.8950065193077,46.7581041394352));
#31529=CARTESIAN_POINT('Ctrl Pts',(44.3686213656833,32.8992269437891,46.6921313676537));
#31530=CARTESIAN_POINT('Ctrl Pts',(44.3247924925016,32.9034473065115,46.626159561277));
#31531=CARTESIAN_POINT('Ctrl Pts',(44.2776442762216,32.9076676692339,46.562394093839));
#31532=CARTESIAN_POINT('Ctrl Pts',(44.2274359277515,32.9118880319562,46.5011776720162));
#31533=CARTESIAN_POINT('Ctrl Pts',(44.1771773450496,32.916112617217,46.4399000022133));
#31534=CARTESIAN_POINT('Ctrl Pts',(44.1238528123531,32.9203372024778,46.3811768364409));
#31535=CARTESIAN_POINT('Ctrl Pts',(44.0677615282317,32.9245617877386,46.3253173656331));
#31536=CARTESIAN_POINT('Ctrl Pts',(44.0116433041987,32.9287884020125,46.2694310662505));
#31537=CARTESIAN_POINT('Ctrl Pts',(43.9527560308078,32.9330150162864,46.2164115162541));
#31538=CARTESIAN_POINT('Ctrl Pts',(43.8914335303496,32.9372416305604,46.1665288479366));
#31539=CARTESIAN_POINT('Ctrl Pts',(43.8299989312255,32.9414759711634,46.116554993178));
#31540=CARTESIAN_POINT('Ctrl Pts',(43.7661205891331,32.9457103117665,46.0697297567315));
#31541=CARTESIAN_POINT('Ctrl Pts',(43.7001627945513,32.9499446523695,46.0262808840758));
#31542=CARTESIAN_POINT('Ctrl Pts',(43.6372697507637,32.9539822429325,45.984850877694));
#31543=CARTESIAN_POINT('Ctrl Pts',(43.5724865318398,32.9580198334955,45.9464905883132));
#31544=CARTESIAN_POINT('Ctrl Pts',(43.5061479811823,32.9620574240585,45.9113575977142));
#31545=CARTESIAN_POINT('Ctrl Pts',(43.4365589853085,32.966292847809,45.8745031667144));
#31546=CARTESIAN_POINT('Ctrl Pts',(43.3649937905135,32.9705282715595,45.8410602963793));
#31547=CARTESIAN_POINT('Ctrl Pts',(43.2918207282089,32.97476369531,45.8112455072263));
#31548=CARTESIAN_POINT('Ctrl Pts',(43.2187537660668,32.9789929777411,45.7814739492006));
#31549=CARTESIAN_POINT('Ctrl Pts',(43.1440839971346,32.9832222601722,45.755320201202));
#31550=CARTESIAN_POINT('Ctrl Pts',(43.0682041896879,32.9874515426033,45.7329548743389));
#31551=CARTESIAN_POINT('Ctrl Pts',(42.9924130213608,32.9916758845913,45.7106156735686));
#31552=CARTESIAN_POINT('Ctrl Pts',(42.915415071303,32.9959002265793,45.6920562317595));
#31553=CARTESIAN_POINT('Ctrl Pts',(42.8376214845264,33.0001245685673,45.6773984678424));
#31554=CARTESIAN_POINT('Ctrl Pts',(42.7598776615587,33.0043462082843,45.6627500803558));
#31555=CARTESIAN_POINT('Ctrl Pts',(42.6813396720579,33.0085678480014,45.6519985036822));
#31556=CARTESIAN_POINT('Ctrl Pts',(42.6024309798725,33.0127894877185,45.6452150545564));
#31557=CARTESIAN_POINT('Ctrl Pts',(42.5235481202644,33.0170097453846,45.6384338261489));
#31558=CARTESIAN_POINT('Ctrl Pts',(42.4442952662404,33.0212300030507,45.6356181859657));
#31559=CARTESIAN_POINT('Ctrl Pts',(42.3651016770439,33.0254502607168,45.6367876633796));
#31560=CARTESIAN_POINT('Ctrl Pts',(42.2859092806767,33.0296704548166,45.6379571231786));
#31561=CARTESIAN_POINT('Ctrl Pts',(42.2067766166628,33.0338906489163,45.6431115729954));
#31562=CARTESIAN_POINT('Ctrl Pts',(42.128132116221,33.0381108430161,45.6522184312271));
#31563=CARTESIAN_POINT('Ctrl Pts',(42.0494089588806,33.0423352579752,45.6613343977528));
#31564=CARTESIAN_POINT('Ctrl Pts',(41.9711754078042,33.0465596729344,45.6744106152543));
#31565=CARTESIAN_POINT('Ctrl Pts',(41.8938533417299,33.0507840878936,45.6913627393586));
#31566=CARTESIAN_POINT('Ctrl Pts',(41.8164941592577,33.0550105306706,45.7083230008784));
#31567=CARTESIAN_POINT('Ctrl Pts',(41.740047786877,33.0592369734476,45.7291627517744));
#31568=CARTESIAN_POINT('Ctrl Pts',(41.6649219867698,33.0634634162246,45.753747397249));
#31569=CARTESIAN_POINT('Ctrl Pts',(41.5896588498976,33.0676975853218,45.7783769856817));
#31570=CARTESIAN_POINT('Ctrl Pts',(41.5157215486243,33.0719317544189,45.806764979937));
#31571=CARTESIAN_POINT('Ctrl Pts',(41.4434986810422,33.076165923516,45.8387282290901));
#31572=CARTESIAN_POINT('Ctrl Pts',(41.3746034611575,33.0802050044988,45.8692187807998));
#31573=CARTESIAN_POINT('Ctrl Pts',(41.3072684728443,33.0842440854816,45.9029621911566));
#31574=CARTESIAN_POINT('Ctrl Pts',(41.2418077577091,33.0882831664644,45.9397618655124));
#31575=CARTESIAN_POINT('Ctrl Pts',(41.1731633574778,33.0925186883492,45.978351293838));
#31576=CARTESIAN_POINT('Ctrl Pts',(41.1063192262536,33.096754210234,46.0204485310013));
#31577=CARTESIAN_POINT('Ctrl Pts',(41.0416567358416,33.1009897321188,46.0658609104784));
#31578=CARTESIAN_POINT('Ctrl Pts',(40.9770879822644,33.1052191140543,46.1112074587033));
#31579=CARTESIAN_POINT('Ctrl Pts',(40.9146949700175,33.1094484959898,46.1598593384299));
#31580=CARTESIAN_POINT('Ctrl Pts',(40.854833677621,33.1136778779252,46.211578495688));
#31581=CARTESIAN_POINT('Ctrl Pts',(40.7950422880421,33.1179023210145,46.2632372580786));
#31582=CARTESIAN_POINT('Ctrl Pts',(40.7377770966868,33.1221267641038,46.3179558750393));
#31583=CARTESIAN_POINT('Ctrl Pts',(40.6833630704725,33.1263512071931,46.3754544964568));
#31584=CARTESIAN_POINT('Ctrl Pts',(40.6289838396155,33.1305729489384,46.4329163500551));
#31585=CARTESIAN_POINT('Ctrl Pts',(40.5774524769848,33.1347946906836,46.4931543398004));
#31586=CARTESIAN_POINT('Ctrl Pts',(40.5290580545538,33.1390164324288,46.5558508810826));
#31587=CARTESIAN_POINT('Ctrl Pts',(40.4806794657617,33.1432367929088,46.6185269093729));
#31588=CARTESIAN_POINT('Ctrl Pts',(40.4354360657627,33.1474571533888,46.6836595206978));
#31589=CARTESIAN_POINT('Ctrl Pts',(40.3935765061138,33.1516775138687,46.7508982411022));
#31590=CARTESIAN_POINT('Ctrl Pts',(40.3517175705451,33.1558978114278,46.8181359590511));
#31591=CARTESIAN_POINT('Ctrl Pts',(40.3132426219625,33.1601181089868,46.8874793245161));
#31592=CARTESIAN_POINT('Ctrl Pts',(40.278356036486,33.1643384065458,46.9585503694444));
#31593=CARTESIAN_POINT('Ctrl Pts',(40.2434345573606,33.1685629252569,47.0296924998073));
#31594=CARTESIAN_POINT('Ctrl Pts',(40.2121088183092,33.1727874439679,47.1025653392601));
#31595=CARTESIAN_POINT('Ctrl Pts',(40.1845361162486,33.177011962679,47.17676842827));
#31596=CARTESIAN_POINT('Ctrl Pts',(40.1569501768173,33.181238509538,47.2510071414195));
#31597=CARTESIAN_POINT('Ctrl Pts',(40.1331210051139,33.185465056397,47.3265769281391));
#31598=CARTESIAN_POINT('Ctrl Pts',(40.1131559989364,33.1896916032561,47.4030620168732));
#31599=CARTESIAN_POINT('Ctrl Pts',(40.0931544990082,33.19392587576,47.4796869116126));
#31600=CARTESIAN_POINT('Ctrl Pts',(40.0770313744407,33.1981601482639,47.5572299908215));
#31601=CARTESIAN_POINT('Ctrl Pts',(40.0648428182954,33.2023944207678,47.6352653325588));
#31602=CARTESIAN_POINT('Ctrl Pts',(40.0532187736082,33.2064325834686,47.7096864771737));
#31603=CARTESIAN_POINT('Ctrl Pts',(40.0451729101829,33.2104707461694,47.7845549367905));
#31604=CARTESIAN_POINT('Ctrl Pts',(40.0407097821507,33.2145089088703,47.8595005022767));
#31605=CARTESIAN_POINT('Ctrl Pts',(40.0379414421964,33.2170136560041,47.9059869131148));
#31606=CARTESIAN_POINT('Ctrl Pts',(40.0365468832596,33.2195184031379,47.9525559457422));
#31607=CARTESIAN_POINT('Ctrl Pts',(40.0365301523605,33.2220231502717,47.9991513546838));
#31608=CARTESIAN_POINT('',(40.0365306333283,34.0157731502431,47.9982697675646));
#31609=CARTESIAN_POINT('Ctrl Pts',(40.0365301523602,33.2220231503183,47.9991513555514));
#31610=CARTESIAN_POINT('Ctrl Pts',(40.0365021154589,33.2262204991601,48.0772339624199));
#31611=CARTESIAN_POINT('Ctrl Pts',(40.0403477846679,33.2304178480019,48.1554743222026));
#31612=CARTESIAN_POINT('Ctrl Pts',(40.0480878668836,33.2346151968436,48.2334518344325));
#31613=CARTESIAN_POINT('Ctrl Pts',(40.0558171140975,33.2388066700007,48.3113201893608));
#31614=CARTESIAN_POINT('Ctrl Pts',(40.0674299063109,33.2429981431578,48.3889259549904));
#31615=CARTESIAN_POINT('Ctrl Pts',(40.0828949330752,33.2471896163149,48.4658482046025));
#31616=CARTESIAN_POINT('Ctrl Pts',(40.0983433617521,33.2513765909064,48.5426878961793));
#31617=CARTESIAN_POINT('Ctrl Pts',(40.1176357195175,33.2555635654978,48.6188450619448));
#31618=CARTESIAN_POINT('Ctrl Pts',(40.1406890375124,33.2597505400893,48.6939051921432));
#31619=CARTESIAN_POINT('Ctrl Pts',(40.1637293049397,33.2639351444191,48.7689228305275));
#31620=CARTESIAN_POINT('Ctrl Pts',(40.1905261684422,33.2681197487489,48.8428442090526));
#31621=CARTESIAN_POINT('Ctrl Pts',(40.220946176901,33.2723043530788,48.9152676531692));
#31622=CARTESIAN_POINT('Ctrl Pts',(40.251358878258,33.276487952237,48.9876737006605));
#31623=CARTESIAN_POINT('Ctrl Pts',(40.2853928113643,33.2806715513951,49.0585820871903));
#31624=CARTESIAN_POINT('Ctrl Pts',(40.3228661062038,33.2848551505533,49.1276104061878));
#31625=CARTESIAN_POINT('Ctrl Pts',(40.3603426120758,33.2890391081981,49.1966446401223));
#31626=CARTESIAN_POINT('Ctrl Pts',(40.4012588342473,33.2932230658428,49.2637980674233));
#31627=CARTESIAN_POINT('Ctrl Pts',(40.445387385082,33.2974070234876,49.3287136510563));
#31628=CARTESIAN_POINT('Ctrl Pts',(40.4895621377561,33.3015953616646,49.3936972001973));
#31629=CARTESIAN_POINT('Ctrl Pts',(40.5369556607667,33.3057836998416,49.4564378340769));
#31630=CARTESIAN_POINT('Ctrl Pts',(40.5872982097622,33.3099720380185,49.5166089346198));
#31631=CARTESIAN_POINT('Ctrl Pts',(40.6376707183786,33.3141628687396,49.576815843905));
#31632=CARTESIAN_POINT('Ctrl Pts',(40.6909954190013,33.3183536994607,49.6344498273763));
#31633=CARTESIAN_POINT('Ctrl Pts',(40.7469651827797,33.3225445301818,49.6892206291534));
#31634=CARTESIAN_POINT('Ctrl Pts',(40.8030277856186,33.3267423123846,49.7440822812297));
#31635=CARTESIAN_POINT('Ctrl Pts',(40.8617438479482,33.3309400945874,49.7960709592963));
#31636=CARTESIAN_POINT('Ctrl Pts',(40.922773184784,33.3351378767901,49.8449366865307));
#31637=CARTESIAN_POINT('Ctrl Pts',(40.9498960335329,33.3370034682855,49.8666537458582));
#31638=CARTESIAN_POINT('Ctrl Pts',(40.9774754008023,33.3388690597808,49.8877545615961));
#31639=CARTESIAN_POINT('Ctrl Pts',(41.005479749451,33.3407346512761,49.9082200375504));
#31640=CARTESIAN_POINT('Ctrl Pts',(41.069058596954,33.3449701419377,49.9546832276463));
#31641=CARTESIAN_POINT('Ctrl Pts',(41.1350829584756,33.3492056325992,49.9980537394834));
#31642=CARTESIAN_POINT('Ctrl Pts',(41.2032193813288,33.3534411232608,50.0380644228466));
#31643=CARTESIAN_POINT('Ctrl Pts',(41.2712570252651,33.3576704736355,50.078017101815));
#31644=CARTESIAN_POINT('Ctrl Pts',(41.341400248826,33.3618998240102,50.114619389241));
#31645=CARTESIAN_POINT('Ctrl Pts',(41.4132848266376,33.366129174385,50.1476460619842));
#31646=CARTESIAN_POINT('Ctrl Pts',(41.4850854547547,33.3703535855546,50.1806341648538));
#31647=CARTESIAN_POINT('Ctrl Pts',(41.5586229716564,33.3745779967243,50.2100547560943));
#31648=CARTESIAN_POINT('Ctrl Pts',(41.6335079770185,33.3788024078939,50.2357281631732));
#31649=CARTESIAN_POINT('Ctrl Pts',(41.7083450927587,33.3830241175153,50.2613851518817));
#31650=CARTESIAN_POINT('Ctrl Pts',(41.7845275438216,33.3872458271367,50.2832995608808));
#31651=CARTESIAN_POINT('Ctrl Pts',(41.8616464758864,33.3914675367582,50.3013400278913));
#31652=CARTESIAN_POINT('Ctrl Pts',(41.9387401731499,33.3956878649548,50.3193745917131));
#31653=CARTESIAN_POINT('Ctrl Pts',(42.0167692862679,33.3999081931514,50.3335376238067));
#31654=CARTESIAN_POINT('Ctrl Pts',(42.0953117925022,33.4041285213481,50.3437481812498));
#31655=CARTESIAN_POINT('Ctrl Pts',(42.1738531256036,33.4083487865087,50.3539585861852));
#31656=CARTESIAN_POINT('Ctrl Pts',(42.2529073709692,33.4125690516694,50.3602165746351));
#31657=CARTESIAN_POINT('Ctrl Pts',(42.3320458456057,33.41678931683,50.3624928939154));
#31658=CARTESIAN_POINT('Ctrl Pts',(42.411263476228,33.4210138031896,50.3647714900186));
#31659=CARTESIAN_POINT('Ctrl Pts',(42.4905650341362,33.4252382895492,50.3630604477787));
#31660=CARTESIAN_POINT('Ctrl Pts',(42.5695208910285,33.4294627759089,50.3573826817903));
#31661=CARTESIAN_POINT('Ctrl Pts',(42.6485146535901,33.4336892903889,50.3517021899811));
#31662=CARTESIAN_POINT('Ctrl Pts',(42.7271619180104,33.4379158048689,50.3420512379268));
#31663=CARTESIAN_POINT('Ctrl Pts',(42.8050398132651,33.4421423193489,50.3285044965751));
#31664=CARTESIAN_POINT('Ctrl Pts',(42.8830600677609,33.4463765598132,50.31493299205));
#31665=CARTESIAN_POINT('Ctrl Pts',(42.9603076838087,33.4506108002775,50.2974515718185));
#31666=CARTESIAN_POINT('Ctrl Pts',(43.0363717860428,33.4548450407418,50.276185710971));
#31667=CARTESIAN_POINT('Ctrl Pts',(43.1089187164316,33.4588834917218,50.255903174515));
#31668=CARTESIAN_POINT('Ctrl Pts',(43.1803888367674,33.4629219427019,50.232178591211));
#31669=CARTESIAN_POINT('Ctrl Pts',(43.250443301507,33.4669603936819,50.2051613618559));
#31670=CARTESIAN_POINT('Ctrl Pts',(43.3239160109902,33.4711958972536,50.1768258510382));
#31671=CARTESIAN_POINT('Ctrl Pts',(43.3961106755326,33.4754314008253,50.1447604597992));
#31672=CARTESIAN_POINT('Ctrl Pts',(43.4666222177561,33.479666904397,50.1091011084083));
#31673=CARTESIAN_POINT('Ctrl Pts',(43.5370315412657,33.4838962678714,50.0734934514339));
#31674=CARTESIAN_POINT('Ctrl Pts',(43.6057621725277,33.4881256313459,50.0343023906085));
#31675=CARTESIAN_POINT('Ctrl Pts',(43.6724276485817,33.4923549948203,49.991712408965));
#31676=CARTESIAN_POINT('Ctrl Pts',(43.7390152737942,33.496579419314,49.9491721631983));
#31677=CARTESIAN_POINT('Ctrl Pts',(43.8035421427342,33.5008038438076,49.9032411355331));
#31678=CARTESIAN_POINT('Ctrl Pts',(43.8656464826084,33.5050282683013,49.8541496241991));
#31679=CARTESIAN_POINT('Ctrl Pts',(43.9277111082535,33.5092499913772,49.8050895057038));
#31680=CARTESIAN_POINT('Ctrl Pts',(43.98735591235,33.5134717144532,49.7528732051682));
#31681=CARTESIAN_POINT('Ctrl Pts',(44.0442492281593,33.5176934375292,49.6977735174627));
#31682=CARTESIAN_POINT('Ctrl Pts',(44.101123928947,33.5219137792923,49.6426918579185));
#31683=CARTESIAN_POINT('Ctrl Pts',(44.1552485921758,33.5261341210555,49.5847290108015));
#31684=CARTESIAN_POINT('Ctrl Pts',(44.2063268313671,33.5303544628186,49.5241961222832));
#31685=CARTESIAN_POINT('Ctrl Pts',(44.2574043087735,33.5345747416393,49.4636641365573));
#31686=CARTESIAN_POINT('Ctrl Pts',(44.3054351507928,33.5387950204599,49.4005625451917));
#31687=CARTESIAN_POINT('Ctrl Pts',(44.3501628408623,33.5430152992805,49.3352360596613));
#31688=CARTESIAN_POINT('Ctrl Pts',(44.3949352689227,33.5472397993519,49.2698442326006));
#31689=CARTESIAN_POINT('Ctrl Pts',(44.4363976792592,33.5514642994233,49.202223454044));
#31690=CARTESIAN_POINT('Ctrl Pts',(44.4743369181271,33.5556887994947,49.1327474524338));
#31691=CARTESIAN_POINT('Ctrl Pts',(44.5122943715217,33.5599153277372,49.0632380955816));
#31692=CARTESIAN_POINT('Ctrl Pts',(44.5467250796167,33.5641418559798,48.9918721646229));
#31693=CARTESIAN_POINT('Ctrl Pts',(44.5774630728789,33.5683683842223,48.9190457046027));
#31694=CARTESIAN_POINT('Ctrl Pts',(44.6082572538374,33.5726026383721,48.8460861210251));
#31695=CARTESIAN_POINT('Ctrl Pts',(44.6353450706936,33.5768368925219,48.7716611157403));
#31696=CARTESIAN_POINT('Ctrl Pts',(44.6586097711944,33.5810711466717,48.6961841296418));
#31697=CARTESIAN_POINT('Ctrl Pts',(44.6807979843064,33.585109476477,48.6241995600339));
#31698=CARTESIAN_POINT('Ctrl Pts',(44.6995090032818,33.5891478062824,48.5512585643751));
#31699=CARTESIAN_POINT('Ctrl Pts',(44.7146851706425,33.5931861360878,48.4777269112241));
#31700=CARTESIAN_POINT('Ctrl Pts',(44.7306023130197,33.5974216369854,48.4006050816728));
#31701=CARTESIAN_POINT('Ctrl Pts',(44.7426911152079,33.601657137883,48.3225402899882));
#31702=CARTESIAN_POINT('Ctrl Pts',(44.750846746316,33.6058926387806,48.2439467487705));
#31703=CARTESIAN_POINT('Ctrl Pts',(44.7589905543899,33.6101219995683,48.1654671428329));
#31704=CARTESIAN_POINT('Ctrl Pts',(44.763212466175,33.6143513603559,48.086460772424));
#31705=CARTESIAN_POINT('Ctrl Pts',(44.7634585636582,33.6185807211436,48.0073524669862));
#31706=CARTESIAN_POINT('Ctrl Pts',(44.7637043737522,33.6228051429444,47.9283365430936));
#31707=CARTESIAN_POINT('Ctrl Pts',(44.7599835943962,33.6270295647452,47.8492193876342));
#31708=CARTESIAN_POINT('Ctrl Pts',(44.7522941966099,33.631253986546,47.7704298505999));
#31709=CARTESIAN_POINT('Ctrl Pts',(44.7446097160159,33.6354757069265,47.6916906976552));
#31710=CARTESIAN_POINT('Ctrl Pts',(44.7329616995274,33.6396974273071,47.6132792131841));
#31711=CARTESIAN_POINT('Ctrl Pts',(44.7174001461527,33.6439191476877,47.5356219174944));
#31712=CARTESIAN_POINT('Ctrl Pts',(44.7018436843879,33.6481394867567,47.4579900306215));
#31713=CARTESIAN_POINT('Ctrl Pts',(44.6823763204877,33.6523598258258,47.3811123023922));
#31714=CARTESIAN_POINT('Ctrl Pts',(44.6590993943052,33.6565801648948,47.3054063291752));
#31715=CARTESIAN_POINT('Ctrl Pts',(44.635822815249,33.6608004410264,47.2297014849533));
#31716=CARTESIAN_POINT('Ctrl Pts',(44.6087369260511,33.665020717158,47.1551688092414));
#31717=CARTESIAN_POINT('Ctrl Pts',(44.5779928652158,33.6692409932895,47.0822105252461));
#31718=CARTESIAN_POINT('Ctrl Pts',(44.5472180530222,33.673465490699,47.0091792656491));
#31719=CARTESIAN_POINT('Ctrl Pts',(44.5127779424928,33.6776899881084,46.9377259771127));
#31720=CARTESIAN_POINT('Ctrl Pts',(44.4748715351361,33.6819144855179,46.8682321114372));
#31721=CARTESIAN_POINT('Ctrl Pts',(44.4369469289101,33.6861410111089,46.7987048817509));
#31722=CARTESIAN_POINT('Ctrl Pts',(44.3955529561559,33.6903675366999,46.7311393497179));
#31723=CARTESIAN_POINT('Ctrl Pts',(44.3509329135256,33.6945940622909,46.6658893569787));
#31724=CARTESIAN_POINT('Ctrl Pts',(44.3062313068501,33.6988283138388,46.6005200892895));
#31725=CARTESIAN_POINT('Ctrl Pts',(44.2582921312371,33.7030625653866,46.5374751934799));
#31726=CARTESIAN_POINT('Ctrl Pts',(44.2073999398629,33.7072968169345,46.4770765290785));
#31727=CARTESIAN_POINT('Ctrl Pts',(44.1588622762872,33.7113351707875,46.4194722095557));
#31728=CARTESIAN_POINT('Ctrl Pts',(44.107639066577,33.7153735246406,46.3642749174909));
#31729=CARTESIAN_POINT('Ctrl Pts',(44.0540067454563,33.7194118784936,46.3117310264993));
#31730=CARTESIAN_POINT('Ctrl Pts',(43.9977561900654,33.7236473775798,46.2566220364553));
#31731=CARTESIAN_POINT('Ctrl Pts',(43.9386414792717,33.7278828766661,46.2042226495555));
#31732=CARTESIAN_POINT('Ctrl Pts',(43.8769542643098,33.7321183757523,46.1548451170601));
#31733=CARTESIAN_POINT('Ctrl Pts',(43.8153564765458,33.7363477346875,46.1055391665671));
#31734=CARTESIAN_POINT('Ctrl Pts',(43.7511939537218,33.7405770936227,46.0592466619137));
#31735=CARTESIAN_POINT('Ctrl Pts',(43.6847948196123,33.7448064525579,46.016242778867));
#31736=CARTESIAN_POINT('Ctrl Pts',(43.6184732263326,33.7490308724528,45.9732891157038));
#31737=CARTESIAN_POINT('Ctrl Pts',(43.5499206040223,33.7532552923477,45.9336166962783));
#31738=CARTESIAN_POINT('Ctrl Pts',(43.4794965294163,33.7574797122426,45.8974592313398));
#31739=CARTESIAN_POINT('Ctrl Pts',(43.4091174899281,33.7617014306856,45.8613248885467));
#31740=CARTESIAN_POINT('Ctrl Pts',(43.3368697898738,33.7659231491286,45.8287012527122));
#31741=CARTESIAN_POINT('Ctrl Pts',(43.2631391934012,33.7701448675717,45.7997770172742));
#31742=CARTESIAN_POINT('Ctrl Pts',(43.1894327214801,33.7743652046741,45.770862245807));
#31743=CARTESIAN_POINT('Ctrl Pts',(43.1142447531929,33.7785855417766,45.7456446424839));
#31744=CARTESIAN_POINT('Ctrl Pts',(43.0379813224048,33.782805878879,45.7242648938941));
#31745=CARTESIAN_POINT('Ctrl Pts',(42.9617190294029,33.7870261530176,45.7028854642723));
#31746=CARTESIAN_POINT('Ctrl Pts',(42.8843817580829,33.7912464271562,45.6853439009779));
#31747=CARTESIAN_POINT('Ctrl Pts',(42.8063895537328,33.7954667012948,45.6717306917977));
#31748=CARTESIAN_POINT('Ctrl Pts',(42.7283193391435,33.7996911966834,45.6581038662604));
#31749=CARTESIAN_POINT('Ctrl Pts',(42.6495933463761,33.803915692072,45.6484133249306));
#31750=CARTESIAN_POINT('Ctrl Pts',(42.5706400448906,33.8081401874606,45.642698064316));
#31751=CARTESIAN_POINT('Ctrl Pts',(42.4916488382462,33.8123667110122,45.636980059828));
#31752=CARTESIAN_POINT('Ctrl Pts',(42.412430575367,33.8165932345639,45.6352411483672));
#31753=CARTESIAN_POINT('Ctrl Pts',(42.3334144681154,33.8208197581155,45.637468136121));
#31754=CARTESIAN_POINT('Ctrl Pts',(42.254253921957,33.8250540076165,45.6396991947369));
#31755=CARTESIAN_POINT('Ctrl Pts',(42.1752967389788,33.8292882571175,45.645910601936));
#31756=CARTESIAN_POINT('Ctrl Pts',(42.0969675526403,33.8335225066185,45.6560371639578));
#31757=CARTESIAN_POINT('Ctrl Pts',(42.0222619057637,33.8375608780455,45.6656952671736));
#31758=CARTESIAN_POINT('Ctrl Pts',(41.9481277827892,33.8415992494725,45.6789142031845));
#31759=CARTESIAN_POINT('Ctrl Pts',(41.8749219445824,33.8456376208995,45.6955947672732));
#31760=CARTESIAN_POINT('Ctrl Pts',(41.7981426318956,33.8498731216483,45.7130895774868));
#31761=CARTESIAN_POINT('Ctrl Pts',(41.72209268972,33.8541086223971,45.7344590981521));
#31762=CARTESIAN_POINT('Ctrl Pts',(41.6471925112131,33.8583441231458,45.7596269672828));
#31763=CARTESIAN_POINT('Ctrl Pts',(41.5724009140803,33.8625734837691,45.784758351029));
#31764=CARTESIAN_POINT('Ctrl Pts',(41.4987562118072,33.8668028443925,45.8136770002822));
#31765=CARTESIAN_POINT('Ctrl Pts',(41.4266673473084,33.8710322050158,45.8462558211096));
#31766=CARTESIAN_POINT('Ctrl Pts',(41.3546626675442,33.8752566266294,45.8787965966799));
#31767=CARTESIAN_POINT('Ctrl Pts',(41.2842106405299,33.879481048243,45.9149888576775));
#31768=CARTESIAN_POINT('Ctrl Pts',(41.2157023516839,33.8837054698566,45.9546566251378));
#31769=CARTESIAN_POINT('Ctrl Pts',(41.1472378725322,33.8879271900363,45.9942990258461));
#31770=CARTESIAN_POINT('Ctrl Pts',(41.0807150695741,33.8921489102159,46.0374122872457));
#31771=CARTESIAN_POINT('Ctrl Pts',(41.0165013345407,33.8963706303955,46.0837740520564));
#31772=CARTESIAN_POINT('Ctrl Pts',(40.9523086099107,33.9005909692501,46.1301206475365));
#31773=CARTESIAN_POINT('Ctrl Pts',(40.8904238332502,33.9048113081046,46.1797133613383));
#31774=CARTESIAN_POINT('Ctrl Pts',(40.8311849869034,33.9090316469591,46.2322868175005));
#31775=CARTESIAN_POINT('Ctrl Pts',(40.771947024166,33.9132519228629,46.2848594894745));
#31776=CARTESIAN_POINT('Ctrl Pts',(40.715355263448,33.9174721987667,46.3404125028882));
#31777=CARTESIAN_POINT('Ctrl Pts',(40.6617130485338,33.9216924746704,46.3986415406716));
#31778=CARTESIAN_POINT('Ctrl Pts',(40.6080171789178,33.9259169718325,46.4569288210476));
#31779=CARTESIAN_POINT('Ctrl Pts',(40.5572770673334,33.9301414689946,46.5178971267101));
#31780=CARTESIAN_POINT('Ctrl Pts',(40.5097573093474,33.9343659661566,46.5812071992943));
#31781=CARTESIAN_POINT('Ctrl Pts',(40.4622147372448,33.9385924914892,46.6445476668856));
#31782=CARTESIAN_POINT('Ctrl Pts',(40.4178958616058,33.9428190168218,46.7102317514898));
#31783=CARTESIAN_POINT('Ctrl Pts',(40.3770217860997,33.9470455421544,46.7778913358524));
#31784=CARTESIAN_POINT('Ctrl Pts',(40.3360729942093,33.9512797934278,46.8456745995751));
#31785=CARTESIAN_POINT('Ctrl Pts',(40.298581808044,33.9555140447013,46.9154401644476));
#31786=CARTESIAN_POINT('Ctrl Pts',(40.2647231209757,33.9597482959747,46.9867956322616));
#31787=CARTESIAN_POINT('Ctrl Pts',(40.2324308889635,33.9637866517516,47.0548498753969));
#31788=CARTESIAN_POINT('Ctrl Pts',(40.2034425813174,33.9678250075285,47.1243498189802));
#31789=CARTESIAN_POINT('Ctrl Pts',(40.177867767415,33.9718633633054,47.194941752538));
#31790=CARTESIAN_POINT('Ctrl Pts',(40.1467834353712,33.9767716919587,47.2807411296398));
#31791=CARTESIAN_POINT('Ctrl Pts',(40.1206435182197,33.981680020612,47.3684219008596));
#31792=CARTESIAN_POINT('Ctrl Pts',(40.0996463022741,33.9865883492653,47.4574474161349));
#31793=CARTESIAN_POINT('Ctrl Pts',(40.0788348930446,33.9914532435684,47.5456851346521));
#31794=CARTESIAN_POINT('Ctrl Pts',(40.0630756547469,33.9963181378716,47.6352437461937));
#31795=CARTESIAN_POINT('Ctrl Pts',(40.0525154170653,34.0011830321747,47.7255795674808));
#31796=CARTESIAN_POINT('Ctrl Pts',(40.0419584823543,34.0060464048642,47.8158871340487));
#31797=CARTESIAN_POINT('Ctrl Pts',(40.0365974704945,34.0109097775536,47.906971285491));
#31798=CARTESIAN_POINT('Ctrl Pts',(40.0365306333283,34.0157731502431,47.9982697675646));
#31799=CARTESIAN_POINT('',(40.0365305376038,34.8095231503011,48.0015941206072));
#31800=CARTESIAN_POINT('Ctrl Pts',(40.0365306333279,34.0157731502717,47.9982697681018));
#31801=CARTESIAN_POINT('Ctrl Pts',(40.0364725206114,34.020001694087,48.0776508183265));
#31802=CARTESIAN_POINT('Ctrl Pts',(40.0404179459887,34.0242302379023,48.1570685937256));
#31803=CARTESIAN_POINT('Ctrl Pts',(40.048351385374,34.0284587817177,48.2360915801712));
#31804=CARTESIAN_POINT('Ctrl Pts',(40.0562842671246,34.0326870283122,48.3151090121576));
#31805=CARTESIAN_POINT('Ctrl Pts',(40.0682045589376,34.0369152749067,48.3937312464129));
#31806=CARTESIAN_POINT('Ctrl Pts',(40.0840448505842,34.0411435215013,48.471531745267));
#31807=CARTESIAN_POINT('Ctrl Pts',(40.0998888941178,34.0453727695864,48.5493506717282));
#31808=CARTESIAN_POINT('Ctrl Pts',(40.1196546870358,34.0496020176715,48.6263470196808));
#31809=CARTESIAN_POINT('Ctrl Pts',(40.1432239853927,34.0538312657566,48.702105733343));
#31810=CARTESIAN_POINT('Ctrl Pts',(40.1668223317924,34.0580657261895,48.7779578160282));
#31811=CARTESIAN_POINT('Ctrl Pts',(40.1942334000401,34.0623001866224,48.8525687743477));
#31812=CARTESIAN_POINT('Ctrl Pts',(40.225289637487,34.0665346470552,48.9255405340008));
#31813=CARTESIAN_POINT('Ctrl Pts',(40.2563674008764,34.0707720425105,48.9985628724116));
#31814=CARTESIAN_POINT('Ctrl Pts',(40.2910951577676,34.0750094379658,49.0699433321022));
#31815=CARTESIAN_POINT('Ctrl Pts',(40.32925907647,34.079246833421,49.1393078901325));
#31816=CARTESIAN_POINT('Ctrl Pts',(40.367491204594,34.0834918022677,49.20879642171));
#31817=CARTESIAN_POINT('Ctrl Pts',(40.4091715081891,34.0877367711143,49.2762614638197));
#31818=CARTESIAN_POINT('Ctrl Pts',(40.4540427571723,34.0919817399609,49.3413578381575));
#31819=CARTESIAN_POINT('Ctrl Pts',(40.4755619672545,34.0940175285443,49.372576549174));
#31820=CARTESIAN_POINT('Ctrl Pts',(40.4978144785519,34.0960533171277,49.4032509714174));
#31821=CARTESIAN_POINT('Ctrl Pts',(40.5207687907589,34.0980891057111,49.4333459118839));
#31822=CARTESIAN_POINT('Ctrl Pts',(40.5685257106106,34.1023246058357,49.4959590560652));
#31823=CARTESIAN_POINT('Ctrl Pts',(40.6195060929958,34.1065601059603,49.5563018166407));
#31824=CARTESIAN_POINT('Ctrl Pts',(40.6734661316249,34.1107956060848,49.6140233090801));
#31825=CARTESIAN_POINT('Ctrl Pts',(40.7273479452908,34.1150249660759,49.6716611236397));
#31826=CARTESIAN_POINT('Ctrl Pts',(40.784200519511,34.119254326067,49.7266848762439));
#31827=CARTESIAN_POINT('Ctrl Pts',(40.8437386309448,34.1234836860581,49.778775138146));
#31828=CARTESIAN_POINT('Ctrl Pts',(40.9032072141622,34.1277081070302,49.8308045693816));
#31829=CARTESIAN_POINT('Ctrl Pts',(40.9653547510696,34.1319325280024,49.8799070099948));
#31830=CARTESIAN_POINT('Ctrl Pts',(41.0298589387366,34.1361569489746,49.9257995516512));
#31831=CARTESIAN_POINT('Ctrl Pts',(41.0943218771653,34.1403786685075,49.9716627458737));
#31832=CARTESIAN_POINT('Ctrl Pts',(41.1611380938088,34.1446003880404,50.0143198438972));
#31833=CARTESIAN_POINT('Ctrl Pts',(41.2299529072174,34.1488221075733,50.0535287291808));
#31834=CARTESIAN_POINT('Ctrl Pts',(41.2987452046983,34.1530424457766,50.0927247854763));
#31835=CARTESIAN_POINT('Ctrl Pts',(41.3695343929576,34.15726278398,50.1284746371659));
#31836=CARTESIAN_POINT('Ctrl Pts',(41.4419388392728,34.1614831221834,50.1605807675729));
#31837=CARTESIAN_POINT('Ctrl Pts',(41.5143422055393,34.1657033974325,50.1926864190565));
#31838=CARTESIAN_POINT('Ctrl Pts',(41.5883603523654,34.1699236726816,50.2211482682615));
#31839=CARTESIAN_POINT('Ctrl Pts',(41.6635905745683,34.1741439479307,50.2458164660175));
#31840=CARTESIAN_POINT('Ctrl Pts',(41.7388960445005,34.1783684444372,50.270509337712));
#31841=CARTESIAN_POINT('Ctrl Pts',(41.8154155645938,34.1825929409436,50.291400831307));
#31842=CARTESIAN_POINT('Ctrl Pts',(41.8927307010451,34.1868174374501,50.3083908462905));
#31843=CARTESIAN_POINT('Ctrl Pts',(41.9700829562763,34.1910439621255,50.3253890181325));
#31844=CARTESIAN_POINT('Ctrl Pts',(42.0482311252671,34.1952704868008,50.3384819022801));
#31845=CARTESIAN_POINT('Ctrl Pts',(42.1267485474494,34.1994970114762,50.3476209414169));
#31846=CARTESIAN_POINT('Ctrl Pts',(42.2054094968579,34.2037312620975,50.356776686412));
#31847=CARTESIAN_POINT('Ctrl Pts',(42.2844405786557,34.2079655127189,50.3619641133402));
#31848=CARTESIAN_POINT('Ctrl Pts',(42.3634121985332,34.2121997633402,50.3631867834947));
#31849=CARTESIAN_POINT('Ctrl Pts',(42.4387303563637,34.2162381249325,50.3643528892908));
#31850=CARTESIAN_POINT('Ctrl Pts',(42.513994076582,34.2202764865248,50.3619130169859));
#31851=CARTESIAN_POINT('Ctrl Pts',(42.5888360551186,34.224314848117,50.3559141294171));
#31852=CARTESIAN_POINT('Ctrl Pts',(42.6673315582741,34.2285503484513,50.3496223970592));
#31853=CARTESIAN_POINT('Ctrl Pts',(42.7456614707067,34.2327858487856,50.3393913836042));
#31854=CARTESIAN_POINT('Ctrl Pts',(42.8233987915123,34.2370213491198,50.3252363114845));
#31855=CARTESIAN_POINT('Ctrl Pts',(42.901023417895,34.241250709324,50.3111017597231));
#31856=CARTESIAN_POINT('Ctrl Pts',(42.9780567007583,34.2454800695281,50.2930545292986));
#31857=CARTESIAN_POINT('Ctrl Pts',(43.0540756881294,34.2497094297322,50.2711616928564));
#31858=CARTESIAN_POINT('Ctrl Pts',(43.1300059011028,34.2539338509215,50.2492944227027));
#31859=CARTESIAN_POINT('Ctrl Pts',(43.2049237237017,34.2581582721109,50.2235905999403));
#31860=CARTESIAN_POINT('Ctrl Pts',(43.2784168589071,34.2623826933002,50.1941682394219));
#31861=CARTESIAN_POINT('Ctrl Pts',(43.3518629966521,34.2666044130526,50.1647646939427));
#31862=CARTESIAN_POINT('Ctrl Pts',(43.4238858207104,34.270826132805,50.131647504368));
#31863=CARTESIAN_POINT('Ctrl Pts',(43.4940898246073,34.2750478525574,50.0949839848053));
#31864=CARTESIAN_POINT('Ctrl Pts',(43.5642708580748,34.2792681909824,50.0583324613788));
#31865=CARTESIAN_POINT('Ctrl Pts',(43.6326338373523,34.2834885294074,50.0181371291271));
#31866=CARTESIAN_POINT('Ctrl Pts',(43.6988061852967,34.2877088678324,49.9746120970801));
#31867=CARTESIAN_POINT('Ctrl Pts',(43.7649775461838,34.2919291433049,49.9310877142726));
#31868=CARTESIAN_POINT('Ctrl Pts',(43.8289579492947,34.2961494187773,49.8842339894366));
#31869=CARTESIAN_POINT('Ctrl Pts',(43.8904035071785,34.3003696942498,49.8343085418463));
#31870=CARTESIAN_POINT('Ctrl Pts',(43.9519105249346,34.3045941909809,49.7843331571776));
#31871=CARTESIAN_POINT('Ctrl Pts',(44.0108772674731,34.308818687712,49.7312802088515));
#31872=CARTESIAN_POINT('Ctrl Pts',(44.0669931783131,34.3130431844431,49.6754474579519));
#31873=CARTESIAN_POINT('Ctrl Pts',(44.1231360302568,34.3172697093442,49.619587901893));
#31874=CARTESIAN_POINT('Ctrl Pts',(44.1764250078465,34.3214962342452,49.5609462324549));
#31875=CARTESIAN_POINT('Ctrl Pts',(44.2265884532666,34.3257227591463,49.4998550140907));
#31876=CARTESIAN_POINT('Ctrl Pts',(44.2768435957747,34.3299570099924,49.4386521230379));
#31877=CARTESIAN_POINT('Ctrl Pts',(44.3239615095059,34.3341912608386,49.3749911138297));
#31878=CARTESIAN_POINT('Ctrl Pts',(44.3677127827298,34.3384255116848,49.3092352140016));
#31879=CARTESIAN_POINT('Ctrl Pts',(44.4094399692409,34.3424638712975,49.2465214117702));
#31880=CARTESIAN_POINT('Ctrl Pts',(44.4481049796522,34.3465022309102,49.1819025916229));
#31881=CARTESIAN_POINT('Ctrl Pts',(44.4835486028899,34.3505405905229,49.1157130725664));
#31882=CARTESIAN_POINT('Ctrl Pts',(44.5207224779323,34.354776090788,49.0462923789195));
#31883=CARTESIAN_POINT('Ctrl Pts',(44.5544937239808,34.3590115910531,48.9748798342005));
#31884=CARTESIAN_POINT('Ctrl Pts',(44.5846441396699,34.3632470913182,48.9018427933437));
#31885=CARTESIAN_POINT('Ctrl Pts',(44.6147508468276,34.3674764514524,48.8289116330103));
#31886=CARTESIAN_POINT('Ctrl Pts',(44.6412469697431,34.3717058115867,48.7543610833301));
#31887=CARTESIAN_POINT('Ctrl Pts',(44.6639601049717,34.375935171721,48.6785831444979));
#31888=CARTESIAN_POINT('Ctrl Pts',(44.6866467159688,34.3801595928398,48.6028936985827));
#31889=CARTESIAN_POINT('Ctrl Pts',(44.7055589841037,34.3843840139585,48.5259801590757));
#31890=CARTESIAN_POINT('Ctrl Pts',(44.7205731139964,34.3886084350773,48.4482531243582));
#31891=CARTESIAN_POINT('Ctrl Pts',(44.7355776426375,34.3928301547587,48.3705757946073));
#31892=CARTESIAN_POINT('Ctrl Pts',(44.7466888919066,34.3970518744402,48.292086461749));
#31893=CARTESIAN_POINT('Ctrl Pts',(44.7538336120224,34.4012735941217,48.213208273324));
#31894=CARTESIAN_POINT('Ctrl Pts',(44.7609759944178,34.4054939324754,48.1343558934879));
#31895=CARTESIAN_POINT('Ctrl Pts',(44.764154382413,34.4097142708292,48.0551153778093));
#31896=CARTESIAN_POINT('Ctrl Pts',(44.7633472866427,34.4139346091829,47.9759159052734));
#31897=CARTESIAN_POINT('Ctrl Pts',(44.7625402029114,34.418154884584,47.8967176141169));
#31898=CARTESIAN_POINT('Ctrl Pts',(44.757747759704,34.422375159985,47.8175608341996));
#31899=CARTESIAN_POINT('Ctrl Pts',(44.7490005818709,34.4265954353861,47.7388741543426));
#31900=CARTESIAN_POINT('Ctrl Pts',(44.7402446548217,34.430819932046,47.6601087694699));
#31901=CARTESIAN_POINT('Ctrl Pts',(44.7275261432045,34.4350444287058,47.581814891553));
#31902=CARTESIAN_POINT('Ctrl Pts',(44.71092746403,34.4392689253657,47.5044147935097));
#31903=CARTESIAN_POINT('Ctrl Pts',(44.6943208158723,34.4434954501955,47.426977535879));
#31904=CARTESIAN_POINT('Ctrl Pts',(44.6738304106541,34.4477219750253,47.3504353669544));
#31905=CARTESIAN_POINT('Ctrl Pts',(44.6495889798429,34.4519484998552,47.2751966731111));
#31906=CARTESIAN_POINT('Ctrl Pts',(44.6253032365076,34.4561827506309,47.1998204454535));
#31907=CARTESIAN_POINT('Ctrl Pts',(44.5972529328508,34.4604170014067,47.1257528941725));
#31908=CARTESIAN_POINT('Ctrl Pts',(44.5656194436254,34.4646512521825,47.0533834639668));
#31909=CARTESIAN_POINT('Ctrl Pts',(44.5354494248471,34.4686896124312,46.9843620843543));
#31910=CARTESIAN_POINT('Ctrl Pts',(44.5020206202816,34.47272797268,46.9168854827684));
#31911=CARTESIAN_POINT('Ctrl Pts',(44.4655280698614,34.4767663329287,46.8512684240805));
#31912=CARTESIAN_POINT('Ctrl Pts',(44.4272540683125,34.4810018331784,46.782448147697));
#31913=CARTESIAN_POINT('Ctrl Pts',(44.3854640708046,34.4852373334281,46.7154120032883));
#31914=CARTESIAN_POINT('Ctrl Pts',(44.3403489880603,34.4894728336778,46.6505422402189));
#31915=CARTESIAN_POINT('Ctrl Pts',(44.2952993078694,34.4937021937961,46.5857665177206));
#31916=CARTESIAN_POINT('Ctrl Pts',(44.2469343804596,34.4979315539145,46.5231513220195));
#31917=CARTESIAN_POINT('Ctrl Pts',(44.1954906201956,34.5021609140329,46.4630537180208));
#31918=CARTESIAN_POINT('Ctrl Pts',(44.1441069355828,34.5063853351351,46.4030262955695));
#31919=CARTESIAN_POINT('Ctrl Pts',(44.0896518665518,34.5106097562374,46.3455109771495));
#31920=CARTESIAN_POINT('Ctrl Pts',(44.0324037656135,34.5148341773396,46.2908340083799));
#31921=CARTESIAN_POINT('Ctrl Pts',(43.9751922737569,34.5190558970041,46.2361920045014));
#31922=CARTESIAN_POINT('Ctrl Pts',(43.9151916335014,34.5232776166686,46.1843850710417));
#31923=CARTESIAN_POINT('Ctrl Pts',(43.8527180962922,34.5274993363332,46.1357037323416));
#31924=CARTESIAN_POINT('Ctrl Pts',(43.7902650001494,34.5317196746696,46.0870383219612));
#31925=CARTESIAN_POINT('Ctrl Pts',(43.7253409836413,34.5359400130061,46.0414967639062));
#31926=CARTESIAN_POINT('Ctrl Pts',(43.6582953727722,34.5401603513425,45.9993293135151));
#31927=CARTESIAN_POINT('Ctrl Pts',(43.591250761995,34.5443806267259,45.9571624921186));
#31928=CARTESIAN_POINT('Ctrl Pts',(43.5220850177789,34.5486009021093,45.9183699270908));
#31929=CARTESIAN_POINT('Ctrl Pts',(43.4511751631312,34.5528211774927,45.883157724979));
#31930=CARTESIAN_POINT('Ctrl Pts',(43.3801943821118,34.5570456741345,45.8479103024631));
#31931=CARTESIAN_POINT('Ctrl Pts',(43.3074664271477,34.5612701707763,45.8162506060025));
#31932=CARTESIAN_POINT('Ctrl Pts',(43.2333910285123,34.5654946674181,45.7883377666345));
#31933=CARTESIAN_POINT('Ctrl Pts',(43.1592800664735,34.5697211922296,45.760411526386));
#31934=CARTESIAN_POINT('Ctrl Pts',(43.0838208196378,34.5739477170411,45.7362358701697));
#31935=CARTESIAN_POINT('Ctrl Pts',(43.0074285589998,34.5781742418525,45.7159201006507));
#31936=CARTESIAN_POINT('Ctrl Pts',(42.9308966558697,34.5824084926097,45.695567194586));
#31937=CARTESIAN_POINT('Ctrl Pts',(42.8534287911998,34.5866427433669,45.6790883721612));
#31938=CARTESIAN_POINT('Ctrl Pts',(42.7754506211068,34.5908769941241,45.6665417783876));
#31939=CARTESIAN_POINT('Ctrl Pts',(42.7010799773968,34.5949153545276,45.6545756312698));
#31940=CARTESIAN_POINT('Ctrl Pts',(42.6262455599381,34.5989537149311,45.6461859265064));
#31941=CARTESIAN_POINT('Ctrl Pts',(42.5513176098108,34.6029920753346,45.641378915158));
#31942=CARTESIAN_POINT('Ctrl Pts',(42.4727319161874,34.6072275756102,45.6363372408506));
#31943=CARTESIAN_POINT('Ctrl Pts',(42.3937446037544,34.6114630758858,45.635217818096));
#31944=CARTESIAN_POINT('Ctrl Pts',(42.3147804360375,34.6156985761613,45.6380668792665));
#31945=CARTESIAN_POINT('Ctrl Pts',(42.235930741297,34.619927936306,45.6409118102027));
#31946=CARTESIAN_POINT('Ctrl Pts',(42.1571045897222,34.6241572964507,45.6477137837584));
#31947=CARTESIAN_POINT('Ctrl Pts',(42.0787301810835,34.6283866565954,45.6584671378874));
#31948=CARTESIAN_POINT('Ctrl Pts',(42.0004472975019,34.6326110777245,45.6692079343287));
#31949=CARTESIAN_POINT('Ctrl Pts',(41.9226155711116,34.6368354988536,45.6838908782171));
#31950=CARTESIAN_POINT('Ctrl Pts',(41.8456599699784,34.6410599199826,45.7024583633771));
#31951=CARTESIAN_POINT('Ctrl Pts',(41.7687535804959,34.6452816396743,45.7210139749818));
#31952=CARTESIAN_POINT('Ctrl Pts',(41.6927226592897,34.6495033593661,45.7434490876825));
#31953=CARTESIAN_POINT('Ctrl Pts',(41.6179826348283,34.6537250790578,45.7696548963289));
#31954=CARTESIAN_POINT('Ctrl Pts',(41.5432670649687,34.6579454174216,45.7958521305518));
#31955=CARTESIAN_POINT('Ctrl Pts',(41.4698419957355,34.6621657557855,45.8258174557124));
#31956=CARTESIAN_POINT('Ctrl Pts',(41.3981068812904,34.6663860941494,45.8593924648403));
#31957=CARTESIAN_POINT('Ctrl Pts',(41.3263728368844,34.6706063695605,45.8929669731456));
#31958=CARTESIAN_POINT('Ctrl Pts',(41.2563291216867,34.6748266449716,45.9301508582183));
#31959=CARTESIAN_POINT('Ctrl Pts',(41.1883530433289,34.6790469203827,45.9707385350109));
#31960=CARTESIAN_POINT('Ctrl Pts',(41.1203089730569,34.6832714170523,46.0113668089357));
#31961=CARTESIAN_POINT('Ctrl Pts',(41.0543370748975,34.687495913722,46.055405434477));
#31962=CARTESIAN_POINT('Ctrl Pts',(40.9907874331974,34.6917204103917,46.1026043157882));
#31963=CARTESIAN_POINT('Ctrl Pts',(40.92720728148,34.6959469352312,46.1498258571593));
#31964=CARTESIAN_POINT('Ctrl Pts',(40.8660520656411,34.7001734600706,46.2002103779536));
#31965=CARTESIAN_POINT('Ctrl Pts',(40.8076383703661,34.7043999849101,46.2534677554166));
#31966=CARTESIAN_POINT('Ctrl Pts',(40.7491178968157,34.7086342356952,46.3068224855789));
#31967=CARTESIAN_POINT('Ctrl Pts',(40.6933492891554,34.7128684864804,46.3630602319651));
#31968=CARTESIAN_POINT('Ctrl Pts',(40.64061172531,34.7171027372655,46.4218544617865));
#31969=CARTESIAN_POINT('Ctrl Pts',(40.5903139778477,34.7211410974238,46.4779286735658));
#31970=CARTESIAN_POINT('Ctrl Pts',(40.5427732208033,34.7251794575822,46.5363277566628));
#31971=CARTESIAN_POINT('Ctrl Pts',(40.4981950087289,34.7292178177405,46.5967437097678));
#31972=CARTESIAN_POINT('Ctrl Pts',(40.4511793296354,34.7334769891256,46.6604631128379));
#31973=CARTESIAN_POINT('Ctrl Pts',(40.407280079481,34.7377361605108,46.7266690778517));
#31974=CARTESIAN_POINT('Ctrl Pts',(40.3667688384094,34.7419953318959,46.7950263552936));
#31975=CARTESIAN_POINT('Ctrl Pts',(40.3263172950927,34.7462482269251,46.8632829007934));
#31976=CARTESIAN_POINT('Ctrl Pts',(40.2892440808813,34.7505011219543,46.933684070064));
#31977=CARTESIAN_POINT('Ctrl Pts',(40.2557791489135,34.7547540169835,47.0058634989773));
#31978=CARTESIAN_POINT('Ctrl Pts',(40.2223534731393,34.7590019231345,47.0779582574765));
#31979=CARTESIAN_POINT('Ctrl Pts',(40.1925278654198,34.7632498292854,47.1518267152404));
#31980=CARTESIAN_POINT('Ctrl Pts',(40.166487024296,34.7674977354364,47.2270768290044));
#31981=CARTESIAN_POINT('Ctrl Pts',(40.1404699613832,34.7717417627722,47.3022582309678));
#31982=CARTESIAN_POINT('Ctrl Pts',(40.1182309459455,34.775985790108,47.378818345628));
#31983=CARTESIAN_POINT('Ctrl Pts',(40.0999065078837,34.7802298174438,47.456345359236));
#31984=CARTESIAN_POINT('Ctrl Pts',(40.0815916823042,34.7844716184829,47.5338317043641));
#31985=CARTESIAN_POINT('Ctrl Pts',(40.0671874585047,34.7887134195219,47.612283491084));
#31986=CARTESIAN_POINT('Ctrl Pts',(40.0567801120093,34.7929552205609,47.6912752076284));
#31987=CARTESIAN_POINT('Ctrl Pts',(40.0463738175627,34.7971965928085,47.7702589391271));
#31988=CARTESIAN_POINT('Ctrl Pts',(40.039963661291,34.8014379650561,47.8497820342824));
#31989=CARTESIAN_POINT('Ctrl Pts',(40.0375843491048,34.8056793373036,47.9294115214396));
#31990=CARTESIAN_POINT('Ctrl Pts',(40.0368655855772,34.806960608293,47.953466696472));
#31991=CARTESIAN_POINT('Ctrl Pts',(40.036514307811,34.8082418792823,47.9775315541757));
#31992=CARTESIAN_POINT('Ctrl Pts',(40.0365305376034,34.8095231502717,48.0015941200547));
#31993=CARTESIAN_POINT('',(40.0365302359838,35.6032731502447,48.0010561633842));
#31994=CARTESIAN_POINT('Ctrl Pts',(40.0365305376038,34.8095231503011,48.0015941206072));
#31995=CARTESIAN_POINT('Ctrl Pts',(40.0365912402537,34.8143153568354,48.0915928690318));
#31996=CARTESIAN_POINT('Ctrl Pts',(40.041796590266,34.8191075633696,48.1813911678018));
#31997=CARTESIAN_POINT('Ctrl Pts',(40.0520539960474,34.8238997699039,48.2704440855758));
#31998=CARTESIAN_POINT('Ctrl Pts',(40.0623637324262,34.8287164250207,48.3599513280101));
#31999=CARTESIAN_POINT('Ctrl Pts',(40.0777770724225,34.8335330801374,48.4487053652302));
#32000=CARTESIAN_POINT('Ctrl Pts',(40.0981505996024,34.8383497352542,48.5361714080302));
#32001=CARTESIAN_POINT('Ctrl Pts',(40.1186432407031,34.8431945509674,48.624148821454));
#32002=CARTESIAN_POINT('Ctrl Pts',(40.1441541195929,34.8480393666806,48.7108229431661));
#32003=CARTESIAN_POINT('Ctrl Pts',(40.1744893222028,34.8528841823937,48.795671203394));
#32004=CARTESIAN_POINT('Ctrl Pts',(40.179831062548,34.8537373083113,48.8106121741438));
#32005=CARTESIAN_POINT('Ctrl Pts',(40.1853222779565,34.8545904342288,48.8254965869542));
#32006=CARTESIAN_POINT('Ctrl Pts',(40.1909617610073,34.8554435601464,48.8403216643452));
#32007=CARTESIAN_POINT('Ctrl Pts',(40.2189600101066,34.8596790604108,48.9139234831599));
#32008=CARTESIAN_POINT('Ctrl Pts',(40.2506939558323,34.8639145606751,48.9862643795161));
#32009=CARTESIAN_POINT('Ctrl Pts',(40.2860295377095,34.8681500609395,49.0569386573795));
#32010=CARTESIAN_POINT('Ctrl Pts',(40.3213138942085,34.8723794210728,49.1275104799722));
#32011=CARTESIAN_POINT('Ctrl Pts',(40.3601893103022,34.8766087812062,49.1964200657025));
#32012=CARTESIAN_POINT('Ctrl Pts',(40.4024730778727,34.8808381413395,49.2632801099822));
#32013=CARTESIAN_POINT('Ctrl Pts',(40.4447074667689,34.8850625624571,49.3300620755916));
#32014=CARTESIAN_POINT('Ctrl Pts',(40.4903420480824,34.8892869835746,49.3947988613403));
#32015=CARTESIAN_POINT('Ctrl Pts',(40.5391481857246,34.8935114046921,49.4571276423869));
#32016=CARTESIAN_POINT('Ctrl Pts',(40.587923112764,34.8977331243722,49.5194165653557));
#32017=CARTESIAN_POINT('Ctrl Pts',(40.6398652821042,34.9019548440522,49.5793001714016));
#32018=CARTESIAN_POINT('Ctrl Pts',(40.6947034233684,34.9061765637322,49.6364455464905));
#32019=CARTESIAN_POINT('Ctrl Pts',(40.7495236218367,34.9103969020844,49.6935722238668));
#32020=CARTESIAN_POINT('Ctrl Pts',(40.8072375859817,34.9146172404365,49.7479621109285));
#32021=CARTESIAN_POINT('Ctrl Pts',(40.8675355327081,34.9188375787886,49.7993173976227));
#32022=CARTESIAN_POINT('Ctrl Pts',(40.9278325799971,34.9230578541879,49.8506719182732));
#32023=CARTESIAN_POINT('Ctrl Pts',(40.9907131750664,34.9272781295871,49.8989916252247));
#32024=CARTESIAN_POINT('Ctrl Pts',(41.0558337870064,34.9314984049863,49.944018423973));
#32025=CARTESIAN_POINT('Ctrl Pts',(41.1210195347285,34.9357229016441,49.9890902600092));
#32026=CARTESIAN_POINT('Ctrl Pts',(41.1884493881031,34.9399473983019,50.0308623407405));
#32027=CARTESIAN_POINT('Ctrl Pts',(41.2577506006802,34.9441718949597,50.0691198009428));
#32028=CARTESIAN_POINT('Ctrl Pts',(41.327085084588,34.9483984197872,50.1073956284515));
#32029=CARTESIAN_POINT('Ctrl Pts',(41.3982922951244,34.9526249446148,50.1421532678384));
#32030=CARTESIAN_POINT('Ctrl Pts',(41.4709769530811,34.9568514694424,50.1732249352503));
#32031=CARTESIAN_POINT('Ctrl Pts',(41.5437944761557,34.9610857202156,50.2043534006284));
#32032=CARTESIAN_POINT('Ctrl Pts',(41.618094401867,34.9653199709889,50.231782267287));
#32033=CARTESIAN_POINT('Ctrl Pts',(41.6934638296276,34.9695542217621,50.2553928883579));
#32034=CARTESIAN_POINT('Ctrl Pts',(41.7653464172302,34.9735925820255,50.2779112036472));
#32035=CARTESIAN_POINT('Ctrl Pts',(41.8382013829943,34.9776309422888,50.2969566951741));
#32036=CARTESIAN_POINT('Ctrl Pts',(41.911663217944,34.9816693025522,50.3124700275228));
#32037=CARTESIAN_POINT('Ctrl Pts',(41.9887112278512,34.9859048028197,50.328740671801));
#32038=CARTESIAN_POINT('Ctrl Pts',(42.0667197466616,34.9901403030872,50.3411873420431));
#32039=CARTESIAN_POINT('Ctrl Pts',(42.1452750470471,34.9943758033547,50.3497033087697));
#32040=CARTESIAN_POINT('Ctrl Pts',(42.2237164671818,34.9986051634912,50.3582069300477));
#32041=CARTESIAN_POINT('Ctrl Pts',(42.3027026321385,35.0028345236277,50.362791113416));
#32042=CARTESIAN_POINT('Ctrl Pts',(42.381808964351,35.0070638837642,50.3633999930444));
#32043=CARTESIAN_POINT('Ctrl Pts',(42.4608229167689,35.011288304885,50.3640081616275));
#32044=CARTESIAN_POINT('Ctrl Pts',(42.5399562906803,35.0155127260058,50.3606502480517));
#32045=CARTESIAN_POINT('Ctrl Pts',(42.6187802500317,35.0197371471265,50.3533222565335));
#32046=CARTESIAN_POINT('Ctrl Pts',(42.6975538029512,35.0239588668099,50.3459989511274));
#32047=CARTESIAN_POINT('Ctrl Pts',(42.7760178679561,35.0281805864932,50.3347106500631));
#32048=CARTESIAN_POINT('Ctrl Pts',(42.8537457000342,35.0324023061765,50.3195053956826));
#32049=CARTESIAN_POINT('Ctrl Pts',(42.9314480999121,35.036622644532,50.3043051163935));
#32050=CARTESIAN_POINT('Ctrl Pts',(43.008414284923,35.0408429828875,50.2851905186792));
#32051=CARTESIAN_POINT('Ctrl Pts',(43.0842261984354,35.0450633212429,50.2622610261141));
#32052=CARTESIAN_POINT('Ctrl Pts',(43.1600369810961,35.0492835966455,50.2393318755777));
#32053=CARTESIAN_POINT('Ctrl Pts',(43.2346930776167,35.0535038720481,50.2125880804597));
#32054=CARTESIAN_POINT('Ctrl Pts',(43.3077915759767,35.0577241474507,50.1821789329672));
#32055=CARTESIAN_POINT('Ctrl Pts',(43.3809631898641,35.0619486441119,50.151739369243));
#32056=CARTESIAN_POINT('Ctrl Pts',(43.4525736589824,35.066173140773,50.1176273101401));
#32057=CARTESIAN_POINT('Ctrl Pts',(43.52224062299,35.0703976374342,50.0800400056276));
#32058=CARTESIAN_POINT('Ctrl Pts',(43.5919410339249,35.0746241622652,50.0424346555484));
#32059=CARTESIAN_POINT('Ctrl Pts',(43.6596956790694,35.0788506870962,50.0013509799785));
#32060=CARTESIAN_POINT('Ctrl Pts',(43.7251496048058,35.0830772119271,49.95703065019));
#32061=CARTESIAN_POINT('Ctrl Pts',(43.790723178124,35.0873114627038,49.9126293043246));
#32062=CARTESIAN_POINT('Ctrl Pts',(43.8539872522894,35.0915457134804,49.8649797648117));
#32063=CARTESIAN_POINT('Ctrl Pts',(43.9146186662522,35.0957799642571,49.8143651056886));
#32064=CARTESIAN_POINT('Ctrl Pts',(43.9724450690735,35.0998183244907,49.7660920492676));
#32065=CARTESIAN_POINT('Ctrl Pts',(44.0278767779848,35.1038566847244,49.7151224274638));
#32066=CARTESIAN_POINT('Ctrl Pts',(44.0806661529964,35.107895044958,49.6617315436232));
#32067=CARTESIAN_POINT('Ctrl Pts',(44.1360325390962,35.1121305452241,49.6057342849271));
#32068=CARTESIAN_POINT('Ctrl Pts',(44.1887024828509,35.1163660454902,49.5468604738782));
#32069=CARTESIAN_POINT('Ctrl Pts',(44.2383623988095,35.1206015457562,49.4854003270308));
#32070=CARTESIAN_POINT('Ctrl Pts',(44.2879503236526,35.1248309058913,49.4240292778883));
#32071=CARTESIAN_POINT('Ctrl Pts',(44.3345365935244,35.1290602660263,49.3600797005107));
#32072=CARTESIAN_POINT('Ctrl Pts',(44.3778445308435,35.1332896261614,49.2938784536085));
#32073=CARTESIAN_POINT('Ctrl Pts',(44.4211018934708,35.1375140472807,49.2277545160374));
#32074=CARTESIAN_POINT('Ctrl Pts',(44.461088275703,35.1417384684,49.1593845249455));
#32075=CARTESIAN_POINT('Ctrl Pts',(44.4975683203187,35.1459628895193,49.0891269818049));
#32076=CARTESIAN_POINT('Ctrl Pts',(44.5340250366355,35.1501846092011,49.018914367035));
#32077=CARTESIAN_POINT('Ctrl Pts',(44.5669796499953,35.1544063288829,48.9468170113821));
#32078=CARTESIAN_POINT('Ctrl Pts',(44.5962416999364,35.1586280485648,48.8732198098763));
#32079=CARTESIAN_POINT('Ctrl Pts',(44.6254941754652,35.1628483869187,48.799646689047));
#32080=CARTESIAN_POINT('Ctrl Pts',(44.6510563133627,35.1670687252727,48.7245751326297));
#32081=CARTESIAN_POINT('Ctrl Pts',(44.6727855665659,35.1712890636266,48.6484105252922));
#32082=CARTESIAN_POINT('Ctrl Pts',(44.6945144956437,35.1755093390277,48.5722470540676));
#32083=CARTESIAN_POINT('Ctrl Pts',(44.712410526193,35.1797296144288,48.4949910160413));
#32084=CARTESIAN_POINT('Ctrl Pts',(44.7263812451759,35.1839498898299,48.4170620373444));
#32085=CARTESIAN_POINT('Ctrl Pts',(44.7403659381325,35.1881743864895,48.3390551115142));
#32086=CARTESIAN_POINT('Ctrl Pts',(44.7504173933706,35.1923988831492,48.2603743635062));
#32087=CARTESIAN_POINT('Ctrl Pts',(44.75649464996,35.1966233798089,48.1814480796533));
#32088=CARTESIAN_POINT('Ctrl Pts',(44.7625748242244,35.2008499046383,48.1024839034978));
#32089=CARTESIAN_POINT('Ctrl Pts',(44.7646769863967,35.2050764294678,48.023274426495));
#32090=CARTESIAN_POINT('Ctrl Pts',(44.7628123619134,35.2093029542972,47.9442489167004));
#32091=CARTESIAN_POINT('Ctrl Pts',(44.7609443289591,35.2135372050724,47.8650789509233));
#32092=CARTESIAN_POINT('Ctrl Pts',(44.7550950545986,35.2177714558475,47.7860940936335));
#32093=CARTESIAN_POINT('Ctrl Pts',(44.7453277846642,35.2220057066227,47.7077192729887));
#32094=CARTESIAN_POINT('Ctrl Pts',(44.7360123811323,35.2260440668698,47.6329703322973));
#32095=CARTESIAN_POINT('Ctrl Pts',(44.723133581382,35.2300824271168,47.5587765774757));
#32096=CARTESIAN_POINT('Ctrl Pts',(44.7067889521281,35.2341207873639,47.4854952174762));
#32097=CARTESIAN_POINT('Ctrl Pts',(44.6896464295898,35.23835628763,47.4086364924533));
#32098=CARTESIAN_POINT('Ctrl Pts',(44.6686258934281,35.242591787896,47.3324893607809));
#32099=CARTESIAN_POINT('Ctrl Pts',(44.6438017768508,35.246827288162,47.2574745613104));
#32100=CARTESIAN_POINT('Ctrl Pts',(44.6190136473631,35.2510566482971,47.1825685094887));
#32101=CARTESIAN_POINT('Ctrl Pts',(44.5904330334664,35.2552860084321,47.1087919719138));
#32102=CARTESIAN_POINT('Ctrl Pts',(44.5581851522933,35.2595153685672,47.0365544699774));
#32103=CARTESIAN_POINT('Ctrl Pts',(44.5259749299596,35.2637397896865,46.9644013264664));
#32104=CARTESIAN_POINT('Ctrl Pts',(44.490106141021,35.2679642108057,46.8937840734335));
#32105=CARTESIAN_POINT('Ctrl Pts',(44.4507529690236,35.272188631925,46.8250945991524));
#32106=CARTESIAN_POINT('Ctrl Pts',(44.4114249626358,35.2764103516068,46.7564490504918));
#32107=CARTESIAN_POINT('Ctrl Pts',(44.3686172283732,35.2806320712886,46.6897292399323));
#32108=CARTESIAN_POINT('Ctrl Pts',(44.32255043627,35.2848537909704,46.6253035750035));
#32109=CARTESIAN_POINT('Ctrl Pts',(44.276498717016,35.2890741293244,46.5608989898654));
#32110=CARTESIAN_POINT('Ctrl Pts',(44.2271903301258,35.2932944676783,46.4987874413494));
#32111=CARTESIAN_POINT('Ctrl Pts',(44.1748890987347,35.2975148060322,46.4393081251917));
#32112=CARTESIAN_POINT('Ctrl Pts',(44.1225886474974,35.3017350814333,46.37982969626));
#32113=CARTESIAN_POINT('Ctrl Pts',(44.0672957514324,35.3059553568343,46.3229837732254));
#32114=CARTESIAN_POINT('Ctrl Pts',(44.0093133332261,35.3101756322354,46.2690750922121));
#32115=CARTESIAN_POINT('Ctrl Pts',(43.9512729190941,35.314400128895,46.2151124899592));
#32116=CARTESIAN_POINT('Ctrl Pts',(43.8905379534679,35.3186246255546,46.1640933189559));
#32117=CARTESIAN_POINT('Ctrl Pts',(43.8274464776591,35.3228491222143,46.1162837277555));
#32118=CARTESIAN_POINT('Ctrl Pts',(43.7643247117978,35.3270756470437,46.0684511832955));
#32119=CARTESIAN_POINT('Ctrl Pts',(43.6988445703532,35.3313021718731,46.0238315529827));
#32120=CARTESIAN_POINT('Ctrl Pts',(43.6313731526737,35.3355286967025,45.9826476262749));
#32121=CARTESIAN_POINT('Ctrl Pts',(43.5637783995047,35.3397629474776,45.9413884167297));
#32122=CARTESIAN_POINT('Ctrl Pts',(43.4941855100515,35.3439971982527,45.9035776850628));
#32123=CARTESIAN_POINT('Ctrl Pts',(43.4229860762779,35.3482314490278,45.8693921222708));
#32124=CARTESIAN_POINT('Ctrl Pts',(43.3550805651844,35.3522698092751,45.8367880973457));
#32125=CARTESIAN_POINT('Ctrl Pts',(43.2857142139623,35.3563081695224,45.8074813394831));
#32126=CARTESIAN_POINT('Ctrl Pts',(43.2152402281285,35.3603465297697,45.7815830393407));
#32127=CARTESIAN_POINT('Ctrl Pts',(43.1413259244272,35.3645820300361,45.7544204658119));
#32128=CARTESIAN_POINT('Ctrl Pts',(43.0659121183401,35.3688175303026,45.7309043765296));
#32129=CARTESIAN_POINT('Ctrl Pts',(42.9893929307821,35.373053030569,45.7111997872151));
#32130=CARTESIAN_POINT('Ctrl Pts',(42.9129846717578,35.3772823907044,45.6915237633006));
#32131=CARTESIAN_POINT('Ctrl Pts',(42.8354746641284,35.3815117508398,45.6756483828109));
#32132=CARTESIAN_POINT('Ctrl Pts',(42.7572750682811,35.3857411109752,45.6636898822107));
#32133=CARTESIAN_POINT('Ctrl Pts',(42.6791667933487,35.3899655320949,45.6517453466598));
#32134=CARTESIAN_POINT('Ctrl Pts',(42.6003709920194,35.3941899532146,45.6437086719844));
#32135=CARTESIAN_POINT('Ctrl Pts',(42.5213114851465,35.3984143743342,45.6396453731544));
#32136=CARTESIAN_POINT('Ctrl Pts',(42.4423025353339,35.4026360940164,45.6355846727272));
#32137=CARTESIAN_POINT('Ctrl Pts',(42.3630306821481,35.4068578136986,45.6354923290302));
#32138=CARTESIAN_POINT('Ctrl Pts',(42.2839251472717,35.4110795333808,45.6393820577094));
#32139=CARTESIAN_POINT('Ctrl Pts',(42.2048454953741,35.4152998717352,45.6432705136867));
#32140=CARTESIAN_POINT('Ctrl Pts',(42.125932522159,35.4195202100895,45.6511384318469));
#32141=CARTESIAN_POINT('Ctrl Pts',(42.0476142268314,35.4237405484438,45.6629474315351));
#32142=CARTESIAN_POINT('Ctrl Pts',(41.9692970997422,35.4279608238453,45.6747562550738));
#32143=CARTESIAN_POINT('Ctrl Pts',(41.8915750968142,35.4321810992468,45.6905059719863));
#32144=CARTESIAN_POINT('Ctrl Pts',(41.814868388276,35.4364013746482,45.7101066754407));
#32145=CARTESIAN_POINT('Ctrl Pts',(41.7380849551596,35.4406258713082,45.7297269841648));
#32146=CARTESIAN_POINT('Ctrl Pts',(41.6623193009106,35.4448503679683,45.7532058575779));
#32147=CARTESIAN_POINT('Ctrl Pts',(41.5879781414048,35.4490748646283,45.7804029775512));
#32148=CARTESIAN_POINT('Ctrl Pts',(41.5136012909027,35.4533013894581,45.8076131547907));
#32149=CARTESIAN_POINT('Ctrl Pts',(41.4406507302551,35.4575279142879,45.838544951297));
#32150=CARTESIAN_POINT('Ctrl Pts',(41.3695124292721,35.4617544391177,45.8730101534151));
#32151=CARTESIAN_POINT('Ctrl Pts',(41.2982440898598,35.4659886898932,45.9075383567672));
#32152=CARTESIAN_POINT('Ctrl Pts',(41.2287950424061,35.4702229406688,45.9456126459984));
#32153=CARTESIAN_POINT('Ctrl Pts',(41.161525736918,35.4744571914443,45.9869992696018));
#32154=CARTESIAN_POINT('Ctrl Pts',(41.0973685333625,35.4784955516881,46.0264712102698));
#32155=CARTESIAN_POINT('Ctrl Pts',(41.035194121869,35.4825339119318,46.0689555518998));
#32156=CARTESIAN_POINT('Ctrl Pts',(40.9752870980793,35.4865722721756,46.1142153919387));
#32157=CARTESIAN_POINT('Ctrl Pts',(40.9131124855492,35.4907634916275,46.1611883984343));
#32158=CARTESIAN_POINT('Ctrl Pts',(40.8531332119513,35.4949547110795,46.2113381526252));
#32159=CARTESIAN_POINT('Ctrl Pts',(40.795697314067,35.4991459305314,46.2644299689128));
#32160=CARTESIAN_POINT('Ctrl Pts',(40.7362412652663,35.5034845646861,46.3193891449053));
#32161=CARTESIAN_POINT('Ctrl Pts',(40.6795113023837,35.5078231988408,46.3775009674271));
#32162=CARTESIAN_POINT('Ctrl Pts',(40.6258601075221,35.5121618329955,46.4384565062674));
#32163=CARTESIAN_POINT('Ctrl Pts',(40.5741683302032,35.5163420140926,46.4971858625887));
#32164=CARTESIAN_POINT('Ctrl Pts',(40.5253347037497,35.5205221951896,46.5585544384093));
#32165=CARTESIAN_POINT('Ctrl Pts',(40.4796388749424,35.5247023762866,46.6222469051868));
#32166=CARTESIAN_POINT('Ctrl Pts',(40.4339704875959,35.5288800470829,46.6859011230829));
#32167=CARTESIAN_POINT('Ctrl Pts',(40.3914364389047,35.5330577178791,46.7518760741883));
#32168=CARTESIAN_POINT('Ctrl Pts',(40.3522756935313,35.5372353886753,46.8198239090724));
#32169=CARTESIAN_POINT('Ctrl Pts',(40.3131256126739,35.5414119217803,46.8877532399478));
#32170=CARTESIAN_POINT('Ctrl Pts',(40.2773472508029,35.5455884548853,46.9576539720652));
#32171=CARTESIAN_POINT('Ctrl Pts',(40.2451349916197,35.5497649879903,47.0291512802923));
#32172=CARTESIAN_POINT('Ctrl Pts',(40.2129209329773,35.5539417544071,47.1006525825418));
#32173=CARTESIAN_POINT('Ctrl Pts',(40.1842735669987,35.5581185208239,47.1737501990012));
#32174=CARTESIAN_POINT('Ctrl Pts',(40.1593395727421,35.5622952872407,47.2480483455564));
#32175=CARTESIAN_POINT('Ctrl Pts',(40.1343816814018,35.566476056728,47.322417700479));
#32176=CARTESIAN_POINT('Ctrl Pts',(40.1131444144949,35.5706568262153,47.3979894250277));
#32177=CARTESIAN_POINT('Ctrl Pts',(40.0957246066908,35.5748375957026,47.4743524444177));
#32178=CARTESIAN_POINT('Ctrl Pts',(40.0782947730842,35.5790207713914,47.5507594138075));
#32179=CARTESIAN_POINT('Ctrl Pts',(40.064686851524,35.5832039470803,47.6279581114337));
#32180=CARTESIAN_POINT('Ctrl Pts',(40.0549461281531,35.5873871227692,47.7055296635727));
#32181=CARTESIAN_POINT('Ctrl Pts',(40.0451907017365,35.5915766127142,47.7832183053804));
#32182=CARTESIAN_POINT('Ctrl Pts',(40.0393141504531,35.5957661026593,47.8612804466963));
#32183=CARTESIAN_POINT('Ctrl Pts',(40.0373097124553,35.5999555926044,47.9392954199253));
#32184=CARTESIAN_POINT('Ctrl Pts',(40.0367806234985,35.6010614451512,47.95988815507));
#32185=CARTESIAN_POINT('Ctrl Pts',(40.036521040056,35.6021672976979,47.9804776262913));
#32186=CARTESIAN_POINT('Ctrl Pts',(40.0365302359838,35.6032731502447,48.0010561633842));
#32187=CARTESIAN_POINT('',(40.0365309734993,36.3970231502996,47.9978548492323));
#32188=CARTESIAN_POINT('Ctrl Pts',(40.036530235984,35.6032731502717,48.0010561638867));
#32189=CARTESIAN_POINT('Ctrl Pts',(40.0365566379387,35.6064481050416,48.0601381135477));
#32190=CARTESIAN_POINT('Ctrl Pts',(40.0387982312214,35.6096230598115,48.1191684352402));
#32191=CARTESIAN_POINT('Ctrl Pts',(40.0432446627774,35.6127980145814,48.1780301136687));
#32192=CARTESIAN_POINT('Ctrl Pts',(40.0491763573697,35.6170335148476,48.256553643206));
#32193=CARTESIAN_POINT('Ctrl Pts',(40.0590480508809,35.6212690151138,48.334929648911));
#32194=CARTESIAN_POINT('Ctrl Pts',(40.0728464792292,35.6255045153801,48.4127310645737));
#32195=CARTESIAN_POINT('Ctrl Pts',(40.0866249042362,35.6297338755153,48.4904196928788));
#32196=CARTESIAN_POINT('Ctrl Pts',(40.1043186784733,35.6339632356505,48.5675349270486));
#32197=CARTESIAN_POINT('Ctrl Pts',(40.1258626696229,35.6381925957857,48.6436535119807));
#32198=CARTESIAN_POINT('Ctrl Pts',(40.1473815018575,35.6424170169052,48.7196832061872));
#32199=CARTESIAN_POINT('Ctrl Pts',(40.1727414889524,35.6466414380247,48.7947181147361));
#32200=CARTESIAN_POINT('Ctrl Pts',(40.2018265080558,35.6508658591441,48.8683454037502));
#32201=CARTESIAN_POINT('Ctrl Pts',(40.2308929278394,35.6550875788261,48.9419256095046));
#32202=CARTESIAN_POINT('Ctrl Pts',(40.2636794797217,35.6593092985082,49.0140995469749));
#32203=CARTESIAN_POINT('Ctrl Pts',(40.3000206651146,35.6635310181902,49.08447094657));
#32204=CARTESIAN_POINT('Ctrl Pts',(40.3363499598335,35.6677513565443,49.1548193209564));
#32205=CARTESIAN_POINT('Ctrl Pts',(40.3762313634132,35.6719716948984,49.2233659118693));
#32206=CARTESIAN_POINT('Ctrl Pts',(40.4194524776835,35.6761920332525,49.2897371642106));
#32207=CARTESIAN_POINT('Ctrl Pts',(40.4626729472441,35.6804123086538,49.3561074265221));
#32208=CARTESIAN_POINT('Ctrl Pts',(40.5092327712286,35.6846325840551,49.420302022182));
#32209=CARTESIAN_POINT('Ctrl Pts',(40.558875910112,35.6888528594563,49.481975885949));
#32210=CARTESIAN_POINT('Ctrl Pts',(40.6085687036992,35.6930773561162,49.5437114379473));
#32211=CARTESIAN_POINT('Ctrl Pts',(40.6613506779281,35.697301852776,49.6029208549052));
#32212=CARTESIAN_POINT('Ctrl Pts',(40.7169254990333,35.7015263494358,49.6592922181146));
#32213=CARTESIAN_POINT('Ctrl Pts',(40.7725270014648,35.7057528742654,49.7156906450682));
#32214=CARTESIAN_POINT('Ctrl Pts',(40.8309236755072,35.7099793990951,49.7692479862471));
#32215=CARTESIAN_POINT('Ctrl Pts',(40.8917842060067,35.7142059239247,49.8196910615951));
#32216=CARTESIAN_POINT('Ctrl Pts',(40.9527559875157,35.7184401747,49.8702263451938));
#32217=CARTESIAN_POINT('Ctrl Pts',(41.0162002482608,35.7226744254753,49.9176357057742));
#32218=CARTESIAN_POINT('Ctrl Pts',(41.0817548165928,35.7269086762506,49.9616880683034));
#32219=CARTESIAN_POINT('Ctrl Pts',(41.1442766124703,35.7309470364962,50.003702421964));
#32220=CARTESIAN_POINT('Ctrl Pts',(41.2087174496573,35.7349853967418,50.0426633669731));
#32221=CARTESIAN_POINT('Ctrl Pts',(41.2747437426207,35.7390237569874,50.0784101607067));
#32222=CARTESIAN_POINT('Ctrl Pts',(41.3439932311313,35.7432592572536,50.1159020002579));
#32223=CARTESIAN_POINT('Ctrl Pts',(41.4152501538411,35.7474947575199,50.1500003809986));
#32224=CARTESIAN_POINT('Ctrl Pts',(41.4881481603261,35.7517302577862,50.1804854192091));
#32225=CARTESIAN_POINT('Ctrl Pts',(41.5609404878403,35.7559596179215,50.2109262637904));
#32226=CARTESIAN_POINT('Ctrl Pts',(41.6353687454045,35.7601889780567,50.2377639884319));
#32227=CARTESIAN_POINT('Ctrl Pts',(41.7110417275687,35.764418338192,50.2608243938326));
#32228=CARTESIAN_POINT('Ctrl Pts',(41.7866263393789,35.7686427593115,50.2838578694609));
#32229=CARTESIAN_POINT('Ctrl Pts',(41.8634523406194,35.7728671804311,50.3031226554696));
#32230=CARTESIAN_POINT('Ctrl Pts',(41.9411097049378,35.7770916015506,50.318493074822));
#32231=CARTESIAN_POINT('Ctrl Pts',(42.0187174088397,35.7813133212326,50.3338536650819));
#32232=CARTESIAN_POINT('Ctrl Pts',(42.09715496145,35.7855350409147,50.3453247406623));
#32233=CARTESIAN_POINT('Ctrl Pts',(42.1759995555927,35.7897567605967,50.3528311120447));
#32234=CARTESIAN_POINT('Ctrl Pts',(42.2548183521354,35.7939770989509,50.3603350273758));
#32235=CARTESIAN_POINT('Ctrl Pts',(42.3340434588698,35.7981974373051,50.363876769935));
#32236=CARTESIAN_POINT('Ctrl Pts',(42.4132457998714,35.8024177756593,50.3634328824161));
#32237=CARTESIAN_POINT('Ctrl Pts',(42.4924469594477,35.8066380510606,50.3629890015185));
#32238=CARTESIAN_POINT('Ctrl Pts',(42.5716248846297,35.8108583264619,50.3585596126844));
#32239=CARTESIAN_POINT('Ctrl Pts',(42.6503508506604,35.8150786018632,50.3501733749819));
#32240=CARTESIAN_POINT('Ctrl Pts',(42.7291555609973,35.819303098523,50.3417787490879));
#32241=CARTESIAN_POINT('Ctrl Pts',(42.8075069413014,35.8235275951829,50.3294194180143));
#32242=CARTESIAN_POINT('Ctrl Pts',(42.8849823451398,35.8277520918428,50.3131758614085));
#32243=CARTESIAN_POINT('Ctrl Pts',(42.9624949447169,35.8319786166724,50.2969245063135));
#32244=CARTESIAN_POINT('Ctrl Pts',(43.0391302754707,35.8362051415021,50.2767853302189));
#32245=CARTESIAN_POINT('Ctrl Pts',(43.1144793466283,35.8404316663318,50.2528891903824));
#32246=CARTESIAN_POINT('Ctrl Pts',(43.1899661533618,35.8446659171071,50.2289493692033));
#32247=CARTESIAN_POINT('Ctrl Pts',(43.2641615613275,35.8489001678825,50.2012390258438));
#32248=CARTESIAN_POINT('Ctrl Pts',(43.3366752981571,35.8531344186579,50.1699377471998));
#32249=CARTESIAN_POINT('Ctrl Pts',(43.4058343082324,35.8571727789029,50.1400845698604));
#32250=CARTESIAN_POINT('Ctrl Pts',(43.4734635009498,35.861211139148,50.1069655568262));
#32251=CARTESIAN_POINT('Ctrl Pts',(43.5392472203167,35.8652494993931,50.0707743025015));
#32252=CARTESIAN_POINT('Ctrl Pts',(43.6082422935601,35.8694849996593,50.0328163051895));
#32253=CARTESIAN_POINT('Ctrl Pts',(43.6754693775186,35.8737204999256,49.9913341670389));
#32254=CARTESIAN_POINT('Ctrl Pts',(43.7405453513509,35.8779560001918,49.9465170438173));
#32255=CARTESIAN_POINT('Ctrl Pts',(43.805526985677,35.8821853603271,49.9017648911991));
#32256=CARTESIAN_POINT('Ctrl Pts',(43.8683633192411,35.8864147204623,49.8536876182718));
#32257=CARTESIAN_POINT('Ctrl Pts',(43.9286962067227,35.8906440805976,49.8025199994596));
#32258=CARTESIAN_POINT('Ctrl Pts',(43.9889586379004,35.8948685017171,49.7514121338177));
#32259=CARTESIAN_POINT('Ctrl Pts',(44.0467230764509,35.8990929228366,49.6972213958138));
#32260=CARTESIAN_POINT('Ctrl Pts',(44.1016620036921,35.9033173439561,49.6402246389109));
#32261=CARTESIAN_POINT('Ctrl Pts',(44.1565657985279,35.9075390636381,49.5832643303568));
#32262=CARTESIAN_POINT('Ctrl Pts',(44.208647343442,35.9117607833201,49.5235019014091));
#32263=CARTESIAN_POINT('Ctrl Pts',(44.2576146668553,35.9159825030021,49.4612522678799));
#32264=CARTESIAN_POINT('Ctrl Pts',(44.3065659683785,35.9202028413563,49.3990230021536));
#32265=CARTESIAN_POINT('Ctrl Pts',(44.352404781752,35.9244231797104,49.3343085164039));
#32266=CARTESIAN_POINT('Ctrl Pts',(44.3948792522998,35.9286435180646,49.267456985323));
#32267=CARTESIAN_POINT('Ctrl Pts',(44.4373530892751,35.9328637934659,49.2006064514359));
#32268=CARTESIAN_POINT('Ctrl Pts',(44.4764624326073,35.9370840688672,49.1316193324528));
#32269=CARTESIAN_POINT('Ctrl Pts',(44.5119994489321,35.9413043442684,49.0608717022386));
#32270=CARTESIAN_POINT('Ctrl Pts',(44.5475720105519,35.9455288409283,48.9900533079128));
#32271=CARTESIAN_POINT('Ctrl Pts',(44.579564896151,35.9497533375881,48.9174713051084));
#32272=CARTESIAN_POINT('Ctrl Pts',(44.6078171432482,35.953977834248,48.843524690142));
#32273=CARTESIAN_POINT('Ctrl Pts',(44.6360829541754,35.9582043590776,48.7695425735992));
#32274=CARTESIAN_POINT('Ctrl Pts',(44.6606044035574,35.9624308839072,48.6941949866861));
#32275=CARTESIAN_POINT('Ctrl Pts',(44.6812702854933,35.9666574087369,48.6178966947843));
#32276=CARTESIAN_POINT('Ctrl Pts',(44.7019739439685,35.9708916595122,48.5414589321629));
#32277=CARTESIAN_POINT('Ctrl Pts',(44.7188078517222,35.9751259102875,48.4640674517408));
#32278=CARTESIAN_POINT('Ctrl Pts',(44.7317119123445,35.9793601610629,48.3861476385152));
#32279=CARTESIAN_POINT('Ctrl Pts',(44.7440189881853,35.9833985213083,48.3118326551205));
#32280=CARTESIAN_POINT('Ctrl Pts',(44.7527517863751,35.9874368815536,48.2370375017441));
#32281=CARTESIAN_POINT('Ctrl Pts',(44.7579023580358,35.991475241799,48.1621323868604));
#32282=CARTESIAN_POINT('Ctrl Pts',(44.7633043643738,35.9957107420653,48.0835706403209));
#32283=CARTESIAN_POINT('Ctrl Pts',(44.7647860022,35.9999462423315,48.0045892921905));
#32284=CARTESIAN_POINT('Ctrl Pts',(44.7622990917098,36.0041817425978,47.9256128895103));
#32285=CARTESIAN_POINT('Ctrl Pts',(44.7598157864504,36.008411102733,47.846750977546));
#32286=CARTESIAN_POINT('Ctrl Pts',(44.7533753722327,36.0126404628683,47.7678944619458));
#32287=CARTESIAN_POINT('Ctrl Pts',(44.7429815473663,36.0168698230036,47.6894715639411));
#32288=CARTESIAN_POINT('Ctrl Pts',(44.7325998603324,36.021094244123,47.6111402476221));
#32289=CARTESIAN_POINT('Ctrl Pts',(44.7182739983652,36.0253186652425,47.5332420055022));
#32290=CARTESIAN_POINT('Ctrl Pts',(44.700059618178,36.029543086362,47.4562020653524));
#32291=CARTESIAN_POINT('Ctrl Pts',(44.6818568857426,36.033764806044,47.3792113907882));
#32292=CARTESIAN_POINT('Ctrl Pts',(44.6597706782225,36.0379865257261,47.3030783843339));
#32293=CARTESIAN_POINT('Ctrl Pts',(44.6339078945148,36.0422082454081,47.2282189690564));
#32294=CARTESIAN_POINT('Ctrl Pts',(44.6080535729948,36.0464285837622,47.1533840474462));
#32295=CARTESIAN_POINT('Ctrl Pts',(44.5784252820845,36.0506489221164,47.0798223328449));
#32296=CARTESIAN_POINT('Ctrl Pts',(44.5451795952357,36.0548692604706,47.0079340016489));
#32297=CARTESIAN_POINT('Ctrl Pts',(44.5119344042977,36.0590895358718,46.9360467427785));
#32298=CARTESIAN_POINT('Ctrl Pts',(44.4750721229008,36.0633098112731,46.8658332431383));
#32299=CARTESIAN_POINT('Ctrl Pts',(44.4347966036396,36.0675300866744,46.7976717491813));
#32300=CARTESIAN_POINT('Ctrl Pts',(44.3944807994765,36.0717545833342,46.7294420778514));
#32301=CARTESIAN_POINT('Ctrl Pts',(44.3507451768233,36.0759790799941,46.6632689173466));
#32302=CARTESIAN_POINT('Ctrl Pts',(44.3038382234481,36.0802035766539,46.5995034952425));
#32303=CARTESIAN_POINT('Ctrl Pts',(44.2569087501673,36.0844301014836,46.5357074595261));
#32304=CARTESIAN_POINT('Ctrl Pts',(44.2068052102526,36.0886566263132,46.474321829111));
#32305=CARTESIAN_POINT('Ctrl Pts',(44.153816271585,36.0928831511428,46.4156645158226));
#32306=CARTESIAN_POINT('Ctrl Pts',(44.100730470914,36.0971174019182,46.3568999789321));
#32307=CARTESIAN_POINT('Ctrl Pts',(44.0447490645993,36.1013516526935,46.3008740577952));
#32308=CARTESIAN_POINT('Ctrl Pts',(43.9861973017163,36.1055859034688,46.2478674248426));
#32309=CARTESIAN_POINT('Ctrl Pts',(43.9303543382109,36.1096242637142,46.1973130551059));
#32310=CARTESIAN_POINT('Ctrl Pts',(43.8721738844849,36.1136626239595,46.1495049853175));
#32311=CARTESIAN_POINT('Ctrl Pts',(43.8119629959803,36.1177009842048,46.1046501803408));
#32312=CARTESIAN_POINT('Ctrl Pts',(43.748812801644,36.1219364844711,46.0576057051378));
#32313=CARTESIAN_POINT('Ctrl Pts',(43.6831888245936,36.1261719847373,46.0136313689946));
#32314=CARTESIAN_POINT('Ctrl Pts',(43.6154220559417,36.1304074850036,45.9729973688151));
#32315=CARTESIAN_POINT('Ctrl Pts',(43.5477535275945,36.1346368451388,45.9324222750382));
#32316=CARTESIAN_POINT('Ctrl Pts',(43.4779487754724,36.1388662052741,45.8951781403443));
#32317=CARTESIAN_POINT('Ctrl Pts',(43.406369946404,36.1430955654094,45.8614935183931));
#32318=CARTESIAN_POINT('Ctrl Pts',(43.3348747065675,36.1473199865289,45.8278482330965));
#32319=CARTESIAN_POINT('Ctrl Pts',(43.2616099292165,36.1515444076484,45.7977543990737));
#32320=CARTESIAN_POINT('Ctrl Pts',(43.1869633526491,36.1557688287679,45.771395252072));
#32321=CARTESIAN_POINT('Ctrl Pts',(43.1123645111564,36.1599905484499,45.7450529612466));
#32322=CARTESIAN_POINT('Ctrl Pts',(43.0363860656463,36.1642122681319,45.7224407731108));
#32323=CARTESIAN_POINT('Ctrl Pts',(42.9594356504853,36.168433987814,45.7036937935314));
#32324=CARTESIAN_POINT('Ctrl Pts',(42.8825104131574,36.1726543261681,45.6849529478802));
#32325=CARTESIAN_POINT('Ctrl Pts',(42.8046142933375,36.1768746645223,45.670074910564));
#32326=CARTESIAN_POINT('Ctrl Pts',(42.7261685555116,36.1810950028765,45.6591444909402));
#32327=CARTESIAN_POINT('Ctrl Pts',(42.6477239878251,36.1853152782777,45.6482142343605));
#32328=CARTESIAN_POINT('Ctrl Pts',(42.5687302834738,36.189535553679,45.6412315418742));
#32329=CARTESIAN_POINT('Ctrl Pts',(42.4896158408591,36.1937558290803,45.6382295958398));
#32330=CARTESIAN_POINT('Ctrl Pts',(42.4104222653713,36.1979803257402,45.63522464716));
#32331=CARTESIAN_POINT('Ctrl Pts',(42.3311081805084,36.2022048224,45.6362084166665));
#32332=CARTESIAN_POINT('Ctrl Pts',(42.2521034082872,36.2064293190599,45.6411619303013));
#32333=CARTESIAN_POINT('Ctrl Pts',(42.1730607060814,36.2106558438895,45.6461178221051));
#32334=CARTESIAN_POINT('Ctrl Pts',(42.0943280793503,36.2148823687192,45.6550472017864));
#32335=CARTESIAN_POINT('Ctrl Pts',(42.0163290677288,36.2191088935488,45.6678792791474));
#32336=CARTESIAN_POINT('Ctrl Pts',(41.9381874765289,36.2233431443242,45.6807348131156));
#32337=CARTESIAN_POINT('Ctrl Pts',(41.8607826400316,36.2275773950995,45.6975072005145));
#32338=CARTESIAN_POINT('Ctrl Pts',(41.7845265686104,36.2318116458749,45.7180747391394));
#32339=CARTESIAN_POINT('Ctrl Pts',(41.7117983567903,36.2358500061202,45.7376907549904));
#32340=CARTESIAN_POINT('Ctrl Pts',(41.64011529799,36.2398883663654,45.7607583906208));
#32341=CARTESIAN_POINT('Ctrl Pts',(41.5698175698493,36.2439267266107,45.7871313700156));
#32342=CARTESIAN_POINT('Ctrl Pts',(41.4960881281522,36.248162226877,45.8147917951544));
#32343=CARTESIAN_POINT('Ctrl Pts',(41.4236024641777,36.2523977271432,45.8461936600882));
#32344=CARTESIAN_POINT('Ctrl Pts',(41.3527668844805,36.2566332274095,45.881204766227));
#32345=CARTESIAN_POINT('Ctrl Pts',(41.2820339938899,36.2608625875447,45.9161651173747));
#32346=CARTESIAN_POINT('Ctrl Pts',(41.212946854495,36.26509194768,45.9547241131883));
#32347=CARTESIAN_POINT('Ctrl Pts',(41.1458936046904,36.2693213078153,45.9967008236053));
#32348=CARTESIAN_POINT('Ctrl Pts',(41.0789186591795,36.2735457289347,46.0386285139276));
#32349=CARTESIAN_POINT('Ctrl Pts',(41.0139732791313,36.2777701500542,46.0839657398779));
#32350=CARTESIAN_POINT('Ctrl Pts',(40.9514213340713,36.2819945711737,46.1324855316447));
#32351=CARTESIAN_POINT('Ctrl Pts',(40.8889093897979,36.2862162908557,46.1809742959219));
#32352=CARTESIAN_POINT('Ctrl Pts',(40.8287882125454,36.2904380105378,46.2326412997073));
#32353=CARTESIAN_POINT('Ctrl Pts',(40.7713919568624,36.2946597302198,46.2872168021821));
#32354=CARTESIAN_POINT('Ctrl Pts',(40.7140144809787,36.298880068574,46.3417744477954));
#32355=CARTESIAN_POINT('Ctrl Pts',(40.6593604961549,36.3031004069281,46.3992383792675));
#32356=CARTESIAN_POINT('Ctrl Pts',(40.6077292299424,36.3073207452822,46.4593001824829));
#32357=CARTESIAN_POINT('Ctrl Pts',(40.5560987338901,36.3115410206835,46.5193610897837));
#32358=CARTESIAN_POINT('Ctrl Pts',(40.5074911717723,36.3157612960848,46.5820194350096));
#32359=CARTESIAN_POINT('Ctrl Pts',(40.4621662107731,36.3199815714861,46.646932874455));
#32360=CARTESIAN_POINT('Ctrl Pts',(40.416795914254,36.3242060681459,46.7119112424621));
#32361=CARTESIAN_POINT('Ctrl Pts',(40.3747150471325,36.3284305648058,46.7791488248277));
#32362=CARTESIAN_POINT('Ctrl Pts',(40.3361401817462,36.3326550614656,46.8482738643682));
#32363=CARTESIAN_POINT('Ctrl Pts',(40.2975467966679,36.3368815862953,46.9174320906594));
#32364=CARTESIAN_POINT('Ctrl Pts',(40.2624629746092,36.3411081111249,46.9884791578979));
#32365=CARTESIAN_POINT('Ctrl Pts',(40.2310583103646,36.3453346359546,47.0610205604692));
#32366=CARTESIAN_POINT('Ctrl Pts',(40.1995962394466,36.3495688867299,47.1336945662924));
#32367=CARTESIAN_POINT('Ctrl Pts',(40.1718269302199,36.3538031375052,47.2078679251033));
#32368=CARTESIAN_POINT('Ctrl Pts',(40.1478709218199,36.3580373882806,47.283128284757));
#32369=CARTESIAN_POINT('Ctrl Pts',(40.1250231980802,36.3620757485259,47.3549068497501));
#32370=CARTESIAN_POINT('Ctrl Pts',(40.1056438023386,36.3661141087712,47.4276737086444));
#32371=CARTESIAN_POINT('Ctrl Pts',(40.0897937455689,36.3701524690165,47.5010636284182));
#32372=CARTESIAN_POINT('Ctrl Pts',(40.0666639190707,36.376045607014,47.6081607912697));
#32373=CARTESIAN_POINT('Ctrl Pts',(40.0509743135021,36.3819387450114,47.7169176509785));
#32374=CARTESIAN_POINT('Ctrl Pts',(40.0429090143393,36.3878318830088,47.8264703880687));
#32375=CARTESIAN_POINT('Ctrl Pts',(40.0387159839485,36.3908956387631,47.8834252445147));
#32376=CARTESIAN_POINT('Ctrl Pts',(40.0365829442789,36.3939593945174,47.9405948654727));
#32377=CARTESIAN_POINT('Ctrl Pts',(40.0365309734998,36.3970231502717,47.9978548487108));
#32378=CARTESIAN_POINT('',(40.0365300000534,37.1907731503223,48.0000158946174));
#32379=CARTESIAN_POINT('Ctrl Pts',(40.0365309734993,36.3970231502996,47.9978548492323));
#32380=CARTESIAN_POINT('Ctrl Pts',(40.0364602792016,36.4011906867027,48.0757439121105));
#32381=CARTESIAN_POINT('Ctrl Pts',(40.0402441056578,36.4053582231059,48.1537521997897));
#32382=CARTESIAN_POINT('Ctrl Pts',(40.047891134619,36.4095257595091,48.2314612846587));
#32383=CARTESIAN_POINT('Ctrl Pts',(40.0555321839855,36.4136900371069,48.3091096049048));
#32384=CARTESIAN_POINT('Ctrl Pts',(40.0670303989496,36.4178543147047,48.3864587069638));
#32385=CARTESIAN_POINT('Ctrl Pts',(40.082342420306,36.4220185923026,48.4630915505459));
#32386=CARTESIAN_POINT('Ctrl Pts',(40.0976475630965,36.4261809991965,48.5396899686227));
#32387=CARTESIAN_POINT('Ctrl Pts',(40.1167630190008,36.4303434060904,48.6155722928962));
#32388=CARTESIAN_POINT('Ctrl Pts',(40.1395939776329,36.4345058129844,48.6903296712053));
#32389=CARTESIAN_POINT('Ctrl Pts',(40.1624222753605,36.4386677347578,48.7650783366855));
#32390=CARTESIAN_POINT('Ctrl Pts',(40.188965073726,36.4428296565312,48.8387018543109));
#32391=CARTESIAN_POINT('Ctrl Pts',(40.2190776109635,36.4469915783046,48.9108062219261));
#32392=CARTESIAN_POINT('Ctrl Pts',(40.2492173909904,36.4511572653654,48.9829758223076));
#32393=CARTESIAN_POINT('Ctrl Pts',(40.2829331750889,36.4553229524263,49.0536230795644));
#32394=CARTESIAN_POINT('Ctrl Pts',(40.3200322191805,36.4594886394871,49.1223744792416));
#32395=CARTESIAN_POINT('Ctrl Pts',(40.3571470655116,36.4636561009113,49.1911551633952));
#32396=CARTESIAN_POINT('Ctrl Pts',(40.3976477897498,36.4678235623355,49.2580379681821));
#32397=CARTESIAN_POINT('Ctrl Pts',(40.44129726956,36.4719910237597,49.3226768519434));
#32398=CARTESIAN_POINT('Ctrl Pts',(40.4850252896868,36.4761659838699,49.387432043125));
#32399=CARTESIAN_POINT('Ctrl Pts',(40.5319130921366,36.48034094398,49.4499348602826));
#32400=CARTESIAN_POINT('Ctrl Pts',(40.581682336817,36.4845159040901,49.5098712914208));
#32401=CARTESIAN_POINT('Ctrl Pts',(40.6288187613196,36.4884700065342,49.5666370526743));
#32402=CARTESIAN_POINT('Ctrl Pts',(40.6785392535147,36.4924241089783,49.6211008174602));
#32403=CARTESIAN_POINT('Ctrl Pts',(40.7305785860932,36.4963782114224,49.6730279685915));
#32404=CARTESIAN_POINT('Ctrl Pts',(40.78632135202,36.5006137116887,49.7286505695615));
#32405=CARTESIAN_POINT('Ctrl Pts',(40.84495300563,36.5048492119549,49.7815899480815));
#32406=CARTESIAN_POINT('Ctrl Pts',(40.9061847714878,36.5090847122211,49.831531191098));
#32407=CARTESIAN_POINT('Ctrl Pts',(40.9673277707206,36.5133140723564,49.8814000351641));
#32408=CARTESIAN_POINT('Ctrl Pts',(41.0310630363231,36.5175434324917,49.9282790806586));
#32409=CARTESIAN_POINT('Ctrl Pts',(41.0970649818335,36.5217727926269,49.971890153973));
#32410=CARTESIAN_POINT('Ctrl Pts',(41.1629898507557,36.5259972137464,50.0154502985955));
#32411=CARTESIAN_POINT('Ctrl Pts',(41.2311757499249,36.5302216348659,50.0557497973636));
#32412=CARTESIAN_POINT('Ctrl Pts',(41.3012652609604,36.5344460559854,50.0925516514838));
#32413=CARTESIAN_POINT('Ctrl Pts',(41.3713099510784,36.5386677756674,50.129329971514));
#32414=CARTESIAN_POINT('Ctrl Pts',(41.4432554225069,36.5428894953494,50.1626148686195));
#32415=CARTESIAN_POINT('Ctrl Pts',(41.5167176576929,36.5471112150315,50.1922141192567));
#32416=CARTESIAN_POINT('Ctrl Pts',(41.5901558563627,36.5513315533856,50.2218036851509));
#32417=CARTESIAN_POINT('Ctrl Pts',(41.6651093983326,36.5555518917398,50.2477098238734));
#32418=CARTESIAN_POINT('Ctrl Pts',(41.7411735569024,36.5597722300939,50.2697881308121));
#32419=CARTESIAN_POINT('Ctrl Pts',(41.8172365808575,36.5639925054952,50.2918661084186));
#32420=CARTESIAN_POINT('Ctrl Pts',(41.8944097373622,36.5682127808965,50.3101162381872));
#32421=CARTESIAN_POINT('Ctrl Pts',(41.9722738284938,36.5724330562978,50.324444183694));
#32422=CARTESIAN_POINT('Ctrl Pts',(42.0502158018559,36.5766575529576,50.3387864604841));
#32423=CARTESIAN_POINT('Ctrl Pts',(42.1288496276913,36.5808820496175,50.3491986309863));
#32424=CARTESIAN_POINT('Ctrl Pts',(42.2077472120124,36.5851065462773,50.3556377706284));
#32425=CARTESIAN_POINT('Ctrl Pts',(42.2866826748575,36.5893330711069,50.3620800016846));
#32426=CARTESIAN_POINT('Ctrl Pts',(42.3658816786816,36.5935595959366,50.3645453873998));
#32427=CARTESIAN_POINT('Ctrl Pts',(42.4449149084639,36.5977861207662,50.3630431845182));
#32428=CARTESIAN_POINT('Ctrl Pts',(42.5240926083407,36.6020203715416,50.36153823566));
#32429=CARTESIAN_POINT('Ctrl Pts',(42.6031034591966,36.6062546223169,50.3560512383724));
#32430=CARTESIAN_POINT('Ctrl Pts',(42.6815222473042,36.6104888730922,50.3466434891506));
#32431=CARTESIAN_POINT('Ctrl Pts',(42.7563131213414,36.6145272333376,50.3376709737113));
#32432=CARTESIAN_POINT('Ctrl Pts',(42.8305651566769,36.6185655935829,50.3251325535074));
#32433=CARTESIAN_POINT('Ctrl Pts',(42.903920700685,36.6226039538282,50.3091241561079));
#32434=CARTESIAN_POINT('Ctrl Pts',(42.9808572311832,36.6268394540945,50.2923342791954));
#32435=CARTESIAN_POINT('Ctrl Pts',(43.0570999599424,36.6310749543607,50.2716631661511));
#32436=CARTESIAN_POINT('Ctrl Pts',(43.1322278111933,36.635310454627,50.2471833199397));
#32437=CARTESIAN_POINT('Ctrl Pts',(43.2072467509061,36.6395398147623,50.2227389617351));
#32438=CARTESIAN_POINT('Ctrl Pts',(43.2811535801512,36.6437691748975,50.1944969791762));
#32439=CARTESIAN_POINT('Ctrl Pts',(43.3535382076112,36.6479985350328,50.1625807100605));
#32440=CARTESIAN_POINT('Ctrl Pts',(43.4258383048338,36.6522229561523,50.1307017125299));
#32441=CARTESIAN_POINT('Ctrl Pts',(43.4966193054986,36.6564473772718,50.0951571434457));
#32442=CARTESIAN_POINT('Ctrl Pts',(43.5654885266666,36.6606717983913,50.0561193873675));
#32443=CARTESIAN_POINT('Ctrl Pts',(43.6343137072693,36.6648935180733,50.0171065951965));
#32444=CARTESIAN_POINT('Ctrl Pts',(43.7012291276562,36.6691152377553,49.9746052805247));
#32445=CARTESIAN_POINT('Ctrl Pts',(43.7658653722042,36.6733369574374,49.9288344215908));
#32446=CARTESIAN_POINT('Ctrl Pts',(43.8304804680608,36.6775572957915,49.8830785386781));
#32447=CARTESIAN_POINT('Ctrl Pts',(43.8928174861141,36.6817776341457,49.8340555067686));
#32448=CARTESIAN_POINT('Ctrl Pts',(43.9525360243316,36.6859979724999,49.7820275907102));
#32449=CARTESIAN_POINT('Ctrl Pts',(44.0122536717547,36.6902182479011,49.7300004507288));
#32450=CARTESIAN_POINT('Ctrl Pts',(44.0693525639732,36.6944385233024,49.6749688250133));
#32451=CARTESIAN_POINT('Ctrl Pts',(44.1235265788985,36.6986587987037,49.6172342355796));
#32452=CARTESIAN_POINT('Ctrl Pts',(44.1777547804591,36.7028832953636,49.5594418981064));
#32453=CARTESIAN_POINT('Ctrl Pts',(44.2290519386273,36.7071077920234,49.4989415392319));
#32454=CARTESIAN_POINT('Ctrl Pts',(44.2771503574292,36.7113322886833,49.4360699761862));
#32455=CARTESIAN_POINT('Ctrl Pts',(44.3252718681562,36.7155588135129,49.3731682286675));
#32456=CARTESIAN_POINT('Ctrl Pts',(44.3701913137622,36.7197853383426,49.3078933963054));
#32457=CARTESIAN_POINT('Ctrl Pts',(44.4116842236564,36.7240118631722,49.2406115529013));
#32458=CARTESIAN_POINT('Ctrl Pts',(44.4532529811988,36.7282461139475,49.173206720543));
#32459=CARTESIAN_POINT('Ctrl Pts',(44.4913824603497,36.7324803647229,49.1037879585842));
#32460=CARTESIAN_POINT('Ctrl Pts',(44.5258941761743,36.7367146154982,49.032746044586));
#32461=CARTESIAN_POINT('Ctrl Pts',(44.5588092651896,36.7407529757435,48.9649907659165));
#32462=CARTESIAN_POINT('Ctrl Pts',(44.5884338210638,36.7447913359888,48.8957595415893));
#32463=CARTESIAN_POINT('Ctrl Pts',(44.6146550345483,36.7488296962341,48.8254050634992));
#32464=CARTESIAN_POINT('Ctrl Pts',(44.6421562850433,36.7530651965004,48.7516161014992));
#32465=CARTESIAN_POINT('Ctrl Pts',(44.6660179661831,36.7573006967666,48.6763109305192));
#32466=CARTESIAN_POINT('Ctrl Pts',(44.6860732565879,36.7615361970329,48.5998829105863));
#32467=CARTESIAN_POINT('Ctrl Pts',(44.7060994731875,36.7657655571681,48.5235656870231));
#32468=CARTESIAN_POINT('Ctrl Pts',(44.7223301388211,36.7699949173034,48.4461292971214));
#32469=CARTESIAN_POINT('Ctrl Pts',(44.7346471281255,36.7742242774386,48.3679853638874));
#32470=CARTESIAN_POINT('Ctrl Pts',(44.7469497337401,36.7784486985581,48.289932686566));
#32471=CARTESIAN_POINT('Ctrl Pts',(44.7553476724894,36.7826731196776,48.2111745690717));
#32472=CARTESIAN_POINT('Ctrl Pts',(44.7597734864983,36.7868975407971,48.1321345273571));
#32473=CARTESIAN_POINT('Ctrl Pts',(44.7641964702827,36.7911192604791,48.0531450302552));
#32474=CARTESIAN_POINT('Ctrl Pts',(44.7646523447103,36.7953409801612,47.9738744341119));
#32475=CARTESIAN_POINT('Ctrl Pts',(44.7611254259176,36.7995626998432,47.8947518931982));
#32476=CARTESIAN_POINT('Ctrl Pts',(44.7575996611171,36.8037830381974,47.8156552408277));
#32477=CARTESIAN_POINT('Ctrl Pts',(44.7500937116094,36.8080033765515,47.736707016026));
#32478=CARTESIAN_POINT('Ctrl Pts',(44.7386439948903,36.8122237149057,47.6583353895069));
#32479=CARTESIAN_POINT('Ctrl Pts',(44.7271944489615,36.8164439903069,47.5799649320218));
#32480=CARTESIAN_POINT('Ctrl Pts',(44.7118013219268,36.8206642657082,47.5021715199513));
#32481=CARTESIAN_POINT('Ctrl Pts',(44.6925525928199,36.8248845411095,47.4253757314081));
#32482=CARTESIAN_POINT('Ctrl Pts',(44.6732846104996,36.8291090377693,47.3485031291859));
#32483=CARTESIAN_POINT('Ctrl Pts',(44.6501534366463,36.8333335344292,47.27263060019));
#32484=CARTESIAN_POINT('Ctrl Pts',(44.6232975227603,36.837558031089,47.1981654995026));
#32485=CARTESIAN_POINT('Ctrl Pts',(44.5964287154202,36.8417845559187,47.1236646483149));
#32486=CARTESIAN_POINT('Ctrl Pts',(44.5658317871443,36.8460110807483,47.0505730050612));
#32487=CARTESIAN_POINT('Ctrl Pts',(44.5316931795947,36.850237605578,46.9792773986193));
#32488=CARTESIAN_POINT('Ctrl Pts',(44.4974921678151,36.8544718563533,46.9078514661991));
#32489=CARTESIAN_POINT('Ctrl Pts',(44.4597367643785,36.8587061071286,46.8382285446606));
#32490=CARTESIAN_POINT('Ctrl Pts',(44.4186590653512,36.862940357904,46.7707701521784));
#32491=CARTESIAN_POINT('Ctrl Pts',(44.3794817573638,36.8669787181493,46.7064326093951));
#32492=CARTESIAN_POINT('Ctrl Pts',(44.3372829872294,36.8710170783946,46.6440640232978));
#32493=CARTESIAN_POINT('Ctrl Pts',(44.2922983498868,36.8750554386399,46.5839500729439));
#32494=CARTESIAN_POINT('Ctrl Pts',(44.245117704311,36.8792909389062,46.5209015489732));
#32495=CARTESIAN_POINT('Ctrl Pts',(44.1946929083828,36.8835264391724,46.4600937488261));
#32496=CARTESIAN_POINT('Ctrl Pts',(44.1412645399784,36.8877619394387,46.4018797783916));
#32497=CARTESIAN_POINT('Ctrl Pts',(44.0879136257495,36.8919912995739,46.3437501997365));
#32498=CARTESIAN_POINT('Ctrl Pts',(44.0315681004492,36.8962206597092,46.2882073265073));
#32499=CARTESIAN_POINT('Ctrl Pts',(43.9725102457625,36.9004500198445,46.2355731899929));
#32500=CARTESIAN_POINT('Ctrl Pts',(43.9135213584058,36.904674440964,46.1830005192374));
#32501=CARTESIAN_POINT('Ctrl Pts',(43.8518267845221,36.9088988620835,46.1333301457761));
#32502=CARTESIAN_POINT('Ctrl Pts',(43.7877462187777,36.913123283203,46.0868479221012));
#32503=CARTESIAN_POINT('Ctrl Pts',(43.7237066313438,36.917345002885,46.0403954229298));
#32504=CARTESIAN_POINT('Ctrl Pts',(43.6572844593278,36.921566722567,45.9971273018812));
#32505=CARTESIAN_POINT('Ctrl Pts',(43.5888321486797,36.9257884422491,45.9572889183329));
#32506=CARTESIAN_POINT('Ctrl Pts',(43.5204022353227,36.9300087806032,45.9174635697262));
#32507=CARTESIAN_POINT('Ctrl Pts',(43.4499439076649,36.9342291189574,45.8810659662195));
#32508=CARTESIAN_POINT('Ctrl Pts',(43.3778369708489,36.9384494573115,45.8482971163888));
#32509=CARTESIAN_POINT('Ctrl Pts',(43.3057311096197,36.9426697327128,45.8155287553562));
#32510=CARTESIAN_POINT('Ctrl Pts',(43.2319771159644,36.9468900081141,45.7863892333742));
#32511=CARTESIAN_POINT('Ctrl Pts',(43.1569763037883,36.9511102835154,45.7610320867857));
#32512=CARTESIAN_POINT('Ctrl Pts',(43.0819004733276,36.9553347801752,45.7356495771434));
#32513=CARTESIAN_POINT('Ctrl Pts',(43.005575778778,36.9595592768351,45.7140571511106));
#32514=CARTESIAN_POINT('Ctrl Pts',(42.92841971828,36.9637837734949,45.6963587427221));
#32515=CARTESIAN_POINT('Ctrl Pts',(42.8512266153592,36.9680102983246,45.678651837374));
#32516=CARTESIAN_POINT('Ctrl Pts',(42.7732018141652,36.9722368231542,45.6648427558669));
#32517=CARTESIAN_POINT('Ctrl Pts',(42.6947715119937,36.9764633479838,45.654983966661));
#32518=CARTESIAN_POINT('Ctrl Pts',(42.6161978418591,36.9806975987592,45.6451071559189));
#32519=CARTESIAN_POINT('Ctrl Pts',(42.5372176588444,36.9849318495345,45.6391951018615));
#32520=CARTESIAN_POINT('Ctrl Pts',(42.4582605718773,36.9891661003099,45.6372481834385));
#32521=CARTESIAN_POINT('Ctrl Pts',(42.3829563024771,36.9932044605552,45.6353913359401));
#32522=CARTESIAN_POINT('Ctrl Pts',(42.3076733956048,36.9972428208005,45.6371408117188));
#32523=CARTESIAN_POINT('Ctrl Pts',(42.2327795702227,37.0012811810458,45.6424530187576));
#32524=CARTESIAN_POINT('Ctrl Pts',(42.1542296643014,37.0055166813121,45.6480245510035));
#32525=CARTESIAN_POINT('Ctrl Pts',(42.0758092122744,37.0097521815783,45.6575367172658));
#32526=CARTESIAN_POINT('Ctrl Pts',(41.9979453366885,37.0139876818446,45.6709782120793));
#32527=CARTESIAN_POINT('Ctrl Pts',(41.920194339007,37.0182170419798,45.6844002209918));
#32528=CARTESIAN_POINT('Ctrl Pts',(41.8429987740852,37.0224464021151,45.7017401674841));
#32529=CARTESIAN_POINT('Ctrl Pts',(41.7667821912645,37.0266757622504,45.7229348609229));
#32530=CARTESIAN_POINT('Ctrl Pts',(41.6906546136108,37.0309001833699,45.744104803354));
#32531=CARTESIAN_POINT('Ctrl Pts',(41.6155041960551,37.0351246044893,45.7691204222288));
#32532=CARTESIAN_POINT('Ctrl Pts',(41.5417443006599,37.0393490256088,45.7978674891256));
#32533=CARTESIAN_POINT('Ctrl Pts',(41.4680315733236,37.0435707452909,45.8265961728164));
#32534=CARTESIAN_POINT('Ctrl Pts',(41.3957080393815,37.0477924649729,45.8590513984745));
#32535=CARTESIAN_POINT('Ctrl Pts',(41.3251707232159,37.0520141846549,45.895069486499));
#32536=CARTESIAN_POINT('Ctrl Pts',(41.2546564865458,37.0562345230091,45.9310757895655));
#32537=CARTESIAN_POINT('Ctrl Pts',(41.185927724836,37.0604548613632,45.9706424269158));
#32538=CARTESIAN_POINT('Ctrl Pts',(41.1193589632904,37.0646751997174,46.013558715694));
#32539=CARTESIAN_POINT('Ctrl Pts',(41.0527911947207,37.0688954751187,46.0564743643095));
#32540=CARTESIAN_POINT('Ctrl Pts',(40.9883837560255,37.07311575052,46.1027393095946));
#32541=CARTESIAN_POINT('Ctrl Pts',(40.9264828829859,37.0773360259213,46.1520990971466));
#32542=CARTESIAN_POINT('Ctrl Pts',(40.8645200946529,37.0815605225811,46.2015082559849));
#32543=CARTESIAN_POINT('Ctrl Pts',(40.8050692481665,37.085785019241,46.2540181475494));
#32544=CARTESIAN_POINT('Ctrl Pts',(40.7484436179076,37.0900095159008,46.3093338716145));
#32545=CARTESIAN_POINT('Ctrl Pts',(40.6917908018319,37.0942360407304,46.364676152614));
#32546=CARTESIAN_POINT('Ctrl Pts',(40.6379662233171,37.0984625655601,46.4228266047286));
#32547=CARTESIAN_POINT('Ctrl Pts',(40.5872445789206,37.1026890903897,46.4834551690612));
#32548=CARTESIAN_POINT('Ctrl Pts',(40.5364302170585,37.1069233411651,46.5441945603769));
#32549=CARTESIAN_POINT('Ctrl Pts',(40.4887304068365,37.1111575919404,46.6074207400574));
#32550=CARTESIAN_POINT('Ctrl Pts',(40.4443778817356,37.1153918427157,46.6727725999457));
#32551=CARTESIAN_POINT('Ctrl Pts',(40.4020772520258,37.119430202961,46.7351010653418));
#32552=CARTESIAN_POINT('Ctrl Pts',(40.3628211983546,37.1234685632063,46.7993625544527));
#32553=CARTESIAN_POINT('Ctrl Pts',(40.3267719914411,37.1275069234516,46.8652242224004));
#32554=CARTESIAN_POINT('Ctrl Pts',(40.2870375488266,37.1319581168942,46.9378187921463));
#32555=CARTESIAN_POINT('Ctrl Pts',(40.2510607328626,37.1364093103368,47.0126102428298));
#32556=CARTESIAN_POINT('Ctrl Pts',(40.2190773612624,37.1408605037794,47.0891943759825));
#32557=CARTESIAN_POINT('Ctrl Pts',(40.1871847111452,37.1452990713214,47.1655612766866));
#32558=CARTESIAN_POINT('Ctrl Pts',(40.1592630955621,37.1497376388635,47.243710364221));
#32559=CARTESIAN_POINT('Ctrl Pts',(40.1355019575057,37.1541762064055,47.3232141724007));
#32560=CARTESIAN_POINT('Ctrl Pts',(40.1117812132541,37.1586072284069,47.4025828245411));
#32561=CARTESIAN_POINT('Ctrl Pts',(40.09220699208,37.1630382504084,47.4833012358813));
#32562=CARTESIAN_POINT('Ctrl Pts',(40.0769205382994,37.1674692724099,47.5649227016671));
#32563=CARTESIAN_POINT('Ctrl Pts',(40.0616673408257,37.1718906545413,47.6463665966073));
#32564=CARTESIAN_POINT('Ctrl Pts',(40.0506834047931,37.1763120366727,47.7287092417238));
#32565=CARTESIAN_POINT('Ctrl Pts',(40.04405967581,37.1807334188041,47.8114910353449));
#32566=CARTESIAN_POINT('Ctrl Pts',(40.039046125874,37.18407999596,47.8741491931837));
#32567=CARTESIAN_POINT('Ctrl Pts',(40.0365295766833,37.1874265731158,47.9370585780173));
#32568=CARTESIAN_POINT('Ctrl Pts',(40.0365300000534,37.1907731502717,48.0000158936656));
#32569=CARTESIAN_POINT('',(40.0365309678968,37.9845231502406,48.0021389691475));
#32570=CARTESIAN_POINT('Ctrl Pts',(40.0365300000535,37.1907731503223,48.0000158946174));
#32571=CARTESIAN_POINT('Ctrl Pts',(40.0365305596263,37.1951960923782,48.0832222712021));
#32572=CARTESIAN_POINT('Ctrl Pts',(40.0409293600083,37.199619034434,48.1663427328736));
#32573=CARTESIAN_POINT('Ctrl Pts',(40.0496735435784,37.2040419764899,48.2489096003468));
#32574=CARTESIAN_POINT('Ctrl Pts',(40.0584419788841,37.2084771854452,48.3317054645947));
#32575=CARTESIAN_POINT('Ctrl Pts',(40.0715798424985,37.2129123944006,48.4139442671402));
#32576=CARTESIAN_POINT('Ctrl Pts',(40.0889826968161,37.217347603356,48.4951660986827));
#32577=CARTESIAN_POINT('Ctrl Pts',(40.106410421701,37.2217891507062,48.5765040050364));
#32578=CARTESIAN_POINT('Ctrl Pts',(40.1281151866957,37.2262306980565,48.6568216568936));
#32579=CARTESIAN_POINT('Ctrl Pts',(40.153942725368,37.2306722454067,48.7356746291485));
#32580=CARTESIAN_POINT('Ctrl Pts',(40.1798413381919,37.235126015339,48.8147445949066));
#32581=CARTESIAN_POINT('Ctrl Pts',(40.2098852628717,37.2395797852712,48.8923414489889));
#32582=CARTESIAN_POINT('Ctrl Pts',(40.2438718313794,37.2440335552035,48.9680401651691));
#32583=CARTESIAN_POINT('Ctrl Pts',(40.268543027072,37.2472665920881,49.0229906330324));
#32584=CARTESIAN_POINT('Ctrl Pts',(40.2952907833685,37.2504996289728,49.076941352625));
#32585=CARTESIAN_POINT('Ctrl Pts',(40.3240230140222,37.2537326658574,49.1297389054956));
#32586=CARTESIAN_POINT('Ctrl Pts',(40.3616642086403,37.2579681661237,49.1989073242974));
#32587=CARTESIAN_POINT('Ctrl Pts',(40.4028376148377,37.2622036663899,49.2663239337141));
#32588=CARTESIAN_POINT('Ctrl Pts',(40.4473558357842,37.2664391666562,49.331604749486));
#32589=CARTESIAN_POINT('Ctrl Pts',(40.4918095194408,37.2706685267914,49.396790928796));
#32590=CARTESIAN_POINT('Ctrl Pts',(40.5395981265472,37.2748978869267,49.4598470785257));
#32591=CARTESIAN_POINT('Ctrl Pts',(40.5904885275618,37.279127247062,49.520413980472));
#32592=CARTESIAN_POINT('Ctrl Pts',(40.6413194991391,37.2833516681814,49.580910152834));
#32593=CARTESIAN_POINT('Ctrl Pts',(40.6952447661712,37.2875760893009,49.6389224965377));
#32594=CARTESIAN_POINT('Ctrl Pts',(40.7519889800698,37.2918005104204,49.6941222267265));
#32595=CARTESIAN_POINT('Ctrl Pts',(40.8086969071162,37.2960222301025,49.7492866577312));
#32596=CARTESIAN_POINT('Ctrl Pts',(40.8682198676082,37.3002439497845,49.8016417186962));
#32597=CARTESIAN_POINT('Ctrl Pts',(40.9302442879937,37.3044656694665,49.8508939969444));
#32598=CARTESIAN_POINT('Ctrl Pts',(40.992248414265,37.3086860078207,49.9001301600665));
#32599=CARTESIAN_POINT('Ctrl Pts',(41.0567520079436,37.3129063461748,49.9462652647038));
#32600=CARTESIAN_POINT('Ctrl Pts',(41.1234080529754,37.317126684529,49.989045862139));
#32601=CARTESIAN_POINT('Ctrl Pts',(41.1900631037294,37.3213469599303,50.0318258214354));
#32602=CARTESIAN_POINT('Ctrl Pts',(41.2588701462979,37.3255672353316,50.0712511206032));
#32603=CARTESIAN_POINT('Ctrl Pts',(41.3294540638705,37.3297875107329,50.1071122038317));
#32604=CARTESIAN_POINT('Ctrl Pts',(41.4001085818039,37.3340120073927,50.1430091564977));
#32605=CARTESIAN_POINT('Ctrl Pts',(41.4725431056581,37.3382365040526,50.1753345584918));
#32606=CARTESIAN_POINT('Ctrl Pts',(41.5463593814678,37.3424610007124,50.2039256192739));
#32607=CARTESIAN_POINT('Ctrl Pts',(41.6202110962784,37.3466875255421,50.2325304065495));
#32608=CARTESIAN_POINT('Ctrl Pts',(41.6954454383171,37.3509140503717,50.2573971335446));
#32609=CARTESIAN_POINT('Ctrl Pts',(41.7716481565412,37.3551405752014,50.2784126934605));
#32610=CARTESIAN_POINT('Ctrl Pts',(41.8479901707795,37.3593748259767,50.2994666691154));
#32611=CARTESIAN_POINT('Ctrl Pts',(41.9253036390266,37.363609076752,50.3166553083815));
#32612=CARTESIAN_POINT('Ctrl Pts',(42.0031634563534,37.3678433275274,50.3299165647136));
#32613=CARTESIAN_POINT('Ctrl Pts',(42.0774212194581,37.3718816877727,50.3425643112019));
#32614=CARTESIAN_POINT('Ctrl Pts',(42.152175538726,37.375920048018,50.3516400196285));
#32615=CARTESIAN_POINT('Ctrl Pts',(42.2270562460282,37.3799584082634,50.3571340434651));
#32616=CARTESIAN_POINT('Ctrl Pts',(42.3055923934863,37.3841939085296,50.3628962682319));
#32617=CARTESIAN_POINT('Ctrl Pts',(42.384566116487,37.3884294087959,50.3647400899557));
#32618=CARTESIAN_POINT('Ctrl Pts',(42.4635530934007,37.3926649090621,50.362615382414));
#32619=CARTESIAN_POINT('Ctrl Pts',(42.5424255642691,37.3968942691974,50.3604937550238));
#32620=CARTESIAN_POINT('Ctrl Pts',(42.6213107856818,37.4011236293326,50.3544150355381));
#32621=CARTESIAN_POINT('Ctrl Pts',(42.6997805239498,37.4053529894679,50.3443809584537));
#32622=CARTESIAN_POINT('Ctrl Pts',(42.7781586258327,37.4095774105874,50.3343585990911));
#32623=CARTESIAN_POINT('Ctrl Pts',(42.8561217456078,37.4138018317069,50.3203901202401));
#32624=CARTESIAN_POINT('Ctrl Pts',(42.9332444047402,37.4180262528264,50.3025292279824));
#32625=CARTESIAN_POINT('Ctrl Pts',(43.0103177453898,37.4222479725084,50.2846797574278));
#32626=CARTESIAN_POINT('Ctrl Pts',(43.086551236123,37.4264696921904,50.2629429194557));
#32627=CARTESIAN_POINT('Ctrl Pts',(43.1615284680203,37.4306914118725,50.2374237044634));
#32628=CARTESIAN_POINT('Ctrl Pts',(43.2364811677012,37.4349117502266,50.2119128392446));
#32629=CARTESIAN_POINT('Ctrl Pts',(43.3101779807556,37.4391320885808,50.1826222055372));
#32630=CARTESIAN_POINT('Ctrl Pts',(43.3822180169668,37.4433524269349,50.149706539983));
#32631=CARTESIAN_POINT('Ctrl Pts',(43.4542569785896,37.4475727023362,50.1167913654169));
#32632=CARTESIAN_POINT('Ctrl Pts',(43.5246387861474,37.4517929777375,50.0802514627571));
#32633=CARTESIAN_POINT('Ctrl Pts',(43.59298426232,37.4560132531388,50.0402889478593));
#32634=CARTESIAN_POINT('Ctrl Pts',(43.6613980998906,37.4602377497986,50.0002864611369));
#32635=CARTESIAN_POINT('Ctrl Pts',(43.7277711311593,37.4644622464585,49.9568547609598));
#32636=CARTESIAN_POINT('Ctrl Pts',(43.7917509927071,37.4686867431183,49.9102407217937));
#32637=CARTESIAN_POINT('Ctrl Pts',(43.8557615708191,37.472913267948,49.8636043033493));
#32638=CARTESIAN_POINT('Ctrl Pts',(43.9173763248841,37.4771397927776,49.8137827978025));
#32639=CARTESIAN_POINT('Ctrl Pts',(43.9762760226218,37.4813663176073,49.7610634120916));
#32640=CARTESIAN_POINT('Ctrl Pts',(44.0352833870323,37.4856005683826,49.7082476571109));
#32641=CARTESIAN_POINT('Ctrl Pts',(44.0915654434044,37.4898348191579,49.6525237679543));
#32642=CARTESIAN_POINT('Ctrl Pts',(44.1448400307035,37.4940690699333,49.5942157031452));
#32643=CARTESIAN_POINT('Ctrl Pts',(44.1956499583269,37.4981074301786,49.5386051634299));
#32644=CARTESIAN_POINT('Ctrl Pts',(44.2437243343442,37.5021457904239,49.4806445638542));
#32645=CARTESIAN_POINT('Ctrl Pts',(44.2888547879471,37.5061841506692,49.420640007514));
#32646=CARTESIAN_POINT('Ctrl Pts',(44.3361883680735,37.5104196509355,49.357706217828));
#32647=CARTESIAN_POINT('Ctrl Pts',(44.3804631859095,37.5146551512017,49.2922845921318));
#32648=CARTESIAN_POINT('Ctrl Pts',(44.4214075295047,37.518890651468,49.2247048789654));
#32649=CARTESIAN_POINT('Ctrl Pts',(44.4622925167979,37.5231200116032,49.1572231349325));
#32650=CARTESIAN_POINT('Ctrl Pts',(44.4998563765131,37.5273493717385,49.0875899141883));
#32651=CARTESIAN_POINT('Ctrl Pts',(44.5338688966298,37.5315787318737,49.016166311632));
#32652=CARTESIAN_POINT('Ctrl Pts',(44.5678416971748,37.5358031529932,48.9448261170354));
#32653=CARTESIAN_POINT('Ctrl Pts',(44.598271198688,37.5400275741127,48.8717001169798));
#32654=CARTESIAN_POINT('Ctrl Pts',(44.6249723892253,37.5442519952322,48.7971752053879));
#32655=CARTESIAN_POINT('Ctrl Pts',(44.6516565048559,37.5484737149142,48.7226979510682));
#32656=CARTESIAN_POINT('Ctrl Pts',(44.6746168837267,37.5526954345963,48.6468240014116));
#32657=CARTESIAN_POINT('Ctrl Pts',(44.6937165520271,37.5569171542783,48.5699603669176));
#32658=CARTESIAN_POINT('Ctrl Pts',(44.7128099710011,37.5611374926325,48.4931218818626));
#32659=CARTESIAN_POINT('Ctrl Pts',(44.7280450746151,37.5653578309866,48.4152948101251));
#32660=CARTESIAN_POINT('Ctrl Pts',(44.7393351225324,37.5695781693408,48.3369000228352));
#32661=CARTESIAN_POINT('Ctrl Pts',(44.7506250020412,37.5737984447421,48.2585064049247));
#32662=CARTESIAN_POINT('Ctrl Pts',(44.7579698772445,37.5780187201433,48.1795455530439));
#32663=CARTESIAN_POINT('Ctrl Pts',(44.7613346015463,37.5822389955446,48.100445708919));
#32664=CARTESIAN_POINT('Ctrl Pts',(44.7647026913562,37.5864634922045,48.0212667465227));
#32665=CARTESIAN_POINT('Ctrl Pts',(44.7640826575644,37.5906879888643,47.9419489842108));
#32666=CARTESIAN_POINT('Ctrl Pts',(44.7594915029145,37.5949124855242,47.8629223264931));
#32667=CARTESIAN_POINT('Ctrl Pts',(44.7548981440633,37.5991390103538,47.7838577282837));
#32668=CARTESIAN_POINT('Ctrl Pts',(44.7463299171458,37.6033655351834,47.7050849803251));
#32669=CARTESIAN_POINT('Ctrl Pts',(44.733855669311,37.6075920600131,47.6270279424343));
#32670=CARTESIAN_POINT('Ctrl Pts',(44.7213586189694,37.6118263107884,47.5488282188951));
#32671=CARTESIAN_POINT('Ctrl Pts',(44.7049413777103,37.6160605615638,47.4713472800671));
#32672=CARTESIAN_POINT('Ctrl Pts',(44.6847237570263,37.6202948123391,47.3949976901039));
#32673=CARTESIAN_POINT('Ctrl Pts',(44.6654414707478,37.6243331725844,47.3221802862202));
#32674=CARTESIAN_POINT('Ctrl Pts',(44.6427028080316,37.6283715328297,47.2503921956308));
#32675=CARTESIAN_POINT('Ctrl Pts',(44.6166524833386,37.632409893075,47.1799742632035));
#32676=CARTESIAN_POINT('Ctrl Pts',(44.5893304638875,37.6366453933413,47.1061187492256));
#32677=CARTESIAN_POINT('Ctrl Pts',(44.5582613401604,37.6408808936075,47.0334898420745));
#32678=CARTESIAN_POINT('Ctrl Pts',(44.5235754460815,37.6451163938738,46.96249445028));
#32679=CARTESIAN_POINT('Ctrl Pts',(44.4889398355394,37.649345754009,46.891601979269));
#32680=CARTESIAN_POINT('Ctrl Pts',(44.4506980709443,37.6535751141443,46.8223387391732));
#32681=CARTESIAN_POINT('Ctrl Pts',(44.4090293004974,37.6578044742796,46.7550936940304));
#32682=CARTESIAN_POINT('Ctrl Pts',(44.3674091905354,37.6620288953991,46.6879271771586));
#32683=CARTESIAN_POINT('Ctrl Pts',(44.322370273441,37.6662533165185,46.6227745686656));
#32684=CARTESIAN_POINT('Ctrl Pts',(44.2741378479749,37.670477737638,46.5600007751086));
#32685=CARTESIAN_POINT('Ctrl Pts',(44.2259362662332,37.6746994573201,46.497267124206));
#32686=CARTESIAN_POINT('Ctrl Pts',(44.1745455146176,37.6789211770021,46.43690964014));
#32687=CARTESIAN_POINT('Ctrl Pts',(44.1202337987159,37.6831428966841,46.3792637109463));
#32688=CARTESIAN_POINT('Ctrl Pts',(44.0659398533657,37.6873632350383,46.3216366432439));
#32689=CARTESIAN_POINT('Ctrl Pts',(44.0087271630969,37.6915835733925,46.266719710067));
#32690=CARTESIAN_POINT('Ctrl Pts',(43.9489027665584,37.6958039117466,46.2148135501725));
#32691=CARTESIAN_POINT('Ctrl Pts',(43.8890792623932,37.7000241871479,46.1629081645386));
#32692=CARTESIAN_POINT('Ctrl Pts',(43.8266444847843,37.7042444625492,46.1140137694976));
#32693=CARTESIAN_POINT('Ctrl Pts',(43.7619395830336,37.7084647379505,46.0683915994523));
#32694=CARTESIAN_POINT('Ctrl Pts',(43.6971699613073,37.7126892346103,46.0227237966088));
#32695=CARTESIAN_POINT('Ctrl Pts',(43.6301260640298,37.7169137312702,45.9803350280738));
#32696=CARTESIAN_POINT('Ctrl Pts',(43.5611786512994,37.72113822793,45.9414435687437));
#32697=CARTESIAN_POINT('Ctrl Pts',(43.4921981370964,37.7253647527597,45.9025334377257));
#32698=CARTESIAN_POINT('Ctrl Pts',(43.4213127073509,37.7295912775893,45.8671241708138));
#32699=CARTESIAN_POINT('Ctrl Pts',(43.3489160857868,37.7338178024189,45.8353871701768));
#32700=CARTESIAN_POINT('Ctrl Pts',(43.2763871256255,37.7380520531943,45.8035921553667));
#32701=CARTESIAN_POINT('Ctrl Pts',(43.2023418936577,37.7422863039696,45.7754829875554));
#32702=CARTESIAN_POINT('Ctrl Pts',(43.1271921849133,37.746520554745,45.7511820956109));
#32703=CARTESIAN_POINT('Ctrl Pts',(43.0555191517504,37.7505589149903,45.7280054437871));
#32704=CARTESIAN_POINT('Ctrl Pts',(42.9828419297207,37.7545972752356,45.7082925512877));
#32705=CARTESIAN_POINT('Ctrl Pts',(42.9095254682162,37.7586356354809,45.692106103362));
#32706=CARTESIAN_POINT('Ctrl Pts',(42.8326299281061,37.7628711357472,45.6751294840575));
#32707=CARTESIAN_POINT('Ctrl Pts',(42.7547388472413,37.7671066360134,45.661967868471));
#32708=CARTESIAN_POINT('Ctrl Pts',(42.6762649566596,37.7713421362797,45.6527317761658));
#32709=CARTESIAN_POINT('Ctrl Pts',(42.5979048283107,37.7755714964149,45.6435090732628));
#32710=CARTESIAN_POINT('Ctrl Pts',(42.5189640302368,37.7798008565502,45.6382006471894));
#32711=CARTESIAN_POINT('Ctrl Pts',(42.4398666097627,37.7840302166855,45.6368662555145));
#32712=CARTESIAN_POINT('Ctrl Pts',(42.3608615586765,37.7882546378049,45.6355334221324));
#32713=CARTESIAN_POINT('Ctrl Pts',(42.2817007154983,37.7924790589244,45.6381654087955));
#32714=CARTESIAN_POINT('Ctrl Pts',(42.2028128615963,37.7967034800439,45.6447701442644));
#32715=CARTESIAN_POINT('Ctrl Pts',(42.1239754549856,37.8009251997259,45.6513706561299));
#32716=CARTESIAN_POINT('Ctrl Pts',(42.0454111576157,37.805146919408,45.6619388354037));
#32717=CARTESIAN_POINT('Ctrl Pts',(41.9675471371779,37.80936863909,45.6764305557318));
#32718=CARTESIAN_POINT('Ctrl Pts',(41.8897085935008,37.8135889774442,45.6909175344335));
#32719=CARTESIAN_POINT('Ctrl Pts',(41.8125703328633,37.8178093157983,45.7093254192435));
#32720=CARTESIAN_POINT('Ctrl Pts',(41.7365513061938,37.8220296541525,45.7315586250496));
#32721=CARTESIAN_POINT('Ctrl Pts',(41.6605334134655,37.8262499295538,45.7537914992131));
#32722=CARTESIAN_POINT('Ctrl Pts',(41.5856351716246,37.830470204955,45.7798494479168));
#32723=CARTESIAN_POINT('Ctrl Pts',(41.5122608450046,37.8346904803563,45.8095868806118));
#32724=CARTESIAN_POINT('Ctrl Pts',(41.4388131269647,37.8389149770162,45.8393540576671));
#32725=CARTESIAN_POINT('Ctrl Pts',(41.3668928050917,37.843139473676,45.8728078939457));
#32726=CARTESIAN_POINT('Ctrl Pts',(41.2968840327574,37.8473639703359,45.9097546546603));
#32727=CARTESIAN_POINT('Ctrl Pts',(41.2268416493946,37.8515904951655,45.946719153418));
#32728=CARTESIAN_POINT('Ctrl Pts',(41.1587130479057,37.8558170199952,45.9871796772976));
#32729=CARTESIAN_POINT('Ctrl Pts',(41.0928553835091,37.8600435448248,46.0308978207115));
#32730=CARTESIAN_POINT('Ctrl Pts',(41.0268773335099,37.8642777956001,46.0746958794258));
#32731=CARTESIAN_POINT('Ctrl Pts',(40.9631788941426,37.8685120463755,46.1217631771429));
#32732=CARTESIAN_POINT('Ctrl Pts',(40.9020858091279,37.8727462971508,46.1718196156604));
#32733=CARTESIAN_POINT('Ctrl Pts',(40.8438190935089,37.8767846573961,46.2195602767729));
#32734=CARTESIAN_POINT('Ctrl Pts',(40.7879222390666,37.8808230176414,46.2700193532216));
#32735=CARTESIAN_POINT('Ctrl Pts',(40.7346454003701,37.8848613778867,46.3229238245114));
#32736=CARTESIAN_POINT('Ctrl Pts',(40.6795730505441,37.8890358370625,46.3776112575783));
#32737=CARTESIAN_POINT('Ctrl Pts',(40.627078497172,37.8932102962383,46.4351326267141));
#32738=CARTESIAN_POINT('Ctrl Pts',(40.5774737031317,37.897384755414,46.4952115304391));
#32739=CARTESIAN_POINT('Ctrl Pts',(40.5279334280921,37.9015537850353,46.5552122919017));
#32740=CARTESIAN_POINT('Ctrl Pts',(40.4812757654333,37.9057228146565,46.6177636240106));
#32741=CARTESIAN_POINT('Ctrl Pts',(40.4377767362262,37.9098918442777,46.6825515934182));
#32742=CARTESIAN_POINT('Ctrl Pts',(40.3943197909756,37.9140568404926,46.7472768824825));
#32743=CARTESIAN_POINT('Ctrl Pts',(40.3540156865703,37.9182218367075,46.8142341180397));
#32744=CARTESIAN_POINT('Ctrl Pts',(40.317099846657,37.9223868329223,46.8830768190679));
#32745=CARTESIAN_POINT('Ctrl Pts',(40.2802074295698,37.9265491864781,46.9518758399137));
#32746=CARTESIAN_POINT('Ctrl Pts',(40.2466992389077,37.9307115400338,47.0225575270902));
#32747=CARTESIAN_POINT('Ctrl Pts',(40.2167661554737,37.9348738935895,47.0947484211476));
#32748=CARTESIAN_POINT('Ctrl Pts',(40.1868300921433,37.9390366615155,47.1669465019482));
#32749=CARTESIAN_POINT('Ctrl Pts',(40.1604700500129,37.9431994294416,47.2406536501797));
#32750=CARTESIAN_POINT('Ctrl Pts',(40.1378293684167,37.9473621973677,47.3154750008202));
#32751=CARTESIAN_POINT('Ctrl Pts',(40.1151890988125,37.9515248895439,47.3902949899385));
#32752=CARTESIAN_POINT('Ctrl Pts',(40.0962681870432,37.9556875817202,47.4662286750739));
#32753=CARTESIAN_POINT('Ctrl Pts',(40.0811598566571,37.9598502738965,47.5428667256461));
#32754=CARTESIAN_POINT('Ctrl Pts',(40.0660351583016,37.9640174758244,47.6195878038747));
#32755=CARTESIAN_POINT('Ctrl Pts',(40.0547313773445,37.9681846777524,47.697014294305));
#32756=CARTESIAN_POINT('Ctrl Pts',(40.0472902807315,37.9723518796803,47.7747281247921));
#32757=CARTESIAN_POINT('Ctrl Pts',(40.0400458033653,37.9764089698671,47.8503884898277));
#32758=CARTESIAN_POINT('Ctrl Pts',(40.0364623514731,37.9804660600538,47.9263207683451));
#32759=CARTESIAN_POINT('Ctrl Pts',(40.0365309678968,37.9845231502406,48.0021389691475));
#32760=CARTESIAN_POINT('',(40.0365302498269,38.7782731502987,47.9989133001977));
#32761=CARTESIAN_POINT('Ctrl Pts',(40.0365309678973,37.9845231502717,48.0021389697293));
#32762=CARTESIAN_POINT('Ctrl Pts',(40.036631185905,37.9904487488876,48.1128755333861));
#32763=CARTESIAN_POINT('Ctrl Pts',(40.0445174814273,37.9963743475034,48.2232732264897));
#32764=CARTESIAN_POINT('Ctrl Pts',(40.0600271988848,38.0022999461193,48.3324420715571));
#32765=CARTESIAN_POINT('Ctrl Pts',(40.0676937429487,38.005229004177,48.3864048702607));
#32766=CARTESIAN_POINT('Ctrl Pts',(40.0772222871004,38.0081580622348,48.440067915169));
#32767=CARTESIAN_POINT('Ctrl Pts',(40.0885892018617,38.0110871202926,48.493326021156));
#32768=CARTESIAN_POINT('Ctrl Pts',(40.1050260800485,38.0153226205589,48.5703387391143));
#32769=CARTESIAN_POINT('Ctrl Pts',(40.1253473352508,38.0195581208251,48.6466754615364));
#32770=CARTESIAN_POINT('Ctrl Pts',(40.1494823962719,38.0237936210914,48.7219147845903));
#32771=CARTESIAN_POINT('Ctrl Pts',(40.1735824691154,38.0280229812266,48.7970450345077));
#32772=CARTESIAN_POINT('Ctrl Pts',(40.2014852263923,38.0322523413619,48.8710806011245));
#32773=CARTESIAN_POINT('Ctrl Pts',(40.2330692122343,38.0364817014972,48.9436108318227));
#32774=CARTESIAN_POINT('Ctrl Pts',(40.2646163145292,38.0407061226167,49.0160563622492));
#32775=CARTESIAN_POINT('Ctrl Pts',(40.2998359162372,38.0449305437362,49.0869996219856));
#32776=CARTESIAN_POINT('Ctrl Pts',(40.3385574354109,38.0491549648557,49.156047141686));
#32777=CARTESIAN_POINT('Ctrl Pts',(40.377254192905,38.0533766845377,49.2250505068028));
#32778=CARTESIAN_POINT('Ctrl Pts',(40.4194481941604,38.0575984042197,49.2921601297526));
#32779=CARTESIAN_POINT('Ctrl Pts',(40.4649221573388,38.0618201239018,49.3570055945875));
#32780=CARTESIAN_POINT('Ctrl Pts',(40.5103812416391,38.0660404622559,49.4218298422752));
#32781=CARTESIAN_POINT('Ctrl Pts',(40.559117887587,38.0702608006101,49.4843910188875));
#32782=CARTESIAN_POINT('Ctrl Pts',(40.6108713941373,38.0744811389643,49.5443475232549));
#32783=CARTESIAN_POINT('Ctrl Pts',(40.662624128704,38.0787014143656,49.6043031332784));
#32784=CARTESIAN_POINT('Ctrl Pts',(40.7173933267255,38.0829216897669,49.6616537938639));
#32785=CARTESIAN_POINT('Ctrl Pts',(40.7748788731974,38.0871419651682,49.7160920033961));
#32786=CARTESIAN_POINT('Ctrl Pts',(40.8324219186076,38.091366461828,49.7705846638196));
#32787=CARTESIAN_POINT('Ctrl Pts',(40.8926863983753,38.0955909584879,49.8221587303494));
#32788=CARTESIAN_POINT('Ctrl Pts',(40.9553367264353,38.0998154551477,49.8705449652209));
#32789=CARTESIAN_POINT('Ctrl Pts',(41.0180171327539,38.1040419799774,49.9189544301973));
#32790=CARTESIAN_POINT('Ctrl Pts',(41.0830852832688,38.108268504807,49.9641727464203));
#32791=CARTESIAN_POINT('Ctrl Pts',(41.1501761374244,38.1124950296367,50.0059737668864));
#32792=CARTESIAN_POINT('Ctrl Pts',(41.2173896314122,38.116729280412,50.0478511982167));
#32793=CARTESIAN_POINT('Ctrl Pts',(41.2866328059631,38.1209635311874,50.0862986229723));
#32794=CARTESIAN_POINT('Ctrl Pts',(41.3575157061365,38.1251977819627,50.1211357660339));
#32795=CARTESIAN_POINT('Ctrl Pts',(41.4251193274894,38.129236142208,50.1543612269389));
#32796=CARTESIAN_POINT('Ctrl Pts',(41.4942139689906,38.1332745024533,50.1843029578225));
#32797=CARTESIAN_POINT('Ctrl Pts',(41.5644474597846,38.1373128626985,50.2108465332174));
#32798=CARTESIAN_POINT('Ctrl Pts',(41.6381095282704,38.1415483629648,50.2386858823157));
#32799=CARTESIAN_POINT('Ctrl Pts',(41.7133044804439,38.145783863231,50.2628926534915));
#32800=CARTESIAN_POINT('Ctrl Pts',(41.7896397254383,38.1500193634973,50.283298223215));
#32801=CARTESIAN_POINT('Ctrl Pts',(41.865864308557,38.1542487236325,50.3036742113395));
#32802=CARTESIAN_POINT('Ctrl Pts',(41.9432254522109,38.1584780837678,50.3202598207785));
#32803=CARTESIAN_POINT('Ctrl Pts',(42.0213120794316,38.1627074439031,50.3329350397548));
#32804=CARTESIAN_POINT('Ctrl Pts',(42.0993075176613,38.1669318650225,50.3455954567033));
#32805=CARTESIAN_POINT('Ctrl Pts',(42.1780262950039,38.171156286142,50.3543544829134));
#32806=CARTESIAN_POINT('Ctrl Pts',(42.2570452093146,38.1753807072615,50.3591427190232));
#32807=CARTESIAN_POINT('Ctrl Pts',(42.3360135925232,38.1796024269436,50.3639278931465));
#32808=CARTESIAN_POINT('Ctrl Pts',(42.4152812645295,38.1838241466256,50.3647472887163));
#32809=CARTESIAN_POINT('Ctrl Pts',(42.4944191474996,38.1880458663076,50.3615832539814));
#32810=CARTESIAN_POINT('Ctrl Pts',(42.5735311369069,38.1922662046618,50.3584202545046));
#32811=CARTESIAN_POINT('Ctrl Pts',(42.6525129529803,38.1964865430159,50.3512764315013));
#32812=CARTESIAN_POINT('Ctrl Pts',(42.7309362625019,38.2007068813701,50.340186238542));
#32813=CARTESIAN_POINT('Ctrl Pts',(42.8093584022186,38.2049271567713,50.3290962110101));
#32814=CARTESIAN_POINT('Ctrl Pts',(42.8872215874029,38.2091474321726,50.3140599975754));
#32815=CARTESIAN_POINT('Ctrl Pts',(42.9641048409025,38.2133677075739,50.2951636476231));
#32816=CARTESIAN_POINT('Ctrl Pts',(43.0410649955664,38.2175922042337,50.2762483969186));
#32817=CARTESIAN_POINT('Ctrl Pts',(43.1170428036769,38.2218167008936,50.2534654090814));
#32818=CARTESIAN_POINT('Ctrl Pts',(43.1916302795124,38.2260411975534,50.2269512660719));
#32819=CARTESIAN_POINT('Ctrl Pts',(43.2662535646001,38.2302677223831,50.2004243936916));
#32820=CARTESIAN_POINT('Ctrl Pts',(43.3394847533105,38.2344942472127,50.1701629771104));
#32821=CARTESIAN_POINT('Ctrl Pts',(43.4109361658329,38.2387207720423,50.1363516820765));
#32822=CARTESIAN_POINT('Ctrl Pts',(43.4825181891421,38.2429550228177,50.1024785811288));
#32823=CARTESIAN_POINT('Ctrl Pts',(43.5523135205644,38.247189273593,50.0650428574967));
#32824=CARTESIAN_POINT('Ctrl Pts',(43.6199595813607,38.2514235243683,50.0242749469245));
#32825=CARTESIAN_POINT('Ctrl Pts',(43.6844761102974,38.2554618846137,49.9853930955476));
#32826=CARTESIAN_POINT('Ctrl Pts',(43.7470375593339,38.259500244859,49.9434807843835));
#32827=CARTESIAN_POINT('Ctrl Pts',(43.8073571720049,38.2635386051043,49.8987722958023));
#32828=CARTESIAN_POINT('Ctrl Pts',(43.870621398079,38.2677741053706,49.8518812797002));
#32829=CARTESIAN_POINT('Ctrl Pts',(43.9316598011957,38.2720096056368,49.8017358716542));
#32830=CARTESIAN_POINT('Ctrl Pts',(43.990118175916,38.2762451059031,49.7485750277073));
#32831=CARTESIAN_POINT('Ctrl Pts',(44.0484918045484,38.2804744660383,49.6954912501102));
#32832=CARTESIAN_POINT('Ctrl Pts',(44.1042924879004,38.2847038261736,49.6394010305941));
#32833=CARTESIAN_POINT('Ctrl Pts',(44.1571969035576,38.2889331863089,49.5805851710767));
#32834=CARTESIAN_POINT('Ctrl Pts',(44.2100395378259,38.2931576074283,49.521837996289));
#32835=CARTESIAN_POINT('Ctrl Pts',(44.259992313289,38.2973820285478,49.4603718538201));
#32836=CARTESIAN_POINT('Ctrl Pts',(44.306767914377,38.3016064496673,49.3965051240874));
#32837=CARTESIAN_POINT('Ctrl Pts',(44.3535136033523,38.3058281693494,49.3326792359213));
#32838=CARTESIAN_POINT('Ctrl Pts',(44.397085873951,38.3100498890314,49.2664561850306));
#32839=CARTESIAN_POINT('Ctrl Pts',(44.4372377530987,38.3142716087134,49.1981872884693));
#32840=CARTESIAN_POINT('Ctrl Pts',(44.4773764947304,38.3184919470676,49.1299407291868));
#32841=CARTESIAN_POINT('Ctrl Pts',(44.514096829383,38.3227122854218,49.0596500576837));
#32842=CARTESIAN_POINT('Ctrl Pts',(44.5471960088507,38.3269326237759,48.9876941533064));
#32843=CARTESIAN_POINT('Ctrl Pts',(44.580294694593,38.3311528991772,48.9157393222626));
#32844=CARTESIAN_POINT('Ctrl Pts',(44.6097721375908,38.3353731745785,48.8421197346801));
#32845=CARTESIAN_POINT('Ctrl Pts',(44.6354729627353,38.3395934499798,48.7672359961443));
#32846=CARTESIAN_POINT('Ctrl Pts',(44.6611994946922,38.3438179466396,48.6922773564249));
#32847=CARTESIAN_POINT('Ctrl Pts',(44.6831417100419,38.3480424432995,48.6160524848565));
#32848=CARTESIAN_POINT('Ctrl Pts',(44.7011937612435,38.3522669399593,48.5389783985599));
#32849=CARTESIAN_POINT('Ctrl Pts',(44.7192544791876,38.356493464789,48.4618673091959));
#32850=CARTESIAN_POINT('Ctrl Pts',(44.7334212283509,38.3607199896186,48.3839066553275));
#32851=CARTESIAN_POINT('Ctrl Pts',(44.7436395863326,38.3649465144483,48.3055223891544));
#32852=CARTESIAN_POINT('Ctrl Pts',(44.7538766231302,38.3691807652236,48.2269948391707));
#32853=CARTESIAN_POINT('Ctrl Pts',(44.7601508091553,38.373415015999,48.1480425986582));
#32854=CARTESIAN_POINT('Ctrl Pts',(44.7624597953243,38.3776492667743,48.0690952702895));
#32855=CARTESIAN_POINT('Ctrl Pts',(44.7646619601101,38.3816876270196,47.9938003080227));
#32856=CARTESIAN_POINT('Ctrl Pts',(44.763257741574,38.3857259872649,47.9185101698709));
#32857=CARTESIAN_POINT('Ctrl Pts',(44.7582890449573,38.3897643475102,47.8435927708376));
#32858=CARTESIAN_POINT('Ctrl Pts',(44.7530777922299,38.3939998477765,47.7650181404736));
#32859=CARTESIAN_POINT('Ctrl Pts',(44.7439253532618,38.3982353480427,47.6865548913434));
#32860=CARTESIAN_POINT('Ctrl Pts',(44.7308410746641,38.402470848309,47.608630193348));
#32861=CARTESIAN_POINT('Ctrl Pts',(44.7177757641172,38.4067002084442,47.5308184614305));
#32862=CARTESIAN_POINT('Ctrl Pts',(44.7007900100373,38.4109295685795,47.4535441892162));
#32863=CARTESIAN_POINT('Ctrl Pts',(44.6799450600438,38.4151589287148,47.3772312113778));
#32864=CARTESIAN_POINT('Ctrl Pts',(44.6591244526301,38.4193833498342,47.3010073512756));
#32865=CARTESIAN_POINT('Ctrl Pts',(44.6344537280659,38.4236077709537,47.2257430051616));
#32866=CARTESIAN_POINT('Ctrl Pts',(44.6060452179403,38.4278321920732,47.1518520545903));
#32867=CARTESIAN_POINT('Ctrl Pts',(44.57765487452,38.4320539117553,47.0780083558852));
#32868=CARTESIAN_POINT('Ctrl Pts',(44.5455316576349,38.4362756314373,47.0055367464692));
#32869=CARTESIAN_POINT('Ctrl Pts',(44.5098374244564,38.4404973511193,46.9348349971655));
#32870=CARTESIAN_POINT('Ctrl Pts',(44.4741548702719,38.4447176894735,46.8641563811594));
#32871=CARTESIAN_POINT('Ctrl Pts',(44.4349038312564,38.4489380278276,46.7952468940508));
#32872=CARTESIAN_POINT('Ctrl Pts',(44.3922932705203,38.4531583661818,46.7284820232732));
#32873=CARTESIAN_POINT('Ctrl Pts',(44.3496833453866,38.4573786415831,46.6617181483968));
#32874=CARTESIAN_POINT('Ctrl Pts',(44.3037142517748,38.4615989169843,46.597099221185));
#32875=CARTESIAN_POINT('Ctrl Pts',(44.2546388536143,38.4658191923856,46.5349726406772));
#32876=CARTESIAN_POINT('Ctrl Pts',(44.2055143686229,38.4700436890455,46.4727839191158));
#32877=CARTESIAN_POINT('Ctrl Pts',(44.1532776640307,38.4742681857053,46.4130928933797));
#32878=CARTESIAN_POINT('Ctrl Pts',(44.0982222003218,38.4784926823652,46.3562141869348));
#32879=CARTESIAN_POINT('Ctrl Pts',(44.0431403046286,38.4827192071948,46.2993081731717));
#32880=CARTESIAN_POINT('Ctrl Pts',(43.9852372973732,38.4869457320244,46.2452174892767));
#32881=CARTESIAN_POINT('Ctrl Pts',(43.9248419742549,38.4911722568541,46.1942183425313));
#32882=CARTESIAN_POINT('Ctrl Pts',(43.8643362505107,38.4954065076294,46.1431259710553));
#32883=CARTESIAN_POINT('Ctrl Pts',(43.8013294815712,38.4996407584048,46.0951367143406));
#32884=CARTESIAN_POINT('Ctrl Pts',(43.7361817045074,38.5038750091801,46.050484959422));
#32885=CARTESIAN_POINT('Ctrl Pts',(43.674047880385,38.5079133694254,46.0078989432614));
#32886=CARTESIAN_POINT('Ctrl Pts',(43.6099670907946,38.5119517296707,45.9683486064981));
#32887=CARTESIAN_POINT('Ctrl Pts',(43.5442714329593,38.515990089916,45.9319977445338));
#32888=CARTESIAN_POINT('Ctrl Pts',(43.4753687201376,38.5202255901823,45.8938723480422));
#32889=CARTESIAN_POINT('Ctrl Pts',(43.404427533846,38.5244610904485,45.8591218560936));
#32890=CARTESIAN_POINT('Ctrl Pts',(43.3318121923973,38.5286965907148,45.8279695032068));
#32891=CARTESIAN_POINT('Ctrl Pts',(43.2593021201448,38.53292595085,45.7968623113436));
#32892=CARTESIAN_POINT('Ctrl Pts',(43.1851231400017,38.5371553109853,45.7693430836499));
#32893=CARTESIAN_POINT('Ctrl Pts',(43.1096648432644,38.5413846711206,45.7455896001095));
#32894=CARTESIAN_POINT('Ctrl Pts',(43.034294666173,38.54560909224,45.7218638557131));
#32895=CARTESIAN_POINT('Ctrl Pts',(42.957648586665,38.5498335133595,45.7018952568009));
#32896=CARTESIAN_POINT('Ctrl Pts',(42.8801354611772,38.554057934479,45.6858132357521));
#32897=CARTESIAN_POINT('Ctrl Pts',(42.8026719038681,38.5582796541611,45.6697414988519));
#32898=CARTESIAN_POINT('Ctrl Pts',(42.724342859386,38.5625013738431,45.6575515019318));
#32899=CARTESIAN_POINT('Ctrl Pts',(42.6455704275094,38.5667230935251,45.6493223091983));
#32900=CARTESIAN_POINT('Ctrl Pts',(42.5668237696217,38.5709434318793,45.64109580902));
#32901=CARTESIAN_POINT('Ctrl Pts',(42.487634478867,38.5751637702335,45.6368275884164));
#32902=CARTESIAN_POINT('Ctrl Pts',(42.4084313979796,38.5793841085876,45.6365450390523));
#32903=CARTESIAN_POINT('Ctrl Pts',(42.3292294985286,38.5836043839889,45.636262493903));
#32904=CARTESIAN_POINT('Ctrl Pts',(42.250014278707,38.5878246593902,45.639965502155));
#32905=CARTESIAN_POINT('Ctrl Pts',(42.171214708091,38.5920449347915,45.6476293380706));
#32906=CARTESIAN_POINT('Ctrl Pts',(42.0923363195471,38.5962694314513,45.6553008396075));
#32907=CARTESIAN_POINT('Ctrl Pts',(42.0138748789772,38.6004939281112,45.6669410373619));
#32908=CARTESIAN_POINT('Ctrl Pts',(41.9362537531706,38.604718424771,45.6824733314476));
#32909=CARTESIAN_POINT('Ctrl Pts',(41.8585953616645,38.6089449496007,45.6980130825471));
#32910=CARTESIAN_POINT('Ctrl Pts',(41.7817785442484,38.6131714744303,45.7174485371472));
#32911=CARTESIAN_POINT('Ctrl Pts',(41.7062134746732,38.61739799926,45.7406525946249));
#32912=CARTESIAN_POINT('Ctrl Pts',(41.6305102746842,38.6216322500353,45.7638990683419));
#32913=CARTESIAN_POINT('Ctrl Pts',(41.5560638371381,38.6258665008106,45.7909277499394));
#32914=CARTESIAN_POINT('Ctrl Pts',(41.4832660651006,38.630100751586,45.8215626395272));
#32915=CARTESIAN_POINT('Ctrl Pts',(41.4138361602268,38.6341391118313,45.8507802571872));
#32916=CARTESIAN_POINT('Ctrl Pts',(41.3459060551789,38.6381774720766,45.8832776041683));
#32917=CARTESIAN_POINT('Ctrl Pts',(41.2797931682581,38.6422158323219,45.9188639893033));
#32918=CARTESIAN_POINT('Ctrl Pts',(41.2104528585419,38.6464513325882,45.9561875896158));
#32919=CARTESIAN_POINT('Ctrl Pts',(41.1428481414697,38.6506868328544,45.997051397964));
#32920=CARTESIAN_POINT('Ctrl Pts',(41.0773638566439,38.6549223331207,46.0412697803965));
#32921=CARTESIAN_POINT('Ctrl Pts',(41.0119745032457,38.6591516932559,46.0854240602098));
#32922=CARTESIAN_POINT('Ctrl Pts',(40.9486998634504,38.6633810533912,46.1329229964788));
#32923=CARTESIAN_POINT('Ctrl Pts',(40.8879002207895,38.6676104135264,46.183535109447));
#32924=CARTESIAN_POINT('Ctrl Pts',(40.8271715795058,38.6718348346459,46.2340881179607));
#32925=CARTESIAN_POINT('Ctrl Pts',(40.7689125506755,38.6760592557654,46.2877467799475));
#32926=CARTESIAN_POINT('Ctrl Pts',(40.7134531784151,38.6802836768849,46.3442372574847));
#32927=CARTESIAN_POINT('Ctrl Pts',(40.658029271375,38.6845053965669,46.4006916104291));
#32928=CARTESIAN_POINT('Ctrl Pts',(40.6054017954103,38.688727116249,46.45997385067));
#32929=CARTESIAN_POINT('Ctrl Pts',(40.5558655981254,38.692948835931,46.5217717535094));
#32930=CARTESIAN_POINT('Ctrl Pts',(40.5063456088636,38.6971691742851,46.5835494363503));
#32931=CARTESIAN_POINT('Ctrl Pts',(40.4599151832051,38.7013895126393,46.6478407814173));
#32932=CARTESIAN_POINT('Ctrl Pts',(40.4168293585783,38.7056098509934,46.7142999385925));
#32933=CARTESIAN_POINT('Ctrl Pts',(40.3737441766433,38.7098301263947,46.7807581044266));
#32934=CARTESIAN_POINT('Ctrl Pts',(40.3340037507722,38.714050401796,46.8493836235362));
#32935=CARTESIAN_POINT('Ctrl Pts',(40.2978193548152,38.7182706771973,46.9198023440545));
#32936=CARTESIAN_POINT('Ctrl Pts',(40.2615987660326,38.7224951738571,46.9902914996981));
#32937=CARTESIAN_POINT('Ctrl Pts',(40.2289415274616,38.726719670517,47.0625770212704));
#32938=CARTESIAN_POINT('Ctrl Pts',(40.2000122542779,38.7309441671768,47.1362614055327));
#32939=CARTESIAN_POINT('Ctrl Pts',(40.1710690922257,38.7351706920065,47.2099811654751));
#32940=CARTESIAN_POINT('Ctrl Pts',(40.1458576105764,38.7393972168361,47.2851006804262));
#32941=CARTESIAN_POINT('Ctrl Pts',(40.1244928146473,38.7436237416657,47.3612062223941));
#32942=CARTESIAN_POINT('Ctrl Pts',(40.1030889645874,38.7478579924411,47.4374508827413));
#32943=CARTESIAN_POINT('Ctrl Pts',(40.0855459552939,38.7520922432164,47.5146847128752));
#32944=CARTESIAN_POINT('Ctrl Pts',(40.0719277821424,38.7563264939918,47.5924828968751));
#32945=CARTESIAN_POINT('Ctrl Pts',(40.0589396309943,38.7603648542371,47.6666818780156));
#32946=CARTESIAN_POINT('Ctrl Pts',(40.049521203197,38.7644032144824,47.7413937910581));
#32947=CARTESIAN_POINT('Ctrl Pts',(40.0436838427263,38.7684415747277,47.8162485160041));
#32948=CARTESIAN_POINT('Ctrl Pts',(40.038946734349,38.7717187665757,47.876994283958));
#32949=CARTESIAN_POINT('Ctrl Pts',(40.0365582913862,38.7749959584237,47.9379255771268));
#32950=CARTESIAN_POINT('Ctrl Pts',(40.0365302498271,38.7782731502717,47.9989132996958));
#32951=CARTESIAN_POINT('',(40.036530522818,39.5720231502423,47.9984279538409));
#32952=CARTESIAN_POINT('Ctrl Pts',(40.0365302498269,38.7782731502987,47.9989133001977));
#32953=CARTESIAN_POINT('Ctrl Pts',(40.0364944094856,38.7824617807574,48.0768626678913));
#32954=CARTESIAN_POINT('Ctrl Pts',(40.0403190670139,38.7866504112161,48.1549693244316));
#32955=CARTESIAN_POINT('Ctrl Pts',(40.0480246341257,38.7908390416748,48.2328139154357));
#32956=CARTESIAN_POINT('Ctrl Pts',(40.0559832392965,38.7951652198189,48.3132147938517));
#32957=CARTESIAN_POINT('Ctrl Pts',(40.0680821762149,38.799491397963,48.3933355850916));
#32958=CARTESIAN_POINT('Ctrl Pts',(40.0842854859267,38.8038175761071,48.4727121007655));
#32959=CARTESIAN_POINT('Ctrl Pts',(40.0999358242399,38.8079961144899,48.5493797289548));
#32960=CARTESIAN_POINT('Ctrl Pts',(40.1194148280676,38.8121746528727,48.6253525429861));
#32961=CARTESIAN_POINT('Ctrl Pts',(40.1426374764409,38.8163531912554,48.7002177362298));
#32962=CARTESIAN_POINT('Ctrl Pts',(40.1658480869031,38.8205295636116,48.7750441216459));
#32963=CARTESIAN_POINT('Ctrl Pts',(40.1927983500028,38.8247059359678,48.8487635673267));
#32964=CARTESIAN_POINT('Ctrl Pts',(40.2233528447225,38.828882308324,48.9209764396131));
#32965=CARTESIAN_POINT('Ctrl Pts',(40.2539015380945,38.8330578877171,48.9931756009222));
#32966=CARTESIAN_POINT('Ctrl Pts',(40.2880529168436,38.8372334671101,49.0638683146151));
#32967=CARTESIAN_POINT('Ctrl Pts',(40.325623280202,38.8414090465031,49.1326745628203));
#32968=CARTESIAN_POINT('Ctrl Pts',(40.3631988521081,38.8455852047755,49.2014903499437));
#32969=CARTESIAN_POINT('Ctrl Pts',(40.4041941166697,38.8497613630478,49.2684187322828));
#32970=CARTESIAN_POINT('Ctrl Pts',(40.4483800556006,38.8539375213201,49.3331054097566));
#32971=CARTESIAN_POINT('Ctrl Pts',(40.4926135023509,38.8581181697125,49.3978616370254));
#32972=CARTESIAN_POINT('Ctrl Pts',(40.5400441945344,38.8622988181049,49.4603709549415));
#32973=CARTESIAN_POINT('Ctrl Pts',(40.59040104084,38.8664794664973,49.5203098525982));
#32974=CARTESIAN_POINT('Ctrl Pts',(40.6407904831372,38.8706628210238,49.5802875487091));
#32975=CARTESIAN_POINT('Ctrl Pts',(40.6941095189094,38.8748461755504,49.6376911652412));
#32976=CARTESIAN_POINT('Ctrl Pts',(40.7500500103594,38.8790295300769,49.6922338705347));
#32977=CARTESIAN_POINT('Ctrl Pts',(40.8060799215419,38.8832195716101,49.7468637612282));
#32978=CARTESIAN_POINT('Ctrl Pts',(40.8647392847159,38.8874096131434,49.7986233057304));
#32979=CARTESIAN_POINT('Ctrl Pts',(40.9256874243613,38.8915996546766,49.8472663235748));
#32980=CARTESIAN_POINT('Ctrl Pts',(40.9405614471548,38.892622208829,49.8591373562326));
#32981=CARTESIAN_POINT('Ctrl Pts',(40.9555716547226,38.8936447629813,49.8708229831906));
#32982=CARTESIAN_POINT('Ctrl Pts',(40.9707128576697,38.8946673171336,49.882320032744));
#32983=CARTESIAN_POINT('Ctrl Pts',(41.0334289191787,38.8989028173999,49.9299417223468));
#32984=CARTESIAN_POINT('Ctrl Pts',(41.0986468176736,38.9031383176661,49.9745160907557));
#32985=CARTESIAN_POINT('Ctrl Pts',(41.1660380541219,38.9073738179324,50.0157699166881));
#32986=CARTESIAN_POINT('Ctrl Pts',(41.2333315946683,38.9116031780677,50.0569639376675));
#32987=CARTESIAN_POINT('Ctrl Pts',(41.3027918196159,38.9158325382029,50.0948467324187));
#32988=CARTESIAN_POINT('Ctrl Pts',(41.3740586935887,38.9200618983382,50.1291864354018));
#32989=CARTESIAN_POINT('Ctrl Pts',(41.4452423426282,38.9242863194577,50.1634860367314));
#32990=CARTESIAN_POINT('Ctrl Pts',(41.5182280275148,38.9285107405772,50.1942505657886));
#32991=CARTESIAN_POINT('Ctrl Pts',(41.5926297068378,38.9327351616967,50.2212932383229));
#32992=CARTESIAN_POINT('Ctrl Pts',(41.6669838076932,38.9369568813787,50.2483186175794));
#32993=CARTESIAN_POINT('Ctrl Pts',(41.7427516658322,38.9411786010607,50.271626704318));
#32994=CARTESIAN_POINT('Ctrl Pts',(41.8195269031812,38.9454003207427,50.2910786596644));
#32995=CARTESIAN_POINT('Ctrl Pts',(41.8962770200146,38.9496206590969,50.3105242504177));
#32996=CARTESIAN_POINT('Ctrl Pts',(41.9740334069304,38.953840997451,50.3261160999281));
#32997=CARTESIAN_POINT('Ctrl Pts',(42.0523755950056,38.9580613358052,50.3377655387041));
#32998=CARTESIAN_POINT('Ctrl Pts',(42.1307166144861,38.9622816112065,50.3494148037106));
#32999=CARTESIAN_POINT('Ctrl Pts',(42.2096429533133,38.9665018866078,50.3571217071647));
#33000=CARTESIAN_POINT('Ctrl Pts',(42.2887265354423,38.9707221620091,50.3608491389721));
#33001=CARTESIAN_POINT('Ctrl Pts',(42.3678892195767,38.9749466586689,50.3645802990797));
#33002=CARTESIAN_POINT('Ctrl Pts',(42.4472089912483,38.9791711553287,50.3643240140422));
#33003=CARTESIAN_POINT('Ctrl Pts',(42.5262558724953,38.9833956519886,50.3600953149313));
#33004=CARTESIAN_POINT('Ctrl Pts',(42.6053407039433,38.9876221768182,50.355864585633));
#33005=CARTESIAN_POINT('Ctrl Pts',(42.6841519165021,38.9918487016479,50.347657691673));
#33006=CARTESIAN_POINT('Ctrl Pts',(42.7622653390865,38.9960752264775,50.3355415357036));
#33007=CARTESIAN_POINT('Ctrl Pts',(42.8405215503886,39.0003094772528,50.3234032318072));
#33008=CARTESIAN_POINT('Ctrl Pts',(42.9180769620872,39.0045437280282,50.3073414819502));
#33009=CARTESIAN_POINT('Ctrl Pts',(42.9945184649252,39.0087779788035,50.2874742043929));
#33010=CARTESIAN_POINT('Ctrl Pts',(43.0674235294882,39.0128163390488,50.2685260532024));
#33011=CARTESIAN_POINT('Ctrl Pts',(43.1393151421295,39.0168546992941,50.2461168416051));
#33012=CARTESIAN_POINT('Ctrl Pts',(43.2098517979214,39.0208930595394,50.2203897194645));
#33013=CARTESIAN_POINT('Ctrl Pts',(43.2838318309644,39.0251285598057,50.1934066802957));
#33014=CARTESIAN_POINT('Ctrl Pts',(43.3566024538726,39.0293640600719,50.1626709511733));
#33015=CARTESIAN_POINT('Ctrl Pts',(43.4277561646983,39.0335995603382,50.1283109986148));
#33016=CARTESIAN_POINT('Ctrl Pts',(43.4988067252283,39.0378289204734,50.0940008570812));
#33017=CARTESIAN_POINT('Ctrl Pts',(43.5682446093869,39.0420582806087,50.0560771279466));
#33018=CARTESIAN_POINT('Ctrl Pts',(43.6356800356732,39.0462876407439,50.0147171737836));
#33019=CARTESIAN_POINT('Ctrl Pts',(43.703036711363,39.0505120618634,49.9734055194719));
#33020=CARTESIAN_POINT('Ctrl Pts',(43.7683951781113,39.0547364829829,49.9286658584228));
#33021=CARTESIAN_POINT('Ctrl Pts',(43.8313895000035,39.0589609041024,49.8807218136077));
#33022=CARTESIAN_POINT('Ctrl Pts',(43.8943435382175,39.0631826237844,49.8328084281031));
#33023=CARTESIAN_POINT('Ctrl Pts',(43.954936059751,39.0674043434665,49.7816950094286));
#33024=CARTESIAN_POINT('Ctrl Pts',(44.0128304501349,39.0716260631485,49.7276482223004));
#33025=CARTESIAN_POINT('Ctrl Pts',(44.070705897732,39.0758464015027,49.6736191190403));
#33026=CARTESIAN_POINT('Ctrl Pts',(44.1258846243335,39.0800667398568,49.6166588731842));
#33027=CARTESIAN_POINT('Ctrl Pts',(44.1780645862994,39.084287078211,49.5570731414574));
#33028=CARTESIAN_POINT('Ctrl Pts',(44.2302437699205,39.0885073536123,49.4974882985438));
#33029=CARTESIAN_POINT('Ctrl Pts',(44.2794239696128,39.0927276290135,49.4352784015845));
#33030=CARTESIAN_POINT('Ctrl Pts',(44.3253423892487,39.0969479044148,49.3707833983026));
#33031=CARTESIAN_POINT('Ctrl Pts',(44.3713067380016,39.1011724010747,49.3062238849925));
#33032=CARTESIAN_POINT('Ctrl Pts',(44.4140025164947,39.1053968977345,49.2393750827672));
#33033=CARTESIAN_POINT('Ctrl Pts',(44.4532097518632,39.1096213943944,49.1706067468428));
#33034=CARTESIAN_POINT('Ctrl Pts',(44.4924358105229,39.113847919224,49.1018053954202));
#33035=CARTESIAN_POINT('Ctrl Pts',(44.5281697776149,39.1180744440537,49.0310830939211));
#33036=CARTESIAN_POINT('Ctrl Pts',(44.5602384472003,39.1223009688833,48.9588327758986));
#33037=CARTESIAN_POINT('Ctrl Pts',(44.5923657372387,39.1265352196587,48.886450386717));
#33038=CARTESIAN_POINT('Ctrl Pts',(44.6208141724858,39.130769470434,48.8125348387977));
#33039=CARTESIAN_POINT('Ctrl Pts',(44.6454594369158,39.1350037212094,48.7374973613957));
#33040=CARTESIAN_POINT('Ctrl Pts',(44.6689645294081,39.1390420814547,48.6659313673799));
#33041=CARTESIAN_POINT('Ctrl Pts',(44.6890105040941,39.1430804417,48.5933453106503));
#33042=CARTESIAN_POINT('Ctrl Pts',(44.7055330027674,39.1471188019453,48.520103849294));
#33043=CARTESIAN_POINT('Ctrl Pts',(44.7228620777578,39.1513543022116,48.4432869706032));
#33044=CARTESIAN_POINT('Ctrl Pts',(44.7363807545826,39.1555898024778,48.3654570664529));
#33045=CARTESIAN_POINT('Ctrl Pts',(44.7459766221029,39.1598253027441,48.287026356711));
#33046=CARTESIAN_POINT('Ctrl Pts',(44.7555585786611,39.1640546628793,48.2087093466035));
#33047=CARTESIAN_POINT('Ctrl Pts',(44.7612289624345,39.1682840230146,48.1297937224487));
#33048=CARTESIAN_POINT('Ctrl Pts',(44.7629260718499,39.1725133831498,48.0507032530708));
#33049=CARTESIAN_POINT('Ctrl Pts',(44.7646211993933,39.1767378042693,47.9717051449633));
#33050=CARTESIAN_POINT('Ctrl Pts',(44.7623522630275,39.1809622253888,47.8925330641883));
#33051=CARTESIAN_POINT('Ctrl Pts',(44.7561093677323,39.1851866465083,47.8136157512448));
#33052=CARTESIAN_POINT('Ctrl Pts',(44.7498704646507,39.1894083661903,47.7347489044312));
#33053=CARTESIAN_POINT('Ctrl Pts',(44.7396626834337,39.1936300858724,47.6561369687152));
#33054=CARTESIAN_POINT('Ctrl Pts',(44.7255281910292,39.1978518055544,47.5782073096548));
#33055=CARTESIAN_POINT('Ctrl Pts',(44.7113983233675,39.2020721439085,47.5003031488318));
#33056=CARTESIAN_POINT('Ctrl Pts',(44.6933443794085,39.2062924822627,47.4230812828554));
#33057=CARTESIAN_POINT('Ctrl Pts',(44.6714600219979,39.2105128206168,47.3469610965911));
#33058=CARTESIAN_POINT('Ctrl Pts',(44.6495759910263,39.2147330960181,47.2708420457771));
#33059=CARTESIAN_POINT('Ctrl Pts',(44.6238617911444,39.2189533714194,47.1958250927204));
#33060=CARTESIAN_POINT('Ctrl Pts',(44.5944611574601,39.2231736468207,47.1223151651653));
#33061=CARTESIAN_POINT('Ctrl Pts',(44.5650311162929,39.2273981434805,47.0487317105576));
#33062=CARTESIAN_POINT('Ctrl Pts',(44.5319074502033,39.2316226401404,46.976658729456));
#33063=CARTESIAN_POINT('Ctrl Pts',(44.495282130258,39.2358471368002,46.9064812596387));
#33064=CARTESIAN_POINT('Ctrl Pts',(44.4586392265924,39.2400736616298,46.8362700978017));
#33065=CARTESIAN_POINT('Ctrl Pts',(44.4184915581805,39.2443001864595,46.7679566653412));
#33066=CARTESIAN_POINT('Ctrl Pts',(44.3750758902299,39.2485267112891,46.701899207021));
#33067=CARTESIAN_POINT('Ctrl Pts',(44.3315808598937,39.2527609620645,46.6357209978816));
#33068=CARTESIAN_POINT('Ctrl Pts',(44.2848061708965,39.2569952128398,46.5718073830453));
#33069=CARTESIAN_POINT('Ctrl Pts',(44.2350304246718,39.2612294636151,46.510485387306));
#33070=CARTESIAN_POINT('Ctrl Pts',(44.1875574700924,39.2652678238605,46.4520003511339));
#33071=CARTESIAN_POINT('Ctrl Pts',(44.1373552608477,39.2693061841058,46.3958726848754));
#33072=CARTESIAN_POINT('Ctrl Pts',(44.0846956673817,39.2733445443511,46.3423537925102));
#33073=CARTESIAN_POINT('Ctrl Pts',(44.029465398511,39.2775800446174,46.286222276476));
#33074=CARTESIAN_POINT('Ctrl Pts',(43.9713217538187,39.2818155448836,46.2327473740915));
#33075=CARTESIAN_POINT('Ctrl Pts',(43.9105506083137,39.2860510451499,46.1822466337197));
#33076=CARTESIAN_POINT('Ctrl Pts',(43.8498675616802,39.2902804052851,46.131819103392));
#33077=CARTESIAN_POINT('Ctrl Pts',(43.7865649362458,39.2945097654204,46.0843574704553));
#33078=CARTESIAN_POINT('Ctrl Pts',(43.7209657534595,39.2987391255556,46.040142882992));
#33079=CARTESIAN_POINT('Ctrl Pts',(43.655443176918,39.3029635466751,45.9959799289997));
#33080=CARTESIAN_POINT('Ctrl Pts',(43.5876297596427,39.3071879677946,45.95505674628));
#33081=CARTESIAN_POINT('Ctrl Pts',(43.5178807313047,39.3114123889141,45.9176136017834));
#33082=CARTESIAN_POINT('Ctrl Pts',(43.448176306152,39.3156341085962,45.8801944014699));
#33083=CARTESIAN_POINT('Ctrl Pts',(43.3765391390938,39.3198558282782,45.8462510437949));
#33084=CARTESIAN_POINT('Ctrl Pts',(43.3033514685189,39.3240775479602,45.8159792663015));
#33085=CARTESIAN_POINT('Ctrl Pts',(43.2301877446238,39.3282978863144,45.785717393599));
#33086=CARTESIAN_POINT('Ctrl Pts',(43.1554749579643,39.3325182246685,45.7591248949027));
#33087=CARTESIAN_POINT('Ctrl Pts',(43.0796164937853,39.3367385630227,45.7363498807733));
#33088=CARTESIAN_POINT('Ctrl Pts',(43.0037591611525,39.340958838424,45.7135752063685));
#33089=CARTESIAN_POINT('Ctrl Pts',(42.9267566348827,39.3451791138253,45.6946180370235));
#33090=CARTESIAN_POINT('Ctrl Pts',(42.8490272300439,39.3493993892265,45.679576549942));
#33091=CARTESIAN_POINT('Ctrl Pts',(42.7712200776924,39.3536238858864,45.6645200178693));
#33092=CARTESIAN_POINT('Ctrl Pts',(42.6926850563059,39.3578483825462,45.6533870813348));
#33093=CARTESIAN_POINT('Ctrl Pts',(42.6138498481755,39.3620728792061,45.6462245894446));
#33094=CARTESIAN_POINT('Ctrl Pts',(42.5349767914677,39.3662994040357,45.6390586588607));
#33095=CARTESIAN_POINT('Ctrl Pts',(42.4558037305286,39.3705259288654,45.6358669892364));
#33096=CARTESIAN_POINT('Ctrl Pts',(42.3767600472215,39.374752453695,45.6366442617552));
#33097=CARTESIAN_POINT('Ctrl Pts',(42.2975718747112,39.3789867044704,45.6374229551021));
#33098=CARTESIAN_POINT('Ctrl Pts',(42.2185140221459,39.3832209552457,45.6421850596758));
#33099=CARTESIAN_POINT('Ctrl Pts',(42.1400122475599,39.387455206021,45.6508731814819));
#33100=CARTESIAN_POINT('Ctrl Pts',(42.0651422262749,39.3914935662664,45.6591593618641));
#33101=CARTESIAN_POINT('Ctrl Pts',(41.9907783157044,39.3955319265117,45.6710162390806));
#33102=CARTESIAN_POINT('Ctrl Pts',(41.9172790332476,39.399570286757,45.6863511698709));
#33103=CARTESIAN_POINT('Ctrl Pts',(41.8401917474427,39.4038057870233,45.7024347036568));
#33104=CARTESIAN_POINT('Ctrl Pts',(41.7637626367544,39.4080412872895,45.7224056736516));
#33105=CARTESIAN_POINT('Ctrl Pts',(41.6884134242154,39.4122767875558,45.7461954419109));
#33106=CARTESIAN_POINT('Ctrl Pts',(41.6131734441177,39.416506147691,45.7699507225575));
#33107=CARTESIAN_POINT('Ctrl Pts',(41.5390106971314,39.4207355078263,45.7975136677444));
#33108=CARTESIAN_POINT('Ctrl Pts',(41.4663363885392,39.4249648679616,45.8287647060869));
#33109=CARTESIAN_POINT('Ctrl Pts',(41.3937469484722,39.4291892890811,45.8599792496957));
#33110=CARTESIAN_POINT('Ctrl Pts',(41.322642921634,39.4334137102005,45.894873143343));
#33111=CARTESIAN_POINT('Ctrl Pts',(41.2534185555025,39.43763813132,45.9332776112806));
#33112=CARTESIAN_POINT('Ctrl Pts',(41.1842384570446,39.4418598510021,45.9716575202869));
#33113=CARTESIAN_POINT('Ctrl Pts',(41.1169360428785,39.4460815706841,46.0135433207662));
#33114=CARTESIAN_POINT('Ctrl Pts',(41.0518827214868,39.4503032903661,46.0587194318507));
#33115=CARTESIAN_POINT('Ctrl Pts',(40.9868506852523,39.4545236287203,46.1038807615127));
#33116=CARTESIAN_POINT('Ctrl Pts',(40.9240666657714,39.4587439670744,46.1523299965446));
#33117=CARTESIAN_POINT('Ctrl Pts',(40.8638734561672,39.4629643054286,46.2038080051864));
#33118=CARTESIAN_POINT('Ctrl Pts',(40.8036811444376,39.4671845808299,46.2552852459544));
#33119=CARTESIAN_POINT('Ctrl Pts',(40.746079921596,39.4714048562312,46.3097908644601));
#33120=CARTESIAN_POINT('Ctrl Pts',(40.6913786623178,39.4756251316324,46.3670261590224));
#33121=CARTESIAN_POINT('Ctrl Pts',(40.6366226890372,39.4798496282923,46.4243187022127));
#33122=CARTESIAN_POINT('Ctrl Pts',(40.5847727987724,39.4840741249521,46.4843460354835));
#33123=CARTESIAN_POINT('Ctrl Pts',(40.5360997654162,39.488298621612,46.5467738109921));
#33124=CARTESIAN_POINT('Ctrl Pts',(40.487403364264,39.4925251464416,46.6092315579124));
#33125=CARTESIAN_POINT('Ctrl Pts',(40.4418871283864,39.4967516712713,46.6740916581663));
#33126=CARTESIAN_POINT('Ctrl Pts',(40.399778876443,39.5009781961009,46.7409901121213));
#33127=CARTESIAN_POINT('Ctrl Pts',(40.3575936520267,39.5052124468762,46.8080108542076));
#33128=CARTESIAN_POINT('Ctrl Pts',(40.3188290902334,39.5094466976516,46.8770769851343));
#33129=CARTESIAN_POINT('Ctrl Pts',(40.2836672525762,39.5136809484269,46.9477993807826));
#33130=CARTESIAN_POINT('Ctrl Pts',(40.2501321185274,39.5177193086722,47.0152499230846));
#33131=CARTESIAN_POINT('Ctrl Pts',(40.2198738423221,39.5217576689175,47.0842065286689));
#33132=CARTESIAN_POINT('Ctrl Pts',(40.19300846324,39.5257960291628,47.154317555125));
#33133=CARTESIAN_POINT('Ctrl Pts',(40.1608768226732,39.5306260053,47.2381720317349));
#33134=CARTESIAN_POINT('Ctrl Pts',(40.1334962853768,39.5354559814371,47.3239427193908));
#33135=CARTESIAN_POINT('Ctrl Pts',(40.1110689014416,39.5402859575742,47.4111155741981));
#33136=CARTESIAN_POINT('Ctrl Pts',(40.088734546621,39.5450958989001,47.4979268347359));
#33137=CARTESIAN_POINT('Ctrl Pts',(40.0713124680133,39.5499058402259,47.5861284659829));
#33138=CARTESIAN_POINT('Ctrl Pts',(40.0589554590699,39.5547157815518,47.6751909818351));
#33139=CARTESIAN_POINT('Ctrl Pts',(40.0466851433725,39.5594919777029,47.7636286605089));
#33140=CARTESIAN_POINT('Ctrl Pts',(40.0394091884403,39.5642681738539,47.8529149815301));
#33141=CARTESIAN_POINT('Ctrl Pts',(40.0372292376017,39.569044370005,47.9425129122682));
#33142=CARTESIAN_POINT('Ctrl Pts',(40.036776046103,39.5700372967507,47.9611394885191));
#33143=CARTESIAN_POINT('Ctrl Pts',(40.0365429267318,39.5710302234965,47.9797794737281));
#33144=CARTESIAN_POINT('Ctrl Pts',(40.036530522818,39.5720231502423,47.9984279538409));
#33145=CARTESIAN_POINT('',(40.0365306476135,40.3657731503002,48.001749637055));
#33146=CARTESIAN_POINT('Ctrl Pts',(40.0365305228177,39.5720231502717,47.998427954393));
#33147=CARTESIAN_POINT('Ctrl Pts',(40.036477506972,39.5762670422148,48.0781338690935));
#33148=CARTESIAN_POINT('Ctrl Pts',(40.0404608398097,39.580510934158,48.1578629671102));
#33149=CARTESIAN_POINT('Ctrl Pts',(40.0484609932266,39.5847548261011,48.2371808182024));
#33150=CARTESIAN_POINT('Ctrl Pts',(40.056461639913,39.588998979712,48.3165035598345));
#33151=CARTESIAN_POINT('Ctrl Pts',(40.0684795521282,39.5932431333228,48.3954145447556));
#33152=CARTESIAN_POINT('Ctrl Pts',(40.0844433687405,39.5974872869337,48.473484876559));
#33153=CARTESIAN_POINT('Ctrl Pts',(40.1004129449128,39.601732971786,48.5515833752332));
#33154=CARTESIAN_POINT('Ctrl Pts',(40.1203311600012,39.6059786566383,48.6288401662839));
#33155=CARTESIAN_POINT('Ctrl Pts',(40.1440759360515,39.6102243414906,48.704838320892));
#33156=CARTESIAN_POINT('Ctrl Pts',(40.1678524071262,39.614475693572,48.780937919429));
#33157=CARTESIAN_POINT('Ctrl Pts',(40.1954654925946,39.6187270456533,48.8557750881277));
#33158=CARTESIAN_POINT('Ctrl Pts',(40.226743968526,39.6229783977347,48.9289503014488));
#33159=CARTESIAN_POINT('Ctrl Pts',(40.258047098849,39.6272331008265,49.0021831931035));
#33160=CARTESIAN_POINT('Ctrl Pts',(40.2930211668911,39.6314878039184,49.0737511082556));
#33161=CARTESIAN_POINT('Ctrl Pts',(40.3314488740314,39.6357425070102,49.1432789161679));
#33162=CARTESIAN_POINT('Ctrl Pts',(40.3699442393029,39.640004701188,49.2129291389184));
#33163=CARTESIAN_POINT('Ctrl Pts',(40.4119051337497,39.6442668953659,49.2805316962437));
#33164=CARTESIAN_POINT('Ctrl Pts',(40.4570711621342,39.6485290895437,49.3457406778015));
#33165=CARTESIAN_POINT('Ctrl Pts',(40.4694083581805,39.6496933168854,49.3635526488388));
#33166=CARTESIAN_POINT('Ctrl Pts',(40.4819844690065,39.650857544227,49.3811862268741));
#33167=CARTESIAN_POINT('Ctrl Pts',(40.494793690343,39.6520217715687,49.3986348195806));
#33168=CARTESIAN_POINT('Ctrl Pts',(40.5413940908316,39.656257271835,49.462113417282));
#33169=CARTESIAN_POINT('Ctrl Pts',(40.5912590564143,39.6604927721012,49.5233811397024));
#33170=CARTESIAN_POINT('Ctrl Pts',(40.6441512579066,39.6647282723675,49.582082689302));
#33171=CARTESIAN_POINT('Ctrl Pts',(40.6969667824954,39.6689576325027,49.6406991402873));
#33172=CARTESIAN_POINT('Ctrl Pts',(40.7528005166242,39.673186992638,49.696756460248));
#33173=CARTESIAN_POINT('Ctrl Pts',(40.8113731440476,39.6774163527732,49.7499300424437));
#33174=CARTESIAN_POINT('Ctrl Pts',(40.869877370786,39.6816407738927,49.8030415289198));
#33175=CARTESIAN_POINT('Ctrl Pts',(40.9311137891788,39.6858651950122,49.8532756558546));
#33176=CARTESIAN_POINT('Ctrl Pts',(40.9947653397528,39.6900896161317,49.9003436506432));
#33177=CARTESIAN_POINT('Ctrl Pts',(41.0583761863633,39.6943113358138,49.9473815463388));
#33178=CARTESIAN_POINT('Ctrl Pts',(41.1243987234273,39.6985330554958,49.9912570501427));
#33179=CARTESIAN_POINT('Ctrl Pts',(41.1924827701755,39.7027547751778,50.0317215804772));
#33180=CARTESIAN_POINT('Ctrl Pts',(41.2605445401268,39.706975113532,50.0721728709977));
#33181=CARTESIAN_POINT('Ctrl Pts',(41.33066607723,39.7111954518861,50.1092151645504));
#33182=CARTESIAN_POINT('Ctrl Pts',(41.4024694359028,39.7154157902403,50.1426439775642));
#33183=CARTESIAN_POINT('Ctrl Pts',(41.4742717235175,39.7196360656416,50.1760722919354));
#33184=CARTESIAN_POINT('Ctrl Pts',(41.5477553567728,39.7238563410429,50.2058870360244));
#33185=CARTESIAN_POINT('Ctrl Pts',(41.6225204468284,39.7280766164441,50.2319309992247));
#33186=CARTESIAN_POINT('Ctrl Pts',(41.6973603193916,39.732301113104,50.2580010124554));
#33187=CARTESIAN_POINT('Ctrl Pts',(41.7734837649345,39.7365256097638,50.280292555667));
#33188=CARTESIAN_POINT('Ctrl Pts',(41.8504742561262,39.7407501064237,50.2986978700386));
#33189=CARTESIAN_POINT('Ctrl Pts',(41.9275017102515,39.7449766312533,50.3171120207535));
#33190=CARTESIAN_POINT('Ctrl Pts',(42.0053965772456,39.749203156083,50.3316361396397));
#33191=CARTESIAN_POINT('Ctrl Pts',(42.0837331589628,39.7534296809126,50.3422138515004));
#33192=CARTESIAN_POINT('Ctrl Pts',(42.1622129373251,39.757663931688,50.3528108990638));
#33193=CARTESIAN_POINT('Ctrl Pts',(42.2411355749332,39.7618981824633,50.3594470851074));
#33194=CARTESIAN_POINT('Ctrl Pts',(42.3200714844046,39.7661324332387,50.3621180904635));
#33195=CARTESIAN_POINT('Ctrl Pts',(42.3953555560499,39.770170793484,50.3646655262241));
#33196=CARTESIAN_POINT('Ctrl Pts',(42.4706513420945,39.7742091537293,50.363606594462));
#33197=CARTESIAN_POINT('Ctrl Pts',(42.5455907392309,39.7782475139745,50.3589815127614));
#33198=CARTESIAN_POINT('Ctrl Pts',(42.6241884415766,39.7824830142408,50.3541306491474));
#33199=CARTESIAN_POINT('Ctrl Pts',(42.7026928376915,39.786718514507,50.3453381299536));
#33200=CARTESIAN_POINT('Ctrl Pts',(42.7806767193037,39.7909540147733,50.3326113427402));
#33201=CARTESIAN_POINT('Ctrl Pts',(42.8585475490406,39.7951833749086,50.3199030053286));
#33202=CARTESIAN_POINT('Ctrl Pts',(42.9358989034339,39.7994127350438,50.3032718008792));
#33203=CARTESIAN_POINT('Ctrl Pts',(43.0123066713929,39.8036420951791,50.2827770327099));
#33204=CARTESIAN_POINT('Ctrl Pts',(43.0886252109205,39.8078665162986,50.2623061981807));
#33205=CARTESIAN_POINT('Ctrl Pts',(43.1640019027486,39.812090937418,50.2379808867639));
#33206=CARTESIAN_POINT('Ctrl Pts',(43.238022354535,39.8163153585375,50.2099115308536));
#33207=CARTESIAN_POINT('Ctrl Pts',(43.3119954716417,39.8205370782196,50.1818601247658));
#33208=CARTESIAN_POINT('Ctrl Pts',(43.3846136324202,39.8247587979016,50.15006959222));
#33209=CARTESIAN_POINT('Ctrl Pts',(43.4554783279712,39.8289805175836,50.1146999645536));
#33210=CARTESIAN_POINT('Ctrl Pts',(43.5263198369095,39.8332008559378,50.0793419096719));
#33211=CARTESIAN_POINT('Ctrl Pts',(43.5954086002184,39.837421194292,50.0404072944587));
#33212=CARTESIAN_POINT('Ctrl Pts',(43.6623681761319,39.8416415326461,49.9981033578845));
#33213=CARTESIAN_POINT('Ctrl Pts',(43.7293267532398,39.8458618080474,49.955800052339));
#33214=CARTESIAN_POINT('Ctrl Pts',(43.7941558100022,39.8500820834487,49.9101277771519));
#33215=CARTESIAN_POINT('Ctrl Pts',(43.8565067914275,39.8543023588499,49.8613378004611));
#33216=CARTESIAN_POINT('Ctrl Pts',(43.9189201383598,39.8585268555098,49.8124990224274));
#33217=CARTESIAN_POINT('Ctrl Pts',(43.9788500880155,39.8627513521696,49.7605366033697));
#33218=CARTESIAN_POINT('Ctrl Pts',(44.0359806744609,39.8669758488295,49.7057425578588));
#33219=CARTESIAN_POINT('Ctrl Pts',(44.0931386891514,39.8712023736591,49.6509222058699));
#33220=CARTESIAN_POINT('Ctrl Pts',(44.1474943408743,39.8754288984888,49.5932678612009));
#33221=CARTESIAN_POINT('Ctrl Pts',(44.1987699174329,39.8796554233184,49.5331070494386));
#33222=CARTESIAN_POINT('Ctrl Pts',(44.2501392240265,39.8838896740938,49.4728362657293));
#33223=CARTESIAN_POINT('Ctrl Pts',(44.2984169179976,39.8881239248691,49.4100502325925));
#33224=CARTESIAN_POINT('Ctrl Pts',(44.3433669636869,39.8923581756444,49.345107908441));
#33225=CARTESIAN_POINT('Ctrl Pts',(44.3862374706948,39.8963965358898,49.2831700322952));
#33226=CARTESIAN_POINT('Ctrl Pts',(44.4260812587883,39.9004348961351,49.2192712898739));
#33227=CARTESIAN_POINT('Ctrl Pts',(44.4627330113282,39.9044732563804,49.1537430237608));
#33228=CARTESIAN_POINT('Ctrl Pts',(44.5011739869249,39.9087087566467,49.0850158741981));
#33229=CARTESIAN_POINT('Ctrl Pts',(44.5362494416739,39.912944256913,49.0142347956722));
#33230=CARTESIAN_POINT('Ctrl Pts',(44.5677344726814,39.9171797571792,48.9417630789369));
#33231=CARTESIAN_POINT('Ctrl Pts',(44.5991738603877,39.9214091173145,48.8693964231874));
#33232=CARTESIAN_POINT('Ctrl Pts',(44.6270329750745,39.9256384774498,48.7953444231009));
#33233=CARTESIAN_POINT('Ctrl Pts',(44.651132252006,39.929867837585,48.7199958505982));
#33234=CARTESIAN_POINT('Ctrl Pts',(44.6752033859784,39.9340922587045,48.6447352696063));
#33235=CARTESIAN_POINT('Ctrl Pts',(44.6955232651173,39.938316679824,48.5681815697724));
#33236=CARTESIAN_POINT('Ctrl Pts',(44.7119605834352,39.9425411009435,48.4907430096722));
#33237=CARTESIAN_POINT('Ctrl Pts',(44.7283873903987,39.9467628206255,48.4133539700674));
#33238=CARTESIAN_POINT('Ctrl Pts',(44.7409364672251,39.9509845403076,48.3350816511724));
#33239=CARTESIAN_POINT('Ctrl Pts',(44.7495268148379,39.9552062599896,48.2563477857479));
#33240=CARTESIAN_POINT('Ctrl Pts',(44.7581143517271,39.9594265983437,48.1776396816935));
#33241=CARTESIAN_POINT('Ctrl Pts',(44.762745680528,39.9636469366979,48.0984707972066));
#33242=CARTESIAN_POINT('Ctrl Pts',(44.7633914432395,39.9678672750521,48.0192698448972));
#33243=CARTESIAN_POINT('Ctrl Pts',(44.7640371963184,39.9720875504533,47.9400700739924));
#33244=CARTESIAN_POINT('Ctrl Pts',(44.7606974989907,39.9763078258546,47.8608387055626));
#33245=CARTESIAN_POINT('Ctrl Pts',(44.7533951095284,39.9805281012559,47.7820048180627));
#33246=CARTESIAN_POINT('Ctrl Pts',(44.7460854159755,39.9847525979158,47.70309207831));
#33247=CARTESIAN_POINT('Ctrl Pts',(44.7348051558609,39.9889770945756,47.6245780821575));
#33248=CARTESIAN_POINT('Ctrl Pts',(44.7196289867533,39.9932015912355,47.5468865432213));
#33249=CARTESIAN_POINT('Ctrl Pts',(44.7044455316066,39.9974281160651,47.4691577047805));
#33250=CARTESIAN_POINT('Ctrl Pts',(44.6853625545606,40.0016546408947,47.3922525663273));
#33251=CARTESIAN_POINT('Ctrl Pts',(44.6625052738913,40.0058811657244,47.3165818801686));
#33252=CARTESIAN_POINT('Ctrl Pts',(44.6396062108793,40.0101154164997,47.2407728705324));
#33253=CARTESIAN_POINT('Ctrl Pts',(44.6129192163879,40.0143496672751,47.1662032653489));
#33254=CARTESIAN_POINT('Ctrl Pts',(44.582618491234,40.0185839180504,47.0932657706783));
#33255=CARTESIAN_POINT('Ctrl Pts',(44.5537195784492,40.0226222782957,47.0237026072055));
#33256=CARTESIAN_POINT('Ctrl Pts',(44.5215340929191,40.026660638541,46.9556241873224));
#33257=CARTESIAN_POINT('Ctrl Pts',(44.4862512681615,40.0306989987863,46.8893488004803));
#33258=CARTESIAN_POINT('Ctrl Pts',(44.4492460470873,40.0349344990526,46.8198380581086));
#33259=CARTESIAN_POINT('Ctrl Pts',(44.408692695973,40.0391699993188,46.7520466551394));
#33260=CARTESIAN_POINT('Ctrl Pts',(44.3647750819876,40.043405499585,46.6863602784246));
#33261=CARTESIAN_POINT('Ctrl Pts',(44.3209211346025,40.0476348597203,46.6207691261064));
#33262=CARTESIAN_POINT('Ctrl Pts',(44.2737128680956,40.0518642198556,46.5572773269405));
#33263=CARTESIAN_POINT('Ctrl Pts',(44.2233801075699,40.0560935799908,46.4962462222097));
#33264=CARTESIAN_POINT('Ctrl Pts',(44.173106125273,40.0603180011103,46.4352863891558));
#33265=CARTESIAN_POINT('Ctrl Pts',(44.1197151967979,40.0645424222298,46.3767819004132));
#33266=CARTESIAN_POINT('Ctrl Pts',(44.0634796436432,40.0687668433493,46.3210640524175));
#33267=CARTESIAN_POINT('Ctrl Pts',(44.0072800520618,40.0729885630313,46.2653818349325));
#33268=CARTESIAN_POINT('Ctrl Pts',(43.9482397788051,40.0772102827133,46.2124830507483));
#33269=CARTESIAN_POINT('Ctrl Pts',(43.8866696931503,40.0814320023954,46.1626639761959));
#33270=CARTESIAN_POINT('Ctrl Pts',(43.8251197529534,40.0856523407495,46.1128612022228));
#33271=CARTESIAN_POINT('Ctrl Pts',(43.7610420085747,40.0898726791037,46.0661364319965));
#33272=CARTESIAN_POINT('Ctrl Pts',(43.6947811369232,40.0940930174578,46.0227462862931));
#33273=CARTESIAN_POINT('Ctrl Pts',(43.628521253655,40.0983132928591,45.9793567878207));
#33274=CARTESIAN_POINT('Ctrl Pts',(43.5600787012306,40.1025335682604,45.9393020710057));
#33275=CARTESIAN_POINT('Ctrl Pts',(43.4898266587049,40.1067538436617,45.9027951232948));
#33276=CARTESIAN_POINT('Ctrl Pts',(43.4195043477707,40.1109783403215,45.8662516601315));
#33277=CARTESIAN_POINT('Ctrl Pts',(43.3473693486783,40.1152028369814,45.8332632717804));
#33278=CARTESIAN_POINT('Ctrl Pts',(43.2738184055801,40.1194273336412,45.803996394591));
#33279=CARTESIAN_POINT('Ctrl Pts',(43.2002321508665,40.1236538584708,45.7747154664504));
#33280=CARTESIAN_POINT('Ctrl Pts',(43.1252290428012,40.1278803833005,45.7491597603559));
#33281=CARTESIAN_POINT('Ctrl Pts',(43.0492222776242,40.1321069081301,45.7274461777251));
#33282=CARTESIAN_POINT('Ctrl Pts',(42.9730765746287,40.1363411589055,45.7056929033931));
#33283=CARTESIAN_POINT('Ctrl Pts',(42.8959240068713,40.1405754096808,45.6877958930098));
#33284=CARTESIAN_POINT('Ctrl Pts',(42.8181890923301,40.1448096604561,45.6738210894353));
#33285=CARTESIAN_POINT('Ctrl Pts',(42.7440504535926,40.1488480207015,45.6604928067742));
#33286=CARTESIAN_POINT('Ctrl Pts',(42.6693825180014,40.1528863809468,45.6507318576801));
#33287=CARTESIAN_POINT('Ctrl Pts',(42.5945553496412,40.1569247411921,45.6445512833377));
#33288=CARTESIAN_POINT('Ctrl Pts',(42.5160753547276,40.1611602414584,45.6380689928331));
#33289=CARTESIAN_POINT('Ctrl Pts',(42.4371218643529,40.1653957417246,45.6355009272594));
#33290=CARTESIAN_POINT('Ctrl Pts',(42.358118722558,40.1696312419909,45.6369011024716));
#33291=CARTESIAN_POINT('Ctrl Pts',(42.2792301102423,40.1738606021261,45.6382992478742));
#33292=CARTESIAN_POINT('Ctrl Pts',(42.200292454752,40.1780899622614,45.6436542019903));
#33293=CARTESIAN_POINT('Ctrl Pts',(42.1217339876723,40.1823193223966,45.6529681580168));
#33294=CARTESIAN_POINT('Ctrl Pts',(42.0432672605946,40.1865437435161,45.6622712372736));
#33295=CARTESIAN_POINT('Ctrl Pts',(41.9651793056406,40.1907681646356,45.6755240761237));
#33296=CARTESIAN_POINT('Ctrl Pts',(41.8878960760243,40.1949925857551,45.6926768730954));
#33297=CARTESIAN_POINT('Ctrl Pts',(41.8106622675724,40.1992143054372,45.7098187011778));
#33298=CARTESIAN_POINT('Ctrl Pts',(41.7342326200377,40.2034360251192,45.7308554360035));
#33299=CARTESIAN_POINT('Ctrl Pts',(41.6590244877631,40.2076577448012,45.7556859107591));
#33300=CARTESIAN_POINT('Ctrl Pts',(41.5838409632544,40.2118780831554,45.780508261094));
#33301=CARTESIAN_POINT('Ctrl Pts',(41.5098786057367,40.2160984215096,45.8091217395229));
#33302=CARTESIAN_POINT('Ctrl Pts',(41.4375397077592,40.2203187598637,45.8413752927478));
#33303=CARTESIAN_POINT('Ctrl Pts',(41.3652018888285,40.224539035265,45.8736283648609));
#33304=CARTESIAN_POINT('Ctrl Pts',(41.2944879094299,40.2287593106663,45.9095212114892));
#33305=CARTESIAN_POINT('Ctrl Pts',(41.2257787846763,40.2329795860676,45.9488552029699));
#33306=CARTESIAN_POINT('Ctrl Pts',(41.1570009347914,40.2372040827274,45.9882285376053));
#33307=CARTESIAN_POINT('Ctrl Pts',(41.0902323537357,40.2414285793873,46.0310496590746));
#33308=CARTESIAN_POINT('Ctrl Pts',(41.0258276543604,40.2456530760471,46.0770749350588));
#33309=CARTESIAN_POINT('Ctrl Pts',(40.9613920344571,40.2498796008768,46.1231223076577));
#33310=CARTESIAN_POINT('Ctrl Pts',(40.8993229252437,40.2541061257064,46.172376607114));
#33311=CARTESIAN_POINT('Ctrl Pts',(40.8399421797426,40.2583326505361,46.2245535664646));
#33312=CARTESIAN_POINT('Ctrl Pts',(40.7804528882295,40.2625669013114,46.2768259035476));
#33313=CARTESIAN_POINT('Ctrl Pts',(40.7236621176619,40.2668011520868,46.3320312481309));
#33314=CARTESIAN_POINT('Ctrl Pts',(40.6698549884491,40.2710354028621,46.3898482432064));
#33315=CARTESIAN_POINT('Ctrl Pts',(40.6185371560732,40.2750737631074,46.4449904317077));
#33316=CARTESIAN_POINT('Ctrl Pts',(40.5699332062563,40.2791121233527,46.5025076708174));
#33317=CARTESIAN_POINT('Ctrl Pts',(40.5242543085212,40.283150483598,46.562095781424));
#33318=CARTESIAN_POINT('Ctrl Pts',(40.4762651280949,40.2873930903168,46.6246976552202));
#33319=CARTESIAN_POINT('Ctrl Pts',(40.4313198957796,40.2916356970356,46.6898264207477));
#33320=CARTESIAN_POINT('Ctrl Pts',(40.3896950661176,40.2958783037544,46.7571546702393));
#33321=CARTESIAN_POINT('Ctrl Pts',(40.3481300765327,40.3001148112792,46.8243861282804));
#33322=CARTESIAN_POINT('Ctrl Pts',(40.3098762568635,40.3043513188039,46.8938104002843));
#33323=CARTESIAN_POINT('Ctrl Pts',(40.2751690774718,40.3085878263287,46.9650681222574));
#33324=CARTESIAN_POINT('Ctrl Pts',(40.2405010940688,40.3128195494226,47.0362453704808));
#33325=CARTESIAN_POINT('Ctrl Pts',(40.2093720001794,40.3170512725164,47.1092515396943));
#33326=CARTESIAN_POINT('Ctrl Pts',(40.1819725145746,40.3212829956103,47.1837007198352));
#33327=CARTESIAN_POINT('Ctrl Pts',(40.154595210532,40.3255112928651,47.2580896288038));
#33328=CARTESIAN_POINT('Ctrl Pts',(40.1309416771006,40.3297395901198,47.3339187912001));
#33329=CARTESIAN_POINT('Ctrl Pts',(40.1111548526966,40.3339678873746,47.4107815917966));
#33330=CARTESIAN_POINT('Ctrl Pts',(40.0913774547657,40.3381941702622,47.4876077748389));
#33331=CARTESIAN_POINT('Ctrl Pts',(40.0754632205032,40.3424204531497,47.5654661658495));
#33332=CARTESIAN_POINT('Ctrl Pts',(40.0635050627558,40.3466467360373,47.6439356109743));
#33333=CARTESIAN_POINT('Ctrl Pts',(40.0515462945462,40.350873234676,47.7224090619528));
#33334=CARTESIAN_POINT('Ctrl Pts',(40.0435440831736,40.3550997333147,47.8014931688741));
#33335=CARTESIAN_POINT('Ctrl Pts',(40.0395399008274,40.3593262319534,47.8807583918517));
#33336=CARTESIAN_POINT('Ctrl Pts',(40.0375039652753,40.3614752047262,47.9210609733895));
#33337=CARTESIAN_POINT('Ctrl Pts',(40.0365007850733,40.3636241774989,47.9614102878016));
#33338=CARTESIAN_POINT('Ctrl Pts',(40.0365306476131,40.3657731502717,48.0017496365208));
#33339=CARTESIAN_POINT('',(40.0365301409399,41.1595231502254,48.0008162196351));
#33340=CARTESIAN_POINT('Ctrl Pts',(40.0365306476135,40.3657731503002,48.001749637055));
#33341=CARTESIAN_POINT('Ctrl Pts',(40.0365982547737,40.37063830587,48.0930756927361));
#33342=CARTESIAN_POINT('Ctrl Pts',(40.0419631966318,40.3755034614398,48.1841861615192));
#33343=CARTESIAN_POINT('Ctrl Pts',(40.052526975406,40.3803686170097,48.2745192884));
#33344=CARTESIAN_POINT('Ctrl Pts',(40.063191471508,40.385280158014,48.3657136706464));
#33345=CARTESIAN_POINT('Ctrl Pts',(40.0791543076126,40.3901916990183,48.4561156530629));
#33346=CARTESIAN_POINT('Ctrl Pts',(40.1002644889058,40.3951032400226,48.5451669651698));
#33347=CARTESIAN_POINT('Ctrl Pts',(40.1207132863672,40.3998609020164,48.631428291856));
#33348=CARTESIAN_POINT('Ctrl Pts',(40.1459915809743,40.4046185640101,48.7164222519164));
#33349=CARTESIAN_POINT('Ctrl Pts',(40.1759197402339,40.4093762260039,48.7996608274879));
#33350=CARTESIAN_POINT('Ctrl Pts',(40.2025632316544,40.4136117262702,48.8737638237618));
#33351=CARTESIAN_POINT('Ctrl Pts',(40.2329649197856,40.4178472265364,48.9466746320274));
#33352=CARTESIAN_POINT('Ctrl Pts',(40.2669982082182,40.4220827268027,49.017985165489));
#33353=CARTESIAN_POINT('Ctrl Pts',(40.3009821591852,40.426312086938,49.0891923213119));
#33354=CARTESIAN_POINT('Ctrl Pts',(40.3385870553058,40.4305414470732,49.1588033892228));
#33355=CARTESIAN_POINT('Ctrl Pts',(40.3796373233663,40.4347708072085,49.2264277784547));
#33356=CARTESIAN_POINT('Ctrl Pts',(40.4206396532244,40.438995228328,49.2939731964204));
#33357=CARTESIAN_POINT('Ctrl Pts',(40.4650791173327,40.4432196494475,49.3595361469052));
#33358=CARTESIAN_POINT('Ctrl Pts',(40.5127337732114,40.447444070567,49.4227496723328));
#33359=CARTESIAN_POINT('Ctrl Pts',(40.5603579548384,40.451665790249,49.4859227739057));
#33360=CARTESIAN_POINT('Ctrl Pts',(40.611192965633,40.4558875099311,49.5467490586181));
#33361=CARTESIAN_POINT('Ctrl Pts',(40.6649736873588,40.4601092296131,49.6048906926463));
#33362=CARTESIAN_POINT('Ctrl Pts',(40.718736812272,40.4643295679673,49.6630133029908));
#33363=CARTESIAN_POINT('Ctrl Pts',(40.7754434158152,40.4685499063214,49.7184526625828));
#33364=CARTESIAN_POINT('Ctrl Pts',(40.834789229615,40.4727702446756,49.7709053292514));
#33365=CARTESIAN_POINT('Ctrl Pts',(40.8941341581803,40.4769905200768,49.8233572135073));
#33366=CARTESIAN_POINT('Ctrl Pts',(40.9561178661875,40.4812107954781,49.8728221835688));
#33367=CARTESIAN_POINT('Ctrl Pts',(41.0204016146411,40.4854310708794,49.9190358871097));
#33368=CARTESIAN_POINT('Ctrl Pts',(41.0847496618188,40.4896555675393,49.9652958151203));
#33369=CARTESIAN_POINT('Ctrl Pts',(41.1514019631305,40.4938800641991,50.0082977056594));
#33370=CARTESIAN_POINT('Ctrl Pts',(41.219989776019,40.4981045608589,50.0478198925199));
#33371=CARTESIAN_POINT('Ctrl Pts',(41.288610517737,40.5023310856886,50.087361053879));
#33372=CARTESIAN_POINT('Ctrl Pts',(41.3591682036669,40.5065576105182,50.123418969649));
#33373=CARTESIAN_POINT('Ctrl Pts',(41.4312706986902,40.5107841353479,50.1558186337639));
#33374=CARTESIAN_POINT('Ctrl Pts',(41.5035049946572,40.5150183861232,50.1882775233787));
#33375=CARTESIAN_POINT('Ctrl Pts',(41.5772893040498,40.5192526368986,50.2170646277777));
#33376=CARTESIAN_POINT('Ctrl Pts',(41.6522129720365,40.5234868876739,50.2420537463918));
#33377=CARTESIAN_POINT('Ctrl Pts',(41.7236704218381,40.5275252479192,50.2658867852291));
#33378=CARTESIAN_POINT('Ctrl Pts',(41.796163786748,40.5315636081644,50.2862654205252));
#33379=CARTESIAN_POINT('Ctrl Pts',(41.869328707653,40.5356019684097,50.3031236224699));
#33380=CARTESIAN_POINT('Ctrl Pts',(41.94606530943,40.5398374686759,50.3208047887078));
#33381=CARTESIAN_POINT('Ctrl Pts',(42.0238324000669,40.5440729689422,50.3346802424668));
#33382=CARTESIAN_POINT('Ctrl Pts',(42.1022182795349,40.5483084692084,50.3446356833967));
#33383=CARTESIAN_POINT('Ctrl Pts',(42.1804905243584,40.5525378293437,50.3545766920972));
#33384=CARTESIAN_POINT('Ctrl Pts',(42.2593793149624,40.5567671894789,50.3606089143199));
#33385=CARTESIAN_POINT('Ctrl Pts',(42.3384611699351,40.5609965496142,50.3626687057847));
#33386=CARTESIAN_POINT('Ctrl Pts',(42.4174506736971,40.5652209707337,50.3647260918401));
#33387=CARTESIAN_POINT('Ctrl Pts',(42.4966323270434,40.5694453918532,50.3628202534882));
#33388=CARTESIAN_POINT('Ctrl Pts',(42.5755774393607,40.5736698129727,50.3569393296578));
#33389=CARTESIAN_POINT('Ctrl Pts',(42.6544720677708,40.5778915326547,50.3510621665669));
#33390=CARTESIAN_POINT('Ctrl Pts',(42.7331299885875,40.5821132523367,50.3412149980812));
#33391=CARTESIAN_POINT('Ctrl Pts',(42.8111236473736,40.5863349720188,50.327438030855));
#33392=CARTESIAN_POINT('Ctrl Pts',(42.8890917869819,40.5905553103729,50.3136655713911));
#33393=CARTESIAN_POINT('Ctrl Pts',(42.9663956342856,40.5947756487271,50.2959659479658));
#33394=CARTESIAN_POINT('Ctrl Pts',(43.042615379302,40.5989959870812,50.2744308991888));
#33395=CARTESIAN_POINT('Ctrl Pts',(43.118833987383,40.6032162624825,50.2528961716403));
#33396=CARTESIAN_POINT('Ctrl Pts',(43.1939680740145,40.6074365378838,50.2275262613617));
#33397=CARTESIAN_POINT('Ctrl Pts',(43.2676120565571,40.6116568132851,50.1984630449968));
#33398=CARTESIAN_POINT('Ctrl Pts',(43.3413297002385,40.6158813099449,50.169370758645));
#33399=CARTESIAN_POINT('Ctrl Pts',(43.4135538248403,40.6201058066047,50.1365779593506));
#33400=CARTESIAN_POINT('Ctrl Pts',(43.4838985162758,40.6243303032646,50.100274850422));
#33401=CARTESIAN_POINT('Ctrl Pts',(43.5542769800138,40.6285568280942,50.0639543124657));
#33402=CARTESIAN_POINT('Ctrl Pts',(43.6227738067827,40.6327833529239,50.0241203438456));
#33403=CARTESIAN_POINT('Ctrl Pts',(43.6890296698075,40.6370098777535,49.9810080644096));
#33404=CARTESIAN_POINT('Ctrl Pts',(43.7554066463287,40.6412441285289,49.9378169771722));
#33405=CARTESIAN_POINT('Ctrl Pts',(43.819534092501,40.6454783793042,49.8913358805884));
#33406=CARTESIAN_POINT('Ctrl Pts',(43.8810837093347,40.6497126300795,49.8418418734634));
#33407=CARTESIAN_POINT('Ctrl Pts',(43.9397858360921,40.6537509903249,49.7946376237956));
#33408=CARTESIAN_POINT('Ctrl Pts',(43.9961431337756,40.6577893505702,49.744693337531));
#33409=CARTESIAN_POINT('Ctrl Pts',(44.0499029542822,40.6618277108155,49.6922797293447));
#33410=CARTESIAN_POINT('Ctrl Pts',(44.1062871598103,40.6660632110818,49.6373074539799));
#33411=CARTESIAN_POINT('Ctrl Pts',(44.1600281400338,40.670298711348,49.5794096505003));
#33412=CARTESIAN_POINT('Ctrl Pts',(44.2108070389384,40.6745342116143,49.5188707346681));
#33413=CARTESIAN_POINT('Ctrl Pts',(44.2615123245573,40.6787635717495,49.4584195810482));
#33414=CARTESIAN_POINT('Ctrl Pts',(44.3092637570627,40.6829929318848,49.3953352749048));
#33415=CARTESIAN_POINT('Ctrl Pts',(44.3537787099889,40.68722229202,49.3299395449772));
#33416=CARTESIAN_POINT('Ctrl Pts',(44.3982416786794,40.6914467131395,49.2646201837036));
#33417=CARTESIAN_POINT('Ctrl Pts',(44.4394754156993,40.695671134259,49.1969951485624));
#33418=CARTESIAN_POINT('Ctrl Pts',(44.4772380275817,40.6998955553785,49.1274185636526));
#33419=CARTESIAN_POINT('Ctrl Pts',(44.5149764909875,40.7041172750605,49.0578864716538));
#33420=CARTESIAN_POINT('Ctrl Pts',(44.5492480116388,40.7083389947426,48.9864057182537));
#33421=CARTESIAN_POINT('Ctrl Pts',(44.5798551011486,40.7125607144246,48.9133576401917));
#33422=CARTESIAN_POINT('Ctrl Pts',(44.610452176155,40.7167810527787,48.8403334631356));
#33423=CARTESIAN_POINT('Ctrl Pts',(44.6373870195651,40.7210013911329,48.765743412272));
#33424=CARTESIAN_POINT('Ctrl Pts',(44.6605096724967,40.7252217294871,48.6899901893861));
#33425=CARTESIAN_POINT('Ctrl Pts',(44.6836319805181,40.7294420048883,48.6142380964766));
#33426=CARTESIAN_POINT('Ctrl Pts',(44.7029420753495,40.7336622802896,48.5373233153283));
#33427=CARTESIAN_POINT('Ctrl Pts',(44.7183398624741,40.7378825556909,48.4596637063808));
#33428=CARTESIAN_POINT('Ctrl Pts',(44.7337530509729,40.7421070523507,48.3819264197327));
#33429=CARTESIAN_POINT('Ctrl Pts',(44.7452460231156,40.7463315490106,48.3034432785405));
#33430=CARTESIAN_POINT('Ctrl Pts',(44.7527699689865,40.7505560456704,48.2246417457535));
#33431=CARTESIAN_POINT('Ctrl Pts',(44.7602975270842,40.7547825705001,48.1458023805566));
#33432=CARTESIAN_POINT('Ctrl Pts',(44.7638522417978,40.7590090953297,48.0666447887745));
#33433=CARTESIAN_POINT('Ctrl Pts',(44.7634374627916,40.7632356201594,47.9875983721466));
#33434=CARTESIAN_POINT('Ctrl Pts',(44.7630219255832,40.7674698709347,47.9084074613192));
#33435=CARTESIAN_POINT('Ctrl Pts',(44.758622421402,40.77170412171,47.8293286015956));
#33436=CARTESIAN_POINT('Ctrl Pts',(44.7502943911612,40.7759383724854,47.7507878097357));
#33437=CARTESIAN_POINT('Ctrl Pts',(44.7423516433102,40.7799767327307,47.675880576246));
#33438=CARTESIAN_POINT('Ctrl Pts',(44.7308359152055,40.784015092976,47.6014630733394));
#33439=CARTESIAN_POINT('Ctrl Pts',(44.7158382050134,40.7880534532213,47.5278942394968));
#33440=CARTESIAN_POINT('Ctrl Pts',(44.7001083538726,40.7922889534876,47.4507340070262));
#33441=CARTESIAN_POINT('Ctrl Pts',(44.6804880890839,40.7965244537538,47.3742141154112));
#33442=CARTESIAN_POINT('Ctrl Pts',(44.6570441138962,40.8007599540201,47.2987565980157));
#33443=CARTESIAN_POINT('Ctrl Pts',(44.6336341250311,40.8049893141553,47.2234084700693));
#33444=CARTESIAN_POINT('Ctrl Pts',(44.6064115715956,40.8092186742906,47.1491201023906));
#33445=CARTESIAN_POINT('Ctrl Pts',(44.5754941379767,40.8134480344259,47.0763032442792));
#33446=CARTESIAN_POINT('Ctrl Pts',(44.5446128095101,40.8176724555454,47.0035714211611));
#33447=CARTESIAN_POINT('Ctrl Pts',(44.5100453577583,40.8218968766648,46.9323081225715));
#33448=CARTESIAN_POINT('Ctrl Pts',(44.4719587487204,40.8261212977843,46.8629083658293));
#33449=CARTESIAN_POINT('Ctrl Pts',(44.4338964953491,40.8303430174664,46.7935529889197));
#33450=CARTESIAN_POINT('Ctrl Pts',(44.3923197765235,40.8345647371484,46.7260591989381));
#33451=CARTESIAN_POINT('Ctrl Pts',(44.3474424676075,40.8387864568304,46.6607993890911));
#33452=CARTESIAN_POINT('Ctrl Pts',(44.3025798423472,40.8430067951846,46.5955609319632));
#33453=CARTESIAN_POINT('Ctrl Pts',(44.254419037141,40.8472271335388,46.5325553899907));
#33454=CARTESIAN_POINT('Ctrl Pts',(44.2032176090137,40.8514474718929,46.4721267410407));
#33455=CARTESIAN_POINT('Ctrl Pts',(44.1520169446349,40.8556677472942,46.4116989934774));
#33456=CARTESIAN_POINT('Ctrl Pts',(44.0977760519236,40.8598880226955,46.3538484197605));
#33457=CARTESIAN_POINT('Ctrl Pts',(44.0407922129559,40.8641082980968,46.2988852611293));
#33458=CARTESIAN_POINT('Ctrl Pts',(43.9837513768743,40.8683327947566,46.2438671265351));
#33459=CARTESIAN_POINT('Ctrl Pts',(43.9239624525029,40.8725572914165,46.1917425029625));
#33460=CARTESIAN_POINT('Ctrl Pts',(43.8617585424306,40.8767817880763,46.142783694738));
#33461=CARTESIAN_POINT('Ctrl Pts',(43.7995247684237,40.881008312906,46.0938013815176));
#33462=CARTESIAN_POINT('Ctrl Pts',(43.7348740824683,40.8852348377356,46.0479881832126));
#33463=CARTESIAN_POINT('Ctrl Pts',(43.6681694356189,40.8894613625653,46.0055735853479));
#33464=CARTESIAN_POINT('Ctrl Pts',(43.6013428549113,40.8936956133406,45.9630814550202));
#33465=CARTESIAN_POINT('Ctrl Pts',(43.5324552201012,40.897929864116,45.9240005714261));
#33466=CARTESIAN_POINT('Ctrl Pts',(43.4618948163027,40.9021641148913,45.8885147786429));
#33467=CARTESIAN_POINT('Ctrl Pts',(43.3945987715684,40.9062024751366,45.8546706767102));
#33468=CARTESIAN_POINT('Ctrl Pts',(43.3257816520912,40.9102408353819,45.8240964915293));
#33469=CARTESIAN_POINT('Ctrl Pts',(43.2557945644409,40.9142791956273,45.7969098737515));
#33470=CARTESIAN_POINT('Ctrl Pts',(43.1823909277244,40.9185146958935,45.7683960909681));
#33471=CARTESIAN_POINT('Ctrl Pts',(43.1074211549665,40.9227501961598,45.7435006742057));
#33472=CARTESIAN_POINT('Ctrl Pts',(43.031276273961,40.926985696426,45.7223958406181));
#33473=CARTESIAN_POINT('Ctrl Pts',(42.9552417788638,40.9312150565613,45.7013216023402));
#33474=CARTESIAN_POINT('Ctrl Pts',(42.8780360069106,40.9354444166965,45.6840271591567));
#33475=CARTESIAN_POINT('Ctrl Pts',(42.8000689170705,40.9396737768318,45.6706362880619));
#33476=CARTESIAN_POINT('Ctrl Pts',(42.7221928766266,40.9438981979513,45.6572610547283));
#33477=CARTESIAN_POINT('Ctrl Pts',(42.643557745202,40.9481226190708,45.6477804138057));
#33478=CARTESIAN_POINT('Ctrl Pts',(42.5645860706328,40.9523470401903,45.6422676432102));
#33479=CARTESIAN_POINT('Ctrl Pts',(42.4856648969569,40.9565687598723,45.6367583979273));
#33480=CARTESIAN_POINT('Ctrl Pts',(42.4064080742356,40.9607904795543,45.6352120194146));
#33481=CARTESIAN_POINT('Ctrl Pts',(42.327244500359,40.9650121992364,45.6376500940437));
#33482=CARTESIAN_POINT('Ctrl Pts',(42.2481068284513,40.9692325375905,45.6400873709456));
#33483=CARTESIAN_POINT('Ctrl Pts',(42.1690628135786,40.9734528759447,45.6465064978454));
#33484=CARTESIAN_POINT('Ctrl Pts',(42.0905410869398,40.9776732142988,45.6568769511552));
#33485=CARTESIAN_POINT('Ctrl Pts',(42.0120205315739,40.9818934897001,45.6672472497738));
#33486=CARTESIAN_POINT('Ctrl Pts',(41.9340227140917,40.9861137651014,45.6815686948655));
#33487=CARTESIAN_POINT('Ctrl Pts',(41.8569693831561,40.9903340405027,45.6997591017309));
#33488=CARTESIAN_POINT('Ctrl Pts',(41.779838980939,40.9945585371625,45.7179677032408));
#33489=CARTESIAN_POINT('Ctrl Pts',(41.7036554103252,40.9987830338224,45.740052888968));
#33490=CARTESIAN_POINT('Ctrl Pts',(41.6288278925616,41.0030075304822,45.7658818246098));
#33491=CARTESIAN_POINT('Ctrl Pts',(41.5539644503024,41.0072340553119,45.791723160656));
#33492=CARTESIAN_POINT('Ctrl Pts',(41.4804587938383,41.0114605801415,45.8213116516826));
#33493=CARTESIAN_POINT('Ctrl Pts',(41.4087002803684,41.0156871049712,45.8544661953821));
#33494=CARTESIAN_POINT('Ctrl Pts',(41.3368105947416,41.0199213557465,45.8876813444759));
#33495=CARTESIAN_POINT('Ctrl Pts',(41.266674850631,41.0241556065219,45.9244753533669));
#33496=CARTESIAN_POINT('Ctrl Pts',(41.1986577250075,41.0283898572972,45.9646211214578));
#33497=CARTESIAN_POINT('Ctrl Pts',(41.1337872979375,41.0324282175425,46.0029096127346));
#33498=CARTESIAN_POINT('Ctrl Pts',(41.0708440741402,41.0364665777878,46.0442463676946));
#33499=CARTESIAN_POINT('Ctrl Pts',(41.0101169467817,41.0405049380331,46.0883997438594));
#33500=CARTESIAN_POINT('Ctrl Pts',(40.9469663954162,41.0447044562254,46.1343151390172));
#33501=CARTESIAN_POINT('Ctrl Pts',(40.8859635327625,41.0489039744176,46.183457914074));
#33502=CARTESIAN_POINT('Ctrl Pts',(40.8274614140943,41.0531034926098,46.2355984479893));
#33503=CARTESIAN_POINT('Ctrl Pts',(40.7690443249774,41.0572969070377,46.2876631985604));
#33504=CARTESIAN_POINT('Ctrl Pts',(40.7131211190808,41.0614903214655,46.3427167443031));
#33505=CARTESIAN_POINT('Ctrl Pts',(40.6600146796133,41.0656837358934,46.4004870973516));
#33506=CARTESIAN_POINT('Ctrl Pts',(40.6069695066388,41.069872312569,46.4581908033612));
#33507=CARTESIAN_POINT('Ctrl Pts',(40.5567349671245,41.0740608892447,46.5186047406997));
#33508=CARTESIAN_POINT('Ctrl Pts',(40.5095984934268,41.0782494659203,46.5814188127409));
#33509=CARTESIAN_POINT('Ctrl Pts',(40.4624910896804,41.0824354594218,46.6441941461604));
#33510=CARTESIAN_POINT('Ctrl Pts',(40.4184782474128,41.0866214529232,46.709366296129));
#33511=CARTESIAN_POINT('Ctrl Pts',(40.3778074617442,41.0908074464247,46.7765917365317));
#33512=CARTESIAN_POINT('Ctrl Pts',(40.3371485197186,41.094992220933,46.8437976003735));
#33513=CARTESIAN_POINT('Ctrl Pts',(40.2998299494773,41.0991769954412,46.9130551586631));
#33514=CARTESIAN_POINT('Ctrl Pts',(40.2660552989271,41.1033617699494,46.9839928870017));
#33515=CARTESIAN_POINT('Ctrl Pts',(40.232279489984,41.1075466879859,47.0549330483418));
#33516=CARTESIAN_POINT('Ctrl Pts',(40.2020480453447,41.1117316060223,47.1275530613374));
#33517=CARTESIAN_POINT('Ctrl Pts',(40.1755173132373,41.1159165240587,47.2014593202643));
#33518=CARTESIAN_POINT('Ctrl Pts',(40.1489607095979,41.1201055230319,47.2754376491261));
#33519=CARTESIAN_POINT('Ctrl Pts',(40.1261121823859,41.1242945220051,47.3507042762981));
#33520=CARTESIAN_POINT('Ctrl Pts',(40.1070786252969,41.1284835209783,47.4268490510088));
#33521=CARTESIAN_POINT('Ctrl Pts',(40.0880345971696,41.1326748244691,47.5030357156744));
#33522=CARTESIAN_POINT('Ctrl Pts',(40.0728098073642,41.13686612796,47.5801010200745));
#33523=CARTESIAN_POINT('Ctrl Pts',(40.0614597913776,41.1410574314508,47.6576257405177));
#33524=CARTESIAN_POINT('Ctrl Pts',(40.0500915413763,41.1452554683497,47.7352750058851));
#33525=CARTESIAN_POINT('Ctrl Pts',(40.0426105323222,41.1494535052486,47.8133846847294));
#33526=CARTESIAN_POINT('Ctrl Pts',(40.0390202890001,41.1536515421475,47.891532285233));
#33527=CARTESIAN_POINT('Ctrl Pts',(40.0373464509499,41.1556087448401,47.9279661465382));
#33528=CARTESIAN_POINT('Ctrl Pts',(40.0365175675292,41.1575659475328,47.9644082776245));
#33529=CARTESIAN_POINT('Ctrl Pts',(40.0365301409399,41.1595231502254,48.0008162196351));
#33530=CARTESIAN_POINT('',(40.0365310012703,41.953273150305,47.9978244670332));
#33531=CARTESIAN_POINT('Ctrl Pts',(40.0365301409402,41.1595231502717,48.0008162204963));
#33532=CARTESIAN_POINT('Ctrl Pts',(40.0365455750992,41.1619256603275,48.0455077831622));
#33533=CARTESIAN_POINT('Ctrl Pts',(40.0378285482484,41.1643281703832,48.0901759288546));
#33534=CARTESIAN_POINT('Ctrl Pts',(40.0403756299082,41.1667306804389,48.1347711874589));
#33535=CARTESIAN_POINT('Ctrl Pts',(40.0448660023929,41.1709661807051,48.2133903088399));
#33536=CARTESIAN_POINT('Ctrl Pts',(40.0532984169016,41.1752016809713,48.2919342009553));
#33537=CARTESIAN_POINT('Ctrl Pts',(40.0656674450805,41.1794371812375,48.369975626147));
#33538=CARTESIAN_POINT('Ctrl Pts',(40.0780185420946,41.1836665413727,48.4479039160434));
#33539=CARTESIAN_POINT('Ctrl Pts',(40.0942948471514,41.1878959015079,48.5253307258805));
#33540=CARTESIAN_POINT('Ctrl Pts',(40.1144390024818,41.1921252616431,48.6018316770691));
#33541=CARTESIAN_POINT('Ctrl Pts',(40.1345596336153,41.1963496827626,48.6782432910075));
#33542=CARTESIAN_POINT('Ctrl Pts',(40.158539020312,41.200574103882,48.7537307433428));
#33543=CARTESIAN_POINT('Ctrl Pts',(40.1862686316953,41.2047985250015,48.8278791396597));
#33544=CARTESIAN_POINT('Ctrl Pts',(40.2139805105162,41.2090202446835,48.9019801194787));
#33545=CARTESIAN_POINT('Ctrl Pts',(40.2454376901529,41.2132419643655,48.9747433044258));
#33546=CARTESIAN_POINT('Ctrl Pts',(40.2804819684672,41.2174636840476,49.0457694559066));
#33547=CARTESIAN_POINT('Ctrl Pts',(40.3155147804497,41.2216840224017,49.116772367947));
#33548=CARTESIAN_POINT('Ctrl Pts',(40.3541321530474,41.2259043607559,49.1860389544874));
#33549=CARTESIAN_POINT('Ctrl Pts',(40.396128575788,41.23012469911,49.2531918273458));
#33550=CARTESIAN_POINT('Ctrl Pts',(40.438124372087,41.2343449745113,49.3203436985154));
#33551=CARTESIAN_POINT('Ctrl Pts',(40.4834988683402,41.2385652499126,49.3853815214434));
#33552=CARTESIAN_POINT('Ctrl Pts',(40.5320023974853,41.2427855253139,49.4479555925163));
#33553=CARTESIAN_POINT('Ctrl Pts',(40.5805544414589,41.2470100219738,49.5105922522376));
#33554=CARTESIAN_POINT('Ctrl Pts',(40.6322414821881,41.2512345186336,49.5707598654583));
#33555=CARTESIAN_POINT('Ctrl Pts',(40.6867729571565,41.2554590152935,49.6281411304214));
#33556=CARTESIAN_POINT('Ctrl Pts',(40.7413306125435,41.2596855401231,49.6855499439798));
#33557=CARTESIAN_POINT('Ctrl Pts',(40.7987350821282,41.2639120649528,49.7401694204061));
#33558=CARTESIAN_POINT('Ctrl Pts',(40.8586601173245,41.2681385897825,49.7917203484288));
#33559=CARTESIAN_POINT('Ctrl Pts',(40.9186946934761,41.2723728405578,49.8433655098197));
#33560=CARTESIAN_POINT('Ctrl Pts',(40.9812586703905,41.2766070913331,49.8919306257449));
#33561=CARTESIAN_POINT('Ctrl Pts',(41.0459941758621,41.2808413421085,49.9371780168846));
#33562=CARTESIAN_POINT('Ctrl Pts',(41.1077348014509,41.284879702354,49.9803321131547));
#33563=CARTESIAN_POINT('Ctrl Pts',(41.171450152885,41.2889180625995,50.0204685146466));
#33564=CARTESIAN_POINT('Ctrl Pts',(41.236809649188,41.292956422845,50.0574203869598));
#33565=CARTESIAN_POINT('Ctrl Pts',(41.3053597901279,41.2971919231113,50.09617613323));
#33566=CARTESIAN_POINT('Ctrl Pts',(41.3759792723293,41.3014274233775,50.1315758131263));
#33567=CARTESIAN_POINT('Ctrl Pts',(41.4483058402374,41.3056629236438,50.1633928601097));
#33568=CARTESIAN_POINT('Ctrl Pts',(41.5205275575793,41.3098922837791,50.1951637824742));
#33569=CARTESIAN_POINT('Ctrl Pts',(41.5944510202613,41.3141216439143,50.2233621982639));
#33570=CARTESIAN_POINT('Ctrl Pts',(41.6696882839139,41.3183510040496,50.2478067617674));
#33571=CARTESIAN_POINT('Ctrl Pts',(41.7448376860415,41.3225754251691,50.2722227790889));
#33572=CARTESIAN_POINT('Ctrl Pts',(41.8212973962415,41.3267998462886,50.292893511118));
#33573=CARTESIAN_POINT('Ctrl Pts',(41.8986597623857,41.3310242674081,50.3096857810206));
#33574=CARTESIAN_POINT('Ctrl Pts',(41.975972656759,41.3352459870901,50.326467312584));
#33575=CARTESIAN_POINT('Ctrl Pts',(42.0541866039638,41.3394677067721,50.3393752054039));
#33576=CARTESIAN_POINT('Ctrl Pts',(42.1328802471267,41.3436894264542,50.348326527237));
#33577=CARTESIAN_POINT('Ctrl Pts',(42.2115481420801,41.3479097648083,50.3572749202374));
#33578=CARTESIAN_POINT('Ctrl Pts',(42.290694955341,41.3521301031625,50.3622692598365));
#33579=CARTESIAN_POINT('Ctrl Pts',(42.3698921134399,41.3563504415166,50.3632782223147));
#33580=CARTESIAN_POINT('Ctrl Pts',(42.4490880901907,41.3605707169179,50.3642871697427));
#33581=CARTESIAN_POINT('Ctrl Pts',(42.5283339409563,41.3647909923191,50.3613108535745));
#33582=CARTESIAN_POINT('Ctrl Pts',(42.6072004874271,41.3690112677204,50.3543700641382));
#33583=CARTESIAN_POINT('Ctrl Pts',(42.6861459188172,41.3732357643802,50.3474223322955));
#33584=CARTESIAN_POINT('Ctrl Pts',(42.7647108193664,41.3774602610401,50.3365022470497));
#33585=CARTESIAN_POINT('Ctrl Pts',(42.8424711375432,41.3816847576999,50.321682522082));
#33586=CARTESIAN_POINT('Ctrl Pts',(42.9202687882454,41.3859112825295,50.3068556822032));
#33587=CARTESIAN_POINT('Ctrl Pts',(42.9972606303851,41.3901378073592,50.288125584035));
#33588=CARTESIAN_POINT('Ctrl Pts',(43.073035341738,41.3943643321888,50.2656155608734));
#33589=CARTESIAN_POINT('Ctrl Pts',(43.1489485667229,41.3985985829641,50.2430643901441));
#33590=CARTESIAN_POINT('Ctrl Pts',(43.2236397713106,41.4028328337395,50.2167196439986));
#33591=CARTESIAN_POINT('Ctrl Pts',(43.2967154547051,41.4070670845148,50.1867537205166));
#33592=CARTESIAN_POINT('Ctrl Pts',(43.3664104138306,41.4111054447601,50.1581741203648));
#33593=CARTESIAN_POINT('Ctrl Pts',(43.4346357168277,41.4151438050053,50.1263011731616));
#33594=CARTESIAN_POINT('Ctrl Pts',(43.5010722097884,41.4191821652505,50.0913226507958));
#33595=CARTESIAN_POINT('Ctrl Pts',(43.5707519229727,41.4234176655168,50.0546365871968));
#33596=CARTESIAN_POINT('Ctrl Pts',(43.6387285861544,41.427653165783,50.0143945461722));
#33597=CARTESIAN_POINT('Ctrl Pts',(43.7046156733432,41.4318886660493,49.9707786242415));
#33598=CARTESIAN_POINT('Ctrl Pts',(43.770407245169,41.4361180261845,49.9272259315534));
#33599=CARTESIAN_POINT('Ctrl Pts',(43.8341148684436,41.4403473863198,49.8803093276203));
#33600=CARTESIAN_POINT('Ctrl Pts',(43.8953761517319,41.4445767464551,49.8302569780584));
#33601=CARTESIAN_POINT('Ctrl Pts',(43.9565658945426,41.4488011675746,49.7802630792635));
#33602=CARTESIAN_POINT('Ctrl Pts',(44.015314612821,41.453025588694,49.727141007136));
#33603=CARTESIAN_POINT('Ctrl Pts',(44.0712897647799,41.4572500098135,49.6711615610234));
#33604=CARTESIAN_POINT('Ctrl Pts',(44.127229121687,41.4614717294956,49.6152179127085));
#33605=CARTESIAN_POINT('Ctrl Pts',(44.1803981016048,41.4656934491776,49.5564208480802));
#33606=CARTESIAN_POINT('Ctrl Pts',(44.2304990057065,41.4699151688597,49.4950798744574));
#33607=CARTESIAN_POINT('Ctrl Pts',(44.2805835170155,41.4741355072138,49.433758971328));
#33608=CARTESIAN_POINT('Ctrl Pts',(44.327601649166,41.478355845568,49.3698961752223));
#33609=CARTESIAN_POINT('Ctrl Pts',(44.3712952034314,41.4825761839222,49.3038349825911));
#33610=CARTESIAN_POINT('Ctrl Pts',(44.4149881059399,41.4867964593235,49.2377747753647));
#33611=CARTESIAN_POINT('Ctrl Pts',(44.4553562713294,41.4910167347247,49.1695166290041));
#33612=CARTESIAN_POINT('Ctrl Pts',(44.4921850030362,41.495237010126,49.0994327419039));
#33613=CARTESIAN_POINT('Ctrl Pts',(44.5290505720545,41.4994615067859,49.0292787545897));
#33614=CARTESIAN_POINT('Ctrl Pts',(44.5623694164245,41.5036860034458,48.9572957950096));
#33615=CARTESIAN_POINT('Ctrl Pts',(44.5919732821235,41.5079105001056,48.8838798398859));
#33616=CARTESIAN_POINT('Ctrl Pts',(44.621591360561,41.5121370249353,48.8104286379541));
#33617=CARTESIAN_POINT('Ctrl Pts',(44.6474907536523,41.5163635497649,48.7355435141247));
#33618=CARTESIAN_POINT('Ctrl Pts',(44.6695526663381,41.5205900745946,48.6596371241962));
#33619=CARTESIAN_POINT('Ctrl Pts',(44.6916549074606,41.5248243253699,48.5835919799317));
#33620=CARTESIAN_POINT('Ctrl Pts',(44.7099055425513,41.5290585761453,48.506522297105));
#33621=CARTESIAN_POINT('Ctrl Pts',(44.7242366826522,41.5332928269206,48.4288522868238));
#33622=CARTESIAN_POINT('Ctrl Pts',(44.7379048165262,41.5373311871659,48.3547755496595));
#33623=CARTESIAN_POINT('Ctrl Pts',(44.7480080816397,41.5413695474113,48.2801531618215));
#33624=CARTESIAN_POINT('Ctrl Pts',(44.7545317398734,41.5454079076566,48.2053551236974));
#33625=CARTESIAN_POINT('Ctrl Pts',(44.7613738625438,41.5496434079228,48.1269056810659));
#33626=CARTESIAN_POINT('Ctrl Pts',(44.7643039728385,41.5538789081891,48.047964797762));
#33627=CARTESIAN_POINT('Ctrl Pts',(44.76326611177,41.5581144084553,47.9689560656592));
#33628=CARTESIAN_POINT('Ctrl Pts',(44.7622297552707,41.5623437685906,47.8900618711397));
#33629=CARTESIAN_POINT('Ctrl Pts',(44.757236856571,41.5665731287258,47.8111004884866));
#33630=CARTESIAN_POINT('Ctrl Pts',(44.7482832586759,41.5708024888611,47.7325001347245));
#33631=CARTESIAN_POINT('Ctrl Pts',(44.7393401167268,41.5750269099806,47.6539915698795));
#33632=CARTESIAN_POINT('Ctrl Pts',(44.7264455197113,41.5792513311001,47.5758436600272));
#33633=CARTESIAN_POINT('Ctrl Pts',(44.7096473152042,41.5834757522196,47.4984825822863));
#33634=CARTESIAN_POINT('Ctrl Pts',(44.6928598528313,41.5876974719016,47.4211709754925));
#33635=CARTESIAN_POINT('Ctrl Pts',(44.6721738368805,41.5919191915836,47.3446456595606));
#33636=CARTESIAN_POINT('Ctrl Pts',(44.6476885191618,41.5961409112656,47.2693244483847));
#33637=CARTESIAN_POINT('Ctrl Pts',(44.62321121293,41.6003612496198,47.1940278819736));
#33638=CARTESIAN_POINT('Ctrl Pts',(44.5949372183358,41.6045815879739,47.1199350840304));
#33639=CARTESIAN_POINT('Ctrl Pts',(44.5630157422213,41.6088019263281,47.0474490355876));
#33640=CARTESIAN_POINT('Ctrl Pts',(44.5310947422649,41.6130222017294,46.9749640683861));
#33641=CARTESIAN_POINT('Ctrl Pts',(44.4955265593229,41.6172424771306,46.9040862320499));
#33642=CARTESIAN_POINT('Ctrl Pts',(44.4565080736778,41.6214627525319,46.8351974485785));
#33643=CARTESIAN_POINT('Ctrl Pts',(44.4174505604573,41.6256872491918,46.7662397602752));
#33644=CARTESIAN_POINT('Ctrl Pts',(44.374936082379,41.6299117458516,46.6992755085151));
#33645=CARTESIAN_POINT('Ctrl Pts',(44.3292066429857,41.6341362425114,46.6346604196904));
#33646=CARTESIAN_POINT('Ctrl Pts',(44.2834552490081,41.6383627673411,46.5700143093305));
#33647=CARTESIAN_POINT('Ctrl Pts',(44.234486109346,41.6425892921707,46.5077199781744));
#33648=CARTESIAN_POINT('Ctrl Pts',(44.1825820119918,41.6468158170004,46.4481005794758));
#33649=CARTESIAN_POINT('Ctrl Pts',(44.1305830356877,41.6510500677757,46.3883721985152));
#33650=CARTESIAN_POINT('Ctrl Pts',(44.0756387076146,41.655284318551,46.3313288596858));
#33651=CARTESIAN_POINT('Ctrl Pts',(44.0180690738715,41.6595185693264,46.2772571541056));
#33652=CARTESIAN_POINT('Ctrl Pts',(43.963162802944,41.6635569295717,46.2256869855449));
#33653=CARTESIAN_POINT('Ctrl Pts',(43.9058690608256,41.667595289817,46.1768197792944));
#33654=CARTESIAN_POINT('Ctrl Pts',(43.84649105503,41.6716336500623,46.130868097587));
#33655=CARTESIAN_POINT('Ctrl Pts',(43.7842144021118,41.6758691503286,46.082673199588));
#33656=CARTESIAN_POINT('Ctrl Pts',(43.719408068394,41.6801046505948,46.0375025485721));
#33657=CARTESIAN_POINT('Ctrl Pts',(43.652398033195,41.6843401508611,45.9956323672167));
#33658=CARTESIAN_POINT('Ctrl Pts',(43.5854851412774,41.6885695109963,45.9538228843342));
#33659=CARTESIAN_POINT('Ctrl Pts',(43.5163752865965,41.6927988711316,45.91530461628));
#33660=CARTESIAN_POINT('Ctrl Pts',(43.4454263627895,41.6970282312668,45.8803127209693));
#33661=CARTESIAN_POINT('Ctrl Pts',(43.3745602926158,41.7012526523863,45.8453616889375));
#33662=CARTESIAN_POINT('Ctrl Pts',(43.3018598398523,41.7054770735058,45.8139290528015));
#33663=CARTESIAN_POINT('Ctrl Pts',(43.2277093165479,41.7097014946253,45.7862051296022));
#33664=CARTESIAN_POINT('Ctrl Pts',(43.1536062111015,41.7139232143074,45.7584989353277));
#33665=CARTESIAN_POINT('Ctrl Pts',(43.0780553140324,41.7181449339894,45.7344969106953));
#33666=CARTESIAN_POINT('Ctrl Pts',(43.0014617129366,41.7223666536714,45.7143416159077));
#33667=CARTESIAN_POINT('Ctrl Pts',(42.9248931729259,41.7265869920256,45.6941929158428));
#33668=CARTESIAN_POINT('Ctrl Pts',(42.8472830598909,41.7308073303798,45.6778885657465));
#33669=CARTESIAN_POINT('Ctrl Pts',(42.7690510118218,41.7350276687339,45.6655210877857));
#33670=CARTESIAN_POINT('Ctrl Pts',(42.6908201307046,41.7392479441352,45.6531537943049));
#33671=CARTESIAN_POINT('Ctrl Pts',(42.6119677967967,41.7434682195365,45.6447233281987));
#33672=CARTESIAN_POINT('Ctrl Pts',(42.532921727776,41.7476884949378,45.6402707241751));
#33673=CARTESIAN_POINT('Ctrl Pts',(42.4537965942717,41.7519129915976,45.6358136665102));
#33674=CARTESIAN_POINT('Ctrl Pts',(42.3744778082822,41.7561374882575,45.6353424455197));
#33675=CARTESIAN_POINT('Ctrl Pts',(42.2953954675445,41.7603619849173,45.6388459743825));
#33676=CARTESIAN_POINT('Ctrl Pts',(42.2162751595817,41.764588509747,45.6423511852804));
#33677=CARTESIAN_POINT('Ctrl Pts',(42.1373919909055,41.7688150345766,45.6498349031435));
#33678=CARTESIAN_POINT('Ctrl Pts',(42.0591707283695,41.7730415594063,45.6612341184933));
#33679=CARTESIAN_POINT('Ctrl Pts',(41.9808064799878,41.7772758101816,45.6726541712267));
#33680=CARTESIAN_POINT('Ctrl Pts',(41.9031070171583,41.781510060957,45.6880039324047));
#33681=CARTESIAN_POINT('Ctrl Pts',(41.8264865132704,41.7857443117323,45.707169277631));
#33682=CARTESIAN_POINT('Ctrl Pts',(41.7534107288416,41.7897826719776,45.7254479702158));
#33683=CARTESIAN_POINT('Ctrl Pts',(41.6813166099833,41.7938210322229,45.7471968726855));
#33684=CARTESIAN_POINT('Ctrl Pts',(41.6105469601833,41.7978593924682,45.7722759733701));
#33685=CARTESIAN_POINT('Ctrl Pts',(41.5363225590991,41.8020948927345,45.7985793567174));
#33686=CARTESIAN_POINT('Ctrl Pts',(41.4632730988246,41.8063303930007,45.8286463644956));
#33687=CARTESIAN_POINT('Ctrl Pts',(41.3918072424209,41.810565893267,45.8623522730663));
#33688=CARTESIAN_POINT('Ctrl Pts',(41.3204449888248,41.8147952534022,45.8960093187682));
#33689=CARTESIAN_POINT('Ctrl Pts',(41.250662201115,41.8190246135375,45.9332945910263));
#33690=CARTESIAN_POINT('Ctrl Pts',(41.18285027111,41.8232539736728,45.9740343096777));
#33691=CARTESIAN_POINT('Ctrl Pts',(41.1151175313799,41.8274783947922,46.0147264527842));
#33692=CARTESIAN_POINT('Ctrl Pts',(41.0493514759781,41.8317028159117,46.0588647853688));
#33693=CARTESIAN_POINT('Ctrl Pts',(40.9859200764249,41.8359272370312,46.1062290501115));
#33694=CARTESIAN_POINT('Ctrl Pts',(40.9225292400528,41.8401489567133,46.1535630263021));
#33695=CARTESIAN_POINT('Ctrl Pts',(40.8614704713665,41.8443706763953,46.2041185601328));
#33696=CARTESIAN_POINT('Ctrl Pts',(40.8030828164395,41.8485923960773,46.2576320854225));
#33697=CARTESIAN_POINT('Ctrl Pts',(40.7447142656932,41.8528127344315,46.311128101325));
#33698=CARTESIAN_POINT('Ctrl Pts',(40.6890154390263,41.8570330727856,46.3675798699888));
#33699=CARTESIAN_POINT('Ctrl Pts',(40.636291170759,41.8612534111398,46.4266845177915));
#33700=CARTESIAN_POINT('Ctrl Pts',(40.5835676889556,41.865473686541,46.4857882839569));
#33701=CARTESIAN_POINT('Ctrl Pts',(40.5338189887963,41.8696939619423,46.5475444994656));
#33702=CARTESIAN_POINT('Ctrl Pts',(40.4873109732458,41.8739142373436,46.6116156411736));
#33703=CARTESIAN_POINT('Ctrl Pts',(40.4407564388452,41.8781387340034,46.6757508689494));
#33704=CARTESIAN_POINT('Ctrl Pts',(40.3974493406097,41.8823632306633,46.7422052676186));
#33705=CARTESIAN_POINT('Ctrl Pts',(40.357613033427,41.8865877273231,46.8106111150374));
#33706=CARTESIAN_POINT('Ctrl Pts',(40.3177576009373,41.8908142521528,46.8790498039248));
#33707=CARTESIAN_POINT('Ctrl Pts',(40.2813764948038,41.8950407769824,46.9494413904245));
#33708=CARTESIAN_POINT('Ctrl Pts',(40.2486465175392,41.8992673018121,47.0213945460995));
#33709=CARTESIAN_POINT('Ctrl Pts',(40.2158567109735,41.9035015525874,47.0934792297308));
#33710=CARTESIAN_POINT('Ctrl Pts',(40.1867315428286,41.9077358033627,47.1671307488784));
#33711=CARTESIAN_POINT('Ctrl Pts',(40.161399095563,41.9119700541381,47.2419390317701));
#33712=CARTESIAN_POINT('Ctrl Pts',(40.1372386115997,41.9160084143834,47.3132864345762));
#33713=CARTESIAN_POINT('Ctrl Pts',(40.1165277442649,41.9200467746287,47.3856855830994));
#33714=CARTESIAN_POINT('Ctrl Pts',(40.0993341935841,41.924085134874,47.458772424863));
#33715=CARTESIAN_POINT('Ctrl Pts',(40.0751743144991,41.9297597216444,47.5614719365866));
#33716=CARTESIAN_POINT('Ctrl Pts',(40.0578822519074,41.9354343084147,47.6658441082782));
#33717=CARTESIAN_POINT('Ctrl Pts',(40.047639778813,41.9411088951851,47.7711073817772));
#33718=CARTESIAN_POINT('Ctrl Pts',(40.0403210634903,41.9451636468806,47.8463228034409));
#33719=CARTESIAN_POINT('Ctrl Pts',(40.0366008029736,41.9492183985762,47.9219928813227));
#33720=CARTESIAN_POINT('Ctrl Pts',(40.0365310012709,41.9532731502717,47.9978244664113));
#33721=CARTESIAN_POINT('',(40.0365300138095,42.7470231503245,48.0002554931331));
#33722=CARTESIAN_POINT('Ctrl Pts',(40.0365310012703,41.953273150305,47.9978244670332));
#33723=CARTESIAN_POINT('Ctrl Pts',(40.036459200662,41.957444018785,48.0758276573125));
#33724=CARTESIAN_POINT('Ctrl Pts',(40.040253223248,41.9616148872651,48.1539409988832));
#33725=CARTESIAN_POINT('Ctrl Pts',(40.0479190791829,41.9657857557452,48.2317450815622));
#33726=CARTESIAN_POINT('Ctrl Pts',(40.0555795272878,41.9699536819122,48.3094942778379));
#33727=CARTESIAN_POINT('Ctrl Pts',(40.0671063450249,41.9741216080792,48.3869341692086));
#33728=CARTESIAN_POINT('Ctrl Pts',(40.0824535028735,41.9782895342462,48.4636471444499));
#33729=CARTESIAN_POINT('Ctrl Pts',(40.0977949205481,41.9824559015173,48.5403314273542));
#33730=CARTESIAN_POINT('Ctrl Pts',(40.1169537485858,41.9866222687885,48.6162888607868));
#33731=CARTESIAN_POINT('Ctrl Pts',(40.1398325646431,41.9907886360596,48.6911104145157));
#33732=CARTESIAN_POINT('Ctrl Pts',(40.1627104054812,41.9949548257376,48.7659287789444));
#33733=CARTESIAN_POINT('Ctrl Pts',(40.1893077766097,41.9991210154155,48.8396108987954));
#33734=CARTESIAN_POINT('Ctrl Pts',(40.2194774146584,42.0032872050935,48.9117629602671));
#33735=CARTESIAN_POINT('Ctrl Pts',(40.2496759753692,42.0074573887636,48.9839841916007));
#33736=CARTESIAN_POINT('Ctrl Pts',(40.2834534545533,42.0116275724336,49.0546719894266));
#33737=CARTESIAN_POINT('Ctrl Pts',(40.3206147694229,42.0157977561037,49.1234533829927));
#33738=CARTESIAN_POINT('Ctrl Pts',(40.3577942885969,42.0199699826319,49.1922684706685));
#33739=CARTESIAN_POINT('Ctrl Pts',(40.3983606912674,42.0241422091601,49.2591748830298));
#33740=CARTESIAN_POINT('Ctrl Pts',(40.4420747218958,42.0283144356882,49.3238274231412));
#33741=CARTESIAN_POINT('Ctrl Pts',(40.4858650365847,42.0324939430454,49.3885927864859));
#33742=CARTESIAN_POINT('Ctrl Pts',(40.53281365624,42.0366734504025,49.451096038529));
#33743=CARTESIAN_POINT('Ctrl Pts',(40.5826404409023,42.0408529577597,49.5110243789748));
#33744=CARTESIAN_POINT('Ctrl Pts',(40.6202252309282,42.0440055975998,49.5562288630193));
#33745=CARTESIAN_POINT('Ctrl Pts',(40.6594467906287,42.0471582374399,49.5999689452227));
#33746=CARTESIAN_POINT('Ctrl Pts',(40.7001717981188,42.0503108772799,49.6421250028512));
#33747=CARTESIAN_POINT('Ctrl Pts',(40.7548849238852,42.0545463775462,49.6987607120874));
#33748=CARTESIAN_POINT('Ctrl Pts',(40.8125356685345,42.0587818778124,49.7527666399521));
#33749=CARTESIAN_POINT('Ctrl Pts',(40.8728410815323,42.0630173780787,49.8038226294856));
#33750=CARTESIAN_POINT('Ctrl Pts',(40.9330590708229,42.0672467382139,49.8548046040402));
#33751=CARTESIAN_POINT('Ctrl Pts',(40.9959237309831,42.0714760983492,49.9028448318794));
#33752=CARTESIAN_POINT('Ctrl Pts',(41.0611146327495,42.0757054584845,49.9476592140984));
#33753=CARTESIAN_POINT('Ctrl Pts',(41.1262294050587,42.079929879604,49.9924212624103));
#33754=CARTESIAN_POINT('Ctrl Pts',(41.1936646358799,42.0841543007234,50.0339646865659));
#33755=CARTESIAN_POINT('Ctrl Pts',(41.2630673141337,42.0883787218429,50.0720459716688));
#33756=CARTESIAN_POINT('Ctrl Pts',(41.3324256106866,42.092600441525,50.1101029045097));
#33757=CARTESIAN_POINT('Ctrl Pts',(41.4037484471551,42.096822161207,50.1447018673911));
#33758=CARTESIAN_POINT('Ctrl Pts',(41.4766553964691,42.101043880889,50.1756436252361));
#33759=CARTESIAN_POINT('Ctrl Pts',(41.549538490954,42.1052642192432,50.2065752590757));
#33760=CARTESIAN_POINT('Ctrl Pts',(41.6240042373583,42.1094845575973,50.2338518807473));
#33761=CARTESIAN_POINT('Ctrl Pts',(41.6996506258257,42.1137048959515,50.2573216862011));
#33762=CARTESIAN_POINT('Ctrl Pts',(41.7752958859104,42.1179251713528,50.2807911415664));
#33763=CARTESIAN_POINT('Ctrl Pts',(41.8521213043839,42.122145446754,50.3004537557839));
#33764=CARTESIAN_POINT('Ctrl Pts',(41.9297094842226,42.1263657221553,50.316207519129));
#33765=CARTESIAN_POINT('Ctrl Pts',(42.0073752703162,42.1305902188152,50.3319770399075));
#33766=CARTESIAN_POINT('Ctrl Pts',(42.0858048807772,42.134814715475,50.343829805956));
#33767=CARTESIAN_POINT('Ctrl Pts',(42.164571080988,42.1390392121349,50.3517150475755));
#33768=CARTESIAN_POINT('Ctrl Pts',(42.2433750966456,42.1432657369645,50.3596040748788));
#33769=CARTESIAN_POINT('Ctrl Pts',(42.3225155545501,42.1474922617941,50.3635217599245));
#33770=CARTESIAN_POINT('Ctrl Pts',(42.401563042116,42.1517187866238,50.3634694831538));
#33771=CARTESIAN_POINT('Ctrl Pts',(42.480755025839,42.1559530373991,50.3634171108229));
#33772=CARTESIAN_POINT('Ctrl Pts',(42.5598532296557,42.1601872881745,50.359380299558));
#33773=CARTESIAN_POINT('Ctrl Pts',(42.6384313870402,42.1644215389498,50.3514125360247));
#33774=CARTESIAN_POINT('Ctrl Pts',(42.7133742574011,42.1684598991951,50.3438133877446));
#33775=CARTESIAN_POINT('Ctrl Pts',(42.7878437876093,42.1724982594404,50.3326390509328));
#33776=CARTESIAN_POINT('Ctrl Pts',(42.8614806256514,42.1765366196857,50.3179788767477));
#33777=CARTESIAN_POINT('Ctrl Pts',(42.9387121820721,42.180772119952,50.302603039058));
#33778=CARTESIAN_POINT('Ctrl Pts',(43.015321245365,42.1850076202182,50.2833338920987));
#33779=CARTESIAN_POINT('Ctrl Pts',(43.0908854807103,42.1892431204845,50.2602362030203));
#33780=CARTESIAN_POINT('Ctrl Pts',(43.1663401718995,42.1934724806197,50.2371719982596));
#33781=CARTESIAN_POINT('Ctrl Pts',(43.240752597952,42.197701840755,50.2102904090784));
#33782=CARTESIAN_POINT('Ctrl Pts',(43.3137104742106,42.2019312008903,50.1797072303908));
#33783=CARTESIAN_POINT('Ctrl Pts',(43.386583150796,42.2061556220098,50.1491597665151));
#33784=CARTESIAN_POINT('Ctrl Pts',(43.4580042224367,42.2103800431293,50.1149194836282));
#33785=CARTESIAN_POINT('Ctrl Pts',(43.5275779102807,42.2146044642488,50.077151534469));
#33786=CARTESIAN_POINT('Ctrl Pts',(43.5971071070664,42.2188261839308,50.0394077371995));
#33787=CARTESIAN_POINT('Ctrl Pts',(43.6647908534378,42.2230479036128,49.9981409744052));
#33788=CARTESIAN_POINT('Ctrl Pts',(43.7302557792961,42.2272696232949,49.9535634114483));
#33789=CARTESIAN_POINT('Ctrl Pts',(43.7956992853222,42.231489961649,49.9090004340714));
#33790=CARTESIAN_POINT('Ctrl Pts',(43.8589250247505,42.2357103000032,49.861129071535));
#33791=CARTESIAN_POINT('Ctrl Pts',(43.9195878422038,42.2399306383573,49.8102053007121));
#33792=CARTESIAN_POINT('Ctrl Pts',(43.9802497547774,42.2441509137586,49.759282289496));
#33793=CARTESIAN_POINT('Ctrl Pts',(44.0383484627454,42.2483711891599,49.7053072632901));
#33794=CARTESIAN_POINT('Ctrl Pts',(44.0935723648291,42.2525914645612,49.6485760783134));
#33795=CARTESIAN_POINT('Ctrl Pts',(44.1488515036799,42.256815961221,49.5917881489356));
#33796=CARTESIAN_POINT('Ctrl Pts',(44.2012497643554,42.2610404578809,49.5322388908524));
#33797=CARTESIAN_POINT('Ctrl Pts',(44.2504933178218,42.2652649545407,49.4702601543934));
#33798=CARTESIAN_POINT('Ctrl Pts',(44.2997605129895,42.2694914793704,49.4082516621051));
#33799=CARTESIAN_POINT('Ctrl Pts',(44.345869710249,42.2737180042,49.3438117500821));
#33800=CARTESIAN_POINT('Ctrl Pts',(44.3885897620363,42.2779445290297,49.277302313168));
#33801=CARTESIAN_POINT('Ctrl Pts',(44.4313879046461,42.282178779805,49.210671299233));
#33802=CARTESIAN_POINT('Ctrl Pts',(44.470784288152,42.2864130305804,49.1419636092785));
#33803=CARTESIAN_POINT('Ctrl Pts',(44.5065932897786,42.2906472813557,49.0715666812476));
#33804=CARTESIAN_POINT('Ctrl Pts',(44.5407456478379,42.294685641601,49.0044265493482));
#33805=CARTESIAN_POINT('Ctrl Pts',(44.5716350990051,42.2987240018463,48.9357503632342));
#33806=CARTESIAN_POINT('Ctrl Pts',(44.5991423837312,42.3027623620916,48.8658886862507));
#33807=CARTESIAN_POINT('Ctrl Pts',(44.627992487413,42.3069978623579,48.7926165823545));
#33808=CARTESIAN_POINT('Ctrl Pts',(44.6532314452433,42.3112333626241,48.7177617654702));
#33809=CARTESIAN_POINT('Ctrl Pts',(44.6746852486706,42.3154688628904,48.6417144695116));
#33810=CARTESIAN_POINT('Ctrl Pts',(44.6961079508926,42.3196982230257,48.5657774179938));
#33811=CARTESIAN_POINT('Ctrl Pts',(44.713756269108,42.3239275831609,48.4886517682259));
#33812=CARTESIAN_POINT('Ctrl Pts',(44.7275045475989,42.3281569432962,48.4107469072391));
#33813=CARTESIAN_POINT('Ctrl Pts',(44.7412367709509,42.3323813644157,48.3329330229782));
#33814=CARTESIAN_POINT('Ctrl Pts',(44.7510779239492,42.3366057855352,48.2543421955609));
#33815=CARTESIAN_POINT('Ctrl Pts',(44.7569527916921,42.3408302066547,48.175396632336));
#33816=CARTESIAN_POINT('Ctrl Pts',(44.7628239025682,42.3450519263367,48.0965015533066));
#33817=CARTESIAN_POINT('Ctrl Pts',(44.7647337275928,42.3492736460187,48.0172526555051));
#33818=CARTESIAN_POINT('Ctrl Pts',(44.7626587137445,42.3534953657008,47.938078733319));
#33819=CARTESIAN_POINT('Ctrl Pts',(44.7605843788314,42.3577157040549,47.8589307164877));
#33820=CARTESIAN_POINT('Ctrl Pts',(44.7545278062901,42.3619360424091,47.7798580953953));
#33821=CARTESIAN_POINT('Ctrl Pts',(44.7445175537334,42.3661563807632,47.7012896367116));
#33822=CARTESIAN_POINT('Ctrl Pts',(44.7345074504951,42.3703766561645,47.6227223499979));
#33823=CARTESIAN_POINT('Ctrl Pts',(44.7205438451144,42.3745969315658,47.5446596761631));
#33824=CARTESIAN_POINT('Ctrl Pts',(44.7027069873352,42.378817206967,47.4675237363247));
#33825=CARTESIAN_POINT('Ctrl Pts',(44.6848522885429,42.3830417036269,47.3903106425766));
#33826=CARTESIAN_POINT('Ctrl Pts',(44.6631167042344,42.3872662002867,47.3140265929015));
#33827=CARTESIAN_POINT('Ctrl Pts',(44.6376311906737,42.3914906969466,47.2390814134061));
#33828=CARTESIAN_POINT('Ctrl Pts',(44.6121334415847,42.3957172217762,47.164100252926));
#33829=CARTESIAN_POINT('Ctrl Pts',(44.5828823502661,42.3999437466058,47.0904596799371));
#33830=CARTESIAN_POINT('Ctrl Pts',(44.5500572315736,42.4041702714355,47.0185498780589));
#33831=CARTESIAN_POINT('Ctrl Pts',(44.5171721096646,42.4084045222108,46.9465086274737));
#33832=CARTESIAN_POINT('Ctrl Pts',(44.4807001222147,42.4126387729862,46.8762048877178));
#33833=CARTESIAN_POINT('Ctrl Pts',(44.4408666950662,42.4168730237615,46.8080043733848));
#33834=CARTESIAN_POINT('Ctrl Pts',(44.4028760948004,42.4209113840068,46.7429590417773));
#33835=CARTESIAN_POINT('Ctrl Pts',(44.3618284249697,42.4249497442521,46.679826914187));
#33836=CARTESIAN_POINT('Ctrl Pts',(44.3179540007854,42.4289881044974,46.6188979430284));
#33837=CARTESIAN_POINT('Ctrl Pts',(44.2719377654755,42.4332236047637,46.5549946115054));
#33838=CARTESIAN_POINT('Ctrl Pts',(44.2226368249494,42.4374591050299,46.493272120739));
#33839=CARTESIAN_POINT('Ctrl Pts',(44.1702852397358,42.4416946052962,46.4340879300313));
#33840=CARTESIAN_POINT('Ctrl Pts',(44.1180095477037,42.4459239654315,46.3749895376144));
#33841=CARTESIAN_POINT('Ctrl Pts',(44.0626923015589,42.4501533255667,46.3184224865432));
#33842=CARTESIAN_POINT('Ctrl Pts',(44.0046098286107,42.454382685702,46.2647139317029));
#33843=CARTESIAN_POINT('Ctrl Pts',(43.9465951839488,42.4586071068215,46.2110680973194));
#33844=CARTESIAN_POINT('Ctrl Pts',(43.8858220723409,42.462831527941,46.1602744426767));
#33845=CARTESIAN_POINT('Ctrl Pts',(43.8226048913956,42.4670559490605,46.1126246362005));
#33846=CARTESIAN_POINT('Ctrl Pts',(43.7594281366426,42.4712776687425,46.0650053008749));
#33847=CARTESIAN_POINT('Ctrl Pts',(43.6938107884397,42.4754993884245,46.0205261051851));
#33848=CARTESIAN_POINT('Ctrl Pts',(43.6261007329175,42.4797211081066,45.9794388319976));
#33849=CARTESIAN_POINT('Ctrl Pts',(43.5584128318239,42.4839414464607,45.938365002383));
#33850=CARTESIAN_POINT('Ctrl Pts',(43.4886339839979,42.4881617848149,45.9006811348342));
#33851=CARTESIAN_POINT('Ctrl Pts',(43.4171402436681,42.492382123169,45.8665951707164));
#33852=CARTESIAN_POINT('Ctrl Pts',(43.3456475697777,42.4966023985703,45.8325097150432));
#33853=CARTESIAN_POINT('Ctrl Pts',(43.2724404784693,42.5008226739716,45.8020222569056));
#33854=CARTESIAN_POINT('Ctrl Pts',(43.1979173998788,42.5050429493729,45.7752936679484));
#33855=CARTESIAN_POINT('Ctrl Pts',(43.123319780849,42.5092674460328,45.7485383441756));
#33856=CARTESIAN_POINT('Ctrl Pts',(43.0474039879245,42.5134919426926,45.7255495589812));
#33857=CARTESIAN_POINT('Ctrl Pts',(42.9705855425879,42.5177164393525,45.7064388869076));
#33858=CARTESIAN_POINT('Ctrl Pts',(42.8937302169165,42.5219429641821,45.6873190398503));
#33859=CARTESIAN_POINT('Ctrl Pts',(42.8159718367486,42.5261694890118,45.6720811053743));
#33860=CARTESIAN_POINT('Ctrl Pts',(42.7377355652697,42.5303960138414,45.6607853606708));
#33861=CARTESIAN_POINT('Ctrl Pts',(42.6593562805094,42.5346302646167,45.6494689677247));
#33862=CARTESIAN_POINT('Ctrl Pts',(42.5804978273916,42.5388645153921,45.6421092079402));
#33863=CARTESIAN_POINT('Ctrl Pts',(42.5015897356161,42.5430987661674,45.6387143403397));
#33864=CARTESIAN_POINT('Ctrl Pts',(42.4263321947273,42.5471371264127,45.6354765306106));
#33865=CARTESIAN_POINT('Ctrl Pts',(42.3510298634973,42.551175486658,45.6358448292773));
#33866=CARTESIAN_POINT('Ctrl Pts',(42.2760511986137,42.5552138469033,45.6397823965713));
#33867=CARTESIAN_POINT('Ctrl Pts',(42.1974123115932,42.5594493471696,45.6439121834919));
#33868=CARTESIAN_POINT('Ctrl Pts',(42.1188305752909,42.5636848474358,45.6519843159781));
#33869=CARTESIAN_POINT('Ctrl Pts',(42.0407332477664,42.5679203477021,45.6639953249962));
#33870=CARTESIAN_POINT('Ctrl Pts',(41.9627491365777,42.5721497078373,45.6759889218637));
#33871=CARTESIAN_POINT('Ctrl Pts',(41.8852484996176,42.5763790679726,45.69190998523));
#33872=CARTESIAN_POINT('Ctrl Pts',(41.8086559740489,42.5806084281079,45.7117031040811));
#33873=CARTESIAN_POINT('Ctrl Pts',(41.7321528926706,42.5848328492274,45.731473108673));
#33874=CARTESIAN_POINT('Ctrl Pts',(41.6565562673637,42.5890572703469,45.7551060663524));
#33875=CARTESIAN_POINT('Ctrl Pts',(41.582281485891,42.5932816914663,45.7824953500425));
#33876=CARTESIAN_POINT('Ctrl Pts',(41.508054201737,42.5975034111484,45.8098671188033));
#33877=CARTESIAN_POINT('Ctrl Pts',(41.4351475228643,42.6017251308304,45.8409902839723));
#33878=CARTESIAN_POINT('Ctrl Pts',(41.3639614091661,42.6059468505124,45.8757084759377));
#33879=CARTESIAN_POINT('Ctrl Pts',(41.2927985872474,42.6101671888666,45.9104153082652));
#33880=CARTESIAN_POINT('Ctrl Pts',(41.2233556341836,42.6143875272207,45.9487146261067));
#33881=CARTESIAN_POINT('Ctrl Pts',(41.156010876636,42.6186078655749,45.9904026518101));
#33882=CARTESIAN_POINT('Ctrl Pts',(41.0886671236395,42.6228281409762,46.0320900556722));
#33883=CARTESIAN_POINT('Ctrl Pts',(41.0234219023212,42.6270484163774,46.0771658187454));
#33884=CARTESIAN_POINT('Ctrl Pts',(40.9606260575622,42.6312686917787,46.1253818802937));
#33885=CARTESIAN_POINT('Ctrl Pts',(40.8977674023296,42.6354931884386,46.173646169136));
#33886=CARTESIAN_POINT('Ctrl Pts',(40.8373633908965,42.6397176850984,46.225056744535));
#33887=CARTESIAN_POINT('Ctrl Pts',(40.7797326541702,42.6439421817583,46.2793245021395));
#33888=CARTESIAN_POINT('Ctrl Pts',(40.7220742490777,42.6481687065879,46.3336183135525));
#33889=CARTESIAN_POINT('Ctrl Pts',(40.6671920966208,42.6523952314176,46.3907717008113));
#33890=CARTESIAN_POINT('Ctrl Pts',(40.6153669012738,42.6566217562472,46.4504596991911));
#33891=CARTESIAN_POINT('Ctrl Pts',(40.5634469712073,42.6608560070225,46.5102568052308));
#33892=CARTESIAN_POINT('Ctrl Pts',(40.5145954546749,42.6650902577979,46.5725974101743));
#33893=CARTESIAN_POINT('Ctrl Pts',(40.4690516696586,42.6693245085732,46.6371247355493));
#33894=CARTESIAN_POINT('Ctrl Pts',(40.4256148916807,42.6733628688185,46.6986668121424));
#33895=CARTESIAN_POINT('Ctrl Pts',(40.3851867208811,42.6774012290638,46.7621974326211));
#33896=CARTESIAN_POINT('Ctrl Pts',(40.3479355059124,42.6814395893091,46.8273867845684));
#33897=CARTESIAN_POINT('Ctrl Pts',(40.3071963122816,42.6858560772042,46.8986800734954));
#33898=CARTESIAN_POINT('Ctrl Pts',(40.270113103662,42.6902725650992,46.9722089595395));
#33899=CARTESIAN_POINT('Ctrl Pts',(40.2369265036252,42.6946890529942,47.0475801922571));
#33900=CARTESIAN_POINT('Ctrl Pts',(40.2038270381793,42.6990939449781,47.1227535305983));
#33901=CARTESIAN_POINT('Ctrl Pts',(40.1746039716191,42.703498836962,47.19975920718));
#33902=CARTESIAN_POINT('Ctrl Pts',(40.1494521309674,42.7079037289459,47.2781795721282));
#33903=CARTESIAN_POINT('Ctrl Pts',(40.1243392761471,42.7123017932634,47.3564783840195));
#33904=CARTESIAN_POINT('Ctrl Pts',(40.1032852240893,42.7166998575809,47.4361871338538));
#33905=CARTESIAN_POINT('Ctrl Pts',(40.0864369623797,42.7210979218985,47.5168680181803));
#33906=CARTESIAN_POINT('Ctrl Pts',(40.0696202029547,42.7254877628707,47.597398048239));
#33907=CARTESIAN_POINT('Ctrl Pts',(40.0569936581839,42.7298776038429,47.6788961913138));
#33908=CARTESIAN_POINT('Ctrl Pts',(40.048654264041,42.7342674448151,47.7609107470266));
#33909=CARTESIAN_POINT('Ctrl Pts',(40.040576913324,42.738519346634,47.8403482120316));
#33910=CARTESIAN_POINT('Ctrl Pts',(40.0365213673141,42.7427712484528,47.9202697353209));
#33911=CARTESIAN_POINT('Ctrl Pts',(40.0365300138094,42.7470231502717,48.0002554921404));
#33912=CARTESIAN_POINT('',(40.0365309117291,43.5407731502446,48.0020759787561));
#33913=CARTESIAN_POINT('Ctrl Pts',(40.0365300138095,42.7470231503245,48.0002554931331));
#33914=CARTESIAN_POINT('Ctrl Pts',(40.0365390801091,42.751481472945,48.0841243885452));
#33915=CARTESIAN_POINT('Ctrl Pts',(40.0410166138422,42.7559397955656,48.1678918268366));
#33916=CARTESIAN_POINT('Ctrl Pts',(40.0499047771218,42.7603981181862,48.2510834210075));
#33917=CARTESIAN_POINT('Ctrl Pts',(40.0588211874745,42.7648706096019,48.3345394026533));
#33918=CARTESIAN_POINT('Ctrl Pts',(40.0721762090108,42.7693431010177,48.4174154972645));
#33919=CARTESIAN_POINT('Ctrl Pts',(40.0898604967801,42.7738155924335,48.4992453470619));
#33920=CARTESIAN_POINT('Ctrl Pts',(40.1075743816014,42.7782955691697,48.5812121502019));
#33921=CARTESIAN_POINT('Ctrl Pts',(40.1296318840185,42.7827755459059,48.6621288448638));
#33922=CARTESIAN_POINT('Ctrl Pts',(40.1558739613116,42.7872555226421,48.7415448492038));
#33923=CARTESIAN_POINT('Ctrl Pts',(40.1821907867162,42.7917482601746,48.821187062631));
#33924=CARTESIAN_POINT('Ctrl Pts',(40.2127158766436,42.7962409977071,48.8993196805187));
#33925=CARTESIAN_POINT('Ctrl Pts',(40.2472419462328,42.8007337352395,48.9755117645834));
#33926=CARTESIAN_POINT('Ctrl Pts',(40.264998067866,42.803044267398,49.0146959499898));
#33927=CARTESIAN_POINT('Ctrl Pts',(40.2838116483987,42.8053547995565,49.0533673052659));
#33928=CARTESIAN_POINT('Ctrl Pts',(40.3036499480538,42.807665331715,49.0914700639985));
#33929=CARTESIAN_POINT('Ctrl Pts',(40.3400160826526,42.8119008319812,49.1613172825985));
#33930=CARTESIAN_POINT('Ctrl Pts',(40.3799459672787,42.8161363322475,49.2294777764117));
#33931=CARTESIAN_POINT('Ctrl Pts',(40.4232592798914,42.8203718325137,49.2955641884386));
#33932=CARTESIAN_POINT('Ctrl Pts',(40.466509801949,42.824601192649,49.3615547961446));
#33933=CARTESIAN_POINT('Ctrl Pts',(40.5131337566303,42.8288305527842,49.4254769037269));
#33934=CARTESIAN_POINT('Ctrl Pts',(40.5629046426042,42.8330599129195,49.4869670772195));
#33935=CARTESIAN_POINT('Ctrl Pts',(40.6126174065022,42.837284334039,49.5483854429382));
#33936=CARTESIAN_POINT('Ctrl Pts',(40.6654695051001,42.8415087551585,49.6073771552396));
#33937=CARTESIAN_POINT('Ctrl Pts',(40.7211916668968,42.8457331762779,49.6636084339782));
#33938=CARTESIAN_POINT('Ctrl Pts',(40.7768781954243,42.84995489596,49.7198037538769));
#33939=CARTESIAN_POINT('Ctrl Pts',(40.8354308148945,42.854176615642,49.77324181136));
#33940=CARTESIAN_POINT('Ctrl Pts',(40.8965413864561,42.858398335324,49.8236234913657));
#33941=CARTESIAN_POINT('Ctrl Pts',(40.9576319629109,42.8626186736782,49.8739886867101));
#33942=CARTESIAN_POINT('Ctrl Pts',(41.0212784676792,42.8668390120323,49.9212991919717));
#33943=CARTESIAN_POINT('Ctrl Pts',(41.0871385919924,42.8710593503865,49.9652952359034));
#33944=CARTESIAN_POINT('Ctrl Pts',(41.1529977339001,42.8752796257877,50.009290623566));
#33945=CARTESIAN_POINT('Ctrl Pts',(41.2210700386964,42.879499901189,50.0499713885688));
#33946=CARTESIAN_POINT('Ctrl Pts',(41.2909842964744,42.8837201765903,50.0871211297463));
#33947=CARTESIAN_POINT('Ctrl Pts',(41.3609684847975,42.8879446732501,50.1243080293194));
#33948=CARTESIAN_POINT('Ctrl Pts',(41.4327978910302,42.89216916991,50.1579566289978));
#33949=CARTESIAN_POINT('Ctrl Pts',(41.5060773142077,42.8963936665698,50.1878968606234));
#33950=CARTESIAN_POINT('Ctrl Pts',(41.5793919186447,42.9006201913995,50.217851466476));
#33951=CARTESIAN_POINT('Ctrl Pts',(41.6541574833693,42.9048467162291,50.2440940018879));
#33952=CARTESIAN_POINT('Ctrl Pts',(41.7299619017027,42.9090732410587,50.2665037806565));
#33953=CARTESIAN_POINT('Ctrl Pts',(41.8059048879714,42.9133074918341,50.2889545237493));
#33954=CARTESIAN_POINT('Ctrl Pts',(41.8828900650561,42.9175417426094,50.3075583997282));
#33955=CARTESIAN_POINT('Ctrl Pts',(41.9604935376409,42.9217759933847,50.322245574965));
#33956=CARTESIAN_POINT('Ctrl Pts',(42.0345068153651,42.9258143536301,50.3362532726051));
#33957=CARTESIAN_POINT('Ctrl Pts',(42.109082086108,42.9298527138755,50.346698641262));
#33958=CARTESIAN_POINT('Ctrl Pts',(42.1838494209599,42.9338910741208,50.3535652461915));
#33959=CARTESIAN_POINT('Ctrl Pts',(42.2622666614811,42.9381265743871,50.3607670571347));
#33960=CARTESIAN_POINT('Ctrl Pts',(42.3411932775508,42.9423620746533,50.3640591505288));
#33961=CARTESIAN_POINT('Ctrl Pts',(42.4202059383712,42.9465975749196,50.3633836254308));
#33962=CARTESIAN_POINT('Ctrl Pts',(42.4991040559129,42.9508269350548,50.3627090796298));
#33963=CARTESIAN_POINT('Ctrl Pts',(42.5780875051341,42.9550562951901,50.3580783413496));
#33964=CARTESIAN_POINT('Ctrl Pts',(42.6567280925766,42.9592856553253,50.3494852898842));
#33965=CARTESIAN_POINT('Ctrl Pts',(42.7352768441173,42.9635100764448,50.3409022733213));
#33966=CARTESIAN_POINT('Ctrl Pts',(42.8134830653811,42.9677344975643,50.3283661893197));
#33967=CARTESIAN_POINT('Ctrl Pts',(42.8909203643071,42.9719589186838,50.3119229305512));
#33968=CARTESIAN_POINT('Ctrl Pts',(42.9683081435441,42.9761806383658,50.295490186936));
#33969=CARTESIAN_POINT('Ctrl Pts',(43.0449275185103,42.9804023580479,50.2751553248965));
#33970=CARTESIAN_POINT('Ctrl Pts',(43.1203602245478,42.9846240777299,50.2510156791523));
#33971=CARTESIAN_POINT('Ctrl Pts',(43.1957682493397,42.988844416084,50.2268839317927));
#33972=CARTESIAN_POINT('Ctrl Pts',(43.2699899295026,42.9930647544382,50.1989500156484));
#33973=CARTESIAN_POINT('Ctrl Pts',(43.3426216039958,42.9972850927923,50.1673612879676));
#33974=CARTESIAN_POINT('Ctrl Pts',(43.4152521950753,43.0015053681936,50.1357730314814));
#33975=CARTESIAN_POINT('Ctrl Pts',(43.4862923977552,43.0057256435949,50.1005302602413));
#33976=CARTESIAN_POINT('Ctrl Pts',(43.5553593911814,43.0099459189962,50.0618281010087));
#33977=CARTESIAN_POINT('Ctrl Pts',(43.6244954676909,43.014170415656,50.0230872306007));
#33978=CARTESIAN_POINT('Ctrl Pts',(43.6916539818663,43.0183949123159,49.9808802900125));
#33979=CARTESIAN_POINT('Ctrl Pts',(43.756478101255,43.0226194089757,49.9354476489215));
#33980=CARTESIAN_POINT('Ctrl Pts',(43.821333342534,43.0268459338054,49.8899931957382));
#33981=CARTESIAN_POINT('Ctrl Pts',(43.8838515855544,43.031072458635,49.8413102457139));
#33982=CARTESIAN_POINT('Ctrl Pts',(43.9437083836268,43.0352989834646,49.7896801019234));
#33983=CARTESIAN_POINT('Ctrl Pts',(44.0036745979194,43.03953323424,49.7379555799608));
#33984=CARTESIAN_POINT('Ctrl Pts',(44.0609693053627,43.0437674850153,49.6832734239026));
#33985=CARTESIAN_POINT('Ctrl Pts',(44.1153044501575,43.0480017357906,49.625952362208));
#33986=CARTESIAN_POINT('Ctrl Pts',(44.1671258703585,43.052040096036,49.5712831635585));
#33987=CARTESIAN_POINT('Ctrl Pts',(44.2162553053429,43.0560784562813,49.5142141233452));
#33988=CARTESIAN_POINT('Ctrl Pts',(44.2624788046377,43.0601168165267,49.4550474711072));
#33989=CARTESIAN_POINT('Ctrl Pts',(44.3109587895019,43.064352316793,49.3929924893615));
#33990=CARTESIAN_POINT('Ctrl Pts',(44.3564261600119,43.0685878170593,49.3283939845637));
#33991=CARTESIAN_POINT('Ctrl Pts',(44.398603201491,43.0728233173255,49.2615766658789));
#33992=CARTESIAN_POINT('Ctrl Pts',(44.4407190996474,43.0770526774608,49.1948562110975));
#33993=CARTESIAN_POINT('Ctrl Pts',(44.4795538926046,43.0812820375961,49.1259237235177));
#33994=CARTESIAN_POINT('Ctrl Pts',(44.5148707836607,43.0855113977314,49.0551360146058));
#33995=CARTESIAN_POINT('Ctrl Pts',(44.5501464319103,43.0897358188509,48.9844309710616));
#33996=CARTESIAN_POINT('Ctrl Pts',(44.5819121335306,43.0939602399704,48.9118754292533));
#33997=CARTESIAN_POINT('Ctrl Pts',(44.6099758110708,43.0981846610899,48.8378528244162));
#33998=CARTESIAN_POINT('Ctrl Pts',(44.6380215424196,43.102406380772,48.7638775556357));
#33999=CARTESIAN_POINT('Ctrl Pts',(44.6623697824841,43.106628100454,48.6884375235558));
#34000=CARTESIAN_POINT('Ctrl Pts',(44.6828761148751,43.1108498201361,48.611937157748));
#34001=CARTESIAN_POINT('Ctrl Pts',(44.7033757376855,43.1150701584902,48.5354618225191));
#34002=CARTESIAN_POINT('Ctrl Pts',(44.7200358274869,43.1192904968444,48.4579272954668));
#34003=CARTESIAN_POINT('Ctrl Pts',(44.7327619386732,43.1235108351986,48.3797527858724));
#34004=CARTESIAN_POINT('Ctrl Pts',(44.7454878600298,43.1277311105999,48.3015794423715));
#34005=CARTESIAN_POINT('Ctrl Pts',(44.7542798453204,43.1319513860012,48.2227665987723));
#34006=CARTESIAN_POINT('Ctrl Pts',(44.7590948988036,43.1361716614025,48.1437417800744));
#34007=CARTESIAN_POINT('Ctrl Pts',(44.763914768462,43.1403961580624,48.0646379181482));
#34008=CARTESIAN_POINT('Ctrl Pts',(44.7647497314263,43.1446206547222,47.9853221271795));
#34009=CARTESIAN_POINT('Ctrl Pts',(44.7616089020215,43.1488451513821,47.9062245512258));
#34010=CARTESIAN_POINT('Ctrl Pts',(44.7584665647128,43.1530716762118,47.8270890007326));
#34011=CARTESIAN_POINT('Ctrl Pts',(44.7513446747799,43.1572982010414,47.7481723420521));
#34012=CARTESIAN_POINT('Ctrl Pts',(44.7403042931064,43.1615247258711,47.6698996265256));
#34013=CARTESIAN_POINT('Ctrl Pts',(44.7292437299852,43.1657589766465,47.5914838310992));
#34014=CARTESIAN_POINT('Ctrl Pts',(44.7142504511103,43.1699932274218,47.5137147930387));
#34015=CARTESIAN_POINT('Ctrl Pts',(44.6954366803258,43.1742274781972,47.43700720474));
#34016=CARTESIAN_POINT('Ctrl Pts',(44.6774932971803,43.1782658384423,47.3638483647189));
#34017=CARTESIAN_POINT('Ctrl Pts',(44.6560752388336,43.1823041986874,47.2916552659579));
#34018=CARTESIAN_POINT('Ctrl Pts',(44.6313209434258,43.1863425589325,47.2207713504179));
#34019=CARTESIAN_POINT('Ctrl Pts',(44.6053582213241,43.1905780591987,47.1464271054972));
#34020=CARTESIAN_POINT('Ctrl Pts',(44.5756265262222,43.194813559465,47.0732405294778));
#34021=CARTESIAN_POINT('Ctrl Pts',(44.5422487063644,43.1990490597312,47.0016208530922));
#34022=CARTESIAN_POINT('Ctrl Pts',(44.5089192737509,43.2032784198664,46.9301050025045));
#34023=CARTESIAN_POINT('Ctrl Pts',(44.471954409482,43.2075077800017,46.8601519625604));
#34024=CARTESIAN_POINT('Ctrl Pts',(44.4315260970149,43.2117371401369,46.7921539178988));
#34025=CARTESIAN_POINT('Ctrl Pts',(44.3911449964349,43.2159615612564,46.7242352808553));
#34026=CARTESIAN_POINT('Ctrl Pts',(44.3473087236237,43.2201859823759,46.6582675036271));
#34027=CARTESIAN_POINT('Ctrl Pts',(44.3002358461097,43.2244104034953,46.5946195639402));
#34028=CARTESIAN_POINT('Ctrl Pts',(44.2531930708112,43.2286321231773,46.5310123259077));
#34029=CARTESIAN_POINT('Ctrl Pts',(44.2029180771509,43.2328538428593,46.4697223573419));
#34030=CARTESIAN_POINT('Ctrl Pts',(44.1496728737119,43.2370755625414,46.4110899094358));
#34031=CARTESIAN_POINT('Ctrl Pts',(44.0964450918662,43.2412959008955,46.3524766458054));
#34032=CARTESIAN_POINT('Ctrl Pts',(44.0402493452888,43.2455162392496,46.2965195234357));
#34033=CARTESIAN_POINT('Ctrl Pts',(43.9813871064818,43.2497365776038,46.2435247623855));
#34034=CARTESIAN_POINT('Ctrl Pts',(43.9225257456961,43.253956853005,46.190530791834));
#34035=CARTESIAN_POINT('Ctrl Pts',(43.8609983214482,43.2581771284063,46.1404994078151));
#34036=CARTESIAN_POINT('Ctrl Pts',(43.7971411339319,43.2623974038076,46.0936980583403));
#34037=CARTESIAN_POINT('Ctrl Pts',(43.7332200743519,43.2666219004674,46.0468498966131));
#34038=CARTESIAN_POINT('Ctrl Pts',(43.6669649758922,43.2708463971272,46.0032385014496));
#34039=CARTESIAN_POINT('Ctrl Pts',(43.59874253255,43.275070893787,45.9630889117206));
#34040=CARTESIAN_POINT('Ctrl Pts',(43.5304873357912,43.2792974186167,45.9229200462786));
#34041=CARTESIAN_POINT('Ctrl Pts',(43.4602633290897,43.2835239434463,45.886216514893));
#34042=CARTESIAN_POINT('Ctrl Pts',(43.3884610259716,43.2877504682759,45.8531569128054));
#34043=CARTESIAN_POINT('Ctrl Pts',(43.3165274706505,43.2919847190512,45.8200368788735));
#34044=CARTESIAN_POINT('Ctrl Pts',(43.2430102906739,43.2962189698265,45.7905742594983));
#34045=CARTESIAN_POINT('Ctrl Pts',(43.1683189661304,43.3004532206019,45.7648990163341));
#34046=CARTESIAN_POINT('Ctrl Pts',(43.0970831107861,43.3044915808474,45.7404115953498));
#34047=CARTESIAN_POINT('Ctrl Pts',(43.0247797012346,43.3085299410929,45.7193689315346));
#34048=CARTESIAN_POINT('Ctrl Pts',(42.9517724756598,43.3125683013385,45.7018403937054));
#34049=CARTESIAN_POINT('Ctrl Pts',(42.8752012674076,43.3168038016047,45.6834561678988));
#34050=CARTESIAN_POINT('Ctrl Pts',(42.7975647088768,43.3210393018709,45.6688680431903));
#34051=CARTESIAN_POINT('Ctrl Pts',(42.7192734344537,43.3252748021371,45.6581940911015));
#34052=CARTESIAN_POINT('Ctrl Pts',(42.641095657528,43.3295041622723,45.6475356128552));
#34053=CARTESIAN_POINT('Ctrl Pts',(42.5622655106308,43.3337335224075,45.6407801019222));
#34054=CARTESIAN_POINT('Ctrl Pts',(42.4832058736375,43.3379628825428,45.6379950839399));
#34055=CARTESIAN_POINT('Ctrl Pts',(42.4042385619087,43.3421873036622,45.6352133182812));
#34056=CARTESIAN_POINT('Ctrl Pts',(42.3250427592673,43.3464117247817,45.636392848));
#34057=CARTESIAN_POINT('Ctrl Pts',(42.2460470295097,43.3506361459011,45.6415494654801));
#34058=CARTESIAN_POINT('Ctrl Pts',(42.167101816028,43.3548578655831,45.6467027854008));
#34059=CARTESIAN_POINT('Ctrl Pts',(42.0883568885804,43.3590795852651,45.6558281147404));
#34060=CARTESIAN_POINT('Ctrl Pts',(42.010240152383,43.3633013049471,45.6688891699266));
#34061=CARTESIAN_POINT('Ctrl Pts',(41.9321489756339,43.3675216433012,45.6819459515936));
#34062=CARTESIAN_POINT('Ctrl Pts',(41.8546860445732,43.3717419816554,45.6989358247166));
#34063=CARTESIAN_POINT('Ctrl Pts',(41.7782719929229,43.3759623200095,45.7197709049054));
#34064=CARTESIAN_POINT('Ctrl Pts',(41.7018590811062,43.3801825954107,45.7406056743068));
#34065=CARTESIAN_POINT('Ctrl Pts',(41.62649547007,43.384402870812,45.7652854120072));
#34066=CARTESIAN_POINT('Ctrl Pts',(41.5525880266408,43.3886231462132,45.7936719672027));
#34067=CARTESIAN_POINT('Ctrl Pts',(41.4786066585505,43.392847642873,45.8220869155663));
#34068=CARTESIAN_POINT('Ctrl Pts',(41.4060848068154,43.3970721395328,45.8542159192995));
#34069=CARTESIAN_POINT('Ctrl Pts',(41.3354101137736,43.4012966361926,45.8898723225728));
#34070=CARTESIAN_POINT('Ctrl Pts',(41.2647014899964,43.4055231610223,45.9255458443921));
#34071=CARTESIAN_POINT('Ctrl Pts',(41.1958421999975,43.4097496858519,45.9647499068625));
#34072=CARTESIAN_POINT('Ctrl Pts',(41.1291937118813,43.4139762106815,46.0072526956541));
#34073=CARTESIAN_POINT('Ctrl Pts',(41.0624233925633,43.4182104614568,46.0498331781186));
#34074=CARTESIAN_POINT('Ctrl Pts',(40.9978723340775,43.4224447122321,46.095724163513));
#34075=CARTESIAN_POINT('Ctrl Pts',(40.9358713630654,43.4266789630074,46.144651575739));
#34076=CARTESIAN_POINT('Ctrl Pts',(40.8767387632706,43.430717323253,46.1913154430772));
#34077=CARTESIAN_POINT('Ctrl Pts',(40.819925763197,43.4347556834987,46.2407407377773));
#34078=CARTESIAN_POINT('Ctrl Pts',(40.7656874832283,43.4387940437443,46.2926590737573));
#34079=CARTESIAN_POINT('Ctrl Pts',(40.7086184111207,43.4430431731818,46.34728711988));
#34080=CARTESIAN_POINT('Ctrl Pts',(40.6541653394365,43.4472923026193,46.40490063856));
#34081=CARTESIAN_POINT('Ctrl Pts',(40.6026626588428,43.4515414320569,46.4652137207474));
#34082=CARTESIAN_POINT('Ctrl Pts',(40.5521635800498,43.4557077612614,46.5243515181305));
#34083=CARTESIAN_POINT('Ctrl Pts',(40.5045013028056,43.4598740904658,46.5860842540786));
#34084=CARTESIAN_POINT('Ctrl Pts',(40.4599566629003,43.4640404196703,46.6501028590759));
#34085=CARTESIAN_POINT('Ctrl Pts',(40.4154544564735,43.4682027800058,46.7140604795843));
#34086=CARTESIAN_POINT('Ctrl Pts',(40.3740642728014,43.4723651403413,46.7802992556056));
#34087=CARTESIAN_POINT('Ctrl Pts',(40.3360268850936,43.4765275006768,46.8484769121534));
#34088=CARTESIAN_POINT('Ctrl Pts',(40.298013037963,43.4806872850109,46.9166123749156));
#34089=CARTESIAN_POINT('Ctrl Pts',(40.2633481050394,43.484847069345,46.9866839154094));
#34090=CARTESIAN_POINT('Ctrl Pts',(40.2322287563103,43.489006853679,47.0583215644755));
#34091=CARTESIAN_POINT('Ctrl Pts',(40.1999567820551,43.4933207117262,47.1326125911449));
#34092=CARTESIAN_POINT('Ctrl Pts',(40.1714984602697,43.4976345697733,47.2085875394332));
#34093=CARTESIAN_POINT('Ctrl Pts',(40.1470194300474,43.5019484278204,47.2858088544962));
#34094=CARTESIAN_POINT('Ctrl Pts',(40.123410782464,43.5061089012311,47.360284468795));
#34095=CARTESIAN_POINT('Ctrl Pts',(40.1035033133508,43.5102693746418,47.4359188077746));
#34096=CARTESIAN_POINT('Ctrl Pts',(40.0873947493397,43.5144298480525,47.5123039927183));
#34097=CARTESIAN_POINT('Ctrl Pts',(40.0712812845998,43.5185915872093,47.588712416424));
#34098=CARTESIAN_POINT('Ctrl Pts',(40.0589691050863,43.5227533263661,47.6658716630413));
#34099=CARTESIAN_POINT('Ctrl Pts',(40.0505044774577,43.5269150655229,47.7433655704048));
#34100=CARTESIAN_POINT('Ctrl Pts',(40.0420309912486,43.5310811601107,47.8209405783258));
#34101=CARTESIAN_POINT('Ctrl Pts',(40.0374131159821,43.5352472546985,47.8988504628412));
#34102=CARTESIAN_POINT('Ctrl Pts',(40.0366450790482,43.5394133492862,47.9766770818087));
#34103=CARTESIAN_POINT('Ctrl Pts',(40.0365615173866,43.5398666162724,47.9851445412663));
#34104=CARTESIAN_POINT('Ctrl Pts',(40.0365234764394,43.5403198832585,47.9936110186486));
#34105=CARTESIAN_POINT('Ctrl Pts',(40.0365309117291,43.5407731502446,48.0020759787561));
#34106=CARTESIAN_POINT('',(40.0365303613413,44.3345231503005,47.9986930805401));
#34107=CARTESIAN_POINT('Ctrl Pts',(40.0365309117295,43.5407731502717,48.0020759792626));
#34108=CARTESIAN_POINT('Ctrl Pts',(40.0366326946382,43.546977995395,48.1179541880231));
#34109=CARTESIAN_POINT('Ctrl Pts',(40.0452598640996,43.5531828405182,48.233471756771));
#34110=CARTESIAN_POINT('Ctrl Pts',(40.0622349480595,43.5593876856415,48.3476276784514));
#34111=CARTESIAN_POINT('Ctrl Pts',(40.0673710085148,43.5612650524777,48.3821672257353));
#34112=CARTESIAN_POINT('Ctrl Pts',(40.0732709855902,43.5631424193139,48.4165823443543));
#34113=CARTESIAN_POINT('Ctrl Pts',(40.0799291996866,43.5650197861502,48.4508457856444));
#34114=CARTESIAN_POINT('Ctrl Pts',(40.0949507005634,43.5692552864162,48.5281470417959));
#34115=CARTESIAN_POINT('Ctrl Pts',(40.1138683244528,43.5734907866822,48.6048436656388));
#34116=CARTESIAN_POINT('Ctrl Pts',(40.1366192416652,43.5777262869483,48.6805130297796));
#34117=CARTESIAN_POINT('Ctrl Pts',(40.159337177269,43.5819556470833,48.7560726973607));
#34118=CARTESIAN_POINT('Ctrl Pts',(40.1858772368616,43.5861850072183,48.8306076168557));
#34119=CARTESIAN_POINT('Ctrl Pts',(40.2161255174371,43.5904143673534,48.9037049769203));
#34120=CARTESIAN_POINT('Ctrl Pts',(40.2463384742922,43.5946387884726,48.9767169744236));
#34121=CARTESIAN_POINT('Ctrl Pts',(40.2802508682226,43.5988632095919,49.0482943170942));
#34122=CARTESIAN_POINT('Ctrl Pts',(40.3176993632225,43.6030876307111,49.1180404728702));
#34123=CARTESIAN_POINT('Ctrl Pts',(40.3551239106177,43.6073093503929,49.187742027298));
#34124=CARTESIAN_POINT('Ctrl Pts',(40.3960798495183,43.6115310700747,49.2556143066362));
#34125=CARTESIAN_POINT('Ctrl Pts',(40.4403567290258,43.6157527897565,49.3212829717458));
#34126=CARTESIAN_POINT('Ctrl Pts',(40.4846191213355,43.6199731281105,49.3869301503607));
#34127=CARTESIAN_POINT('Ctrl Pts',(40.5322000344415,43.6241934664644,49.4503747575766));
#34128=CARTESIAN_POINT('Ctrl Pts',(40.5828450770055,43.6284138048183,49.5112704677644));
#34129=CARTESIAN_POINT('Ctrl Pts',(40.6334893641205,43.6326340802194,49.5721652695987));
#34130=CARTESIAN_POINT('Ctrl Pts',(40.6871973886971,43.6368543556204,49.630510889974));
#34131=CARTESIAN_POINT('Ctrl Pts',(40.7436747265954,43.6410746310215,49.685994374125));
#34132=CARTESIAN_POINT('Ctrl Pts',(40.8002085549886,43.6452991276811,49.7415333546857));
#34133=CARTESIAN_POINT('Ctrl Pts',(40.8595168944304,43.6495236243407,49.7942041505038));
#34134=CARTESIAN_POINT('Ctrl Pts',(40.9212691538297,43.6537481210003,49.843731413597));
#34135=CARTESIAN_POINT('Ctrl Pts',(40.9830510603273,43.6579746458298,49.8932824545998));
#34136=CARTESIAN_POINT('Ctrl Pts',(41.0472788432116,43.6622011706592,49.9396866811162));
#34137=CARTESIAN_POINT('Ctrl Pts',(41.1135916714608,43.6664276954886,49.9827112884041));
#34138=CARTESIAN_POINT('Ctrl Pts',(41.1800257173371,43.6706619462637,50.0258145432318));
#34139=CARTESIAN_POINT('Ctrl Pts',(41.2485520174761,43.6748961970388,50.0655255981262));
#34140=CARTESIAN_POINT('Ctrl Pts',(41.3187839892539,43.679130447814,50.1016570555174));
#34141=CARTESIAN_POINT('Ctrl Pts',(41.3857667963626,43.6831688080613,50.1361169514841));
#34142=CARTESIAN_POINT('Ctrl Pts',(41.4543006048555,43.6872071683086,50.1673210190355));
#34143=CARTESIAN_POINT('Ctrl Pts',(41.5240354019836,43.691245528556,50.1951483922328));
#34144=CARTESIAN_POINT('Ctrl Pts',(41.5971744321095,43.695481028822,50.2243342100801));
#34145=CARTESIAN_POINT('Ctrl Pts',(41.6719127188849,43.6997165290881,50.2499161781902));
#34146=CARTESIAN_POINT('Ctrl Pts',(41.7478608304828,43.7039520293542,50.2717185002727));
#34147=CARTESIAN_POINT('Ctrl Pts',(41.8236988414257,43.7081813894892,50.2934892159086));
#34148=CARTESIAN_POINT('Ctrl Pts',(41.9007427470158,43.7124107496243,50.3114910380031));
#34149=CARTESIAN_POINT('Ctrl Pts',(41.9785837407698,43.7166401097594,50.3255964347574));
#34150=CARTESIAN_POINT('Ctrl Pts',(42.0563338323817,43.7208645308787,50.3396853593327));
#34151=CARTESIAN_POINT('Ctrl Pts',(42.1348787029864,43.725088951998,50.3498868174432));
#34152=CARTESIAN_POINT('Ctrl Pts',(42.2137964946016,43.7293133731173,50.3561236587831));
#34153=CARTESIAN_POINT('Ctrl Pts',(42.2926638197806,43.7335350927991,50.3623565117808));
#34154=CARTESIAN_POINT('Ctrl Pts',(42.3719031260178,43.7377568124809,50.364629743154));
#34155=CARTESIAN_POINT('Ctrl Pts',(42.4510857314457,43.7419785321628,50.3629178337265));
#34156=CARTESIAN_POINT('Ctrl Pts',(42.5302424286777,43.7461988705167,50.3612064844281));
#34157=CARTESIAN_POINT('Ctrl Pts',(42.6093419930523,43.7504192088707,50.3555125936196));
#34158=CARTESIAN_POINT('Ctrl Pts',(42.6879555314468,43.7546395472246,50.3458627523385));
#34159=CARTESIAN_POINT('Ctrl Pts',(42.7665678971988,43.7588598226257,50.3362130549997));
#34160=CARTESIAN_POINT('Ctrl Pts',(42.8446937856893,43.7630800980268,50.3226075829935));
#34161=CARTESIAN_POINT('Ctrl Pts',(42.9219107122232,43.7673003734279,50.3051246494206));
#34162=CARTESIAN_POINT('Ctrl Pts',(42.9992048736722,43.7715248700875,50.2876242288414));
#34163=CARTESIAN_POINT('Ctrl Pts',(43.0755877981171,43.7757493667472,50.2662387030641));
#34164=CARTESIAN_POINT('Ctrl Pts',(43.1506490632099,43.7799738634068,50.2410971475601));
#34165=CARTESIAN_POINT('Ctrl Pts',(43.2257463650198,43.7842003882363,50.2159435216611));
#34166=CARTESIAN_POINT('Ctrl Pts',(43.2995203058357,43.7884269130657,50.1870304452184));
#34167=CARTESIAN_POINT('Ctrl Pts',(43.3715798838236,43.7926534378952,50.1545354418643));
#34168=CARTESIAN_POINT('Ctrl Pts',(43.4437711843042,43.7968876886703,50.1219810387335));
#34169=CARTESIAN_POINT('Ctrl Pts',(43.5142414411835,43.8011219394454,50.0858318397518));
#34170=CARTESIAN_POINT('Ctrl Pts',(43.5826239099361,43.8053561902206,50.0463115912655));
#34171=CARTESIAN_POINT('Ctrl Pts',(43.6478427781782,43.8093945504677,50.0086196809566));
#34172=CARTESIAN_POINT('Ctrl Pts',(43.7111624818923,43.8134329107148,49.9678619594898));
#34173=CARTESIAN_POINT('Ctrl Pts',(43.7722920155135,43.8174712709618,49.9242674099662));
#34174=CARTESIAN_POINT('Ctrl Pts',(43.836405700318,43.8217067712294,49.8785447119219));
#34175=CARTESIAN_POINT('Ctrl Pts',(43.8983536305805,43.825942271497,49.8295273421116));
#34176=CARTESIAN_POINT('Ctrl Pts',(43.9577772773827,43.8301777717645,49.7774477193353));
#34177=CARTESIAN_POINT('Ctrl Pts',(44.0171147787588,43.8344071319011,49.7254435954812));
#34178=CARTESIAN_POINT('Ctrl Pts',(44.073934913626,43.8386364920377,49.6703863410523));
#34179=CARTESIAN_POINT('Ctrl Pts',(44.1279092633336,43.8428658521743,49.6125507801573));
#34180=CARTESIAN_POINT('Ctrl Pts',(44.1818205821912,43.8470902732951,49.5547827592063));
#34181=CARTESIAN_POINT('Ctrl Pts',(44.232892401313,43.8513146944159,49.4942432205423));
#34182=CARTESIAN_POINT('Ctrl Pts',(44.2808316135483,43.8555391155367,49.4312452209098));
#34183=CARTESIAN_POINT('Ctrl Pts',(44.3287401695636,43.85976083522,49.3682875073074));
#34184=CARTESIAN_POINT('Ctrl Pts',(44.3735198112441,43.8639825549034,49.3028748255943));
#34185=CARTESIAN_POINT('Ctrl Pts',(44.4149171630047,43.8682042745867,49.2353539035958));
#34186=CARTESIAN_POINT('Ctrl Pts',(44.456300969736,43.8724246129422,49.1678550741423));
#34187=CARTESIAN_POINT('Ctrl Pts',(44.4943044388895,43.8766449512977,49.098249773962));
#34188=CARTESIAN_POINT('Ctrl Pts',(44.5287179067445,43.8808652896531,49.026913099734));
#34189=CARTESIAN_POINT('Ctrl Pts',(44.5631308612694,43.8850855650557,48.9555774896029));
#34190=CARTESIAN_POINT('Ctrl Pts',(44.5939537182137,43.8893058404583,48.8825109800734));
#34191=CARTESIAN_POINT('Ctrl Pts',(44.6210237804686,43.8935261158609,48.8081112593529));
#34192=CARTESIAN_POINT('Ctrl Pts',(44.6481209190919,43.897750612522,48.7336371215798));
#34193=CARTESIAN_POINT('Ctrl Pts',(44.6714576037361,43.9019751091832,48.6578275508552));
#34194=CARTESIAN_POINT('Ctrl Pts',(44.6909203554978,43.9061996058443,48.5810975526244));
#34195=CARTESIAN_POINT('Ctrl Pts',(44.7103924512756,43.9104261306752,48.5043307165222));
#34196=CARTESIAN_POINT('Ctrl Pts',(44.7259868165942,43.9146526555062,48.4266430334096));
#34197=CARTESIAN_POINT('Ctrl Pts',(44.7376412251462,43.9188791803371,48.3484593855776));
#34198=CARTESIAN_POINT('Ctrl Pts',(44.7493169375662,43.9231134311137,48.270132820659));
#34199=CARTESIAN_POINT('Ctrl Pts',(44.7570382558388,43.9273476818903,48.191308947752));
#34200=CARTESIAN_POINT('Ctrl Pts',(44.7607949512539,43.9315819326669,48.1124172541651));
#34201=CARTESIAN_POINT('Ctrl Pts',(44.7643778494276,43.9356202929005,48.0371753530702));
#34202=CARTESIAN_POINT('Ctrl Pts',(44.7643548825488,43.9396586531341,47.9618721249029));
#34203=CARTESIAN_POINT('Ctrl Pts',(44.7607612002978,43.9436970133677,47.886876191416));
#34204=CARTESIAN_POINT('Ctrl Pts',(44.7569920857951,43.9479325136319,47.8082191926045));
#34205=CARTESIAN_POINT('Ctrl Pts',(44.7492804050985,43.9521680138961,47.7296012647612));
#34206=CARTESIAN_POINT('Ctrl Pts',(44.737627667848,43.9564035141602,47.6514496773612));
#34207=CARTESIAN_POINT('Ctrl Pts',(44.7259918233678,43.9606328742934,47.5734113849567));
#34208=CARTESIAN_POINT('Ctrl Pts',(44.7104263365325,43.9648622344266,47.4958385507813));
#34209=CARTESIAN_POINT('Ctrl Pts',(44.6909846704357,43.9690915945598,47.4191560616409));
#34210=CARTESIAN_POINT('Ctrl Pts',(44.6715657081741,43.9733160156772,47.3425631217491));
#34211=CARTESIAN_POINT('Ctrl Pts',(44.6482796765435,43.9775404367947,47.2668589133324));
#34212=CARTESIAN_POINT('Ctrl Pts',(44.6212312965784,43.9817648579121,47.1924593087648));
#34213=CARTESIAN_POINT('Ctrl Pts',(44.594200213541,43.9859865775921,47.1181072813378));
#34214=CARTESIAN_POINT('Ctrl Pts',(44.5634117173996,43.9902082972721,47.0450586418268));
#34215=CARTESIAN_POINT('Ctrl Pts',(44.529020341951,43.9944300169521,46.9737140630122));
#34216=CARTESIAN_POINT('Ctrl Pts',(44.4946402192072,43.9986503553042,46.9023928278259));
#34217=CARTESIAN_POINT('Ctrl Pts',(44.4566597616052,44.0028706936563,46.8327749686778));
#34218=CARTESIAN_POINT('Ctrl Pts',(44.4152810096909,44.0070910320084,46.765239742752));
#34219=CARTESIAN_POINT('Ctrl Pts',(44.3739028750046,44.0113113074077,46.6977055242182));
#34220=CARTESIAN_POINT('Ctrl Pts',(44.3291267931115,44.015531582807,46.632254276664));
#34221=CARTESIAN_POINT('Ctrl Pts',(44.2811992132045,44.0197518582062,46.5692379788592));
#34222=CARTESIAN_POINT('Ctrl Pts',(44.2332236945518,44.0239763548641,46.5061586500757));
#34223=CARTESIAN_POINT('Ctrl Pts',(44.1820906657114,44.028200851522,46.4455195107658));
#34224=CARTESIAN_POINT('Ctrl Pts',(44.1280877667894,44.0324253481799,46.3876405142857));
#34225=CARTESIAN_POINT('Ctrl Pts',(44.0740589412166,44.0366518730075,46.3297337302505));
#34226=CARTESIAN_POINT('Ctrl Pts',(44.0171578382906,44.0408783978352,46.2745900559656));
#34227=CARTESIAN_POINT('Ctrl Pts',(43.95770813204,44.0451049226629,46.2224916832047));
#34228=CARTESIAN_POINT('Ctrl Pts',(43.8981497537186,44.0493391734364,46.1702980763643));
#34229=CARTESIAN_POINT('Ctrl Pts',(43.8360338318456,44.0535734242098,46.1211611865935));
#34230=CARTESIAN_POINT('Ctrl Pts',(43.771716043656,44.0578076749833,46.0753219655027));
#34231=CARTESIAN_POINT('Ctrl Pts',(43.7103738100583,44.0618460352467,46.0316034190904));
#34232=CARTESIAN_POINT('Ctrl Pts',(43.6470292563365,44.0658843955101,45.9908843290108));
#34233=CARTESIAN_POINT('Ctrl Pts',(43.5820114194165,44.0699227557735,45.9533345546307));
#34234=CARTESIAN_POINT('Ctrl Pts',(43.5138196169086,44.0741582560391,45.9139517187806));
#34235=CARTESIAN_POINT('Ctrl Pts',(43.443527779424,44.0783937563046,45.8779058288163));
#34236=CARTESIAN_POINT('Ctrl Pts',(43.3714960692856,44.0826292565701,45.8454267642378));
#34237=CARTESIAN_POINT('Ctrl Pts',(43.2995687822636,44.0868586167047,45.812994783994));
#34238=CARTESIAN_POINT('Ctrl Pts',(43.2259070556054,44.0910879768392,45.7841195522038));
#34239=CARTESIAN_POINT('Ctrl Pts',(43.1508971541187,44.0953173369737,45.7589859650514));
#34240=CARTESIAN_POINT('Ctrl Pts',(43.0759748486458,44.0995417580924,45.7338817287181));
#34241=CARTESIAN_POINT('Ctrl Pts',(42.9997079396694,44.1037661792111,45.7125106024248));
#34242=CARTESIAN_POINT('Ctrl Pts',(42.9225028407167,44.1079906003299,45.6950094962575));
#34243=CARTESIAN_POINT('Ctrl Pts',(42.8453471129659,44.1122123200111,45.6775195817169));
#34244=CARTESIAN_POINT('Ctrl Pts',(42.7672548425226,44.1164340396924,45.6638948788254));
#34245=CARTESIAN_POINT('Ctrl Pts',(42.6886466079096,44.1206557593736,45.6542221808871));
#34246=CARTESIAN_POINT('Ctrl Pts',(42.6100640935613,44.1248760977269,45.6445526478124));
#34247=CARTESIAN_POINT('Ctrl Pts',(42.5309664157519,44.1290964360803,45.6388326093437));
#34248=CARTESIAN_POINT('Ctrl Pts',(42.4517818426335,44.1333167744336,45.6370973186199));
#34249=CARTESIAN_POINT('Ctrl Pts',(42.3725984506758,44.1375370498341,45.6353620537806));
#34250=CARTESIAN_POINT('Ctrl Pts',(42.2933286352536,44.1417573252345,45.6376114274847));
#34251=CARTESIAN_POINT('Ctrl Pts',(42.2144017473073,44.145977600635,45.6438285865631));
#34252=CARTESIAN_POINT('Ctrl Pts',(42.1353959140864,44.150202097294,45.6500519642489));
#34253=CARTESIAN_POINT('Ctrl Pts',(42.0567341625618,44.154426593953,45.6602510183619));
#34254=CARTESIAN_POINT('Ctrl Pts',(41.9788411933351,44.158651090612,45.6743569275427));
#34255=CARTESIAN_POINT('Ctrl Pts',(41.9009108278979,44.1628776154408,45.6884696089336));
#34256=CARTESIAN_POINT('Ctrl Pts',(41.8237504377088,44.1671041402696,45.7064927750539));
#34257=CARTESIAN_POINT('Ctrl Pts',(41.7477724588646,44.1713306650983,45.7283068703092));
#34258=CARTESIAN_POINT('Ctrl Pts',(41.6716555948225,44.1755649158728,45.7501608409993));
#34259=CARTESIAN_POINT('Ctrl Pts',(41.5967259063327,44.1797991666473,45.7758194355191));
#34260=CARTESIAN_POINT('Ctrl Pts',(41.5233784588197,44.1840334174217,45.8051138721021));
#34261=CARTESIAN_POINT('Ctrl Pts',(41.4534243081469,44.1880717776743,45.8330530506295));
#34262=CARTESIAN_POINT('Ctrl Pts',(41.3849095462803,44.1921101379269,45.8642989169101));
#34263=CARTESIAN_POINT('Ctrl Pts',(41.3181550358887,44.1961484981794,45.898666634128));
#34264=CARTESIAN_POINT('Ctrl Pts',(41.2481417806304,44.2003839984554,45.9347120750144));
#34265=CARTESIAN_POINT('Ctrl Pts',(41.1797988894822,44.2046194987314,45.9743289635968));
#34266=CARTESIAN_POINT('Ctrl Pts',(41.1135145423081,44.2088549990074,46.017338756104));
#34267=CARTESIAN_POINT('Ctrl Pts',(41.0473262863973,44.2130843591525,46.0602861980643));
#34268=CARTESIAN_POINT('Ctrl Pts',(40.9831910386942,44.2173137192975,46.1066165230949));
#34269=CARTESIAN_POINT('Ctrl Pts',(40.9214732680534,44.2215430794425,46.1561048989112));
#34270=CARTESIAN_POINT('Ctrl Pts',(40.8598275709725,44.2257675005718,46.2055354825652));
#34271=CARTESIAN_POINT('Ctrl Pts',(40.8005941051742,44.2299919217011,46.2581164962757));
#34272=CARTESIAN_POINT('Ctrl Pts',(40.7441078821434,44.2342163428303,46.3135802020492));
#34273=CARTESIAN_POINT('Ctrl Pts',(40.6876577809846,44.2384380625221,46.3690084398312));
#34274=CARTESIAN_POINT('Ctrl Pts',(40.6339517696957,44.242659782214,46.4273153829194));
#34275=CARTESIAN_POINT('Ctrl Pts',(40.5832903732837,44.2468815019058,46.4881942674086));
#34276=CARTESIAN_POINT('Ctrl Pts',(40.532645553055,44.2511018402697,46.5490532325979));
#34277=CARTESIAN_POINT('Ctrl Pts',(40.4850436696072,44.2553221786336,46.6124821076934));
#34278=CARTESIAN_POINT('Ctrl Pts',(40.4407460612456,44.2595425169975,46.6781397788059));
#34279=CARTESIAN_POINT('Ctrl Pts',(40.3964491136516,44.2637627924085,46.7437964705323));
#34280=CARTESIAN_POINT('Ctrl Pts',(40.3554566045661,44.2679830678196,46.8116815023639));
#34281=CARTESIAN_POINT('Ctrl Pts',(40.3179866352061,44.2722033432306,46.8814246606869));
#34282=CARTESIAN_POINT('Ctrl Pts',(40.2804791871488,44.2764278399,46.9512375784136));
#34283=CARTESIAN_POINT('Ctrl Pts',(40.2465015398371,44.2806523365695,47.0229119208925));
#34284=CARTESIAN_POINT('Ctrl Pts',(40.2162255719881,44.284876833239,47.0960532712261));
#34285=CARTESIAN_POINT('Ctrl Pts',(40.1859350687264,44.2891033580782,47.1692297365297));
#34286=CARTESIAN_POINT('Ctrl Pts',(40.1593499429503,44.2933298829174,47.2438741699996));
#34287=CARTESIAN_POINT('Ctrl Pts',(40.1365927694682,44.2975564077566,47.319575022742));
#34288=CARTESIAN_POINT('Ctrl Pts',(40.1137939966372,44.3017906585413,47.3954142541016));
#34289=CARTESIAN_POINT('Ctrl Pts',(40.0948372711182,44.3060249093261,47.4723133066147));
#34290=CARTESIAN_POINT('Ctrl Pts',(40.0797943697413,44.3102591601108,47.5498486096703));
#34291=CARTESIAN_POINT('Ctrl Pts',(40.0654474033776,44.3142975202689,47.6237968698538));
#34292=CARTESIAN_POINT('Ctrl Pts',(40.0546601511491,44.3183358804271,47.6983234535545));
#34293=CARTESIAN_POINT('Ctrl Pts',(40.0474507440786,44.3223742405853,47.7730585111452));
#34294=CARTESIAN_POINT('Ctrl Pts',(40.0402212060184,44.3264238771474,47.84800225312));
#34295=CARTESIAN_POINT('Ctrl Pts',(40.0365720529249,44.3304735137096,47.9232968877507));
#34296=CARTESIAN_POINT('Ctrl Pts',(40.0365303613416,44.3345231502717,47.9986930800047));
#34297=CARTESIAN_POINT('',(40.0365304116029,45.1282731502432,47.9986051444044));
#34298=CARTESIAN_POINT('Ctrl Pts',(40.0365303613413,44.3345231503005,47.9986930805401));
#34299=CARTESIAN_POINT('Ctrl Pts',(40.0364873138526,44.3387044920006,48.0765413609645));
#34300=CARTESIAN_POINT('Ctrl Pts',(40.0402947576141,44.3428858337008,48.1545451941626));
#34301=CARTESIAN_POINT('Ctrl Pts',(40.047972454677,44.347067175401,48.2322861746675));
#34302=CARTESIAN_POINT('Ctrl Pts',(40.0557404770259,44.3512977090506,48.3109417492561));
#34303=CARTESIAN_POINT('Ctrl Pts',(40.0674704954214,44.3555282427002,48.3893277508716));
#34304=CARTESIAN_POINT('Ctrl Pts',(40.0831286024023,44.3597587763497,48.4670089591152));
#34305=CARTESIAN_POINT('Ctrl Pts',(40.0985691505288,44.3639305295825,48.5436108392703));
#34306=CARTESIAN_POINT('Ctrl Pts',(40.1178292293051,44.3681022828153,48.6195268984098));
#34307=CARTESIAN_POINT('Ctrl Pts',(40.140824253703,44.3722740360481,48.6943452946794));
#34308=CARTESIAN_POINT('Ctrl Pts',(40.1638081619622,44.376443772593,48.7691275226171));
#34309=CARTESIAN_POINT('Ctrl Pts',(40.1905232926915,44.3806135091379,48.842812680392));
#34310=CARTESIAN_POINT('Ctrl Pts',(40.2208346617081,44.3847832456828,48.9150021143622));
#34311=CARTESIAN_POINT('Ctrl Pts',(40.2511413964841,44.3889523447255,48.9871805114433));
#34312=CARTESIAN_POINT('Ctrl Pts',(40.2850430906621,44.3931214437682,49.0578631947279));
#34313=CARTESIAN_POINT('Ctrl Pts',(40.3223564941723,44.397290542811,49.1266711603622));
#34314=CARTESIAN_POINT('Ctrl Pts',(40.3606247512086,44.4015663294926,49.197239928347));
#34315=CARTESIAN_POINT('Ctrl Pts',(40.4024815024921,44.4058421161743,49.2658362304326));
#34316=CARTESIAN_POINT('Ctrl Pts',(40.4476797591311,44.410117902856,49.3320796214918));
#34317=CARTESIAN_POINT('Ctrl Pts',(40.4918069478713,44.4142923657655,49.3967532358614));
#34318=CARTESIAN_POINT('Ctrl Pts',(40.5391186654831,44.418466828675,49.4591838745681));
#34319=CARTESIAN_POINT('Ctrl Pts',(40.5893433779465,44.4226412915845,49.5190500445719));
#34320=CARTESIAN_POINT('Ctrl Pts',(40.6413966935497,44.4269677401523,49.5810958480881));
#34321=CARTESIAN_POINT('Ctrl Pts',(40.6965788149973,44.43129418872,49.6403864316954));
#34322=CARTESIAN_POINT('Ctrl Pts',(40.7545465108049,44.4356206372878,49.6966063938921));
#34323=CARTESIAN_POINT('Ctrl Pts',(40.8125142066124,44.4399470858555,49.7528263560887));
#34324=CARTESIAN_POINT('Ctrl Pts',(40.8732669979703,44.4442735344233,49.8059753825312));
#34325=CARTESIAN_POINT('Ctrl Pts',(40.936426713427,44.448599982991,49.8557865382985));
#34326=CARTESIAN_POINT('Ctrl Pts',(40.9982587189332,44.4528354832578,49.9045505904384));
#34327=CARTESIAN_POINT('Ctrl Pts',(41.0626480362529,44.4570709835245,49.950313724215));
#34328=CARTESIAN_POINT('Ctrl Pts',(41.1292712332043,44.4613064837913,49.9927967387915));
#34329=CARTESIAN_POINT('Ctrl Pts',(41.1957978476641,44.4655358439268,50.0352181664795));
#34330=CARTESIAN_POINT('Ctrl Pts',(41.2645515184387,44.4697652040624,50.0743686676054));
#34331=CARTESIAN_POINT('Ctrl Pts',(41.3351765237371,44.473994564198,50.1100098116595));
#34332=CARTESIAN_POINT('Ctrl Pts',(41.4057190536672,44.4782189853175,50.1456093342444));
#34333=CARTESIAN_POINT('Ctrl Pts',(41.4781281586208,44.482443406437,50.1777074332868));
#34334=CARTESIAN_POINT('Ctrl Pts',(41.5520212882403,44.4866678275565,50.2061102749641));
#34335=CARTESIAN_POINT('Ctrl Pts',(41.6258671645971,44.4908895472384,50.23449495356));
#34336=CARTESIAN_POINT('Ctrl Pts',(41.7011947451277,44.4951112669203,50.2591888969931));
#34337=CARTESIAN_POINT('Ctrl Pts',(41.777600266791,44.4993329866022,50.2800458357238));
#34338=CARTESIAN_POINT('Ctrl Pts',(41.8539807889048,44.503553324956,50.3008959501562));
#34339=CARTESIAN_POINT('Ctrl Pts',(41.9314380993689,44.5077736633099,50.3179114292895));
#34340=CARTESIAN_POINT('Ctrl Pts',(42.0095534264271,44.5119940016637,50.3309959060636));
#34341=CARTESIAN_POINT('Ctrl Pts',(42.0876675882715,44.5162142770645,50.344080187662));
#34342=CARTESIAN_POINT('Ctrl Pts',(42.1664392840762,44.5204345524653,50.3532335072376));
#34343=CARTESIAN_POINT('Ctrl Pts',(42.2454411905109,44.5246548278662,50.3584109089193));
#34344=CARTESIAN_POINT('Ctrl Pts',(42.3245221172514,44.5288793245253,50.3635934892084));
#34345=CARTESIAN_POINT('Ctrl Pts',(42.403833245138,44.5331038211844,50.36479217659));
#34346=CARTESIAN_POINT('Ctrl Pts',(42.4829443928394,44.5373283178435,50.3620141127005));
#34347=CARTESIAN_POINT('Ctrl Pts',(42.5620935215933,44.5415548426723,50.35923471507));
#34348=CARTESIAN_POINT('Ctrl Pts',(42.6410420106153,44.545781367501,50.3524748028493));
#34349=CARTESIAN_POINT('Ctrl Pts',(42.7193645330155,44.5500078923298,50.3417934870419));
#34350=CARTESIAN_POINT('Ctrl Pts',(42.7978302263567,44.5542421431041,50.3310926461478));
#34351=CARTESIAN_POINT('Ctrl Pts',(42.8756672041234,44.5584763938783,50.3164561648982));
#34352=CARTESIAN_POINT('Ctrl Pts',(42.9524602636344,44.5627106446525,50.2979943642239));
#34353=CARTESIAN_POINT('Ctrl Pts',(43.0257006207594,44.5667490049007,50.2803866678624));
#34354=CARTESIAN_POINT('Ctrl Pts',(43.0979911812455,44.5707873651488,50.2592999040496));
#34355=CARTESIAN_POINT('Ctrl Pts',(43.1689878718805,44.574825725397,50.2348709344839));
#34356=CARTESIAN_POINT('Ctrl Pts',(43.2434503984069,44.5790612257338,50.2092494191986));
#34357=CARTESIAN_POINT('Ctrl Pts',(43.3167725522144,44.5832967260707,50.1798536614904));
#34358=CARTESIAN_POINT('Ctrl Pts',(43.3885445434963,44.5875322264075,50.1468046316383));
#34359=CARTESIAN_POINT('Ctrl Pts',(43.4602124881788,44.5917615866137,50.1138035123863));
#34360=CARTESIAN_POINT('Ctrl Pts',(43.5303343102457,44.5959909468198,50.0771598327297));
#34361=CARTESIAN_POINT('Ctrl Pts',(43.5985170404772,44.600220307026,50.0370437758148));
#34362=CARTESIAN_POINT('Ctrl Pts',(43.666620147419,44.6044447282165,49.9969745661354));
#34363=CARTESIAN_POINT('Ctrl Pts',(43.7327882599967,44.608669149407,49.9534412740424));
#34364=CARTESIAN_POINT('Ctrl Pts',(43.796651402031,44.6128935705975,49.9066607726874));
#34365=CARTESIAN_POINT('Ctrl Pts',(43.8604737047943,44.6171152903506,49.8599101865778));
#34366=CARTESIAN_POINT('Ctrl Pts',(43.9219935849465,44.6213370101036,49.8099167892779));
#34367=CARTESIAN_POINT('Ctrl Pts',(43.9808695933246,44.6255587298567,49.7569410262731));
#34368=CARTESIAN_POINT('Ctrl Pts',(44.0397263377345,44.6297790682818,49.7039825967025));
#34369=CARTESIAN_POINT('Ctrl Pts',(44.0959405794593,44.6339994067069,49.6480440527762));
#34370=CARTESIAN_POINT('Ctrl Pts',(44.1492047191353,44.6382197451321,49.5894254595465));
#34371=CARTESIAN_POINT('Ctrl Pts',(44.2024680642923,44.6424400206042,49.5308077407061));
#34372=CARTESIAN_POINT('Ctrl Pts',(44.2527810802238,44.6466602960763,49.4695104002925));
#34373=CARTESIAN_POINT('Ctrl Pts',(44.2998747794902,44.6508805715483,49.4058685084875));
#34374=CARTESIAN_POINT('Ctrl Pts',(44.3470155834178,44.6551050682783,49.3421629599771));
#34375=CARTESIAN_POINT('Ctrl Pts',(44.3909303583399,44.6593295650082,49.2761085536373));
#34376=CARTESIAN_POINT('Ctrl Pts',(44.4313923861292,44.6635540617381,49.2080709476171));
#34377=CARTESIAN_POINT('Ctrl Pts',(44.471873839629,44.6677805866375,49.1400006769254));
#34378=CARTESIAN_POINT('Ctrl Pts',(44.5088990241303,44.6720071115369,49.0699457253269));
#34379=CARTESIAN_POINT('Ctrl Pts',(44.5422875554129,44.6762336364363,48.998295783234));
#34380=CARTESIAN_POINT('Ctrl Pts',(44.5757371197999,44.6804678872801,48.9265148674738));
#34381=CARTESIAN_POINT('Ctrl Pts',(44.6055365702878,44.6847021381238,48.8531335711954));
#34382=CARTESIAN_POINT('Ctrl Pts',(44.631554068754,44.6889363889676,48.7785607742029));
#34383=CARTESIAN_POINT('Ctrl Pts',(44.6563679068757,44.6929747485793,48.7074379752427));
#34384=CARTESIAN_POINT('Ctrl Pts',(44.6777419208073,44.6970131081911,48.635231836396));
#34385=CARTESIAN_POINT('Ctrl Pts',(44.6956050744272,44.7010514678028,48.5623057737249));
#34386=CARTESIAN_POINT('Ctrl Pts',(44.7143402531728,44.7052869679152,48.4858196812667));
#34387=CARTESIAN_POINT('Ctrl Pts',(44.7292842565899,44.7095224680277,48.4082508412591));
#34388=CARTESIAN_POINT('Ctrl Pts',(44.7403171312684,44.7137579681401,48.3300093422795));
#34389=CARTESIAN_POINT('Ctrl Pts',(44.7513340117802,44.7179873281217,48.251881268641));
#34390=CARTESIAN_POINT('Ctrl Pts',(44.7584509579835,44.7222166881032,48.1730829333129));
#34391=CARTESIAN_POINT('Ctrl Pts',(44.7615985056644,44.7264460480847,48.0940369020325));
#34392=CARTESIAN_POINT('Ctrl Pts',(44.7647423776626,44.7306704690514,48.0150831801147));
#34393=CARTESIAN_POINT('Ctrl Pts',(44.7639260440308,44.7348948900181,47.9358828035966));
#34394=CARTESIAN_POINT('Ctrl Pts',(44.7591317471986,44.7391193109847,47.8568642593213));
#34395=CARTESIAN_POINT('Ctrl Pts',(44.7543405162281,44.7433410305145,47.7778962459021));
#34396=CARTESIAN_POINT('Ctrl Pts',(44.7455763993675,44.7475627500444,47.6991103011625));
#34397=CARTESIAN_POINT('Ctrl Pts',(44.7328737174753,44.7517844695742,47.6209344921877));
#34398=CARTESIAN_POINT('Ctrl Pts',(44.7201751918418,44.7560048077769,47.5427842619756));
#34399=CARTESIAN_POINT('Ctrl Pts',(44.7035407352886,44.7602251459796,47.4652442340471));
#34400=CARTESIAN_POINT('Ctrl Pts',(44.6830563022954,44.7644454841824,47.3887354407056));
#34401=CARTESIAN_POINT('Ctrl Pts',(44.6625721748543,44.7686657594332,47.3122277885927));
#34402=CARTESIAN_POINT('Ctrl Pts',(44.6382383078035,44.7728860346841,47.2367517935278));
#34403=CARTESIAN_POINT('Ctrl Pts',(44.6101909846418,44.777106309935,47.1627149515796));
#34404=CARTESIAN_POINT('Ctrl Pts',(44.5821156076045,44.781330806447,47.0886040554932));
#34405=CARTESIAN_POINT('Ctrl Pts',(44.5503195212965,44.7855553029591,47.015935628046));
#34406=CARTESIAN_POINT('Ctrl Pts',(44.5149876018931,44.7897797994711,46.9450981634586));
#34407=CARTESIAN_POINT('Ctrl Pts',(44.4796387197172,44.7940063241541,46.8742266899686));
#34408=CARTESIAN_POINT('Ctrl Pts',(44.4407508533913,44.7982328488372,46.8051883399968));
#34409=CARTESIAN_POINT('Ctrl Pts',(44.3985541571483,44.8024593735202,46.7383456408964));
#34410=CARTESIAN_POINT('Ctrl Pts',(44.3562803267192,44.8066936241527,46.6713807555194));
#34411=CARTESIAN_POINT('Ctrl Pts',(44.3106858510907,44.8109278747852,46.6066199258715));
#34412=CARTESIAN_POINT('Ctrl Pts',(44.2620432863374,44.8151621254177,46.544395231972));
#34413=CARTESIAN_POINT('Ctrl Pts',(44.215651071391,44.8192004870146,46.4850492375945));
#34414=CARTESIAN_POINT('Ctrl Pts',(44.1664868188274,44.8232388486116,46.4280101564727));
#34415=CARTESIAN_POINT('Ctrl Pts',(44.1148177422448,44.8272772102086,46.3735343373491));
#34416=CARTESIAN_POINT('Ctrl Pts',(44.0606263616456,44.8315127105267,46.3163991988324));
#34417=CARTESIAN_POINT('Ctrl Pts',(44.0034733661707,44.8357482108448,46.2618667882227));
#34418=CARTESIAN_POINT('Ctrl Pts',(43.9436387580783,44.8399837111628,46.210259844151));
#34419=CARTESIAN_POINT('Ctrl Pts',(43.8838908911942,44.8442130713485,46.1587277137837));
#34420=CARTESIAN_POINT('Ctrl Pts',(43.8214694839679,44.8484424315342,46.1101129320315));
#34421=CARTESIAN_POINT('Ctrl Pts',(43.7566923465237,44.8526717917199,46.0647025247306));
#34422=CARTESIAN_POINT('Ctrl Pts',(43.6919908553802,44.8568962128875,46.0193451473947));
#34423=CARTESIAN_POINT('Ctrl Pts',(43.6249394831052,44.8611206340551,45.9771849763871));
#34424=CARTESIAN_POINT('Ctrl Pts',(43.5558889924924,44.8653450552227,45.9384687540726));
#34425=CARTESIAN_POINT('Ctrl Pts',(43.4868826583859,44.8695667749514,45.8997772900633));
#34426=CARTESIAN_POINT('Ctrl Pts',(43.4158801515753,44.8737884946802,45.8645256324937));
#34427=CARTESIAN_POINT('Ctrl Pts',(43.3432600558127,44.8780102144089,45.832916497223));
#34428=CARTESIAN_POINT('Ctrl Pts',(43.2706637210468,44.8822305528083,45.8013177043314));
#34429=CARTESIAN_POINT('Ctrl Pts',(43.1964512783069,44.8864508912077,45.773359254359));
#34430=CARTESIAN_POINT('Ctrl Pts',(43.1210233282464,44.8906712296071,45.7491966320834));
#34431=CARTESIAN_POINT('Ctrl Pts',(43.0455965033378,44.8948915050521,45.7250343702396));
#34432=CARTESIAN_POINT('Ctrl Pts',(42.9689546545346,44.8991117804971,45.7046679654549));
#34433=CARTESIAN_POINT('Ctrl Pts',(42.8915142257092,44.903332055942,45.6882032514026));
#34434=CARTESIAN_POINT('Ctrl Pts',(42.8139963384641,44.9075565526429,45.6717220688112));
#34435=CARTESIAN_POINT('Ctrl Pts',(42.7356787357484,44.9117810493438,45.659150470723));
#34436=CARTESIAN_POINT('Ctrl Pts',(42.6569881685724,44.9160055460447,45.6505431431682));
#34437=CARTESIAN_POINT('Ctrl Pts',(42.5782598222871,44.920232070914,45.6419316832609));
#34438=CARTESIAN_POINT('Ctrl Pts',(42.4991586240225,44.9244585957833,45.6372883129055));
#34439=CARTESIAN_POINT('Ctrl Pts',(42.4201139809706,44.9286851206526,45.6366155901611));
#34440=CARTESIAN_POINT('Ctrl Pts',(42.3409248470153,44.9329193714647,45.6359416377026));
#34441=CARTESIAN_POINT('Ctrl Pts',(42.2617929450269,44.9371536222769,45.6392528167839));
#34442=CARTESIAN_POINT('Ctrl Pts',(42.1831450141727,44.9413878730891,45.6464995525767));
#34443=CARTESIAN_POINT('Ctrl Pts',(42.1081356064422,44.9454262329309,45.653411029508));
#34444=CARTESIAN_POINT('Ctrl Pts',(42.0335667283851,44.9494645927727,45.6639018852172));
#34445=CARTESIAN_POINT('Ctrl Pts',(41.9597985362927,44.9535029526145,45.6778860682021));
#34446=CARTESIAN_POINT('Ctrl Pts',(41.8824291967322,44.9577384533772,45.692552918116));
#34447=CARTESIAN_POINT('Ctrl Pts',(41.805646616342,44.9619739541399,45.7111186237424));
#34448=CARTESIAN_POINT('Ctrl Pts',(41.7298737062781,44.9662094549025,45.7335222940954));
#34449=CARTESIAN_POINT('Ctrl Pts',(41.6542106428243,44.9704388155368,45.7558934862549));
#34450=CARTESIAN_POINT('Ctrl Pts',(41.5795547893287,44.974668176171,45.7820914624098));
#34451=CARTESIAN_POINT('Ctrl Pts',(41.5063194752089,44.9788975368052,45.8120042137817));
#34452=CARTESIAN_POINT('Ctrl Pts',(41.4331696847166,44.9831219584251,45.8418820332763));
#34453=CARTESIAN_POINT('Ctrl Pts',(41.361437569315,44.9873463800451,45.8754658308542));
#34454=CARTESIAN_POINT('Ctrl Pts',(41.2915204059977,44.991570801665,45.9125940906042));
#34455=CARTESIAN_POINT('Ctrl Pts',(41.2216479533683,44.9957925218481,45.9496986075427));
#34456=CARTESIAN_POINT('Ctrl Pts',(41.1535885626358,45.0000142420313,45.990342868372));
#34457=CARTESIAN_POINT('Ctrl Pts',(41.0877175341625,45.0042359622144,46.0343181410118));
#34458=CARTESIAN_POINT('Ctrl Pts',(41.0218680583941,45.0084563010697,46.0782790251398));
#34459=CARTESIAN_POINT('Ctrl Pts',(40.958205913163,45.012676639925,46.1255684965106));
#34460=CARTESIAN_POINT('Ctrl Pts',(40.8970785871185,45.0168969787802,46.1759337546015));
#34461=CARTESIAN_POINT('Ctrl Pts',(40.8359521728926,45.0211172546819,46.2262982614084));
#34462=CARTESIAN_POINT('Ctrl Pts',(40.7773608640782,45.0253375305836,46.2797381642466));
#34463=CARTESIAN_POINT('Ctrl Pts',(40.7216189623958,45.0295578064853,46.3359604771789));
#34464=CARTESIAN_POINT('Ctrl Pts',(40.6658213058933,45.033782303641,46.3922390254539));
#34465=CARTESIAN_POINT('Ctrl Pts',(40.6128790811359,45.0380068007966,46.4513052092275));
#34466=CARTESIAN_POINT('Ctrl Pts',(40.5630691493132,45.0422312979523,46.5128297035326));
#34467=CARTESIAN_POINT('Ctrl Pts',(40.5132353038953,45.046457823276,46.5743837355584));
#34468=CARTESIAN_POINT('Ctrl Pts',(40.4665370241649,45.0506843485998,46.6383980495722));
#34469=CARTESIAN_POINT('Ctrl Pts',(40.4232087671965,45.0549108739235,46.7045128858954));
#34470=CARTESIAN_POINT('Ctrl Pts',(40.3798013077261,45.0591451251842,46.7707485777715));
#34471=CARTESIAN_POINT('Ctrl Pts',(40.3397764185185,45.0633793764449,46.8390920584642));
#34472=CARTESIAN_POINT('Ctrl Pts',(40.303323268048,45.0676136277056,46.9091576087302));
#34473=CARTESIAN_POINT('Ctrl Pts',(40.2685566041134,45.0716519834771,46.9759816118151));
#34474=CARTESIAN_POINT('Ctrl Pts',(40.2370386144975,45.0756903392487,47.0443715272226));
#34475=CARTESIAN_POINT('Ctrl Pts',(40.2088917686089,45.0797286950203,47.1139779013873));
#34476=CARTESIAN_POINT('Ctrl Pts',(40.1757163997721,45.0844885158097,47.1960196742183));
#34477=CARTESIAN_POINT('Ctrl Pts',(40.1471176123712,45.0892483365991,47.2800134669348));
#34478=CARTESIAN_POINT('Ctrl Pts',(40.1233014859866,45.0940081573885,47.3654652750329));
#34479=CARTESIAN_POINT('Ctrl Pts',(40.0995701814865,45.0987510259261,47.450612743824));
#34480=CARTESIAN_POINT('Ctrl Pts',(40.0805876735128,45.1034938944638,47.5372076374993));
#34481=CARTESIAN_POINT('Ctrl Pts',(40.066511289221,45.1082367630015,47.6247389207938));
#34482=CARTESIAN_POINT('Ctrl Pts',(40.052520392988,45.112950827365,47.7117386130679));
#34483=CARTESIAN_POINT('Ctrl Pts',(40.0433763266751,45.1176648917286,47.7996631151682));
#34484=CARTESIAN_POINT('Ctrl Pts',(40.0391855935731,45.1223789560921,47.8879920569462));
#34485=CARTESIAN_POINT('Ctrl Pts',(40.0374389765965,45.1243436874758,47.9248058614714));
#34486=CARTESIAN_POINT('Ctrl Pts',(40.036552198086,45.1263084188595,47.9616897171321));
#34487=CARTESIAN_POINT('Ctrl Pts',(40.0365304116029,45.1282731502432,47.9986051444044));
#34488=CARTESIAN_POINT('',(40.0365307523589,45.9220231503247,48.0018858300131));
#34489=CARTESIAN_POINT('Ctrl Pts',(40.0365304116026,45.1282731502717,47.9986051449398));
#34490=CARTESIAN_POINT('Ctrl Pts',(40.0364831607206,45.132534293567,48.0786679599995));
#34491=CARTESIAN_POINT('Ctrl Pts',(40.0405084554841,45.1367954368622,48.1587400086586));
#34492=CARTESIAN_POINT('Ctrl Pts',(40.048582621628,45.1410565801575,48.2383836269337));
#34493=CARTESIAN_POINT('Ctrl Pts',(40.0566584521647,45.1453186018365,48.3180436627888));
#34494=CARTESIAN_POINT('Ctrl Pts',(40.0687847659602,45.1495806235155,48.3972746385648));
#34495=CARTESIAN_POINT('Ctrl Pts',(40.0848861177655,45.1538426451946,48.4756449865026));
#34496=CARTESIAN_POINT('Ctrl Pts',(40.1012920702124,45.1581852945472,48.5554979216514));
#34497=CARTESIAN_POINT('Ctrl Pts',(40.1218249154472,45.1625279438999,48.6344568465592));
#34498=CARTESIAN_POINT('Ctrl Pts',(40.146351044666,45.1668705932525,48.7120792280512));
#34499=CARTESIAN_POINT('Ctrl Pts',(40.1704688745975,45.1711409482525,48.7884093892029));
#34500=CARTESIAN_POINT('Ctrl Pts',(40.1984478103584,45.1754113032524,48.8634467624919));
#34501=CARTESIAN_POINT('Ctrl Pts',(40.230111961434,45.1796816582524,48.9367904466786));
#34502=CARTESIAN_POINT('Ctrl Pts',(40.2625801929569,45.1840604547813,49.0119966226859));
#34503=CARTESIAN_POINT('Ctrl Pts',(40.2989231194113,45.1884392513103,49.0854214593619));
#34504=CARTESIAN_POINT('Ctrl Pts',(40.3389017872644,45.1928180478393,49.1566609694972));
#34505=CARTESIAN_POINT('Ctrl Pts',(40.3788804551175,45.1971968443683,49.2279004796325));
#34506=CARTESIAN_POINT('Ctrl Pts',(40.4224945307587,45.2015756408973,49.2969542716546));
#34507=CARTESIAN_POINT('Ctrl Pts',(40.4694596645134,45.2059544374263,49.3634531359601));
#34508=CARTESIAN_POINT('Ctrl Pts',(40.5148878710121,45.2101899384678,49.4277758344831));
#34509=CARTESIAN_POINT('Ctrl Pts',(40.5636206474227,45.2144254395093,49.4899479095042));
#34510=CARTESIAN_POINT('Ctrl Pts',(40.6154272214919,45.2186609405509,49.5496097699446));
#34511=CARTESIAN_POINT('Ctrl Pts',(40.6671586923627,45.2228903014513,49.6091851394982));
#34512=CARTESIAN_POINT('Ctrl Pts',(40.7219548068612,45.2271196623518,49.6662571695286));
#34513=CARTESIAN_POINT('Ctrl Pts',(40.7795422497894,45.2313490232522,49.7204961844429));
#34514=CARTESIAN_POINT('Ctrl Pts',(40.8370624422827,45.2355734451183,49.7746718592058));
#34515=CARTESIAN_POINT('Ctrl Pts',(40.8973671456749,45.2397978669843,49.8260207731037));
#34516=CARTESIAN_POINT('Ctrl Pts',(40.9601446506006,45.2440222888504,49.8742483863421));
#34517=CARTESIAN_POINT('Ctrl Pts',(41.0228820103333,45.2482440092674,49.9224451588065));
#34518=CARTESIAN_POINT('Ctrl Pts',(41.0880886618312,45.2524657296844,49.9675243071242));
#34519=CARTESIAN_POINT('Ctrl Pts',(41.1554190427955,45.2566874501014,50.0092308682339));
#34520=CARTESIAN_POINT('Ctrl Pts',(41.2227273933636,45.260907789178,50.0509237830215));
#34521=CARTESIAN_POINT('Ctrl Pts',(41.2921576948924,45.2651281282547,50.0892460548279));
#34522=CARTESIAN_POINT('Ctrl Pts',(41.3633358160648,45.2693484673313,50.123986301897));
#34523=CARTESIAN_POINT('Ctrl Pts',(41.4345128752798,45.2735687434417,50.1587260306514));
#34524=CARTESIAN_POINT('Ctrl Pts',(41.5074372799248,45.277789019552,50.1898836362334));
#34525=CARTESIAN_POINT('Ctrl Pts',(41.5817120920012,45.2820092956624,50.2172945993988));
#34526=CARTESIAN_POINT('Ctrl Pts',(41.6560611957255,45.2862337930055,50.2447329797406));
#34527=CARTESIAN_POINT('Ctrl Pts',(41.7317629637269,45.2904582903486,50.2684170686901));
#34528=CARTESIAN_POINT('Ctrl Pts',(41.8084029152355,45.2946827876917,50.2882314852738));
#34529=CARTESIAN_POINT('Ctrl Pts',(41.8850796611432,45.2989093131916,50.3080554146446));
#34530=CARTESIAN_POINT('Ctrl Pts',(41.9626950274675,45.3031358386915,50.3240058760595));
#34531=CARTESIAN_POINT('Ctrl Pts',(42.0408244216449,45.3073623641914,50.3360186953048));
#34532=CARTESIAN_POINT('Ctrl Pts',(42.119096633161,45.3115966156072,50.3480534734925));
#34533=CARTESIAN_POINT('Ctrl Pts',(42.1978842819863,45.3158308670229,50.3561361784949));
#34534=CARTESIAN_POINT('Ctrl Pts',(42.2767579321219,45.3200651184387,50.3602546120292));
#34535=CARTESIAN_POINT('Ctrl Pts',(42.3519824932765,45.3241034722365,50.3641825062592));
#34536=CARTESIAN_POINT('Ctrl Pts',(42.4272849167069,45.3281418260342,50.3645048659867));
#34537=CARTESIAN_POINT('Ctrl Pts',(42.5022964251498,45.332180179832,50.3612551497671));
#34538=CARTESIAN_POINT('Ctrl Pts',(42.5809699470928,45.3364156834596,50.357846784496));
#34539=CARTESIAN_POINT('Ctrl Pts',(42.6596224767622,45.3406511870872,50.3504957088366));
#34540=CARTESIAN_POINT('Ctrl Pts',(42.7378267416534,45.3448866907148,50.3392014734785));
#34541=CARTESIAN_POINT('Ctrl Pts',(42.8159176356725,45.3491160542331,50.3279236111061));
#34542=CARTESIAN_POINT('Ctrl Pts',(42.8935610947764,45.3533454177513,50.3127140071283));
#34543=CARTESIAN_POINT('Ctrl Pts',(42.9703319909164,45.3575747812695,50.2936241760666));
#34544=CARTESIAN_POINT('Ctrl Pts',(43.0470132349386,45.3617992057885,50.2745566378773));
#34545=CARTESIAN_POINT('Ctrl Pts',(43.1228234877626,45.3660236303075,50.2516179897764));
#34546=CARTESIAN_POINT('Ctrl Pts',(43.1973464006665,45.3702480548265,50.2249110450183));
#34547=CARTESIAN_POINT('Ctrl Pts',(43.2718216577657,45.3744697779167,50.1982211787786));
#34548=CARTESIAN_POINT('Ctrl Pts',(43.3450107682317,45.3786915010068,50.1677679566239));
#34549=CARTESIAN_POINT('Ctrl Pts',(43.4165123543819,45.3829132240969,50.1337040737387));
#34550=CARTESIAN_POINT('Ctrl Pts',(43.4879905456159,45.387133565863,50.099651336364));
#34551=CARTESIAN_POINT('Ctrl Pts',(43.557781885516,45.3913539076292,50.0619904858153));
#34552=CARTESIAN_POINT('Ctrl Pts',(43.625506193939,45.3955742493953,50.0209218217232));
#34553=CARTESIAN_POINT('Ctrl Pts',(43.6932294921368,45.3997945282077,49.9798537702414));
#34554=CARTESIAN_POINT('Ctrl Pts',(43.7588854195137,45.4040148070201,49.9353782507703));
#34555=CARTESIAN_POINT('Ctrl Pts',(43.8221208704177,45.4082350858325,49.8877400962056));
#34556=CARTESIAN_POINT('Ctrl Pts',(43.8854195710733,45.4124595858781,49.8400542927131));
#34557=CARTESIAN_POINT('Ctrl Pts',(43.9462925831825,45.4166840859238,49.7891998180229));
#34558=CARTESIAN_POINT('Ctrl Pts',(44.004418637284,45.4209085859694,49.7354628423668));
#34559=CARTESIAN_POINT('Ctrl Pts',(44.0625725974162,45.4251351141766,49.6817000678549));
#34560=CARTESIAN_POINT('Ctrl Pts',(44.1179766436995,45.4293616423837,49.6250523715345));
#34561=CARTESIAN_POINT('Ctrl Pts',(44.1703471026072,45.4335881705909,49.5658421303536));
#34562=CARTESIAN_POINT('Ctrl Pts',(44.2228132922078,45.4378224246894,49.5065236556851));
#34563=CARTESIAN_POINT('Ctrl Pts',(44.2722345200738,45.4420566787879,49.4446336437347));
#34564=CARTESIAN_POINT('Ctrl Pts',(44.318368205642,45.4462909328864,49.3805266634448));
#34565=CARTESIAN_POINT('Ctrl Pts',(44.3623672269892,45.4503292626703,49.3193859945487));
#34566=CARTESIAN_POINT('Ctrl Pts',(44.4033760505672,45.4543675924541,49.2562293028178));
#34567=CARTESIAN_POINT('Ctrl Pts',(44.4412233136354,45.458405922238,49.1913848348756));
#34568=CARTESIAN_POINT('Ctrl Pts',(44.4809183637648,45.4626414122104,49.1233745166407));
#34569=CARTESIAN_POINT('Ctrl Pts',(44.5172861515701,45.4668769021828,49.053248888801));
#34570=CARTESIAN_POINT('Ctrl Pts',(44.5500951483325,45.4711123921553,48.9813670536639));
#34571=CARTESIAN_POINT('Ctrl Pts',(44.5828565822975,45.4753417419902,48.9095894247354));
#34572=CARTESIAN_POINT('Ctrl Pts',(44.6120692771118,45.4795710918251,48.8360610676888));
#34573=CARTESIAN_POINT('Ctrl Pts',(44.6375465671233,45.48380044166,48.7611673934522));
#34574=CARTESIAN_POINT('Ctrl Pts',(44.6629941050983,45.4880248525171,48.6863611790406));
#34575=CARTESIAN_POINT('Ctrl Pts',(44.6847147563111,45.4922492633742,48.6101932578452));
#34576=CARTESIAN_POINT('Ctrl Pts',(44.7025697482568,45.4964736742313,48.53306940947));
#34577=CARTESIAN_POINT('Ctrl Pts',(44.7204133223606,45.5006953836784,48.4559948799579));
#34578=CARTESIAN_POINT('Ctrl Pts',(44.7343960380072,45.5049170931254,48.3779660925758));
#34579=CARTESIAN_POINT('Ctrl Pts',(44.7444291739671,45.5091388025724,48.2994032216792));
#34580=CARTESIAN_POINT('Ctrl Pts',(44.7544590272192,45.5133591307326,48.2208660555029));
#34581=CARTESIAN_POINT('Ctrl Pts',(44.7605418073509,45.5175794588928,48.141795618018));
#34582=CARTESIAN_POINT('Ctrl Pts',(44.7626402974864,45.521799787053,48.0626200095295));
#34583=CARTESIAN_POINT('Ctrl Pts',(44.7647387563468,45.526020052315,47.9834455810443));
#34584=CARTESIAN_POINT('Ctrl Pts',(44.7628530321443,45.530240317577,47.9041664538956));
#34585=CARTESIAN_POINT('Ctrl Pts',(44.7569980087985,45.534460582839,47.8252120501289));
#34586=CARTESIAN_POINT('Ctrl Pts',(44.7511371288338,45.5386850695163,47.7461786704446));
#34587=CARTESIAN_POINT('Ctrl Pts',(44.7412990531836,45.5429095561935,47.6674711321817));
#34588=CARTESIAN_POINT('Ctrl Pts',(44.7275506547398,45.5471340428707,47.5895144454181));
#34589=CARTESIAN_POINT('Ctrl Pts',(44.7137956554857,45.5513605577868,47.5115203304913));
#34590=CARTESIAN_POINT('Ctrl Pts',(44.6961266982247,45.5555870727028,47.4342782433785));
#34591=CARTESIAN_POINT('Ctrl Pts',(44.6746614457831,45.5598135876188,47.358201162382));
#34592=CARTESIAN_POINT('Ctrl Pts',(44.6531569542943,45.5640478287155,47.2819850104764));
#34593=CARTESIAN_POINT('Ctrl Pts',(44.6278424508328,45.5682820698122,47.2069385661546));
#34594=CARTESIAN_POINT('Ctrl Pts',(44.5988849035263,45.5725163109089,47.1334576629246));
#34595=CARTESIAN_POINT('Ctrl Pts',(44.5712663432456,45.5765547621538,47.0633744913818));
#34596=CARTESIAN_POINT('Ctrl Pts',(44.5403343790282,45.5805932133988,46.9947155913935));
#34597=CARTESIAN_POINT('Ctrl Pts',(44.5062723882212,45.5846316646438,46.9278026918907));
#34598=CARTESIAN_POINT('Ctrl Pts',(44.4705483286529,45.5888671737677,46.8576247501119));
#34599=CARTESIAN_POINT('Ctrl Pts',(44.4312451870556,45.5931026828915,46.7891007845917));
#34600=CARTESIAN_POINT('Ctrl Pts',(44.3885397261206,45.5973381920153,46.7226197909235));
#34601=CARTESIAN_POINT('Ctrl Pts',(44.3458961751394,45.6015675609368,46.6562351745138));
#34602=CARTESIAN_POINT('Ctrl Pts',(44.2998603510811,45.6057969298582,46.591888040118));
#34603=CARTESIAN_POINT('Ctrl Pts',(44.2506554133761,45.6100262987796,46.5299438847983));
#34604=CARTESIAN_POINT('Ctrl Pts',(44.2015079384275,45.6142507285383,46.4680720694119));
#34605=CARTESIAN_POINT('Ctrl Pts',(44.1491989947642,45.6184751582969,46.4085980221448));
#34606=CARTESIAN_POINT('Ctrl Pts',(44.0939947821361,45.6226995880556,46.3518579797251));
#34607=CARTESIAN_POINT('Ctrl Pts',(44.0388258726987,45.626921316284,46.2951542226621));
#34608=CARTESIAN_POINT('Ctrl Pts',(43.9807656955991,45.6311430445124,46.241181335737));
#34609=CARTESIAN_POINT('Ctrl Pts',(43.9201196342383,45.6353647727409,46.1902412485352));
#34610=CARTESIAN_POINT('Ctrl Pts',(43.8594934174458,45.6395851195379,46.1393178299187));
#34611=CARTESIAN_POINT('Ctrl Pts',(43.7962833556874,45.6438054663349,46.0914255421101));
#34612=CARTESIAN_POINT('Ctrl Pts',(43.7308293617135,45.6480258131319,46.0468272859521));
#34613=CARTESIAN_POINT('Ctrl Pts',(43.6653763458594,45.6522460968616,46.0022296962537));
#34614=CARTESIAN_POINT('Ctrl Pts',(43.5976798530667,45.6564663805913,45.960926303538));
#34615=CARTESIAN_POINT('Ctrl Pts',(43.5281090938304,45.6606866643211,45.9231369054949));
#34616=CARTESIAN_POINT('Ctrl Pts',(43.4584687516683,45.6649111690725,45.8853097114452));
#34617=CARTESIAN_POINT('Ctrl Pts',(43.3869508117429,45.669135673824,45.8510037575045));
#34618=CARTESIAN_POINT('Ctrl Pts',(43.3139488995933,45.6733601785755,45.8203927303681));
#34619=CARTESIAN_POINT('Ctrl Pts',(43.2409119414849,45.677586711381,45.7897670078249));
#34620=CARTESIAN_POINT('Ctrl Pts',(43.1663900339697,45.6818132441865,45.7628399054713));
#34621=CARTESIAN_POINT('Ctrl Pts',(43.0907941606151,45.686039776992,45.7397358852205));
#34622=CARTESIAN_POINT('Ctrl Pts',(43.0150601059946,45.6902740354527,45.7165896332628));
#34623=CARTESIAN_POINT('Ctrl Pts',(42.9382486191926,45.6945082939134,45.6972805421796));
#34624=CARTESIAN_POINT('Ctrl Pts',(42.8607829384152,45.6987425523741,45.6818823315963));
#34625=CARTESIAN_POINT('Ctrl Pts',(42.7869025904808,45.7027808372659,45.6671967941551));
#34626=CARTESIAN_POINT('Ctrl Pts',(42.7124276233734,45.7068191221578,45.6560681495653));
#34627=CARTESIAN_POINT('Ctrl Pts',(42.6377277782365,45.7108574070496,45.6485162249433));
#34628=CARTESIAN_POINT('Ctrl Pts',(42.5593794600486,45.7150929289448,45.6405954509159));
#34629=CARTESIAN_POINT('Ctrl Pts',(42.4804859357017,45.7193284508399,45.6365796021642));
#34630=CARTESIAN_POINT('Ctrl Pts',(42.4014699915066,45.723563972735,45.6365304571404));
#34631=CARTESIAN_POINT('Ctrl Pts',(42.3225685914181,45.7277933546786,45.6364813833589));
#34632=CARTESIAN_POINT('Ctrl Pts',(42.2435455892698,45.7320227366221,45.6403875945823));
#34633=CARTESIAN_POINT('Ctrl Pts',(42.1648291082892,45.7362521185657,45.6482591357482));
#34634=CARTESIAN_POINT('Ctrl Pts',(42.0862045482709,45.7404765616596,45.6561214849427));
#34635=CARTESIAN_POINT('Ctrl Pts',(42.0078862627192,45.7447010047536,45.6679399159463));
#34636=CARTESIAN_POINT('Ctrl Pts',(41.9303010502155,45.7489254478476,45.6836724459889));
#34637=CARTESIAN_POINT('Ctrl Pts',(41.8527654500533,45.7531471895955,45.6993949157682));
#34638=CARTESIAN_POINT('Ctrl Pts',(41.7759624512762,45.7573689313433,45.7190264238513));
#34639=CARTESIAN_POINT('Ctrl Pts',(41.7003111969052,45.7615906730912,45.7424734730853));
#34640=CARTESIAN_POINT('Ctrl Pts',(41.6246846940734,45.7658110335717,45.7659128509255));
#34641=CARTESIAN_POINT('Ctrl Pts',(41.5502096353618,45.7700313940522,45.7931651522315));
#34642=CARTESIAN_POINT('Ctrl Pts',(41.4772910193502,45.7742517545327,45.8240867255499));
#34643=CARTESIAN_POINT('Ctrl Pts',(41.4043734905107,45.7784720520902,45.8550078378465));
#34644=CARTESIAN_POINT('Ctrl Pts',(41.3330127898229,45.7826923496478,45.8895979289479));
#34645=CARTESIAN_POINT('Ctrl Pts',(41.2635935145341,45.7869126472053,45.9276653888209));
#34646=CARTESIAN_POINT('Ctrl Pts',(41.1941048059683,45.7911371659116,45.9657709238319));
#34647=CARTESIAN_POINT('Ctrl Pts',(41.1265618143403,45.7953616846179,46.0073605492878));
#34648=CARTESIAN_POINT('Ctrl Pts',(41.0613235644421,45.7995862033242,46.0521971758461));
#34649=CARTESIAN_POINT('Ctrl Pts',(40.9960539943587,45.8038127501767,46.0970553279887));
#34650=CARTESIAN_POINT('Ctrl Pts',(40.9330917437077,45.8080392970292,46.1451633013083));
#34651=CARTESIAN_POINT('Ctrl Pts',(40.872763828304,45.8122658438817,46.1962427777655));
#34652=CARTESIAN_POINT('Ctrl Pts',(40.8123256404039,45.8165001163761,46.2474156216355));
#34653=CARTESIAN_POINT('Ctrl Pts',(40.7545317531609,45.8207343888705,46.3015705004234));
#34654=CARTESIAN_POINT('Ctrl Pts',(40.6996731362859,45.8249686613649,46.3583913385242));
#34655=CARTESIAN_POINT('Ctrl Pts',(40.6473552893458,45.8290068240618,46.4125805266612));
#34656=CARTESIAN_POINT('Ctrl Pts',(40.5977070470928,45.8330449867586,46.4691939018447));
#34657=CARTESIAN_POINT('Ctrl Pts',(40.5509450912843,45.8370831494555,46.527931256546));
#34658=CARTESIAN_POINT('Ctrl Pts',(40.5019863988631,45.8413110129399,46.5894279162287));
#34659=CARTESIAN_POINT('Ctrl Pts',(40.456001613711,45.8455388764243,46.6534920074066));
#34660=CARTESIAN_POINT('Ctrl Pts',(40.4132720529381,45.8497667399087,46.7198037239302));
#34661=CARTESIAN_POINT('Ctrl Pts',(40.3706026233879,45.8539886537274,46.7860221232156));
#34662=CARTESIAN_POINT('Ctrl Pts',(40.3311795791544,45.8582105675462,46.8544814788692));
#34663=CARTESIAN_POINT('Ctrl Pts',(40.2952439087338,45.8624324813649,46.924829205578));
#34664=CARTESIAN_POINT('Ctrl Pts',(40.259347505455,45.8666497818708,46.9951000628667));
#34665=CARTESIAN_POINT('Ctrl Pts',(40.2269311231829,45.8708670823768,47.0672547778774));
#34666=CARTESIAN_POINT('Ctrl Pts',(40.1981915184993,45.8750843828827,47.140913361941));
#34667=CARTESIAN_POINT('Ctrl Pts',(40.1694724175153,45.8792986746394,47.2145193957521));
#34668=CARTESIAN_POINT('Ctrl Pts',(40.1444250573977,45.8835129663961,47.289626731564));
#34669=CARTESIAN_POINT('Ctrl Pts',(40.1231988235759,45.8877272581529,47.3658337410947));
#34670=CARTESIAN_POINT('Ctrl Pts',(40.101981865698,45.8919397082483,47.4420074478764));
#34671=CARTESIAN_POINT('Ctrl Pts',(40.0845828410875,45.8961521583437,47.5192794202338));
#34672=CARTESIAN_POINT('Ctrl Pts',(40.0711013561075,45.9003646084391,47.5972326386414));
#34673=CARTESIAN_POINT('Ctrl Pts',(40.0576170767114,45.9045779316831,47.6752020150418));
#34674=CARTESIAN_POINT('Ctrl Pts',(40.0480520456333,45.908791254927,47.7538524565879));
#34675=CARTESIAN_POINT('Ctrl Pts',(40.0424545776666,45.913004578171,47.832757593492));
#34676=CARTESIAN_POINT('Ctrl Pts',(40.038460804777,45.9160107688712,47.8890561196266));
#34677=CARTESIAN_POINT('Ctrl Pts',(40.0364857490142,45.9190169595715,47.9454840988405));
#34678=CARTESIAN_POINT('Ctrl Pts',(40.0365307523581,45.9220231502717,48.001885829018));
#34679=CARTESIAN_POINT('Ctrl Pts',(40.0365307523589,45.9220231503247,48.0018858300131));
#34680=CARTESIAN_POINT('Ctrl Pts',(40.036604800625,45.9269695181273,48.0946888920839));
#34681=CARTESIAN_POINT('Ctrl Pts',(40.0421487212102,45.9319158859298,48.1872613527968));
#34682=CARTESIAN_POINT('Ctrl Pts',(40.0530579116337,45.9368622537323,48.2790219969011));
#34683=CARTESIAN_POINT('Ctrl Pts',(40.0640877371016,45.9418633190216,48.3717973404419));
#34684=CARTESIAN_POINT('Ctrl Pts',(40.0806020526626,45.946864384311,48.4637427056642));
#34685=CARTESIAN_POINT('Ctrl Pts',(40.1024434110274,45.9518654496003,48.5542780542008));
#34686=CARTESIAN_POINT('Ctrl Pts',(40.1191025498901,45.955679930354,48.6233324105306));
#34687=CARTESIAN_POINT('Ctrl Pts',(40.138859746909,45.9594944111076,48.6915668875298));
#34688=CARTESIAN_POINT('Ctrl Pts',(40.1616266405747,45.9633088918613,48.7587325910458));
#34689=CARTESIAN_POINT('Ctrl Pts',(40.1869069439293,45.9675444820129,48.8333132248749));
#34690=CARTESIAN_POINT('Ctrl Pts',(40.2159668137028,45.9717800721645,48.9067707372094));
#34691=CARTESIAN_POINT('Ctrl Pts',(40.2486871505458,45.9760156623161,48.9786947760529));
#34692=CARTESIAN_POINT('Ctrl Pts',(40.281360050537,45.9802451118505,49.0505145418265));
#34693=CARTESIAN_POINT('Ctrl Pts',(40.3176826864701,45.9844745613849,49.1208048253659));
#34694=CARTESIAN_POINT('Ctrl Pts',(40.3574866697458,45.9887040109194,49.1891718700987));
#34695=CARTESIAN_POINT('Ctrl Pts',(40.3972441604984,45.9929285203005,49.2574590595971));
#34696=CARTESIAN_POINT('Ctrl Pts',(40.4404746830861,45.9971530296815,49.3238270708495));
#34697=CARTESIAN_POINT('Ctrl Pts',(40.4869630542426,46.0013775390626,49.3879049265231));
#34698=CARTESIAN_POINT('Ctrl Pts',(40.5334216895834,46.0055993462791,49.4519417954454));
#34699=CARTESIAN_POINT('Ctrl Pts',(40.5831337626294,46.0098211534956,49.5136910373979));
#34700=CARTESIAN_POINT('Ctrl Pts',(40.6358403875421,46.0140429607121,49.5728100020893));
#34701=CARTESIAN_POINT('Ctrl Pts',(40.6885297569592,46.0182633857612,49.6319096119647));
#34702=CARTESIAN_POINT('Ctrl Pts',(40.7442114194451,46.0224838108103,49.6883803044246));
#34703=CARTESIAN_POINT('Ctrl Pts',(40.8025867147373,46.0267042358594,49.7419130968468));
#34704=CARTESIAN_POINT('Ctrl Pts',(40.8609611261152,46.0309245970032,49.7954450786794));
#34705=CARTESIAN_POINT('Ctrl Pts',(40.9220287424196,46.035144958147,49.8460389326746));
#34706=CARTESIAN_POINT('Ctrl Pts',(40.9854557212912,46.0393653192907,49.8934241269384));
#34707=CARTESIAN_POINT('Ctrl Pts',(41.0489461092583,46.0435898996057,49.9408566930359));
#34708=CARTESIAN_POINT('Ctrl Pts',(41.1148001947032,46.0478144799207,49.9850739099351));
#34709=CARTESIAN_POINT('Ctrl Pts',(41.1826533535065,46.0520390602356,50.0258473741057));
#34710=CARTESIAN_POINT('Ctrl Pts',(41.2505390717185,46.0562656677198,50.0666404034654));
#34711=CARTESIAN_POINT('Ctrl Pts',(41.320425359749,46.0604922752041,50.1039861666234));
#34712=CARTESIAN_POINT('Ctrl Pts',(41.3919233481216,46.0647188826883,50.1377024827692));
#34713=CARTESIAN_POINT('Ctrl Pts',(41.4635519846217,46.0689532134437,50.1714804086704));
#34714=CARTESIAN_POINT('Ctrl Pts',(41.5367977712082,46.0731875441991,50.2016154560557));
#34715=CARTESIAN_POINT('Ctrl Pts',(41.611252425834,46.0774218749545,50.2279739013613));
#34716=CARTESIAN_POINT('Ctrl Pts',(41.682247612818,46.0814594613921,50.2531076255387));
#34717=CARTESIAN_POINT('Ctrl Pts',(41.7543414734322,46.0854970478296,50.2748078360182));
#34718=CARTESIAN_POINT('Ctrl Pts',(41.8271711395766,46.0895346342672,50.2930018616578));
#34719=CARTESIAN_POINT('Ctrl Pts',(41.9035730842204,46.0937702633979,50.3120883001018));
#34720=CARTESIAN_POINT('Ctrl Pts',(41.9810751446395,46.0980058925286,50.3273882921773));
#34721=CARTESIAN_POINT('Ctrl Pts',(42.0592677571527,46.1022415216593,50.338780019494));
#34722=CARTESIAN_POINT('Ctrl Pts',(42.1373470455186,46.1064710121146,50.3501552368394));
#34723=CARTESIAN_POINT('Ctrl Pts',(42.2161144380453,46.11070050257,50.3576333705177));
#34724=CARTESIAN_POINT('Ctrl Pts',(42.2951476654467,46.1149299930254,50.361143034388));
#34725=CARTESIAN_POINT('Ctrl Pts',(42.3740886304944,46.119154546029,50.3646486011226));
#34726=CARTESIAN_POINT('Ctrl Pts',(42.4532943473058,46.1233790990327,50.3641948834675));
#34727=CARTESIAN_POINT('Ctrl Pts',(42.5323363909304,46.1276036520363,50.3597621745709));
#34728=CARTESIAN_POINT('Ctrl Pts',(42.611327906917,46.1318255044939,50.3553322992841));
#34729=CARTESIAN_POINT('Ctrl Pts',(42.6901554900649,46.1360473569514,50.3469285074188));
#34730=CARTESIAN_POINT('Ctrl Pts',(42.7683908985587,46.1402692094089,50.3345831719515));
#34731=CARTESIAN_POINT('Ctrl Pts',(42.8466007226081,46.1444896812416,50.3222418736402));
#34732=CARTESIAN_POINT('Ctrl Pts',(42.9242182933021,46.1487101530743,50.3059616642739));
#34733=CARTESIAN_POINT('Ctrl Pts',(43.000822168485,46.1529306249069,50.2858265819517));
#34734=CARTESIAN_POINT('Ctrl Pts',(43.0774249103957,46.1571510343023,50.2656917975065));
#34735=CARTESIAN_POINT('Ctrl Pts',(43.1530135330446,46.1613714436976,50.2417023740636));
#34736=CARTESIAN_POINT('Ctrl Pts',(43.2271799008161,46.1655918530929,50.2139927399578));
#34737=CARTESIAN_POINT('Ctrl Pts',(43.3014204473718,46.1698164836041,50.186255391579));
#34738=CARTESIAN_POINT('Ctrl Pts',(43.3742354567555,46.1740411141154,50.1547905643507));
#34739=CARTESIAN_POINT('Ctrl Pts',(43.4452355730499,46.1782657446267,50.1197813655495));
#34740=CARTESIAN_POINT('Ctrl Pts',(43.5162697776245,46.1824924034499,50.0847553582776));
#34741=CARTESIAN_POINT('Ctrl Pts',(43.5854869427322,46.1867190622732,50.0461818181882));
#34742=CARTESIAN_POINT('Ctrl Pts',(43.6525234717276,46.1909457210965,50.0042892490036));
#34743=CARTESIAN_POINT('Ctrl Pts',(43.7196825156794,46.1951801044981,49.962320117587));
#34744=CARTESIAN_POINT('Ctrl Pts',(43.7846525739653,46.1994144878997,49.9170201052931));
#34745=CARTESIAN_POINT('Ctrl Pts',(43.8471003027147,46.2036488713014,49.8686602566499));
#34746=CARTESIAN_POINT('Ctrl Pts',(43.9066395500663,46.2076860397586,49.8225527512544));
#34747=CARTESIAN_POINT('Ctrl Pts',(43.9638859411231,46.2117232082158,49.7736643427086));
#34748=CARTESIAN_POINT('Ctrl Pts',(44.0185821359781,46.215760376673,49.7222608135798));
#34749=CARTESIAN_POINT('Ctrl Pts',(44.0759567971213,46.2199952447991,49.6683400596197));
#34750=CARTESIAN_POINT('Ctrl Pts',(44.1307433138437,46.2242301129252,49.6114464648617));
#34751=CARTESIAN_POINT('Ctrl Pts',(44.1826177016614,46.2284649810513,49.5518584248003));
#34752=CARTESIAN_POINT('Ctrl Pts',(44.2344168621055,46.2326937078421,49.4923567983224));
#34753=CARTESIAN_POINT('Ctrl Pts',(44.2833119742782,46.236922434633,49.4301688370739));
#34754=CARTESIAN_POINT('Ctrl Pts',(44.3290145857132,46.2411511614238,49.3656109142087));
#34755=CARTESIAN_POINT('Ctrl Pts',(44.3746638302279,46.2453749503321,49.3011283756031));
#34756=CARTESIAN_POINT('Ctrl Pts',(44.4171277120583,46.2495987392405,49.2342817558782));
#34757=CARTESIAN_POINT('Ctrl Pts',(44.456157905618,46.2538225281488,49.1654205713238));
#34758=CARTESIAN_POINT('Ctrl Pts',(44.4951631451948,46.2580436165746,49.0966034132181));
#34759=CARTESIAN_POINT('Ctrl Pts',(44.5307388228312,46.2622647050004,49.0257746540407));
#34760=CARTESIAN_POINT('Ctrl Pts',(44.5626805084814,46.2664857934262,48.9533118372992));
#34761=CARTESIAN_POINT('Ctrl Pts',(44.5946117550196,46.2707055023251,48.8808727026973));
#34762=CARTESIAN_POINT('Ctrl Pts',(44.6229111785989,46.274925211224,48.806801000239));
#34763=CARTESIAN_POINT('Ctrl Pts',(44.6474214773925,46.2791449201229,48.7314965098038));
#34764=CARTESIAN_POINT('Ctrl Pts',(44.6719314259048,46.2833645687172,48.6561930955591));
#34765=CARTESIAN_POINT('Ctrl Pts',(44.6926522132296,46.2875842173114,48.5796573752252));
#34766=CARTESIAN_POINT('Ctrl Pts',(44.7094761151086,46.2918038659056,48.5023052006926));
#34767=CARTESIAN_POINT('Ctrl Pts',(44.7263168813563,46.2960277442981,48.4248754879294));
#34768=CARTESIAN_POINT('Ctrl Pts',(44.7392528589133,46.3002516226905,48.3466281459569));
#34769=CARTESIAN_POINT('Ctrl Pts',(44.7482274233652,46.3044755010829,48.2679895689311));
#34770=CARTESIAN_POINT('Ctrl Pts',(44.7572063048397,46.3087014112819,48.189313164496));
#34771=CARTESIAN_POINT('Ctrl Pts',(44.7622199474325,46.3129273214809,48.1102456193126));
#34772=CARTESIAN_POINT('Ctrl Pts',(44.7632638423439,46.3171532316798,48.0312162196629));
#34773=CARTESIAN_POINT('Ctrl Pts',(44.7643096490701,46.3213868813149,47.9520420836223));
#34774=CARTESIAN_POINT('Ctrl Pts',(44.761371197878,46.32562053095,47.872906703128));
#34775=CARTESIAN_POINT('Ctrl Pts',(44.7544961246778,46.3298541805851,47.794236932912));
#34776=CARTESIAN_POINT('Ctrl Pts',(44.7479290590336,46.333898160083,47.7190916173384));
#34777=CARTESIAN_POINT('Ctrl Pts',(44.7377706425223,46.3379421395809,47.6443714367161));
#34778=CARTESIAN_POINT('Ctrl Pts',(44.7241057095372,46.3419861190788,47.5704384889254));
#34779=CARTESIAN_POINT('Ctrl Pts',(44.7097907356966,46.3462224706795,47.492988550844));
#34780=CARTESIAN_POINT('Ctrl Pts',(44.6915728757931,46.3504588222802,47.4161079843623));
#34781=CARTESIAN_POINT('Ctrl Pts',(44.6695111642325,46.3546951738808,47.3402201000908));
#34782=CARTESIAN_POINT('Ctrl Pts',(44.6474814451446,46.3589253821973,47.26444226354));
#34783=CARTESIAN_POINT('Ctrl Pts',(44.6216190735712,46.3631555905138,47.189654697226));
#34784=CARTESIAN_POINT('Ctrl Pts',(44.592034243633,46.3673857988303,47.1162713563314));
#34785=CARTESIAN_POINT('Ctrl Pts',(44.5624840160413,46.3716110595052,47.0429738444173));
#34786=CARTESIAN_POINT('Ctrl Pts',(44.5292201564919,46.3758363201802,46.971077727025));
#34787=CARTESIAN_POINT('Ctrl Pts',(44.492402437075,46.3800615808551,46.9009811274493));
#34788=CARTESIAN_POINT('Ctrl Pts',(44.4556083059308,46.384284134502,46.8309294371654));
#34789=CARTESIAN_POINT('Ctrl Pts',(44.4152650516619,46.3885066881488,46.7626753906071));
#34790=CARTESIAN_POINT('Ctrl Pts',(44.3715797613306,46.3927292417956,46.696595348477));
#34791=CARTESIAN_POINT('Ctrl Pts',(44.3279088308731,46.396950407439,46.6305370276418));
#34792=CARTESIAN_POINT('Ctrl Pts',(44.2808983043025,46.4011715730822,46.5666516832776));
#34793=CARTESIAN_POINT('Ctrl Pts',(44.230799463836,46.4053927387255,46.5052880665098));
#34794=CARTESIAN_POINT('Ctrl Pts',(44.1807014627008,46.4096138336495,46.443925477798));
#34795=CARTESIAN_POINT('Ctrl Pts',(44.1275155482453,46.4138349285735,46.3850848952801));
#34796=CARTESIAN_POINT('Ctrl Pts',(44.0715333412382,46.4180560234974,46.3290820696309));
#34797=CARTESIAN_POINT('Ctrl Pts',(44.0154953868851,46.4222813218076,46.2730234761036));
#34798=CARTESIAN_POINT('Ctrl Pts',(43.9566559099006,46.4265066201179,46.2198086170687));
#34799=CARTESIAN_POINT('Ctrl Pts',(43.8953430429374,46.4307319184281,46.1697159715392));
#34800=CARTESIAN_POINT('Ctrl Pts',(43.8340008677528,46.4349592364771,46.1195993811769));
#34801=CARTESIAN_POINT('Ctrl Pts',(43.7701833255224,46.4391865545262,46.0726082561226));
#34802=CARTESIAN_POINT('Ctrl Pts',(43.7042491842033,46.4434138725752,46.028978816348));
#34803=CARTESIAN_POINT('Ctrl Pts',(43.6381949096214,46.4476488928784,45.9852698829021));
#34804=CARTESIAN_POINT('Ctrl Pts',(43.5700167345931,46.4518839131816,45.9449351136142));
#34805=CARTESIAN_POINT('Ctrl Pts',(43.5000995997961,46.4561189334847,45.9081655630934));
#34806=CARTESIAN_POINT('Ctrl Pts',(43.4335510894747,46.4601499094847,45.8731675784154));
#34807=CARTESIAN_POINT('Ctrl Pts',(43.3654276541714,46.4641808854847,45.8413993118555));
#34808=CARTESIAN_POINT('Ctrl Pts',(43.2960761658031,46.4682118614847,45.8129842373729));
#34809=CARTESIAN_POINT('Ctrl Pts',(43.2231943976194,46.4724480309643,45.7831227171648));
#34810=CARTESIAN_POINT('Ctrl Pts',(43.1486802469155,46.4766842004438,45.7568517691367));
#34811=CARTESIAN_POINT('Ctrl Pts',(43.0729216966716,46.4809203699234,45.7343506822439));
#34812=CARTESIAN_POINT('Ctrl Pts',(42.9972727479057,46.485150410848,45.7118821481438));
#34813=CARTESIAN_POINT('Ctrl Pts',(42.9203834206851,46.4893804517726,45.6931727769525));
#34814=CARTESIAN_POINT('Ctrl Pts',(42.84266149648,46.4936104926973,45.678353765012));
#34815=CARTESIAN_POINT('Ctrl Pts',(42.7650300620964,46.497835608684,45.663552006501));
#34816=CARTESIAN_POINT('Ctrl Pts',(42.6865684155536,46.5020607246708,45.6526316937259));
#34817=CARTESIAN_POINT('Ctrl Pts',(42.6076978358981,46.5062858406575,45.6456737588297));
#34818=CARTESIAN_POINT('Ctrl Pts',(42.5288775305307,46.5105082634385,45.6387202591135));
#34819=CARTESIAN_POINT('Ctrl Pts',(42.4496492755223,46.5147306862195,45.6357241653015));
#34820=CARTESIAN_POINT('Ctrl Pts',(42.3704416321956,46.5189531090005,45.6367148407793));
#34821=CARTESIAN_POINT('Ctrl Pts',(42.2912597658661,46.5231741576543,45.637705193856));
#34822=CARTESIAN_POINT('Ctrl Pts',(42.21209896668,46.527395206308,45.6426797340462));
#34823=CARTESIAN_POINT('Ctrl Pts',(42.1333884725642,46.5316162549618,45.651615718342));
#34824=CARTESIAN_POINT('Ctrl Pts',(42.0546790371533,46.5358372468398,45.6605515824433));
#34825=CARTESIAN_POINT('Ctrl Pts',(41.9764203607963,46.5400582387179,45.673448730472));
#34826=CARTESIAN_POINT('Ctrl Pts',(41.8990357375915,46.5442792305959,45.6902326418686));
#34827=CARTESIAN_POINT('Ctrl Pts',(41.8215736413307,46.5485044482894,45.7070333563567));
#34828=CARTESIAN_POINT('Ctrl Pts',(41.744987805847,46.552729665983,45.7277285076792));
#34829=CARTESIAN_POINT('Ctrl Pts',(41.6696899214558,46.5569548836765,45.7521927061964));
#34830=CARTESIAN_POINT('Ctrl Pts',(41.5943558275568,46.5611821332074,45.7766686691422));
#34831=CARTESIAN_POINT('Ctrl Pts',(41.520311357542,46.5654093827383,45.8049171225106));
#34832=CARTESIAN_POINT('Ctrl Pts',(41.447949221445,46.5696366322692,45.8367640544885));
#34833=CARTESIAN_POINT('Ctrl Pts',(41.3754548756137,46.5738716052251,45.8686691726208));
#34834=CARTESIAN_POINT('Ctrl Pts',(41.3046494261874,46.5781065781811,45.9041856961053));
#34835=CARTESIAN_POINT('Ctrl Pts',(41.2359017471559,46.582341551137,45.9430931721088));
#34836=CARTESIAN_POINT('Ctrl Pts',(41.1704487079906,46.5863735687216,45.9801360597606));
#34837=CARTESIAN_POINT('Ctrl Pts',(41.1068610136877,46.5904055863061,46.0202521262543));
#34838=CARTESIAN_POINT('Ctrl Pts',(41.0454303341048,46.5944376038906,46.0632162069202));
#34839=CARTESIAN_POINT('Ctrl Pts',(40.9813670517248,46.5986424129996,46.1080215069851));
#34840=CARTESIAN_POINT('Ctrl Pts',(40.9193984368704,46.6028472221085,46.1561003933127));
#34841=CARTESIAN_POINT('Ctrl Pts',(40.8598822810811,46.6070520312174,46.2072290015811));
#34842=CARTESIAN_POINT('Ctrl Pts',(40.8004528399889,46.6112507139437,46.2582831157609));
#34843=CARTESIAN_POINT('Ctrl Pts',(40.7434691234988,46.6154493966699,46.3123778236317));
#34844=CARTESIAN_POINT('Ctrl Pts',(40.6892595063388,46.6196480793961,46.3692463692367));
#34845=CARTESIAN_POINT('Ctrl Pts',(40.6351126114818,46.6238419041089,46.4260491160713));
#34846=CARTESIAN_POINT('Ctrl Pts',(40.5837337673293,46.6280357288216,46.4856189820183));
#34847=CARTESIAN_POINT('Ctrl Pts',(40.5354165933514,46.6322295535344,46.5476504688778));
#34848=CARTESIAN_POINT('Ctrl Pts',(40.4871295028087,46.636420767071,46.609643333441));
#34849=CARTESIAN_POINT('Ctrl Pts',(40.4419005926706,46.6406119806076,46.6740944028798));
#34850=CARTESIAN_POINT('Ctrl Pts',(40.399984167694,46.6448031941441,46.7406640196416));
#34851=CARTESIAN_POINT('Ctrl Pts',(40.3580802737597,46.6489931547047,46.8072137352147));
#34852=CARTESIAN_POINT('Ctrl Pts',(40.3194871530234,46.6531831152653,46.8758803375015));
#34853=CARTESIAN_POINT('Ctrl Pts',(40.2844156950254,46.6573730758259,46.9462953499936));
#34854=CARTESIAN_POINT('Ctrl Pts',(40.2493433702582,46.6615631399387,47.0167121027487));
#34855=CARTESIAN_POINT('Ctrl Pts',(40.2177930917328,46.6657532040516,47.0888769236911));
#34856=CARTESIAN_POINT('Ctrl Pts',(40.1899289772536,46.6699432681644,47.1623983552328));
#34857=CARTESIAN_POINT('Ctrl Pts',(40.162036879065,46.6741375403254,47.2359936237658));
#34858=CARTESIAN_POINT('Ctrl Pts',(40.1378385045712,46.6783318124865,47.3109477759341));
#34859=CARTESIAN_POINT('Ctrl Pts',(40.1174488569127,46.6825260846475,47.3868517959816));
#34860=CARTESIAN_POINT('Ctrl Pts',(40.0970482647868,46.6867226081508,47.4627965587186));
#34861=CARTESIAN_POINT('Ctrl Pts',(40.0804605684087,46.6909191316541,47.5396917377188));
#34862=CARTESIAN_POINT('Ctrl Pts',(40.0677495871925,46.6951156551574,47.6171182260029));
#34863=CARTESIAN_POINT('Ctrl Pts',(40.0550169035634,46.6993193437005,47.6946769103458));
#34864=CARTESIAN_POINT('Ctrl Pts',(40.0461742027216,46.7035230322435,47.7727682411818));
#34865=CARTESIAN_POINT('Ctrl Pts',(40.0412333527236,46.7077267207866,47.850968645593));
#34866=CARTESIAN_POINT('Ctrl Pts',(40.0380808672715,46.7104088639365,47.9008640355258));
#34867=CARTESIAN_POINT('Ctrl Pts',(40.0365157731703,46.7130910070864,47.9508038052924));
#34868=CARTESIAN_POINT('Ctrl Pts',(40.0365300974769,46.7157731502363,48.000678798438));
#34869=CARTESIAN_POINT('Origin',(42.4,48.4493818343519,48.));
#34870=CARTESIAN_POINT('',(40.4708708151857,32.1775068343172,48.0017734705773));
#34871=CARTESIAN_POINT('Ctrl Pts',(41.794138831786,32.3337813919524,49.8315225365117));
#34872=CARTESIAN_POINT('Ctrl Pts',(41.7886782500385,32.3333951108295,49.8297161954099));
#34873=CARTESIAN_POINT('Ctrl Pts',(41.7832256701112,32.333010105823,49.8278854083931));
#34874=CARTESIAN_POINT('Ctrl Pts',(41.7717294671852,32.3321999839773,49.8239680839032));
#34875=CARTESIAN_POINT('Ctrl Pts',(41.7656878576262,32.331775190185,49.8218758306898));
#34876=CARTESIAN_POINT('Ctrl Pts',(41.7549590389245,32.3310226658072,49.818100524036));
#34877=CARTESIAN_POINT('Ctrl Pts',(41.750267836368,32.3306942574116,49.8164293199577));
#34878=CARTESIAN_POINT('Ctrl Pts',(41.740062550579,32.329981234195,49.8127491712764));
#34879=CARTESIAN_POINT('Ctrl Pts',(41.7345511388645,32.3295970385137,49.8107332245768));
#34880=CARTESIAN_POINT('Ctrl Pts',(41.719807971515,32.3285714368358,49.8052641102468));
#34881=CARTESIAN_POINT('Ctrl Pts',(41.7105931909916,32.3279326625102,49.8017652358244));
#34882=CARTESIAN_POINT('Ctrl Pts',(41.6549588428836,32.324087358939,49.7801514297329));
#34883=CARTESIAN_POINT('Ctrl Pts',(41.6092242731332,32.3209740058822,49.7603125122545));
#34884=CARTESIAN_POINT('Ctrl Pts',(41.4367611911365,32.3092305662373,49.6774203503844));
#34885=CARTESIAN_POINT('Ctrl Pts',(41.3163440513153,32.3009949294976,49.602267998054));
#34886=CARTESIAN_POINT('Ctrl Pts',(41.1418884809709,32.2875473795785,49.4646521162385));
#34887=CARTESIAN_POINT('Ctrl Pts',(41.0817544458631,32.2825785173526,49.4107716797351));
#34888=CARTESIAN_POINT('Ctrl Pts',(41.0126677973322,32.2763154243633,49.3405855876347));
#34889=CARTESIAN_POINT('Ctrl Pts',(41.0003391713107,32.2751744139912,49.327708510472));
#34890=CARTESIAN_POINT('Ctrl Pts',(40.9811716296557,32.2733619595949,49.3071245959298));
#34891=CARTESIAN_POINT('Ctrl Pts',(40.9742127639004,32.2726956732212,49.2995304553285));
#34892=CARTESIAN_POINT('Ctrl Pts',(40.9613827771837,32.2714515228676,49.2853021119403));
#34893=CARTESIAN_POINT('Ctrl Pts',(40.9554958680582,32.2708743482146,49.2786824629801));
#34894=CARTESIAN_POINT('Ctrl Pts',(40.9425244019797,32.2695883164697,49.2638925503667));
#34895=CARTESIAN_POINT('Ctrl Pts',(40.9354625748005,32.268878539553,49.2557028389643));
#34896=CARTESIAN_POINT('Ctrl Pts',(40.9160472984658,32.2668998177003,49.232800068835));
#34897=CARTESIAN_POINT('Ctrl Pts',(40.9038444957099,32.2656247932808,49.2179615312213));
#34898=CARTESIAN_POINT('Ctrl Pts',(40.8350337196072,32.2582493481227,49.131693242776));
#34899=CARTESIAN_POINT('Ctrl Pts',(40.78333075363,32.2519582845867,49.0565156218265));
#34900=CARTESIAN_POINT('Ctrl Pts',(40.6973836322991,32.240006539079,48.9103789886614));
#34901=CARTESIAN_POINT('Ctrl Pts',(40.6617881943141,32.2343928873117,48.8404232095297));
#34902=CARTESIAN_POINT('Ctrl Pts',(40.5920584116766,32.2219013084359,48.6798721347924));
#34903=CARTESIAN_POINT('Ctrl Pts',(40.5602747001927,32.2150479309445,48.5884676141541));
#34904=CARTESIAN_POINT('Ctrl Pts',(40.5327816114671,32.207814182667,48.4849206391801));
#34905=CARTESIAN_POINT('Ctrl Pts',(40.530173009105,32.2071101367896,48.4747626489807));
#34906=CARTESIAN_POINT('Ctrl Pts',(40.5260985363842,32.2059815621403,48.4583418160482));
#34907=CARTESIAN_POINT('Ctrl Pts',(40.5245809627852,32.2055542574737,48.4520921957861));
#34908=CARTESIAN_POINT('Ctrl Pts',(40.5219404904334,32.2047983045004,48.4409761623109));
#34909=CARTESIAN_POINT('Ctrl Pts',(40.52080520832,32.2044689657767,48.4361128684041));
#34910=CARTESIAN_POINT('Ctrl Pts',(40.5183764236116,32.2037548602556,48.425522900488));
#34911=CARTESIAN_POINT('Ctrl Pts',(40.5170901699271,32.2033705065886,48.4197947071277));
#34912=CARTESIAN_POINT('Ctrl Pts',(40.5144844887396,32.2025786931522,48.4079376366705));
#34913=CARTESIAN_POINT('Ctrl Pts',(40.5131687454796,32.2021714395008,48.4018080115956));
#34914=CARTESIAN_POINT('Ctrl Pts',(40.5098570521573,32.2011265739235,48.3860048585975));
#34915=CARTESIAN_POINT('Ctrl Pts',(40.5079054436263,32.2004912822652,48.3763220871882));
#34916=CARTESIAN_POINT('Ctrl Pts',(40.5023681338805,32.1986277657745,48.3477165039367));
#34917=CARTESIAN_POINT('Ctrl Pts',(40.4989912261293,32.1974095732903,48.3287539631835));
#34918=CARTESIAN_POINT('Ctrl Pts',(40.4793365194097,32.189737888435,48.2079295422149));
#34919=CARTESIAN_POINT('Ctrl Pts',(40.4709658658183,32.1835991181717,48.1049438817111));
#34920=CARTESIAN_POINT('Ctrl Pts',(40.4708708187116,32.1774426331651,48.0017773017898));
#34921=CARTESIAN_POINT('',(43.9476533605231,31.6998,49.1516560391721));
#34922=CARTESIAN_POINT('Ctrl Pts',(40.4708708151857,32.1775068343172,48.0017734705773));
#34923=CARTESIAN_POINT('Ctrl Pts',(40.4708092245439,32.1731176722038,47.9347769800571));
#34924=CARTESIAN_POINT('Ctrl Pts',(40.4742419471142,32.1687285100904,47.8676805505439));
#34925=CARTESIAN_POINT('Ctrl Pts',(40.4811735403552,32.164339347977,47.8008830126105));
#34926=CARTESIAN_POINT('Ctrl Pts',(40.4881000068995,32.1599534321451,47.7341348790066));
#34927=CARTESIAN_POINT('Ctrl Pts',(40.4985201638095,32.1555675163132,47.6676857020333));
#34928=CARTESIAN_POINT('Ctrl Pts',(40.512386543448,32.1511816004813,47.6019321721817));
#34929=CARTESIAN_POINT('Ctrl Pts',(40.5262477497833,32.1467973209578,47.5362031738203));
#34930=CARTESIAN_POINT('Ctrl Pts',(40.5435525244123,32.1424130414343,47.4711698040497));
#34931=CARTESIAN_POINT('Ctrl Pts',(40.5642021288926,32.1380287619108,47.4072194897456));
#34932=CARTESIAN_POINT('Ctrl Pts',(40.5848515974943,32.1336445112367,47.3432695962476));
#34933=CARTESIAN_POINT('Ctrl Pts',(40.6088456934916,32.1292602605626,47.2804032260941));
#34934=CARTESIAN_POINT('Ctrl Pts',(40.636036159954,32.1248760098885,47.2189915954934));
#34935=CARTESIAN_POINT('Ctrl Pts',(40.6632540336694,32.1204873400087,47.1575180636339));
#34936=CARTESIAN_POINT('Ctrl Pts',(40.6936744995961,32.1160986701287,47.097502661538));
#34937=CARTESIAN_POINT('Ctrl Pts',(40.7271021030885,32.1117100002489,47.0392944345904));
#34938=CARTESIAN_POINT('Ctrl Pts',(40.7605491529565,32.1073187772777,46.9810523452378));
#34939=CARTESIAN_POINT('Ctrl Pts',(40.7970065427126,32.1029275543065,46.9246199469879));
#34940=CARTESIAN_POINT('Ctrl Pts',(40.8362356319982,32.0985363313353,46.8703170540952));
#34941=CARTESIAN_POINT('Ctrl Pts',(40.8755312425507,32.0941376621114,46.815922079095));
#34942=CARTESIAN_POINT('Ctrl Pts',(40.9176076082244,32.0897389928874,46.7636642053333));
#34943=CARTESIAN_POINT('Ctrl Pts',(40.9621867732401,32.0853403236635,46.7138290619617));
#34944=CARTESIAN_POINT('Ctrl Pts',(40.9796790097263,32.0836143478122,46.6942744535954));
#34945=CARTESIAN_POINT('Ctrl Pts',(40.99755621004,32.0818883719608,46.6750924473109));
#34946=CARTESIAN_POINT('Ctrl Pts',(41.0158001753889,32.0801623961095,46.6562986185739));
#34947=CARTESIAN_POINT('Ctrl Pts',(41.0628485759409,32.0757113679671,46.607832204315));
#34948=CARTESIAN_POINT('Ctrl Pts',(41.1125409804307,32.0712603398248,46.5617415422288));
#34949=CARTESIAN_POINT('Ctrl Pts',(41.1646076147278,32.0668093116824,46.5183292500318));
#34950=CARTESIAN_POINT('Ctrl Pts',(41.2165950871786,32.0623650508606,46.4749829616632));
#34951=CARTESIAN_POINT('Ctrl Pts',(41.270949249308,32.0579207900388,46.4343072768261));
#34952=CARTESIAN_POINT('Ctrl Pts',(41.3273631296451,32.0534765292169,46.3965684606897));
#34953=CARTESIAN_POINT('Ctrl Pts',(41.3837102631183,32.0490375266839,46.3588742957563));
#34954=CARTESIAN_POINT('Ctrl Pts',(41.4421118661863,32.0445985241508,46.3241103733826));
#34955=CARTESIAN_POINT('Ctrl Pts',(41.5022289657174,32.0401595216177,46.2925019101319));
#34956=CARTESIAN_POINT('Ctrl Pts',(41.5623082273727,32.0357233130057,46.2609133413392));
#34957=CARTESIAN_POINT('Ctrl Pts',(41.6241004068553,32.0312871043936,46.2324765224017));
#34958=CARTESIAN_POINT('Ctrl Pts',(41.6872400822758,32.0268508957815,46.2073718019105));
#34959=CARTESIAN_POINT('Ctrl Pts',(41.7503619725508,32.022415936758,46.1822741529016));
#34960=CARTESIAN_POINT('Ctrl Pts',(41.8148301456332,32.0179809777345,46.1605069221356));
#34961=CARTESIAN_POINT('Ctrl Pts',(41.8802589664987,32.0135460187109,46.1422024289512));
#34962=CARTESIAN_POINT('Ctrl Pts',(41.9456921080106,32.0091107668212,46.1238967270143));
#34963=CARTESIAN_POINT('Ctrl Pts',(42.012085545857,32.0046755149315,46.1090543474025));
#34964=CARTESIAN_POINT('Ctrl Pts',(42.0790400437406,32.0002402630417,46.0977573069196));
#34965=CARTESIAN_POINT('Ctrl Pts',(42.146067428378,31.995800182931,46.0864479684636));
#34966=CARTESIAN_POINT('Ctrl Pts',(42.2136566028683,31.9913601028203,46.0786917534496));
#34967=CARTESIAN_POINT('Ctrl Pts',(42.2814007672019,31.9869200227096,46.074519078547));
#34968=CARTESIAN_POINT('Ctrl Pts',(42.3491864044555,31.9824772243856,46.0703438491363));
#34969=CARTESIAN_POINT('Ctrl Pts',(42.4171267253904,31.9780344260616,46.0697565293414));
#34970=CARTESIAN_POINT('Ctrl Pts',(42.484815352849,31.9735916277376,46.072735380696));
#34971=CARTESIAN_POINT('Ctrl Pts',(42.5526229951648,31.9691410177762,46.0757194696744));
#34972=CARTESIAN_POINT('Ctrl Pts',(42.620177568542,31.9646904078149,46.0822821953618));
#34973=CARTESIAN_POINT('Ctrl Pts',(42.6870791397067,31.9602397978536,46.0923501043312));
#34974=CARTESIAN_POINT('Ctrl Pts',(42.7186620950456,31.9581387498036,46.0971029720711));
#34975=CARTESIAN_POINT('Ctrl Pts',(42.7500996918463,31.9560377017536,46.1026362702326));
#34976=CARTESIAN_POINT('Ctrl Pts',(42.7813509885611,31.9539366537035,46.1089383985646));
#34977=CARTESIAN_POINT('Ctrl Pts',(42.8477518181369,31.949472476272,46.1223287725116));
#34978=CARTESIAN_POINT('Ctrl Pts',(42.9135772124744,31.9450082988405,46.1392470232286));
#34979=CARTESIAN_POINT('Ctrl Pts',(42.9784249626804,31.940544121409,46.1596285376457));
#34980=CARTESIAN_POINT('Ctrl Pts',(43.0431742857848,31.9360867197876,46.1799791166273));
#34981=CARTESIAN_POINT('Ctrl Pts',(43.106948444429,31.9316293181663,46.2037823800547));
#34982=CARTESIAN_POINT('Ctrl Pts',(43.1693558339415,31.9271719165449,46.2309227948786));
#34983=CARTESIAN_POINT('Ctrl Pts',(43.2316885407987,31.922719849077,46.2580307308845));
#34984=CARTESIAN_POINT('Ctrl Pts',(43.2926572782625,31.9182677816091,46.2884676911477));
#34985=CARTESIAN_POINT('Ctrl Pts',(43.3518877729144,31.9138157141411,46.3220690643903));
#34986=CARTESIAN_POINT('Ctrl Pts',(43.4110803695575,31.9093664952817,46.3556489381478));
#34987=CARTESIAN_POINT('Ctrl Pts',(43.4685365029924,31.9049172764223,46.3923889661042));
#34988=CARTESIAN_POINT('Ctrl Pts',(43.5239053920692,31.9004680575629,46.4320780546922));
#34989=CARTESIAN_POINT('Ctrl Pts',(43.5792578099748,31.8960201622598,46.4717553365456));
#34990=CARTESIAN_POINT('Ctrl Pts',(43.6325238167008,31.8915722669568,46.5143796509825));
#34991=CARTESIAN_POINT('Ctrl Pts',(43.6833821151811,31.8871243716537,46.5596969404555));
#34992=CARTESIAN_POINT('Ctrl Pts',(43.7342426953449,31.8826762768023,46.6050162630226));
#34993=CARTESIAN_POINT('Ctrl Pts',(43.782694987332,31.878228181951,46.6530284714022));
#34994=CARTESIAN_POINT('Ctrl Pts',(43.8284526329951,31.8737800870996,46.7034408489431));
#34995=CARTESIAN_POINT('Ctrl Pts',(43.8742576062804,31.8693273915361,46.7539053685451));
#34996=CARTESIAN_POINT('Ctrl Pts',(43.9173620398033,31.8648746959727,46.8067746468774));
#34997=CARTESIAN_POINT('Ctrl Pts',(43.9575188633162,31.8604220004092,46.8617216740559));
#34998=CARTESIAN_POINT('Ctrl Pts',(43.9976991946313,31.855966698238,46.9167008672208));
#34999=CARTESIAN_POINT('Ctrl Pts',(44.0349282123254,31.8515113960668,46.9737598184123));
#35000=CARTESIAN_POINT('Ctrl Pts',(44.0690028814936,31.8470560938957,47.0325435728334));
#35001=CARTESIAN_POINT('Ctrl Pts',(44.1031349884786,31.8425932816639,47.0914264158325));
#35002=CARTESIAN_POINT('Ctrl Pts',(44.1341019109925,31.8381304694322,47.1520394271205));
#35003=CARTESIAN_POINT('Ctrl Pts',(44.1617475480732,31.8336676572004,47.2140050039865));
#35004=CARTESIAN_POINT('Ctrl Pts',(44.174047567796,31.8316820752328,47.2415745555713));
#35005=CARTESIAN_POINT('Ctrl Pts',(44.1856907859411,31.8296964932652,47.2694116151986));
#35006=CARTESIAN_POINT('Ctrl Pts',(44.1966666295966,31.8277109112976,47.2974819724776));
#35007=CARTESIAN_POINT('Ctrl Pts',(44.221315821241,31.8232517560854,47.3605214651867));
#35008=CARTESIAN_POINT('Ctrl Pts',(44.2426914939263,31.8187926008732,47.4249833216754));
#35009=CARTESIAN_POINT('Ctrl Pts',(44.2606307944358,31.814333445661,47.4904947461534));
#35010=CARTESIAN_POINT('Ctrl Pts',(44.2785433129736,31.8098809476185,47.5559083672021));
#35011=CARTESIAN_POINT('Ctrl Pts',(44.2930295119248,31.805428449576,47.622367974857));
#35012=CARTESIAN_POINT('Ctrl Pts',(44.303975115198,31.8009759515335,47.6894821782782));
#35013=CARTESIAN_POINT('Ctrl Pts',(44.3149080885458,31.7965285911446,47.756518939885));
#35014=CARTESIAN_POINT('Ctrl Pts',(44.3223085006713,31.7920812307556,47.8242083130688));
#35015=CARTESIAN_POINT('Ctrl Pts',(44.3261127378193,31.7876338703667,47.8921469605884));
#35016=CARTESIAN_POINT('Ctrl Pts',(44.3299146448619,31.7831892339979,47.9600439955047));
#35017=CARTESIAN_POINT('Ctrl Pts',(44.3301247188218,31.7787445976292,48.0281895108933));
#35018=CARTESIAN_POINT('Ctrl Pts',(44.3267311582565,31.7742999612604,48.0961748444436));
#35019=CARTESIAN_POINT('Ctrl Pts',(44.323338508612,31.7698565179488,48.164141928944));
#35020=CARTESIAN_POINT('Ctrl Pts',(44.3163441693474,31.7654130746372,48.2319484249721));
#35021=CARTESIAN_POINT('Ctrl Pts',(44.3057884235369,31.7609696313256,48.299187301891));
#35022=CARTESIAN_POINT('Ctrl Pts',(44.2952318793074,31.7565258519194,48.3664312646459));
#35023=CARTESIAN_POINT('Ctrl Pts',(44.2811134727428,31.7520820725132,48.4331070366154));
#35024=CARTESIAN_POINT('Ctrl Pts',(44.2635248878602,31.747638293107,48.4988161477195));
#35025=CARTESIAN_POINT('Ctrl Pts',(44.2459171715654,31.7431896801241,48.5645967317758));
#35026=CARTESIAN_POINT('Ctrl Pts',(44.2248318721696,31.7387410671411,48.6294080797517));
#35027=CARTESIAN_POINT('Ctrl Pts',(44.2004107481887,31.7342924541581,48.6928662891976));
#35028=CARTESIAN_POINT('Ctrl Pts',(44.1759746161275,31.7298411072657,48.7563634970905));
#35029=CARTESIAN_POINT('Ctrl Pts',(44.1481987808603,31.7253897603733,48.8185054616234));
#35030=CARTESIAN_POINT('Ctrl Pts',(44.1172722746545,31.7209384134809,48.8789303110048));
#35031=CARTESIAN_POINT('Ctrl Pts',(44.0862919625275,31.7164793221372,48.9394602875111));
#35032=CARTESIAN_POINT('Ctrl Pts',(44.0521502870094,31.7120202307936,48.9982667608184));
#35033=CARTESIAN_POINT('Ctrl Pts',(44.015080659964,31.7075611394499,49.055015174635));
#35034=CARTESIAN_POINT('Ctrl Pts',(43.9982436001863,31.7055358159306,49.0807903580366));
#35035=CARTESIAN_POINT('Ctrl Pts',(43.9808030739588,31.7035104924113,49.106141402521));
#35036=CARTESIAN_POINT('Ctrl Pts',(43.9627836415489,31.701485168892,49.1310392772168));
#35037=CARTESIAN_POINT('Ctrl Pts',(43.9577859565441,31.700923445928,49.1379446964436));
#35038=CARTESIAN_POINT('Ctrl Pts',(43.9527424375441,31.700361722964,49.144817081284));
#35039=CARTESIAN_POINT('Ctrl Pts',(43.9476533605231,31.6998,49.1516560391721));
#35040=CARTESIAN_POINT('',(43.8578594651099,31.6998,46.7365965264851));
#35041=CARTESIAN_POINT('Origin',(42.4,31.6998,48.));
#35042=CARTESIAN_POINT('',(40.470870167032,32.0064681656139,47.9991972218753));
#35043=CARTESIAN_POINT('Ctrl Pts',(40.470870167032,32.0064681656139,47.9991972218753));
#35044=CARTESIAN_POINT('Ctrl Pts',(40.4709011975406,32.0016092260085,47.9246288223946));
#35045=CARTESIAN_POINT('Ctrl Pts',(40.475259964132,31.996750286403,47.8501996671079));
#35046=CARTESIAN_POINT('Ctrl Pts',(40.483873195406,31.9918913467975,47.7763918033335));
#35047=CARTESIAN_POINT('Ctrl Pts',(40.492513155862,31.9870173285907,47.7023548938321));
#35048=CARTESIAN_POINT('Ctrl Pts',(40.5054338919586,31.9821433103839,47.6289434528292));
#35049=CARTESIAN_POINT('Ctrl Pts',(40.5225112662355,31.9772692921771,47.5566281340821));
#35050=CARTESIAN_POINT('Ctrl Pts',(40.5396666955009,31.9723729964569,47.4839822861055));
#35051=CARTESIAN_POINT('Ctrl Pts',(40.5610166993639,31.9674767007366,47.4124429092672));
#35052=CARTESIAN_POINT('Ctrl Pts',(40.5863869842789,31.9625804050164,47.3424664372772));
#35053=CARTESIAN_POINT('Ctrl Pts',(40.6042268414166,31.9591374316148,47.29326043634));
#35054=CARTESIAN_POINT('Ctrl Pts',(40.6240535527847,31.9556944582133,47.2448268014045));
#35055=CARTESIAN_POINT('Ctrl Pts',(40.6457929214645,31.9522514848117,47.1973169476587));
#35056=CARTESIAN_POINT('Ctrl Pts',(40.6736626774029,31.9478376110779,47.1364095658451));
#35057=CARTESIAN_POINT('Ctrl Pts',(40.7047702000245,31.9434237373442,47.0768205595951));
#35058=CARTESIAN_POINT('Ctrl Pts',(40.7389679731072,31.9390098636104,47.0189214289689));
#35059=CARTESIAN_POINT('Ctrl Pts',(40.7731133247939,31.9346027558559,46.9611110512929));
#35060=CARTESIAN_POINT('Ctrl Pts',(40.8103392783329,31.9301956481014,46.9049858417072));
#35061=CARTESIAN_POINT('Ctrl Pts',(40.8504509007865,31.9257885403469,46.8508959376859));
#35062=CARTESIAN_POINT('Ctrl Pts',(40.8905162115877,31.9213865209042,46.7968684842135));
#35063=CARTESIAN_POINT('Ctrl Pts',(40.9334602813578,31.9169845014615,46.7448720758815));
#35064=CARTESIAN_POINT('Ctrl Pts',(40.9790440695699,31.9125824820188,46.6952292152736));
#35065=CARTESIAN_POINT('Ctrl Pts',(41.0246001405321,31.9081831392267,46.6456165400371));
#35066=CARTESIAN_POINT('Ctrl Pts',(41.0727924085359,31.9037837964345,46.5983549464344));
#35067=CARTESIAN_POINT('Ctrl Pts',(41.1233417319082,31.8993844536424,46.5537336955412));
#35068=CARTESIAN_POINT('Ctrl Pts',(41.1738785930472,31.8949861954471,46.5091234453974));
#35069=CARTESIAN_POINT('Ctrl Pts',(41.2267709791414,31.8905879372519,46.4671525800915));
#35070=CARTESIAN_POINT('Ctrl Pts',(41.281704532659,31.8861896790566,46.4280719467404));
#35071=CARTESIAN_POINT('Ctrl Pts',(41.3366444025176,31.8817909151431,46.3889868198405));
#35072=CARTESIAN_POINT('Ctrl Pts',(41.3936254931727,31.8773921512296,46.35279287411));
#35073=CARTESIAN_POINT('Ctrl Pts',(41.4523037936787,31.8729933873161,46.3196981052727));
#35074=CARTESIAN_POINT('Ctrl Pts',(41.5110540263297,31.8685892310766,46.2865627664514));
#35075=CARTESIAN_POINT('Ctrl Pts',(41.5715051800388,31.8641850748372,46.2565344326099));
#35076=CARTESIAN_POINT('Ctrl Pts',(41.6332888846635,31.8597809185977,46.2297749796934));
#35077=CARTESIAN_POINT('Ctrl Pts',(41.6951143419729,31.8553737860824,46.2029974430605));
#35078=CARTESIAN_POINT('Ctrl Pts',(41.7582736681009,31.8509666535671,46.1794933537636));
#35079=CARTESIAN_POINT('Ctrl Pts',(41.8223816805205,31.8465595210518,46.1593752055615));
#35080=CARTESIAN_POINT('Ctrl Pts',(41.8866147410499,31.8421437920512,46.1392178152068));
#35081=CARTESIAN_POINT('Ctrl Pts',(41.9517996925201,31.8377280630505,46.1224596681049));
#35082=CARTESIAN_POINT('Ctrl Pts',(42.0175403705868,31.8333123340499,46.1091623050169));
#35083=CARTESIAN_POINT('Ctrl Pts',(42.0537009136062,31.8308834701685,46.101848114106));
#35084=CARTESIAN_POINT('Ctrl Pts',(42.0900294839137,31.8284546062872,46.0955800777092));
#35085=CARTESIAN_POINT('Ctrl Pts',(42.1264598712172,31.8260257424059,46.0903617214652));
#35086=CARTESIAN_POINT('Ctrl Pts',(42.1951041302893,31.8214491355164,46.0805289904826));
#35087=CARTESIAN_POINT('Ctrl Pts',(42.2643926296832,31.8168725286268,46.074385533138));
#35088=CARTESIAN_POINT('Ctrl Pts',(42.3339066447597,31.8122959217373,46.072002534936));
#35089=CARTESIAN_POINT('Ctrl Pts',(42.4051024326407,31.8076085916649,46.0695618841648));
#35090=CARTESIAN_POINT('Ctrl Pts',(42.4765343220368,31.8029212615926,46.0710661782557));
#35091=CARTESIAN_POINT('Ctrl Pts',(42.5477432913384,31.7982339315202,46.0765358134957));
#35092=CARTESIAN_POINT('Ctrl Pts',(42.6170367640556,31.7936726890015,46.0818583174443));
#35093=CARTESIAN_POINT('Ctrl Pts',(42.6861186630357,31.7891114464829,46.0909354908467));
#35094=CARTESIAN_POINT('Ctrl Pts',(42.7545645738241,31.7845502039642,46.1037335314126));
#35095=CARTESIAN_POINT('Ctrl Pts',(42.8229452737836,31.7799933071019,46.1165193788347));
#35096=CARTESIAN_POINT('Ctrl Pts',(42.8906907376217,31.7754364102396,46.1330189646288));
#35097=CARTESIAN_POINT('Ctrl Pts',(42.957383288383,31.7708795133773,46.1531468854477));
#35098=CARTESIAN_POINT('Ctrl Pts',(43.0240307330039,31.7663256984788,46.1732611931598));
#35099=CARTESIAN_POINT('Ctrl Pts',(43.0896262391683,31.7617718835803,46.1969988247196));
#35100=CARTESIAN_POINT('Ctrl Pts',(43.1537653134501,31.7572180686819,46.2242239980393));
#35101=CARTESIAN_POINT('Ctrl Pts',(43.2211582915429,31.752433229625,46.252830358977));
#35102=CARTESIAN_POINT('Ctrl Pts',(43.2869426173446,31.7476483905682,46.2852873672686));
#35103=CARTESIAN_POINT('Ctrl Pts',(43.3506717289978,31.7428635515114,46.3213797866747));
#35104=CARTESIAN_POINT('Ctrl Pts',(43.4113091777405,31.7383108372883,46.3557212701029));
#35105=CARTESIAN_POINT('Ctrl Pts',(43.4700857694018,31.7337581230652,46.393353355447));
#35106=CARTESIAN_POINT('Ctrl Pts',(43.5266429201655,31.7292054088421,46.4340439701764));
#35107=CARTESIAN_POINT('Ctrl Pts',(43.5832059084648,31.7246522247115,46.4747387847798));
#35108=CARTESIAN_POINT('Ctrl Pts',(43.6375486304879,31.7200990405808,46.5184924801764));
#35109=CARTESIAN_POINT('Ctrl Pts',(43.6893437163278,31.7155458564502,46.565031241432));
#35110=CARTESIAN_POINT('Ctrl Pts',(43.7411749505203,31.7109894946029,46.6116024825943));
#35111=CARTESIAN_POINT('Ctrl Pts',(43.7904546638894,31.7064331327557,46.6609623523788));
#35112=CARTESIAN_POINT('Ctrl Pts',(43.8368913921465,31.7018767709084,46.7127992836875));
#35113=CARTESIAN_POINT('Ctrl Pts',(43.8439466151188,31.7011845139389,46.7206749700744));
#35114=CARTESIAN_POINT('Ctrl Pts',(43.8509362865415,31.7004922569695,46.7286077710193));
#35115=CARTESIAN_POINT('Ctrl Pts',(43.8578594651099,31.6998,46.7365965264851));
#35116=CARTESIAN_POINT('Ctrl Pts',(40.4708701307726,32.004994408738,47.9992896799358));
#35117=CARTESIAN_POINT('Ctrl Pts',(40.4708627806638,32.006246742668,48.019251546574));
#35118=CARTESIAN_POINT('Ctrl Pts',(40.4711652667494,32.0075076083347,48.0392118611536));
#35119=CARTESIAN_POINT('Ctrl Pts',(40.4722595512005,32.0097780261629,48.0748761664676));
#35120=CARTESIAN_POINT('Ctrl Pts',(40.4729336918832,32.0107839605529,48.0905820021913));
#35121=CARTESIAN_POINT('Ctrl Pts',(40.4742865346698,32.0123646478213,48.1151012709811));
#35122=CARTESIAN_POINT('Ctrl Pts',(40.4748340034472,32.012935338653,48.1239214856286));
#35123=CARTESIAN_POINT('Ctrl Pts',(40.4760361467134,32.0140673468661,48.1413513319663));
#35124=CARTESIAN_POINT('Ctrl Pts',(40.4766880604071,32.0146285658266,48.1499609509146));
#35125=CARTESIAN_POINT('Ctrl Pts',(40.4782001442076,32.0158281715614,48.1682948913855));
#35126=CARTESIAN_POINT('Ctrl Pts',(40.4790763729743,32.016467042734,48.1780176099576));
#35127=CARTESIAN_POINT('Ctrl Pts',(40.4815310931312,32.0181238404701,48.2031223876356));
#35128=CARTESIAN_POINT('Ctrl Pts',(40.4832207742616,32.01914519036,48.2184926253707));
#35129=CARTESIAN_POINT('Ctrl Pts',(40.4908944015245,32.0233503744575,48.2813314655605));
#35130=CARTESIAN_POINT('Ctrl Pts',(40.4984580254018,32.0265824797393,48.3285864122701));
#35131=CARTESIAN_POINT('Ctrl Pts',(40.5385013013827,32.0406916259529,48.5303692624794));
#35132=CARTESIAN_POINT('Ctrl Pts',(40.5881266008019,32.0520648312043,48.6808605516744));
#35133=CARTESIAN_POINT('Ctrl Pts',(40.6737664730247,32.0662119589922,48.8622577614324));
#35134=CARTESIAN_POINT('Ctrl Pts',(40.6933016176098,32.069201237967,48.9003064586181));
#35135=CARTESIAN_POINT('Ctrl Pts',(40.7224301145485,32.0733186864852,48.9526786002534));
#35136=CARTESIAN_POINT('Ctrl Pts',(40.7309741434781,32.0744896615469,48.967569103407));
#35137=CARTESIAN_POINT('Ctrl Pts',(40.7463153549934,32.0765266631546,48.9934976615909));
#35138=CARTESIAN_POINT('Ctrl Pts',(40.7530270446214,32.0773970370017,49.0045847971862));
#35139=CARTESIAN_POINT('Ctrl Pts',(40.7632177908763,32.0786870647035,49.021042347508));
#35140=CARTESIAN_POINT('Ctrl Pts',(40.7666125005188,32.079111738868,49.0264642004913));
#35141=CARTESIAN_POINT('Ctrl Pts',(40.7724859266638,32.079837752799,49.0357420084307));
#35142=CARTESIAN_POINT('Ctrl Pts',(40.7749515128934,32.0801399266426,49.0396061673923));
#35143=CARTESIAN_POINT('Ctrl Pts',(40.7805996582828,32.0808262099835,49.0483889592649));
#35144=CARTESIAN_POINT('Ctrl Pts',(40.7837908817173,32.0812097457134,49.0533019343326));
#35145=CARTESIAN_POINT('Ctrl Pts',(40.7926643282636,32.0822648566423,49.066827566897));
#35146=CARTESIAN_POINT('Ctrl Pts',(40.7983934424351,32.082933435362,49.0754094407244));
#35147=CARTESIAN_POINT('Ctrl Pts',(40.8297882516345,32.0865318647349,49.1216295926669));
#35148=CARTESIAN_POINT('Ctrl Pts',(40.8567143551735,32.0893859367888,49.1583989078264));
#35149=CARTESIAN_POINT('Ctrl Pts',(40.9936490432383,32.1030102574597,49.3321302540539));
#35150=CARTESIAN_POINT('Ctrl Pts',(41.1207104482148,32.1131255583394,49.4545860986199));
#35151=CARTESIAN_POINT('Ctrl Pts',(41.29172446324,32.1261562670014,49.5794202035729));
#35152=CARTESIAN_POINT('Ctrl Pts',(41.3214387021441,32.1283986821038,49.5998587870614));
#35153=CARTESIAN_POINT('Ctrl Pts',(41.3670653712595,32.1318229677713,49.6293935461119));
#35154=CARTESIAN_POINT('Ctrl Pts',(41.382564013842,32.1329829233396,49.6391159978181));
#35155=CARTESIAN_POINT('Ctrl Pts',(41.4080311090721,32.1348852155009,49.6545913889043));
#35156=CARTESIAN_POINT('Ctrl Pts',(41.4179171073616,32.1356227606144,49.6604782827849));
#35157=CARTESIAN_POINT('Ctrl Pts',(41.4370348504081,32.1370476868972,49.6716320262033));
#35158=CARTESIAN_POINT('Ctrl Pts',(41.4462586410076,32.1377345776486,49.6769117219052));
#35159=CARTESIAN_POINT('Ctrl Pts',(41.4631418143845,32.1389910156643,49.6863912933081));
#35160=CARTESIAN_POINT('Ctrl Pts',(41.4707870415153,32.1395596585546,49.6906159018776));
#35161=CARTESIAN_POINT('Ctrl Pts',(41.4874912159891,32.1408015587082,49.6996987792366));
#35162=CARTESIAN_POINT('Ctrl Pts',(41.4965607920905,32.1414755120483,49.7045368320232));
#35163=CARTESIAN_POINT('Ctrl Pts',(41.5212500645083,32.1433094770585,49.7174546159945));
#35164=CARTESIAN_POINT('Ctrl Pts',(41.5369419645521,32.1444743813436,49.7253934622963));
#35165=CARTESIAN_POINT('Ctrl Pts',(41.6200254063973,32.150640158119,49.7660100611101));
#35166=CARTESIAN_POINT('Ctrl Pts',(41.6891609547765,32.1557676430686,49.7949532734779));
#35167=CARTESIAN_POINT('Ctrl Pts',(41.7712093451674,32.1618454763861,49.8238177671504));
#35168=CARTESIAN_POINT('Ctrl Pts',(41.7826573950548,32.1626932439883,49.8277245182302));
#35169=CARTESIAN_POINT('Ctrl Pts',(41.7941388784248,32.1635431008229,49.8315225519397));
#35170=CARTESIAN_POINT('Origin',(42.4,31.6998,48.));
#35171=CARTESIAN_POINT('',(40.2836156024077,31.6998,46.9479032732073));
#35172=CARTESIAN_POINT('Origin',(42.4,31.6998,48.));
#35173=CARTESIAN_POINT('Ctrl Pts',(40.2836156024078,31.6998,46.9479032732073));
#35174=CARTESIAN_POINT('Ctrl Pts',(40.3278926679427,31.6998,46.8769610634086));
#35175=CARTESIAN_POINT('Ctrl Pts',(40.3762433003066,31.6998,46.8085972732121));
#35176=CARTESIAN_POINT('Ctrl Pts',(40.4283168746136,31.6998,46.7430091960712));
#35177=CARTESIAN_POINT('Ctrl Pts',(40.4725499800367,31.6998,46.6872964018317));
#35178=CARTESIAN_POINT('Ctrl Pts',(40.5194704001647,31.6998,46.6335868254742));
#35179=CARTESIAN_POINT('Ctrl Pts',(40.5688802061001,31.6998,46.5820255156089));
#35180=CARTESIAN_POINT('Ctrl Pts',(40.5804814395833,31.6998,46.5699191172306));
#35181=CARTESIAN_POINT('Ctrl Pts',(40.5922183828339,31.6998,46.5579330154579));
#35182=CARTESIAN_POINT('Ctrl Pts',(40.6040806009517,31.6998,46.5460766914988));
#35183=CARTESIAN_POINT('Ctrl Pts',(40.6628239074511,31.6998,46.4873625736696));
#35184=CARTESIAN_POINT('Ctrl Pts',(40.7246897231953,31.6998,46.4317723406803));
#35185=CARTESIAN_POINT('Ctrl Pts',(40.7893476148646,31.6998,46.3795180785659));
#35186=CARTESIAN_POINT('Ctrl Pts',(40.8357795880102,31.6998,46.3419933707134));
#35187=CARTESIAN_POINT('Ctrl Pts',(40.8836521335364,31.6998,46.3061898568887));
#35188=CARTESIAN_POINT('Ctrl Pts',(40.9328489705532,31.6998,46.2722015277962));
#35189=CARTESIAN_POINT('Ctrl Pts',(40.9448895535959,31.6998,46.2638831210909));
#35190=CARTESIAN_POINT('Ctrl Pts',(40.9570094754657,31.6998,46.2556735073344));
#35191=CARTESIAN_POINT('Ctrl Pts',(40.9692070552756,31.6998,46.2475741931581));
#35192=CARTESIAN_POINT('Ctrl Pts',(40.9813625143741,31.6998,46.2395028475525));
#35193=CARTESIAN_POINT('Ctrl Pts',(40.9935877226732,31.6998,46.2315459621755));
#35194=CARTESIAN_POINT('Ctrl Pts',(41.0058778593767,31.6998,46.2237064435508));
#35195=CARTESIAN_POINT('Ctrl Pts',(41.0743104083663,31.6998,46.1800553227145));
#35196=CARTESIAN_POINT('Ctrl Pts',(41.1447837982158,31.6998,46.1400195296668));
#35197=CARTESIAN_POINT('Ctrl Pts',(41.2169884141849,31.6998,46.1037900354922));
#35198=CARTESIAN_POINT('Ctrl Pts',(41.2875858943175,31.6998,46.0683669401558));
#35199=CARTESIAN_POINT('Ctrl Pts',(41.3598393097106,31.6998,46.0365823804477));
#35200=CARTESIAN_POINT('Ctrl Pts',(41.4334713794664,31.6998,46.0086619738273));
#35201=CARTESIAN_POINT('Ctrl Pts',(41.5055827727076,31.6998,45.9813181896864));
#35202=CARTESIAN_POINT('Ctrl Pts',(41.5790172237879,31.6998,45.9576804264826));
#35203=CARTESIAN_POINT('Ctrl Pts',(41.6535138228268,31.6998,45.9380090899685));
#35204=CARTESIAN_POINT('Ctrl Pts',(41.6874584785425,31.6998,45.9290457714539));
#35205=CARTESIAN_POINT('Ctrl Pts',(41.7216235827886,31.6998,45.9209066525431));
#35206=CARTESIAN_POINT('Ctrl Pts',(41.7559837827323,31.6998,45.9136199602272));
#35207=CARTESIAN_POINT('Ctrl Pts',(41.7681538566628,31.6998,45.9110390793144));
#35208=CARTESIAN_POINT('Ctrl Pts',(41.7803434987159,31.6998,45.9085662449037));
#35209=CARTESIAN_POINT('Ctrl Pts',(41.7925438080729,31.6998,45.9062038693017));
#35210=CARTESIAN_POINT('Ctrl Pts',(41.8673941835534,31.6998,45.8917104088767));
#35211=CARTESIAN_POINT('Ctrl Pts',(41.9427350306394,31.6998,45.8813514036828));
#35212=CARTESIAN_POINT('Ctrl Pts',(42.0183083661715,31.6998,45.8753295077184));
#35213=CARTESIAN_POINT('Ctrl Pts',(42.0438483937305,31.6998,45.8732944064779));
#35214=CARTESIAN_POINT('Ctrl Pts',(42.069414977119,31.6998,45.8717550820673));
#35215=CARTESIAN_POINT('Ctrl Pts',(42.0949980865043,31.6998,45.8707207179083));
#35216=CARTESIAN_POINT('Ctrl Pts',(42.1725910153043,31.6998,45.8675835173696));
#35217=CARTESIAN_POINT('Ctrl Pts',(42.2503372664716,31.6998,45.8690877185585));
#35218=CARTESIAN_POINT('Ctrl Pts',(42.3278997019256,31.6998,45.87507693665));
#35219=CARTESIAN_POINT('Ctrl Pts',(42.4026205805095,31.6998,45.8808467353317));
#35220=CARTESIAN_POINT('Ctrl Pts',(42.4771715618792,31.6998,45.8907797086975));
#35221=CARTESIAN_POINT('Ctrl Pts',(42.5512293212772,31.6998,45.9047761999135));
#35222=CARTESIAN_POINT('Ctrl Pts',(42.5694631410037,31.6998,45.9082222871258));
#35223=CARTESIAN_POINT('Ctrl Pts',(42.5876734448574,31.6998,45.9119164301344));
#35224=CARTESIAN_POINT('Ctrl Pts',(42.6058197878003,31.6998,45.9158493587107));
#35225=CARTESIAN_POINT('Ctrl Pts',(42.6799748837184,31.6998,45.9319212855299));
#35226=CARTESIAN_POINT('Ctrl Pts',(42.7531518432347,31.6998,45.9519905284711));
#35227=CARTESIAN_POINT('Ctrl Pts',(42.82504465412,31.6998,45.9758841810461));
#35228=CARTESIAN_POINT('Ctrl Pts',(42.8966173594445,31.6998,45.9996714461958));
#35229=CARTESIAN_POINT('Ctrl Pts',(42.966918187902,31.6998,46.027249759349));
#35230=CARTESIAN_POINT('Ctrl Pts',(43.0356198557269,31.6998,46.0584926500212));
#35231=CARTESIAN_POINT('Ctrl Pts',(43.1037385474373,31.6998,46.0894704254554));
#35232=CARTESIAN_POINT('Ctrl Pts',(43.1702858755638,31.6998,46.1240514433707));
#35233=CARTESIAN_POINT('Ctrl Pts',(43.2349057444967,31.6998,46.162146870017));
#35234=CARTESIAN_POINT('Ctrl Pts',(43.2584962714637,31.6998,46.1760542208745));
#35235=CARTESIAN_POINT('Ctrl Pts',(43.2818295034026,31.6998,46.1904302386159));
#35236=CARTESIAN_POINT('Ctrl Pts',(43.3048865617406,31.6998,46.2052715243424));
#35237=CARTESIAN_POINT('Ctrl Pts',(43.3148243102554,31.6998,46.2116682191429));
#35238=CARTESIAN_POINT('Ctrl Pts',(43.3247094403455,31.6998,46.2181505929569));
#35239=CARTESIAN_POINT('Ctrl Pts',(43.3345306217168,31.6998,46.2247115366551));
#35240=CARTESIAN_POINT('Ctrl Pts',(43.3953085048616,31.6998,46.2653136041996));
#35241=CARTESIAN_POINT('Ctrl Pts',(43.4537463558528,31.6998,46.308989429215));
#35242=CARTESIAN_POINT('Ctrl Pts',(43.5095482320819,31.6998,46.3556161784622));
#35243=CARTESIAN_POINT('Ctrl Pts',(43.5644246533789,31.6998,46.401469639104));
#35244=CARTESIAN_POINT('Ctrl Pts',(43.6167524175643,31.6998,46.4501775666));
#35245=CARTESIAN_POINT('Ctrl Pts',(43.6662103729083,31.6998,46.501653076856));
#35246=CARTESIAN_POINT('Ctrl Pts',(43.7140843356336,31.6998,46.5514799781526));
#35247=CARTESIAN_POINT('Ctrl Pts',(43.7592697324565,31.6998,46.6039005799531));
#35248=CARTESIAN_POINT('Ctrl Pts',(43.8014309498606,31.6998,46.6588558401277));
#35249=CARTESIAN_POINT('Ctrl Pts',(43.8208980948003,31.6998,46.6842303924031));
#35250=CARTESIAN_POINT('Ctrl Pts',(43.8397198334818,31.6998,46.710145554351));
#35251=CARTESIAN_POINT('Ctrl Pts',(43.8578594651099,31.6998,46.7365965264851));
#35252=CARTESIAN_POINT('Ctrl Pts',(43.9504717140164,31.6998,49.1537532619121));
#35253=CARTESIAN_POINT('Ctrl Pts',(43.91517156945,31.6998,49.2142805813239));
#35254=CARTESIAN_POINT('Ctrl Pts',(43.876313406039,31.6998,49.2725892970532));
#35255=CARTESIAN_POINT('Ctrl Pts',(43.8342551647323,31.6998,49.3285785621835));
#35256=CARTESIAN_POINT('Ctrl Pts',(43.7956027712495,31.6998,49.3800338546398));
#35257=CARTESIAN_POINT('Ctrl Pts',(43.7542466023904,31.6998,49.4295303540662));
#35258=CARTESIAN_POINT('Ctrl Pts',(43.710427710391,31.6998,49.4769775792939));
#35259=CARTESIAN_POINT('Ctrl Pts',(43.6962200999558,31.6998,49.4923616216899));
#35260=CARTESIAN_POINT('Ctrl Pts',(43.6817503327117,31.6998,49.5075329290985));
#35261=CARTESIAN_POINT('Ctrl Pts',(43.6670459663506,31.6998,49.5224684275058));
#35262=CARTESIAN_POINT('Ctrl Pts',(43.6155359597312,31.6998,49.5747880992909));
#35263=CARTESIAN_POINT('Ctrl Pts',(43.5611098000689,31.6998,49.6242627199654));
#35264=CARTESIAN_POINT('Ctrl Pts',(43.5041269281797,31.6998,49.6707695142619));
#35265=CARTESIAN_POINT('Ctrl Pts',(43.4585949524133,31.6998,49.707930614794));
#35266=CARTESIAN_POINT('Ctrl Pts',(43.4114293717005,31.6998,49.7431966047481));
#35267=CARTESIAN_POINT('Ctrl Pts',(43.3627930380821,31.6998,49.776492738111));
#35268=CARTESIAN_POINT('Ctrl Pts',(43.3508526583872,31.6998,49.784667048244));
#35269=CARTESIAN_POINT('Ctrl Pts',(43.3388230033905,31.6998,49.7927228207283));
#35270=CARTESIAN_POINT('Ctrl Pts',(43.3267198102625,31.6998,49.8006503503805));
#35271=CARTESIAN_POINT('Ctrl Pts',(43.2630423735884,31.6998,49.8423587460136));
#35272=CARTESIAN_POINT('Ctrl Pts',(43.1972476615927,31.6998,49.8805790577778));
#35273=CARTESIAN_POINT('Ctrl Pts',(43.1297134118621,31.6998,49.91518907178));
#35274=CARTESIAN_POINT('Ctrl Pts',(43.0621791621316,31.6998,49.9497990857822));
#35275=CARTESIAN_POINT('Ctrl Pts',(42.9929045405879,31.6998,49.9807994335801));
#35276=CARTESIAN_POINT('Ctrl Pts',(42.9222254461525,31.6998,50.0080367038729));
#35277=CARTESIAN_POINT('Ctrl Pts',(42.8709659946502,31.6998,50.0277903176789));
#35278=CARTESIAN_POINT('Ctrl Pts',(42.8189669079838,31.6998,50.04556403106));
#35279=CARTESIAN_POINT('Ctrl Pts',(42.7663463649455,31.6998,50.0612861622637));
#35280=CARTESIAN_POINT('Ctrl Pts',(42.7262965849615,31.6998,50.0732523613797));
#35281=CARTESIAN_POINT('Ctrl Pts',(42.6858866223729,31.6998,50.0840299036639));
#35282=CARTESIAN_POINT('Ctrl Pts',(42.6451663824038,31.6998,50.0935820856434));
#35283=CARTESIAN_POINT('Ctrl Pts',(42.6267637139364,31.6998000000001,50.0978989963061));
#35284=CARTESIAN_POINT('Ctrl Pts',(42.6082907905384,31.6998,50.1019668307642));
#35285=CARTESIAN_POINT('Ctrl Pts',(42.5897891748184,31.6998,50.1057747222131));
#35286=CARTESIAN_POINT('Ctrl Pts',(42.5127566104579,31.6998,50.1216291020441));
#35287=CARTESIAN_POINT('Ctrl Pts',(42.4351379902024,31.6998000000001,50.1330052928323));
#35288=CARTESIAN_POINT('Ctrl Pts',(42.3572965076711,31.6998,50.1397510062613));
#35289=CARTESIAN_POINT('Ctrl Pts',(42.33214112474,31.6998,50.1419309622299));
#35290=CARTESIAN_POINT('Ctrl Pts',(42.3069622193782,31.6998,50.1436270192556));
#35291=CARTESIAN_POINT('Ctrl Pts',(42.2817714200905,31.6998,50.1448330571849));
#35292=CARTESIAN_POINT('Ctrl Pts',(42.2057610810024,31.6998,50.1484721379029));
#35293=CARTESIAN_POINT('Ctrl Pts',(42.1296433545669,31.6998,50.1476538965692));
#35294=CARTESIAN_POINT('Ctrl Pts',(42.0536890631274,31.6998,50.1425994759693));
#35295=CARTESIAN_POINT('Ctrl Pts',(41.9777347716879,31.6998,50.1375450553693));
#35296=CARTESIAN_POINT('Ctrl Pts',(41.901943126711,31.6998,50.1282542163723));
#35297=CARTESIAN_POINT('Ctrl Pts',(41.8265789334743,31.6998,50.1148961512031));
#35298=CARTESIAN_POINT('Ctrl Pts',(41.8136579892345,31.6998,50.112605954655));
#35299=CARTESIAN_POINT('Ctrl Pts',(41.8007475854246,31.6998,50.1101956878563));
#35300=CARTESIAN_POINT('Ctrl Pts',(41.7878555222505,31.6998,50.1076673315445));
#35301=CARTESIAN_POINT('Ctrl Pts',(41.7108587708215,31.6998,50.0925669383931));
#35302=CARTESIAN_POINT('Ctrl Pts',(41.6347686710189,31.6998,50.07330942136));
#35303=CARTESIAN_POINT('Ctrl Pts',(41.559869491234,31.6998,50.0501532594334));
#35304=CARTESIAN_POINT('Ctrl Pts',(41.4830476814102,31.6998,50.0264026886945));
#35305=CARTESIAN_POINT('Ctrl Pts',(41.4074778770195,31.6998,49.9985506735256));
#35306=CARTESIAN_POINT('Ctrl Pts',(41.3334597411236,31.6998,49.9668200521561));
#35307=CARTESIAN_POINT('Ctrl Pts',(41.2594416052277,31.6998,49.9350894307866));
#35308=CARTESIAN_POINT('Ctrl Pts',(41.1869742146367,31.6998,49.8994798787782));
#35309=CARTESIAN_POINT('Ctrl Pts',(41.1163636595774,31.6998,49.8601622832682));
#35310=CARTESIAN_POINT('Ctrl Pts',(41.0932456719035,31.6998,49.8472896512998));
#35311=CARTESIAN_POINT('Ctrl Pts',(41.0703268321719,31.6998,49.8340191546822));
#35312=CARTESIAN_POINT('Ctrl Pts',(41.0476182929131,31.6998,49.8203556713237));
#35313=CARTESIAN_POINT('Ctrl Pts',(41.0335607423107,31.6998,49.8118973946143));
#35314=CARTESIAN_POINT('Ctrl Pts',(41.0195837865544,31.6998,49.8032885094608));
#35315=CARTESIAN_POINT('Ctrl Pts',(41.0056901258032,31.6998,49.7945300723272));
#35316=CARTESIAN_POINT('Ctrl Pts',(40.9940648543958,31.6998,49.7872016071657));
#35317=CARTESIAN_POINT('Ctrl Pts',(40.982497025284,31.6998,49.7797677651481));
#35318=CARTESIAN_POINT('Ctrl Pts',(40.9710026743328,31.6998,49.7722388696788));
#35319=CARTESIAN_POINT('Ctrl Pts',(40.901156575791,31.6998,49.7264890942377));
#35320=CARTESIAN_POINT('Ctrl Pts',(40.8338981111519,31.6998,49.6771563319653));
#35321=CARTESIAN_POINT('Ctrl Pts',(40.7695370495458,31.6998,49.6244758840085));
#35322=CARTESIAN_POINT('Ctrl Pts',(40.7050594972812,31.6998,49.5717000867843));
#35323=CARTESIAN_POINT('Ctrl Pts',(40.6434888697281,31.6998,49.51556410536));
#35324=CARTESIAN_POINT('Ctrl Pts',(40.5851503766946,31.6998,49.4562541551619));
#35325=CARTESIAN_POINT('Ctrl Pts',(40.5280447210914,31.6998,49.3981975716997));
#35326=CARTESIAN_POINT('Ctrl Pts',(40.4740352031396,31.6998,49.337099242441));
#35327=CARTESIAN_POINT('Ctrl Pts',(40.4234532661656,31.6998,49.2730923705311));
#35328=CARTESIAN_POINT('Ctrl Pts',(40.3963290195265,31.6998,49.2387690866844));
#35329=CARTESIAN_POINT('Ctrl Pts',(40.3701909267342,31.6998,49.203608761589));
#35330=CARTESIAN_POINT('Ctrl Pts',(40.3450946017473,31.6998,49.167627614067));
#35331=CARTESIAN_POINT('Ctrl Pts',(41.5114521803192,47.2275992105786,49.7083478852713));
#35332=CARTESIAN_POINT('Ctrl Pts',(40.9424693995619,47.18552396311,49.4124079226697));
#35333=CARTESIAN_POINT('Ctrl Pts',(40.1335936552416,47.1013734681727,48.2118988144355));
#35334=CARTESIAN_POINT('Ctrl Pts',(40.9966811811913,46.975147725767,46.2047778501544));
#35335=CARTESIAN_POINT('Ctrl Pts',(43.1502053828948,46.848921983361,45.8504054458902));
#35336=CARTESIAN_POINT('Ctrl Pts',(44.6139419964807,46.7226962409553,47.467111741601));
#35337=CARTESIAN_POINT('Ctrl Pts',(44.0457885266063,46.5964704985493,49.5741617337718));
#35338=CARTESIAN_POINT('Ctrl Pts',(41.966498311004,46.4702447561435,50.2355298325241));
#35339=CARTESIAN_POINT('Ctrl Pts',(40.2853083124169,46.3440190137377,48.8449325541533));
#35340=CARTESIAN_POINT('Ctrl Pts',(40.5453717036046,46.2177932713318,46.6785273809893));
#35341=CARTESIAN_POINT('Ctrl Pts',(42.5080504436644,46.091567528926,45.7253297325292));
#35342=CARTESIAN_POINT('Ctrl Pts',(44.3715194260783,45.9653417865201,46.8602812964785));
#35343=CARTESIAN_POINT('Ctrl Pts',(44.4251088775567,45.8391160441143,49.041532550479));
#35344=CARTESIAN_POINT('Ctrl Pts',(42.6196094511424,45.7128903017084,50.2666298767135));
#35345=CARTESIAN_POINT('Ctrl Pts',(40.6125070533099,45.5866645593025,49.4109270826402));
#35346=CARTESIAN_POINT('Ctrl Pts',(40.2463524779982,45.4604388168967,47.2599668519521));
#35347=CARTESIAN_POINT('Ctrl Pts',(41.8572835539691,45.3342130744908,45.7883708343257));
#35348=CARTESIAN_POINT('Ctrl Pts',(43.966437279631,45.2079873320851,46.3470874390647));
#35349=CARTESIAN_POINT('Ctrl Pts',(44.637575063142,45.081761589679,48.4232062102119));
#35350=CARTESIAN_POINT('Ctrl Pts',(43.2545807794454,44.9555358472734,50.1108143256454));
#35351=CARTESIAN_POINT('Ctrl Pts',(41.0870668303238,44.8293101048674,49.860659036887));
#35352=CARTESIAN_POINT('Ctrl Pts',(40.1248478607906,44.7030843624616,47.9023870427558));
#35353=CARTESIAN_POINT('Ctrl Pts',(41.251257290822,44.5768586200558,46.0337254241421));
#35354=CARTESIAN_POINT('Ctrl Pts',(43.4322320766004,44.4506328776498,45.9701373254779));
#35355=CARTESIAN_POINT('Ctrl Pts',(44.665600248225,44.324407135244,47.769997718258));
#35356=CARTESIAN_POINT('Ctrl Pts',(43.8191088268314,44.1981813928382,49.7810041182161));
#35357=CARTESIAN_POINT('Ctrl Pts',(41.6698513475981,44.0719556504323,50.1570184234761));
#35358=CARTESIAN_POINT('Ctrl Pts',(40.1908827592175,43.9457299080265,48.5528530996183));
#35359=CARTESIAN_POINT('Ctrl Pts',(40.7399214005723,43.8195041656206,46.4411592202193));
#35360=CARTESIAN_POINT('Ctrl Pts',(42.8129404531986,43.6932784232148,45.7605077103516));
#35361=CARTESIAN_POINT('Ctrl Pts',(44.5068731409494,43.5670526808089,47.1357482420377));
#35362=CARTESIAN_POINT('Ctrl Pts',(44.2666604230926,43.4408269384031,49.3043865983774));
#35363=CARTESIAN_POINT('Ctrl Pts',(42.3128216634364,43.3146011959972,50.2755758547758));
#35364=CARTESIAN_POINT('Ctrl Pts',(40.4390141006492,43.1883754535914,49.1577477427049));
#35365=CARTESIAN_POINT('Ctrl Pts',(40.3654249724418,43.0621497111855,46.9770874962022));
#35366=CARTESIAN_POINT('Ctrl Pts',(42.1596103511045,42.9359239687796,45.7354783397155));
#35367=CARTESIAN_POINT('Ctrl Pts',(44.1744775192528,42.8096982263738,46.5727386129868));
#35368=CARTESIAN_POINT('Ctrl Pts',(44.5603441204102,42.6834724839679,48.7202491337033));
#35369=CARTESIAN_POINT('Ctrl Pts',(42.9629780466766,42.557246741562,50.2065586899405));
#35370=CARTESIAN_POINT('Ctrl Pts',(40.848788543348,42.4310209991563,49.6672098098151));
#35371=CARTESIAN_POINT('Ctrl Pts',(40.1586375612129,42.3047952567503,47.5973339458232));
#35372=CARTESIAN_POINT('Ctrl Pts',(41.5260954492946,42.1785695143446,45.8971123735567));
#35373=CARTESIAN_POINT('Ctrl Pts',(43.6958125901134,42.0523437719386,46.1273774367225));
#35374=CARTESIAN_POINT('Ctrl Pts',(44.6759517164996,41.9261180295328,48.0767418878717));
#35375=CARTESIAN_POINT('Ctrl Pts',(43.5667284269667,41.799892287127,49.9556559796906));
#35376=CARTESIAN_POINT('Ctrl Pts',(41.3864285819795,41.6736665447211,50.0392445939032));
#35377=CARTESIAN_POINT('Ctrl Pts',(40.1366045512679,41.5474408023153,48.2507719598567));
#35378=CARTESIAN_POINT('Ctrl Pts',(40.964616068938,41.4212150599094,46.2320863981401));
#35379=CARTESIAN_POINT('Ctrl Pts',(43.1103344677488,41.2949893175036,45.8363756155191));
#35380=CARTESIAN_POINT('Ctrl Pts',(44.6039537341892,41.1687635750977,47.4269088460414));
#35381=CARTESIAN_POINT('Ctrl Pts',(44.0743059579869,41.0425378326919,49.543549510784));
#35382=CARTESIAN_POINT('Ctrl Pts',(42.0076168131093,40.916312090286,50.2431854510578));
#35383=CARTESIAN_POINT('Ctrl Pts',(40.3011421127583,40.7900863478802,48.88353896482));
#35384=CARTESIAN_POINT('Ctrl Pts',(40.5214546786603,40.6638606054743,46.7127886696953));
#35385=CARTESIAN_POINT('Ctrl Pts',(42.4663038252612,40.5376348630684,45.7237202860924));
#35386=CARTESIAN_POINT('Ctrl Pts',(44.3502849316801,40.4114091206626,46.8243154256119));
#35387=CARTESIAN_POINT('Ctrl Pts',(44.4438712739898,40.2851833782568,49.0042090163662));
#35388=CARTESIAN_POINT('Ctrl Pts',(42.6611489969678,40.1589576358509,50.2622216369255));
#35389=CARTESIAN_POINT('Ctrl Pts',(40.6386874955747,40.032731893445,49.4434762883218));
#35390=CARTESIAN_POINT('Ctrl Pts',(40.2331408534716,39.9065061510392,47.2995951368686));
#35391=CARTESIAN_POINT('Ctrl Pts',(41.8168077911319,39.7802804086334,45.79869757173));
#35392=CARTESIAN_POINT('Ctrl Pts',(43.9358551033548,39.6540546662275,46.3186331052709));
#35393=CARTESIAN_POINT('Ctrl Pts',(44.6449612880996,39.5278289238216,48.3820920676043));
#35394=CARTESIAN_POINT('Ctrl Pts',(43.2931547977007,39.4016031814158,50.0947840080867));
#35395=CARTESIAN_POINT('Ctrl Pts',(41.1214170001545,39.2753774390099,49.8844285727238));
#35396=CARTESIAN_POINT('Ctrl Pts',(40.1234401599009,39.1491516966041,47.9441356317494));
#35397=CARTESIAN_POINT('Ctrl Pts',(41.2153840033819,39.0229259541982,46.0551271317259));
#35398=CARTESIAN_POINT('Ctrl Pts',(43.3948254957311,38.8967002117924,45.9515450294831));
#35399=CARTESIAN_POINT('Ctrl Pts',(44.6610002495504,38.7704744693865,47.7284794580054));
#35400=CARTESIAN_POINT('Ctrl Pts',(43.8515382886068,38.6442487269807,49.7546743657729));
#35401=CARTESIAN_POINT('Ctrl Pts',(41.7095394713246,38.5180229845748,50.1700483385246));
#35402=CARTESIAN_POINT('Ctrl Pts',(40.2013951720587,38.391797242169,48.5932809989753));
#35403=CARTESIAN_POINT('Ctrl Pts',(40.7116075284533,38.2655714997631,46.4718716038183));
#35404=CARTESIAN_POINT('Ctrl Pts',(42.7717929127451,38.1393457573573,45.7533100874343));
#35405=CARTESIAN_POINT('Ctrl Pts',(44.4906660746539,38.0131200149514,47.0972481528774));
#35406=CARTESIAN_POINT('Ctrl Pts',(44.2902721937023,37.8868942725456,49.2699277801937));
#35407=CARTESIAN_POINT('Ctrl Pts',(42.3545762636138,37.7606685301397,50.2767920891826));
#35408=CARTESIAN_POINT('Ctrl Pts',(40.460580096709,37.6344427877339,49.193522505825));
#35409=CARTESIAN_POINT('Ctrl Pts',(40.3470044129129,37.508217045328,47.014578946545));
#35410=CARTESIAN_POINT('Ctrl Pts',(42.1181136231814,37.3819913029222,45.7402686877073));
#35411=CARTESIAN_POINT('Ctrl Pts',(44.147999325506,37.2557655605163,46.5404302376307));
#35412=CARTESIAN_POINT('Ctrl Pts',(44.5731918933992,37.1295398181104,48.6805016735148));
#35413=CARTESIAN_POINT('Ctrl Pts',(43.0033573121084,37.0033140757046,50.1958609899347));
#35414=CARTESIAN_POINT('Ctrl Pts',(40.8796304482396,36.8770883332987,49.6953825406888));
#35415=CARTESIAN_POINT('Ctrl Pts',(40.1516287118976,36.7508625908929,47.6385140610914));
#35416=CARTESIAN_POINT('Ctrl Pts',(41.487670088745,36.624636848487,45.9134958264548));
#35417=CARTESIAN_POINT('Ctrl Pts',(43.6612458533724,36.4984111060812,46.1039239386188));
#35418=CARTESIAN_POINT('Ctrl Pts',(44.6769764562741,36.3721853636753,48.0349821492397));
#35419=CARTESIAN_POINT('Ctrl Pts',(43.6024039147009,36.2459596212695,49.933926151409));
#35420=CARTESIAN_POINT('Ctrl Pts',(41.4240041126824,36.1197338788636,50.0574930282095));
#35421=CARTESIAN_POINT('Ctrl Pts',(40.1415851481607,35.9935081364578,48.2922462834413));
#35422=CARTESIAN_POINT('Ctrl Pts',(40.9324294592972,35.8672823940519,46.2587124759964));
#35423=CARTESIAN_POINT('Ctrl Pts',(43.0705285070869,35.7410566516461,45.823710254958));
#35424=CARTESIAN_POINT('Ctrl Pts',(44.5930709719577,35.6148309092402,47.386579063643));
#35425=CARTESIAN_POINT('Ctrl Pts',(44.1023369551445,35.4886051668344,49.5125787332619));
#35426=CARTESIAN_POINT('Ctrl Pts',(42.0488286371567,35.3623794244285,50.2500053793523));
#35427=CARTESIAN_POINT('Ctrl Pts',(40.3177016076886,35.2361536820227,48.9218887886614));
#35428=CARTESIAN_POINT('Ctrl Pts',(40.4981599463454,35.1099279396168,46.7474625980434));
#35429=CARTESIAN_POINT('Ctrl Pts',(42.4245398263078,34.983702197211,45.7228870624835));
#35430=CARTESIAN_POINT('Ctrl Pts',(44.3283917283527,34.8574764548051,46.7887399635747));
#35431=CARTESIAN_POINT('Ctrl Pts',(44.4619471989263,34.7312507123993,48.9665501954546));
#35432=CARTESIAN_POINT('Ctrl Pts',(42.7026000447332,34.6050249699934,50.2570508960347));
#35433=CARTESIAN_POINT('Ctrl Pts',(40.6654608961038,34.4787992275875,49.475540455032));
#35434=CARTESIAN_POINT('Ctrl Pts',(40.2206581746343,34.3525734851817,47.3394587614941));
#35435=CARTESIAN_POINT('Ctrl Pts',(41.7765283340811,34.2263477427758,45.8097651660685));
#35436=CARTESIAN_POINT('Ctrl Pts',(43.9047561161392,34.10012200037,46.2907444338171));
#35437=CARTESIAN_POINT('Ctrl Pts',(44.6515921288771,33.9738962579641,48.3408493965467));
#35438=CARTESIAN_POINT('Ctrl Pts',(43.3314283241735,33.8476705155583,50.0780488291867));
#35439=CARTESIAN_POINT('Ctrl Pts',(41.1561972997618,33.7214447731524,49.9075640298549));
#35440=CARTESIAN_POINT('Ctrl Pts',(40.12279865113,33.5952190307466,47.9859030514586));
#35441=CARTESIAN_POINT('Ctrl Pts',(41.1799089551562,33.4689932883407,46.0771831726539));
#35442=CARTESIAN_POINT('Ctrl Pts',(43.3570848922405,33.3427675459349,45.9336421471489));
#35443=CARTESIAN_POINT('Ctrl Pts',(44.6556380509762,33.216541803529,47.6870522535155));
#35444=CARTESIAN_POINT('Ctrl Pts',(43.8834821652962,33.0903160611232,49.7277548104157));
#35445=CARTESIAN_POINT('Ctrl Pts',(41.7494543021213,32.9640903187173,50.1823468710386));
#35446=CARTESIAN_POINT('Ctrl Pts',(40.2126585350139,32.8378645763115,48.6335116728557));
#35447=CARTESIAN_POINT('Ctrl Pts',(40.6838395690534,32.7116388339056,46.503093397757));
#35448=CARTESIAN_POINT('Ctrl Pts',(42.7305643873577,32.5854130914998,45.7468779126706));
#35449=CARTESIAN_POINT('Ctrl Pts',(44.4736678592443,32.4591873490939,47.0590329676311));
#35450=CARTESIAN_POINT('Ctrl Pts',(44.3134222176753,32.332961606688,49.2350791291602));
#35451=CARTESIAN_POINT('Ctrl Pts',(42.3959996514303,32.2067358642822,50.2771677709232));
#35452=CARTESIAN_POINT('Ctrl Pts',(40.4834883240295,32.0805101218763,49.2290434733774));
#35453=CARTESIAN_POINT('Ctrl Pts',(40.3278918291434,31.9542843794705,47.052110764494));
#35454=CARTESIAN_POINT('Ctrl Pts',(42.079842082062,31.8280415161295,45.7461934776559));
#35455=CARTESIAN_POINT('Ctrl Pts',(43.4357287145305,31.7438739002569,46.2544404205575));
#35456=CARTESIAN_POINT('Ctrl Pts',(43.8557111658903,31.701781531853,46.7394942770224));
#35457=CARTESIAN_POINT('Ctrl Pts',(41.4436260057576,47.1427351163746,49.8387524614932));
#35458=CARTESIAN_POINT('Ctrl Pts',(40.8312106437082,47.1006598689058,49.5202222959576));
#35459=CARTESIAN_POINT('Ctrl Pts',(39.9605903919818,47.0165093739687,48.2280738425644));
#35460=CARTESIAN_POINT('Ctrl Pts',(40.8895606131567,46.8902836315629,46.067741836768));
#35461=CARTESIAN_POINT('Ctrl Pts',(43.2074713624294,46.764057889157,45.6863188630025));
#35462=CARTESIAN_POINT('Ctrl Pts',(44.7829404600371,46.6378321467512,47.4264343900444));
#35463=CARTESIAN_POINT('Ctrl Pts',(44.1714177132687,46.5116064043452,49.6943233797499));
#35464=CARTESIAN_POINT('Ctrl Pts',(41.9334075075836,46.3853806619395,50.4061761762548));
#35465=CARTESIAN_POINT('Ctrl Pts',(40.1238859957233,46.2591549195336,48.909429412557));
#35466=CARTESIAN_POINT('Ctrl Pts',(40.4038009971191,46.1329291771276,46.5776544391508));
#35467=CARTESIAN_POINT('Ctrl Pts',(42.5162983376901,46.0067034347219,45.5516956531759));
#35468=CARTESIAN_POINT('Ctrl Pts',(44.5220128691805,45.8804776923159,46.7732823100154));
#35469=CARTESIAN_POINT('Ctrl Pts',(44.5796930036929,45.7542519499102,49.1210366210712));
#35470=CARTESIAN_POINT('Ctrl Pts',(42.6363730609772,45.6280262075043,50.4396502030025));
#35471=CARTESIAN_POINT('Ctrl Pts',(40.4760610388754,45.5018004650984,49.5186284178764));
#35472=CARTESIAN_POINT('Ctrl Pts',(40.0819565169301,45.3755747226925,47.2034773571056));
#35473=CARTESIAN_POINT('Ctrl Pts',(41.8158559801338,45.2493489802868,45.619548917785));
#35474=CARTESIAN_POINT('Ctrl Pts',(44.0860092891672,45.1231232378808,46.2209144482476));
#35475=CARTESIAN_POINT('Ctrl Pts',(44.8083775269665,44.996897495475,48.4555111212743));
#35476=CARTESIAN_POINT('Ctrl Pts',(43.31981412293,44.8706717530692,50.2719406688171));
#35477=CARTESIAN_POINT('Ctrl Pts',(40.9868457365551,44.7444460106634,50.0026900923241));
#35478=CARTESIAN_POINT('Ctrl Pts',(39.9511769983675,44.6182202682575,47.8949358810616));
#35479=CARTESIAN_POINT('Ctrl Pts',(41.1635694682946,44.4919945258517,45.8836323400513));
#35480=CARTESIAN_POINT('Ctrl Pts',(43.5110262072764,44.3657687834457,45.8151903242601));
#35481=CARTESIAN_POINT('Ctrl Pts',(44.8385419791249,44.23954304104,47.7524407848375));
#35482=CARTESIAN_POINT('Ctrl Pts',(43.9274347051677,44.1133172986341,49.9169548161318));
#35483=CARTESIAN_POINT('Ctrl Pts',(41.6141163732311,43.9870915562282,50.321671698047));
#35484=CARTESIAN_POINT('Ctrl Pts',(40.0222525872881,43.8608658138223,48.595054442091));
#35485=CARTESIAN_POINT('Ctrl Pts',(40.6132013992659,43.7346400714165,46.3221670798963));
#35486=CARTESIAN_POINT('Ctrl Pts',(42.8444617406766,43.6084143290108,45.5895588974655));
#35487=CARTESIAN_POINT('Ctrl Pts',(44.6676986387696,43.4821885866047,47.0697766766335));
#35488=CARTESIAN_POINT('Ctrl Pts',(44.4091495867591,43.355962844199,49.4039553004303));
#35489=CARTESIAN_POINT('Ctrl Pts',(42.306167015321,43.229737101793,50.4492790609911));
#35490=CARTESIAN_POINT('Ctrl Pts',(40.2893247209937,43.1035113593872,49.2461229530827));
#35491=CARTESIAN_POINT('Ctrl Pts',(40.2101182597121,42.9772856169814,46.899004763335));
#35492=CARTESIAN_POINT('Ctrl Pts',(42.1412605111437,42.8510598745756,45.5626189414625));
#35493=CARTESIAN_POINT('Ctrl Pts',(44.309930017487,42.7248341321696,46.4637904192753));
#35494=CARTESIAN_POINT('Ctrl Pts',(44.7252512578526,42.5986083897639,48.7752284408247));
#35495=CARTESIAN_POINT('Ctrl Pts',(43.0059522641835,42.472382647358,50.374993558126));
#35496=CARTESIAN_POINT('Ctrl Pts',(40.7303787777615,42.3461569049521,49.7944741630515));
#35497=CARTESIAN_POINT('Ctrl Pts',(39.9875459928562,42.2199311625463,47.5665969416062));
#35498=CARTESIAN_POINT('Ctrl Pts',(41.459387050159,42.0937054201404,45.7365911049481));
#35499=CARTESIAN_POINT('Ctrl Pts',(43.794726806084,41.9674796777346,45.9844331606221));
#35500=CARTESIAN_POINT('Ctrl Pts',(44.8496836136446,41.8412539353288,48.0825998828696));
#35501=CARTESIAN_POINT('Ctrl Pts',(43.6557891665248,41.7150281929229,50.1049385066667));
#35502=CARTESIAN_POINT('Ctrl Pts',(41.3090588890865,41.5888024505171,50.194907752077));
#35503=CARTESIAN_POINT('Ctrl Pts',(39.96383112095,41.4625767081111,48.2699143204002));
#35504=CARTESIAN_POINT('Ctrl Pts',(40.8550478510946,41.3363509657054,46.0971349482422));
#35505=CARTESIAN_POINT('Ctrl Pts',(43.1645569513782,41.2101252232995,45.6712180832658));
#35506=CARTESIAN_POINT('Ctrl Pts',(44.7721897563704,41.0838994808936,47.3831626572747));
#35507=CARTESIAN_POINT('Ctrl Pts',(44.2021119867235,40.9576737384876,49.6613744114186));
#35508=CARTESIAN_POINT('Ctrl Pts',(41.9776647385675,40.831447996082,50.4144161767515));
#35509=CARTESIAN_POINT('Ctrl Pts',(40.1409284491974,40.705222253676,48.9509827947776));
#35510=CARTESIAN_POINT('Ctrl Pts',(40.3780582963104,40.5789965112702,46.6145310200189));
#35511=CARTESIAN_POINT('Ctrl Pts',(42.4713650439449,40.4527707688644,45.5499633516799));
#35512=CARTESIAN_POINT('Ctrl Pts',(44.4991574664958,40.3265450264584,46.7345710298625));
#35513=CARTESIAN_POINT('Ctrl Pts',(44.5998876039393,40.2003192840526,49.0808640421642));
#35514=CARTESIAN_POINT('Ctrl Pts',(42.681083475521,40.0740935416469,50.4349054658031));
#35515=CARTESIAN_POINT('Ctrl Pts',(40.5042399321047,39.947867799241,49.5536622260268));
#35516=CARTESIAN_POINT('Ctrl Pts',(40.0677363997466,39.821642056835,47.2461306170551));
#35517=CARTESIAN_POINT('Ctrl Pts',(41.7722905511079,39.6954163144293,45.6306639336346));
#35518=CARTESIAN_POINT('Ctrl Pts',(44.053092661125,39.5691905720234,46.1902880888541));
#35519=CARTESIAN_POINT('Ctrl Pts',(44.816327570069,39.4429648296175,48.411258582565));
#35520=CARTESIAN_POINT('Ctrl Pts',(43.3613326401056,39.3167390872117,50.2546866972324));
#35521=CARTESIAN_POINT('Ctrl Pts',(41.0238179831763,39.1905133448058,50.0282740456309));
#35522=CARTESIAN_POINT('Ctrl Pts',(39.9496618424098,39.0642876024,47.9398712958198));
#35523=CARTESIAN_POINT('Ctrl Pts',(41.1249578388071,38.9380618599941,45.9066677199284));
#35524=CARTESIAN_POINT('Ctrl Pts',(43.4707642423434,38.8118361175882,45.7951788088538));
#35525=CARTESIAN_POINT('Ctrl Pts',(44.8335908453665,38.6856103751823,47.7077532806737));
#35526=CARTESIAN_POINT('Ctrl Pts',(43.9623396289119,38.5593846327765,49.8886152153205));
#35527=CARTESIAN_POINT('Ctrl Pts',(41.6568340397108,38.4331588903706,50.3356962351891));
#35528=CARTESIAN_POINT('Ctrl Pts',(40.0335674518741,38.3069331479648,48.6385683540385));
#35529=CARTESIAN_POINT('Ctrl Pts',(40.5827262235116,38.180707405559,46.3552238544726));
#35530=CARTESIAN_POINT('Ctrl Pts',(42.8001732547391,38.0544816631531,45.5818118531015));
#35531=CARTESIAN_POINT('Ctrl Pts',(44.6502544265565,37.9282559207474,47.0283377318369));
#35532=CARTESIAN_POINT('Ctrl Pts',(44.4345637320296,37.8020301783415,49.3668661119213));
#35533=CARTESIAN_POINT('Ctrl Pts',(42.351108900119,37.6758044359356,50.450588135114));
#35534=CARTESIAN_POINT('Ctrl Pts',(40.3125369301003,37.5495786935296,49.2846285375211));
#35535=CARTESIAN_POINT('Ctrl Pts',(40.1902915900575,37.4233529511239,46.9393580761451));
#35536=CARTESIAN_POINT('Ctrl Pts',(42.0965961829524,37.2971272087181,45.5677749546126));
#35537=CARTESIAN_POINT('Ctrl Pts',(44.281430644293,37.1709014663122,46.4290158249288));
#35538=CARTESIAN_POINT('Ctrl Pts',(44.739079749351,37.0446757239063,48.7324469085092));
#35539=CARTESIAN_POINT('Ctrl Pts',(43.0494138297966,36.9184499815005,50.3634792627137));
#35540=CARTESIAN_POINT('Ctrl Pts',(40.7635749604744,36.7922242390946,49.8247974237219));
#35541=CARTESIAN_POINT('Ctrl Pts',(39.9800021318887,36.6659984966887,47.6109204889157));
#35542=CARTESIAN_POINT('Ctrl Pts',(41.4180285382873,36.5397727542828,45.7542251680121));
#35543=CARTESIAN_POINT('Ctrl Pts',(43.7575214611913,36.413547011877,45.9591893693892));
#35544=CARTESIAN_POINT('Ctrl Pts',(44.8507865756343,36.2873212694711,48.0376524673795));
#35545=CARTESIAN_POINT('Ctrl Pts',(43.6941878975161,36.1610955270653,50.0815499594128));
#35546=CARTESIAN_POINT('Ctrl Pts',(41.3495027004248,36.0348697846594,50.2145491575474));
#35547=CARTESIAN_POINT('Ctrl Pts',(39.9691919054106,35.9086440422536,48.314554534046));
#35548=CARTESIAN_POINT('Ctrl Pts',(40.8204043172953,35.7824182998477,46.1257934940924));
#35549=CARTESIAN_POINT('Ctrl Pts',(43.12171245303,35.6561925574419,45.6575859284171));
#35550=CARTESIAN_POINT('Ctrl Pts',(44.7604762722412,35.5299668150361,47.3397543519194));
#35551=CARTESIAN_POINT('Ctrl Pts',(44.2322826946139,35.4037410726303,49.6280395187459));
#35552=CARTESIAN_POINT('Ctrl Pts',(42.0220224151058,35.2775153302245,50.421756695651));
#35553=CARTESIAN_POINT('Ctrl Pts',(40.1587519922397,35.1512895878186,48.9922600039424));
#35554=CARTESIAN_POINT('Ctrl Pts',(40.3529853900521,35.0250638454127,46.6518517388546));
#35555=CARTESIAN_POINT('Ctrl Pts',(42.4264130429271,34.8988381030069,45.5490665250003));
#35556=CARTESIAN_POINT('Ctrl Pts',(44.4755930731687,34.772612360601,46.6962799599032));
#35557=CARTESIAN_POINT('Ctrl Pts',(44.6193433317553,34.6463866181951,49.0403305827646));
#35558=CARTESIAN_POINT('Ctrl Pts',(42.7256986366174,34.5201608757894,50.4293400229428));
#35559=CARTESIAN_POINT('Ctrl Pts',(40.5330570463177,34.3939351333834,49.5881739703691));
#35560=CARTESIAN_POINT('Ctrl Pts',(40.0543008714003,34.2677093909775,47.289037181073));
#35561=CARTESIAN_POINT('Ctrl Pts',(41.728936412622,34.1414836485718,45.6425763587958));
#35562=CARTESIAN_POINT('Ctrl Pts',(44.019619772034,34.0152579061658,46.1602705709202));
#35563=CARTESIAN_POINT('Ctrl Pts',(44.8234645676949,33.8890321637599,48.3668677043488));
#35564=CARTESIAN_POINT('Ctrl Pts',(43.4025277278384,33.7628064213541,50.2366740596067));
#35565=CARTESIAN_POINT('Ctrl Pts',(41.0612531929868,33.6365806789483,50.0531755186354));
#35566=CARTESIAN_POINT('Ctrl Pts',(39.9489713648778,33.5103549365424,47.9848269787123));
#35567=CARTESIAN_POINT('Ctrl Pts',(41.0867748476205,33.3841291941365,45.9304073808587));
#35568=CARTESIAN_POINT('Ctrl Pts',(43.4301427575952,33.2579034517307,45.7759093326285));
#35569=CARTESIAN_POINT('Ctrl Pts',(44.8278193301428,33.1316777093248,47.663163782899));
#35570=CARTESIAN_POINT('Ctrl Pts',(43.9967219010468,33.0054519669191,49.8596407897353));
#35571=CARTESIAN_POINT('Ctrl Pts',(41.6997957186581,32.8792262245131,50.3489335606354));
#35572=CARTESIAN_POINT('Ctrl Pts',(40.0456905894021,32.7530004821074,48.6818699855523));
#35573=CARTESIAN_POINT('Ctrl Pts',(40.5528386320335,32.6267747397014,46.3888289245825));
#35574=CARTESIAN_POINT('Ctrl Pts',(42.7557976019851,32.5005489972957,45.5748886864084));
#35575=CARTESIAN_POINT('Ctrl Pts',(44.6319586738618,32.3743232548897,46.9872054387344));
#35576=CARTESIAN_POINT('Ctrl Pts',(44.4594808838175,32.248097512484,49.3293573331649));
#35577=CARTESIAN_POINT('Ctrl Pts',(42.3956942898794,32.1218717700782,50.4509924940452));
#35578=CARTESIAN_POINT('Ctrl Pts',(40.3371938279938,31.9956460276723,49.322860953228));
#35579=CARTESIAN_POINT('Ctrl Pts',(40.1697200713673,31.8694202852663,46.9797548379716));
#35580=CARTESIAN_POINT('Ctrl Pts',(42.0554032321223,31.7431774219253,45.574152005912));
#35581=CARTESIAN_POINT('Ctrl Pts',(43.5147897566423,31.6590098060527,46.121195336702));
#35582=CARTESIAN_POINT('Ctrl Pts',(43.9668310375078,31.6169174376488,46.6432751661215));
#35583=CARTESIAN_POINT('Ctrl Pts',(41.375799831196,47.0578710221704,49.9691570377152));
#35584=CARTESIAN_POINT('Ctrl Pts',(40.7199518878545,47.0157957747018,49.6280366692455));
#35585=CARTESIAN_POINT('Ctrl Pts',(39.7875871287221,46.9316452797646,48.2442488706934));
#35586=CARTESIAN_POINT('Ctrl Pts',(40.7824400451221,46.8054195373585,45.9307058233814));
#35587=CARTESIAN_POINT('Ctrl Pts',(43.2647373419639,46.6791937949528,45.5222322801147));
#35588=CARTESIAN_POINT('Ctrl Pts',(44.9519389235938,46.5529680525469,47.3857570384877));
#35589=CARTESIAN_POINT('Ctrl Pts',(44.2970468999311,46.4267423101412,49.8144850257279));
#35590=CARTESIAN_POINT('Ctrl Pts',(41.9003167041634,46.3005165677351,50.5768225199857));
#35591=CARTESIAN_POINT('Ctrl Pts',(39.9624636790296,46.1742908253294,48.9739262709606));
#35592=CARTESIAN_POINT('Ctrl Pts',(40.2622302906338,46.0480650829236,46.4767814973122));
#35593=CARTESIAN_POINT('Ctrl Pts',(42.5245462317156,45.9218393405177,45.3780615738228));
#35594=CARTESIAN_POINT('Ctrl Pts',(44.6725063122828,45.7956135981119,46.6862833235523));
#35595=CARTESIAN_POINT('Ctrl Pts',(44.7342771298289,45.669387855706,49.2005406916632));
#35596=CARTESIAN_POINT('Ctrl Pts',(42.6531366708118,45.5431621133002,50.6126705292915));
#35597=CARTESIAN_POINT('Ctrl Pts',(40.339615024441,45.4169363708943,49.6263297531126));
#35598=CARTESIAN_POINT('Ctrl Pts',(39.917560555862,45.2907106284885,47.1469878622588));
#35599=CARTESIAN_POINT('Ctrl Pts',(41.7744284062985,45.1644848860825,45.4507270012443));
#35600=CARTESIAN_POINT('Ctrl Pts',(44.2055812987032,45.0382591436767,46.0947414574306));
#35601=CARTESIAN_POINT('Ctrl Pts',(44.979179990791,44.9120334012709,48.4878160323366));
#35602=CARTESIAN_POINT('Ctrl Pts',(43.3850474664145,44.7858076588651,50.4330670119889));
#35603=CARTESIAN_POINT('Ctrl Pts',(40.8866246427863,44.6595819164592,50.1447211477612));
#35604=CARTESIAN_POINT('Ctrl Pts',(39.7775061359443,44.5333561740533,47.8874847193674));
#35605=CARTESIAN_POINT('Ctrl Pts',(41.0758816457674,44.4071304316475,45.7335392559602));
#35606=CARTESIAN_POINT('Ctrl Pts',(43.5898203379522,44.2809046892416,45.6602433230422));
#35607=CARTESIAN_POINT('Ctrl Pts',(45.0114837100247,44.1546789468357,47.7348838514171));
#35608=CARTESIAN_POINT('Ctrl Pts',(44.035760583504,44.02845320443,50.0529055140476));
#35609=CARTESIAN_POINT('Ctrl Pts',(41.5583813988641,43.9022274620241,50.486324972618));
#35610=CARTESIAN_POINT('Ctrl Pts',(39.8536224153584,43.7760017196182,48.6372557845636));
#35611=CARTESIAN_POINT('Ctrl Pts',(40.4864813979593,43.6497759772124,46.2031749395733));
#35612=CARTESIAN_POINT('Ctrl Pts',(42.8759830281547,43.5235502348065,45.4186100845792));
#35613=CARTESIAN_POINT('Ctrl Pts',(44.8285241365898,43.3973244924007,47.0038051112294));
#35614=CARTESIAN_POINT('Ctrl Pts',(44.5516387504256,43.2710987499948,49.503524002483));
#35615=CARTESIAN_POINT('Ctrl Pts',(42.2995123672055,43.144873007589,50.6229822672065));
#35616=CARTESIAN_POINT('Ctrl Pts',(40.1396353413383,43.0186472651831,49.3344981634606));
#35617=CARTESIAN_POINT('Ctrl Pts',(40.0548115469822,42.8924215227773,46.8209220304679));
#35618=CARTESIAN_POINT('Ctrl Pts',(42.1229106711827,42.7661957803713,45.3897595432095));
#35619=CARTESIAN_POINT('Ctrl Pts',(44.4453825157214,42.6399700379655,46.3548422255637));
#35620=CARTESIAN_POINT('Ctrl Pts',(44.8901583952948,42.5137442955597,48.8302077479463));
#35621=CARTESIAN_POINT('Ctrl Pts',(43.0489264816905,42.3875185531538,50.5434284263114));
#35622=CARTESIAN_POINT('Ctrl Pts',(40.6119690121749,42.261292810748,49.921738516288));
#35623=CARTESIAN_POINT('Ctrl Pts',(39.8164544244997,42.1350670683421,47.5358599373892));
#35624=CARTESIAN_POINT('Ctrl Pts',(41.3926786510233,42.0088413259363,45.5760698363395));
#35625=CARTESIAN_POINT('Ctrl Pts',(43.8936410220548,41.8826155835305,45.8414888845218));
#35626=CARTESIAN_POINT('Ctrl Pts',(45.0234155107894,41.7563898411245,48.0884578778673));
#35627=CARTESIAN_POINT('Ctrl Pts',(43.7448499060829,41.6301640987188,50.2542210336426));
#35628=CARTESIAN_POINT('Ctrl Pts',(41.2316891961937,41.5039383563129,50.3505709102508));
#35629=CARTESIAN_POINT('Ctrl Pts',(39.7910576906322,41.377712613907,48.2890566809437));
#35630=CARTESIAN_POINT('Ctrl Pts',(40.7454796332511,41.2514868715012,45.9621834983442));
#35631=CARTESIAN_POINT('Ctrl Pts',(43.2187794350078,41.1252611290953,45.5060605510125));
#35632=CARTESIAN_POINT('Ctrl Pts',(44.9404257785515,40.9990353866895,47.3394164685078));
#35633=CARTESIAN_POINT('Ctrl Pts',(44.3299180154603,40.8728096442837,49.7791993120531));
#35634=CARTESIAN_POINT('Ctrl Pts',(41.9477126640256,40.7465839018778,50.5856469024452));
#35635=CARTESIAN_POINT('Ctrl Pts',(39.9807147856365,40.6203581594719,49.0184266247355));
#35636=CARTESIAN_POINT('Ctrl Pts',(40.2346619139606,40.4941324170661,46.5162733703425));
#35637=CARTESIAN_POINT('Ctrl Pts',(42.4764262626284,40.3679066746601,45.3762064172675));
#35638=CARTESIAN_POINT('Ctrl Pts',(44.6480300013119,40.2416809322544,46.6448266341129));
#35639=CARTESIAN_POINT('Ctrl Pts',(44.7559039338887,40.1154551898485,49.1575190679622));
#35640=CARTESIAN_POINT('Ctrl Pts',(42.7010179540743,39.9892294474426,50.6075892946806));
#35641=CARTESIAN_POINT('Ctrl Pts',(40.3697923686348,39.8630037050366,49.6638481637318));
#35642=CARTESIAN_POINT('Ctrl Pts',(39.9023319460215,39.736777962631,47.1926660972417));
#35643=CARTESIAN_POINT('Ctrl Pts',(41.7277733110837,39.610552220225,45.462630295539));
#35644=CARTESIAN_POINT('Ctrl Pts',(44.1703302188954,39.4843264778193,46.0619430724373));
#35645=CARTESIAN_POINT('Ctrl Pts',(44.9876938520384,39.3581007354134,48.4404250975257));
#35646=CARTESIAN_POINT('Ctrl Pts',(43.4295104825105,39.2318749930075,50.4145893863779));
#35647=CARTESIAN_POINT('Ctrl Pts',(40.9262189661981,39.1056492506017,50.1721195185379));
#35648=CARTESIAN_POINT('Ctrl Pts',(39.7758835249186,38.9794235081958,47.9356069598901));
#35649=CARTESIAN_POINT('Ctrl Pts',(41.0345316742323,38.85319776579,45.7582083081311));
#35650=CARTESIAN_POINT('Ctrl Pts',(43.5467029889559,38.7269720233841,45.6388125882245));
#35651=CARTESIAN_POINT('Ctrl Pts',(45.0061814411827,38.6007462809783,47.687027103342));
#35652=CARTESIAN_POINT('Ctrl Pts',(44.0731409692172,38.4745205385724,50.0225560648681));
#35653=CARTESIAN_POINT('Ctrl Pts',(41.6041286080969,38.3482947961665,50.5013441318535));
#35654=CARTESIAN_POINT('Ctrl Pts',(39.8657397316897,38.2220690537607,48.6838557091019));
#35655=CARTESIAN_POINT('Ctrl Pts',(40.4538449185697,38.0958433113549,46.2385761051266));
#35656=CARTESIAN_POINT('Ctrl Pts',(42.8285535967332,37.969617568949,45.4103136187687));
#35657=CARTESIAN_POINT('Ctrl Pts',(44.8098427784591,37.8433918265431,46.9594273107965));
#35658=CARTESIAN_POINT('Ctrl Pts',(44.5788552703569,37.7171660841372,49.4638044436488));
#35659=CARTESIAN_POINT('Ctrl Pts',(42.347641536624,37.5909403417315,50.6243841810452));
#35660=CARTESIAN_POINT('Ctrl Pts',(40.1644937634915,37.4647145993256,49.3757345692172));
#35661=CARTESIAN_POINT('Ctrl Pts',(40.0335787672024,37.3384888569198,46.8641372057452));
#35662=CARTESIAN_POINT('Ctrl Pts',(42.0750787427234,37.2122631145138,45.3952812215179));
#35663=CARTESIAN_POINT('Ctrl Pts',(44.4148619630801,37.0860373721079,46.3176014122269));
#35664=CARTESIAN_POINT('Ctrl Pts',(44.9049676053029,36.9598116297022,48.7843921435038));
#35665=CARTESIAN_POINT('Ctrl Pts',(43.0954703474852,36.8335858872964,50.5310975354926));
#35666=CARTESIAN_POINT('Ctrl Pts',(40.647519472709,36.7073601448905,49.9542123067552));
#35667=CARTESIAN_POINT('Ctrl Pts',(39.8083755518798,36.5811344024847,47.5833269167399));
#35668=CARTESIAN_POINT('Ctrl Pts',(41.3483869878293,36.4549086600788,45.5949545095694));
#35669=CARTESIAN_POINT('Ctrl Pts',(43.8537970690102,36.3286829176729,45.8144548001597));
#35670=CARTESIAN_POINT('Ctrl Pts',(45.0245966949945,36.2024571752671,48.0403227855192));
#35671=CARTESIAN_POINT('Ctrl Pts',(43.7859718803313,36.0762314328613,50.2291737674166));
#35672=CARTESIAN_POINT('Ctrl Pts',(41.2750012881672,35.9500056904552,50.3716052868853));
#35673=CARTESIAN_POINT('Ctrl Pts',(39.7967986626603,35.8237799480496,48.3368627846507));
#35674=CARTESIAN_POINT('Ctrl Pts',(40.7083791752934,35.6975542056437,45.9928745121884));
#35675=CARTESIAN_POINT('Ctrl Pts',(43.1728963989727,35.5713284632378,45.4914616018761));
#35676=CARTESIAN_POINT('Ctrl Pts',(44.927881572525,35.4451027208319,47.2929296401959));
#35677=CARTESIAN_POINT('Ctrl Pts',(44.3622284340833,35.3188769784261,49.7435003042299));
#35678=CARTESIAN_POINT('Ctrl Pts',(41.9952161930549,35.1926512360203,50.5935080119497));
#35679=CARTESIAN_POINT('Ctrl Pts',(39.9998023767907,35.0664254936144,49.0626312192234));
#35680=CARTESIAN_POINT('Ctrl Pts',(40.2078108337589,34.9401997512085,46.5562408796657));
#35681=CARTESIAN_POINT('Ctrl Pts',(42.4282862595464,34.8139740088026,45.3752459875171));
#35682=CARTESIAN_POINT('Ctrl Pts',(44.6227944179848,34.6877482663969,46.6038199562315));
#35683=CARTESIAN_POINT('Ctrl Pts',(44.776739464584,34.561522523991,49.1141109700746));
#35684=CARTESIAN_POINT('Ctrl Pts',(42.7487972285017,34.435296781585,50.601629149851));
#35685=CARTESIAN_POINT('Ctrl Pts',(40.4006531965316,34.3090710391792,49.7008074857061));
#35686=CARTESIAN_POINT('Ctrl Pts',(39.8879435681661,34.1828452967733,47.2386156006519));
#35687=CARTESIAN_POINT('Ctrl Pts',(41.6813444911631,34.0566195543676,45.4753875515231));
#35688=CARTESIAN_POINT('Ctrl Pts',(44.1344834279288,33.9303938119617,46.0297967080234));
#35689=CARTESIAN_POINT('Ctrl Pts',(44.9953370065128,33.8041680695559,48.3928860121509));
#35690=CARTESIAN_POINT('Ctrl Pts',(43.4736271315033,33.6779423271499,50.3952992900265));
#35691=CARTESIAN_POINT('Ctrl Pts',(40.9663090862117,33.5517165847442,50.1987870074159));
#35692=CARTESIAN_POINT('Ctrl Pts',(39.7751440786257,33.4254908423384,47.9837509059659));
#35693=CARTESIAN_POINT('Ctrl Pts',(40.9936407400849,33.2992650999325,45.7836315890635));
#35694=CARTESIAN_POINT('Ctrl Pts',(43.5032006229498,33.1730393575266,45.6181765181081));
#35695=CARTESIAN_POINT('Ctrl Pts',(45.0000006093094,33.0468136151207,47.6392753122826));
#35696=CARTESIAN_POINT('Ctrl Pts',(44.1099616367975,32.9205878727149,49.9915267690549));
#35697=CARTESIAN_POINT('Ctrl Pts',(41.650137135195,32.7943621303091,50.5155202502322));
#35698=CARTESIAN_POINT('Ctrl Pts',(39.8787226437902,32.6681363879032,48.7302282982488));
#35699=CARTESIAN_POINT('Ctrl Pts',(40.4218376950136,32.5419106454973,46.274564451408));
#35700=CARTESIAN_POINT('Ctrl Pts',(42.7810308166128,32.4156849030914,45.4028994601463));
#35701=CARTESIAN_POINT('Ctrl Pts',(44.7902494884793,32.2894591606857,46.9153779098378));
#35702=CARTESIAN_POINT('Ctrl Pts',(44.6055395499598,32.1632334182798,49.4236355371696));
#35703=CARTESIAN_POINT('Ctrl Pts',(42.3953889283282,32.0370076758738,50.6248172171673));
#35704=CARTESIAN_POINT('Ctrl Pts',(40.1908993319584,31.9107819334682,49.4166784330786));
#35705=CARTESIAN_POINT('Ctrl Pts',(40.0115483135911,31.7845561910622,46.9073989114492));
#35706=CARTESIAN_POINT('Ctrl Pts',(42.0309643821828,31.6583133277211,45.4021105341682));
#35707=CARTESIAN_POINT('Ctrl Pts',(43.5938507987542,31.5741457118486,45.9879502528466));
#35708=CARTESIAN_POINT('Ctrl Pts',(44.0779509091253,31.5320533434447,46.5470560552206));
#35709=CARTESIAN_POINT('Ctrl Pts',(41.3079736566343,46.9730069279662,50.0995616139371));
#35710=CARTESIAN_POINT('Ctrl Pts',(40.6086931320009,46.9309316804976,49.7358510425334));
#35711=CARTESIAN_POINT('Ctrl Pts',(39.6145838654623,46.8467811855604,48.2604238988224));
#35712=CARTESIAN_POINT('Ctrl Pts',(40.6753194770875,46.7205554431545,45.7936698099951));
#35713=CARTESIAN_POINT('Ctrl Pts',(43.3220033214984,46.5943297007486,45.358145697227));
#35714=CARTESIAN_POINT('Ctrl Pts',(45.1209373871503,46.4681039583428,47.3450796869312));
#35715=CARTESIAN_POINT('Ctrl Pts',(44.4226760865935,46.341878215937,49.9346466717058));
#35716=CARTESIAN_POINT('Ctrl Pts',(41.8672259007431,46.2156524735311,50.7474688637164));
#35717=CARTESIAN_POINT('Ctrl Pts',(39.8010413623359,46.0894267311253,49.0384231293642));
#35718=CARTESIAN_POINT('Ctrl Pts',(40.1206595841484,45.9632009887194,46.3759085554738));
#35719=CARTESIAN_POINT('Ctrl Pts',(42.5327941257413,45.8369752463135,45.2044274944695));
#35720=CARTESIAN_POINT('Ctrl Pts',(44.8229997553851,45.7107495039077,46.5992843370893));
#35721=CARTESIAN_POINT('Ctrl Pts',(44.888861255965,45.5845237615018,49.2800447622554));
#35722=CARTESIAN_POINT('Ctrl Pts',(42.6699002806466,45.458298019096,50.7856908555805));
#35723=CARTESIAN_POINT('Ctrl Pts',(40.2031690100066,45.3320722766902,49.7340310883488));
#35724=CARTESIAN_POINT('Ctrl Pts',(39.7531645947938,45.2058465342842,47.0904983674123));
#35725=CARTESIAN_POINT('Ctrl Pts',(41.7330008324632,45.0796207918785,45.2819050847036));
#35726=CARTESIAN_POINT('Ctrl Pts',(44.3251533082391,44.9533950494725,45.9685684666135));
#35727=CARTESIAN_POINT('Ctrl Pts',(45.1499824546155,44.8271693070668,48.5201209433989));
#35728=CARTESIAN_POINT('Ctrl Pts',(43.4502808098991,44.7009435646609,50.5941933551607));
#35729=CARTESIAN_POINT('Ctrl Pts',(40.7864035490177,44.5747178222551,50.2867522031983));
#35730=CARTESIAN_POINT('Ctrl Pts',(39.6038352735211,44.4484920798491,47.8800335576731));
#35731=CARTESIAN_POINT('Ctrl Pts',(40.9881938232402,44.3222663374434,45.5834461718693));
#35732=CARTESIAN_POINT('Ctrl Pts',(43.6686144686279,44.1960405950374,45.5052963218242));
#35733=CARTESIAN_POINT('Ctrl Pts',(45.1844254409248,44.0698148526316,47.7173269179967));
#35734=CARTESIAN_POINT('Ctrl Pts',(44.14408646184,43.9435891102256,50.1888562119632));
#35735=CARTESIAN_POINT('Ctrl Pts',(41.5026464244972,43.8173633678199,50.650978247189));
#35736=CARTESIAN_POINT('Ctrl Pts',(39.6849922434289,43.6911376254141,48.6794571270361));
#35737=CARTESIAN_POINT('Ctrl Pts',(40.359761396653,43.5649118830082,46.0841827992503));
#35738=CARTESIAN_POINT('Ctrl Pts',(42.9075043156328,43.4386861406023,45.2476612716929));
#35739=CARTESIAN_POINT('Ctrl Pts',(44.9893496344101,43.3124603981964,46.9378335458254));
#35740=CARTESIAN_POINT('Ctrl Pts',(44.694127914092,43.1862346557907,49.6030927045356));
#35741=CARTESIAN_POINT('Ctrl Pts',(42.29285771909,43.0600089133848,50.7966854734219));
#35742=CARTESIAN_POINT('Ctrl Pts',(39.9899459616828,42.9337831709789,49.4228733738384));
#35743=CARTESIAN_POINT('Ctrl Pts',(39.8995048342524,42.8075574285731,46.7428392976006));
#35744=CARTESIAN_POINT('Ctrl Pts',(42.1045608312217,42.6813316861672,45.2169001449566));
#35745=CARTESIAN_POINT('Ctrl Pts',(44.5808350139558,42.5551059437613,46.245894031852));
#35746=CARTESIAN_POINT('Ctrl Pts',(45.0550655327371,42.4288802013556,48.8851870550678));
#35747=CARTESIAN_POINT('Ctrl Pts',(43.0919006991974,42.3026544589497,50.7118632944967));
#35748=CARTESIAN_POINT('Ctrl Pts',(40.4935592465884,42.1764287165438,50.0490028695245));
#35749=CARTESIAN_POINT('Ctrl Pts',(39.6453628561431,42.050202974138,47.505122933172));
#35750=CARTESIAN_POINT('Ctrl Pts',(41.3259702518877,41.9239772317321,45.4155485677308));
#35751=CARTESIAN_POINT('Ctrl Pts',(43.9925552380253,41.7977514893263,45.6985446084214));
#35752=CARTESIAN_POINT('Ctrl Pts',(45.1971474079345,41.6715257469204,48.094315872865));
#35753=CARTESIAN_POINT('Ctrl Pts',(43.8339106456409,41.5453000045146,50.4035035606187));
#35754=CARTESIAN_POINT('Ctrl Pts',(41.154319503301,41.4190742621087,50.5062340684245));
#35755=CARTESIAN_POINT('Ctrl Pts',(39.6182842603143,41.2928485197029,48.3081990414871));
#35756=CARTESIAN_POINT('Ctrl Pts',(40.6359114154075,41.166622777297,45.8272320484462));
#35757=CARTESIAN_POINT('Ctrl Pts',(43.2730019186371,41.0403970348911,45.3409030187592));
#35758=CARTESIAN_POINT('Ctrl Pts',(45.1086618007328,40.9141712924853,47.2956702797409));
#35759=CARTESIAN_POINT('Ctrl Pts',(44.4577240441967,40.7879455500795,49.8970242126877));
#35760=CARTESIAN_POINT('Ctrl Pts',(41.9177605894838,40.6617198076736,50.756877628139));
#35761=CARTESIAN_POINT('Ctrl Pts',(39.8205011220756,40.5354940652678,49.0858704546932));
#35762=CARTESIAN_POINT('Ctrl Pts',(40.0912655316106,40.4092683228619,46.4180157206662));
#35763=CARTESIAN_POINT('Ctrl Pts',(42.4814874813122,40.283042580456,45.202449482855));
#35764=CARTESIAN_POINT('Ctrl Pts',(44.7969025361278,40.1568168380502,46.5550822383634));
#35765=CARTESIAN_POINT('Ctrl Pts',(44.9119202638379,40.0305910956443,49.2341740937601));
#35766=CARTESIAN_POINT('Ctrl Pts',(42.7209524326276,39.9043653532385,50.780273123558));
#35767=CARTESIAN_POINT('Ctrl Pts',(40.2353448051647,39.7781396108327,49.7740341014369));
#35768=CARTESIAN_POINT('Ctrl Pts',(39.7369274922965,39.6519138684268,47.1392015774281));
#35769=CARTESIAN_POINT('Ctrl Pts',(41.6832560710595,39.525688126021,45.2945966574436));
#35770=CARTESIAN_POINT('Ctrl Pts',(44.2875677766657,39.3994623836151,45.9335980560206));
#35771=CARTESIAN_POINT('Ctrl Pts',(45.1590601340077,39.2732366412092,48.4695916124862));
#35772=CARTESIAN_POINT('Ctrl Pts',(43.4976883249155,39.1470108988034,50.5744920755234));
#35773=CARTESIAN_POINT('Ctrl Pts',(40.8286199492197,39.0207851563975,50.3159649914449));
#35774=CARTESIAN_POINT('Ctrl Pts',(39.6021052074275,38.8945594139917,47.9313426239604));
#35775=CARTESIAN_POINT('Ctrl Pts',(40.9441055096574,38.7683336715858,45.6097488963336));
#35776=CARTESIAN_POINT('Ctrl Pts',(43.6226417355683,38.64210792918,45.4824463675952));
#35777=CARTESIAN_POINT('Ctrl Pts',(45.1787720369989,38.515882186774,47.6663009260103));
#35778=CARTESIAN_POINT('Ctrl Pts',(44.1839423095224,38.3896564443681,50.1564969144156));
#35779=CARTESIAN_POINT('Ctrl Pts',(41.5514231764831,38.2634307019625,50.666992028518));
#35780=CARTESIAN_POINT('Ctrl Pts',(39.6979120115051,38.1372049595565,48.7291430641652));
#35781=CARTESIAN_POINT('Ctrl Pts',(40.324963613628,38.0109792171507,46.1219283557807));
#35782=CARTESIAN_POINT('Ctrl Pts',(42.8569339387272,37.8847534747447,45.2388153844359));
#35783=CARTESIAN_POINT('Ctrl Pts',(44.9694311303618,37.758527732339,46.8905168897562));
#35784=CARTESIAN_POINT('Ctrl Pts',(44.723146808684,37.6323019899332,49.5607427753764));
#35785=CARTESIAN_POINT('Ctrl Pts',(42.3441741731293,37.5060762475273,50.7981802269766));
#35786=CARTESIAN_POINT('Ctrl Pts',(40.0164505968826,37.3798505051215,49.4668406009133));
#35787=CARTESIAN_POINT('Ctrl Pts',(39.8768659443472,37.2536247627156,46.7889163353453));
#35788=CARTESIAN_POINT('Ctrl Pts',(42.0535613024942,37.1273990203097,45.2227874884231));
#35789=CARTESIAN_POINT('Ctrl Pts',(44.5482932818671,37.0011732779039,46.206186999525));
#35790=CARTESIAN_POINT('Ctrl Pts',(45.0708554612549,36.874947535498,48.8363373784985));
#35791=CARTESIAN_POINT('Ctrl Pts',(43.1415268651735,36.7487217930922,50.6987158082714));
#35792=CARTESIAN_POINT('Ctrl Pts',(40.5314639849437,36.6224960506863,50.0836271897885));
#35793=CARTESIAN_POINT('Ctrl Pts',(39.6367489718709,36.4962703082805,47.5557333445642));
#35794=CARTESIAN_POINT('Ctrl Pts',(41.2787454373714,36.3700445658746,45.4356838511265));
#35795=CARTESIAN_POINT('Ctrl Pts',(43.9500726768291,36.2438188234688,45.6697202309303));
#35796=CARTESIAN_POINT('Ctrl Pts',(45.1984068143546,36.1175930810629,48.0429931036587));
#35797=CARTESIAN_POINT('Ctrl Pts',(43.8777558631465,35.991367338657,50.3767975754204));
#35798=CARTESIAN_POINT('Ctrl Pts',(41.2004998759096,35.8651415962512,50.528661416223));
#35799=CARTESIAN_POINT('Ctrl Pts',(39.6244054199101,35.7389158538454,48.3591710352555));
#35800=CARTESIAN_POINT('Ctrl Pts',(40.5963540332916,35.6126901114394,45.8599555302844));
#35801=CARTESIAN_POINT('Ctrl Pts',(43.2240803449157,35.4864643690335,45.3253372753352));
#35802=CARTESIAN_POINT('Ctrl Pts',(45.0952868728086,35.3602386266278,47.2461049284724));
#35803=CARTESIAN_POINT('Ctrl Pts',(44.4921741735526,35.234012884222,49.858961089714));
#35804=CARTESIAN_POINT('Ctrl Pts',(41.968409971004,35.1077871418161,50.7652593282483));
#35805=CARTESIAN_POINT('Ctrl Pts',(39.8408527613417,34.9815613994102,49.1330024345044));
#35806=CARTESIAN_POINT('Ctrl Pts',(40.0626362774657,34.8553356570044,46.4606300204769));
#35807=CARTESIAN_POINT('Ctrl Pts',(42.4301594761657,34.7291099145985,45.2014254500338));
#35808=CARTESIAN_POINT('Ctrl Pts',(44.7699957628009,34.6028841721927,46.5113599525599));
#35809=CARTESIAN_POINT('Ctrl Pts',(44.9341355974128,34.4766584297868,49.1878913573846));
#35810=CARTESIAN_POINT('Ctrl Pts',(42.7718958203859,34.350432687381,50.773918276759));
#35811=CARTESIAN_POINT('Ctrl Pts',(40.2682493467455,34.2242069449751,49.8134410010433));
#35812=CARTESIAN_POINT('Ctrl Pts',(39.7215862649318,34.0979812025693,47.1881940202308));
#35813=CARTESIAN_POINT('Ctrl Pts',(41.633752569704,33.9717554601635,45.3081987442505));
#35814=CARTESIAN_POINT('Ctrl Pts',(44.2493470838237,33.8455297177575,45.8993228451264));
#35815=CARTESIAN_POINT('Ctrl Pts',(45.1672094453306,33.7193039753518,48.4189043199531));
#35816=CARTESIAN_POINT('Ctrl Pts',(43.5447265351681,33.5930782329459,50.5539245204464));
#35817=CARTESIAN_POINT('Ctrl Pts',(40.8713649794366,33.46685249054,50.3443984961964));
#35818=CARTESIAN_POINT('Ctrl Pts',(39.6013167923734,33.3406267481341,47.9826748332197));
#35819=CARTESIAN_POINT('Ctrl Pts',(40.9005066325494,33.2144010057282,45.6368557972682));
#35820=CARTESIAN_POINT('Ctrl Pts',(43.5762584883044,33.0881752633225,45.4604437035877));
#35821=CARTESIAN_POINT('Ctrl Pts',(45.1721818884761,32.9619495209166,47.6153868416661));
#35822=CARTESIAN_POINT('Ctrl Pts',(44.223201372548,32.8357237785108,50.1234127483746));
#35823=CARTESIAN_POINT('Ctrl Pts',(41.6004785517319,32.7094980361049,50.6821069398291));
#35824=CARTESIAN_POINT('Ctrl Pts',(39.7117546981783,32.583272293699,48.7785866109453));
#35825=CARTESIAN_POINT('Ctrl Pts',(40.2908367579938,32.4570465512932,46.1602999782335));
#35826=CARTESIAN_POINT('Ctrl Pts',(42.8062640312401,32.3308208088874,45.2309102338841));
#35827=CARTESIAN_POINT('Ctrl Pts',(44.9485403030968,32.2045950664815,46.843550380941));
#35828=CARTESIAN_POINT('Ctrl Pts',(44.7515982161019,32.0783693240757,49.5179137411743));
#35829=CARTESIAN_POINT('Ctrl Pts',(42.3950835667773,31.9521435816698,50.7986419402894));
#35830=CARTESIAN_POINT('Ctrl Pts',(40.0446048359227,31.8259178392639,49.510495912929));
#35831=CARTESIAN_POINT('Ctrl Pts',(39.8533765558149,31.6996920968581,46.8350429849268));
#35832=CARTESIAN_POINT('Ctrl Pts',(42.0065255322431,31.5734492335169,45.2300690624244));
#35833=CARTESIAN_POINT('Ctrl Pts',(43.6729118408661,31.4892816176444,45.8547051689911));
#35834=CARTESIAN_POINT('Ctrl Pts',(44.1890707807428,31.4471892492405,46.4508369443197));
#35835=CARTESIAN_POINT('Ctrl Pts',(40.2631768443428,31.6998,46.9876066983108));
#35836=CARTESIAN_POINT('Ctrl Pts',(40.2699897636978,31.6998,46.9743722232763));
#35837=CARTESIAN_POINT('Ctrl Pts',(40.2768026830528,31.6998,46.9611377482418));
#35838=CARTESIAN_POINT('Ctrl Pts',(40.2836156024077,31.6998,46.9479032732073));
#35839=CARTESIAN_POINT('Ctrl Pts',(41.1894856841367,46.9748,46.4934199857144));
#35840=CARTESIAN_POINT('Ctrl Pts',(41.1303103774516,46.9748,46.5309428133167));
#35841=CARTESIAN_POINT('Ctrl Pts',(41.0734841647242,46.9748,46.5719388529248));
#35842=CARTESIAN_POINT('Ctrl Pts',(41.0190945497751,46.9748,46.6160466749811));
#35843=CARTESIAN_POINT('Ctrl Pts',(40.9691207710807,46.9748,46.6565734288513));
#35844=CARTESIAN_POINT('Ctrl Pts',(40.9212038267111,46.9748,46.6997281928621));
#35845=CARTESIAN_POINT('Ctrl Pts',(40.8754251407322,46.9748,46.7452668914558));
#35846=CARTESIAN_POINT('Ctrl Pts',(40.8605791100933,46.9748,46.7600350941711));
#35847=CARTESIAN_POINT('Ctrl Pts',(40.8459553825702,46.9748,46.7750573691295));
#35848=CARTESIAN_POINT('Ctrl Pts',(40.831575992807,46.9748,46.7903053231744));
#35849=CARTESIAN_POINT('Ctrl Pts',(40.7812255431889,46.9748,46.8436971120169));
#35850=CARTESIAN_POINT('Ctrl Pts',(40.7338237459469,46.9748,46.8998950177031));
#35851=CARTESIAN_POINT('Ctrl Pts',(40.6894798075503,46.9748,46.9585357637079));
#35852=CARTESIAN_POINT('Ctrl Pts',(40.6540114853422,46.9748,47.0054393304417));
#35853=CARTESIAN_POINT('Ctrl Pts',(40.620499707712,46.9748,47.0539069081057));
#35854=CARTESIAN_POINT('Ctrl Pts',(40.5890132394166,46.9748,47.1037727021388));
#35855=CARTESIAN_POINT('Ctrl Pts',(40.5812875236016,46.9748,47.1160080836993));
#35856=CARTESIAN_POINT('Ctrl Pts',(40.5736835750194,46.9748,47.1283282812167));
#35857=CARTESIAN_POINT('Ctrl Pts',(40.5662105083118,46.9748,47.1407172084176));
#35858=CARTESIAN_POINT('Ctrl Pts',(40.526893031703,46.9748,47.2058981273756));
#35859=CARTESIAN_POINT('Ctrl Pts',(40.4911397818449,46.9748000000001,47.2730654660139));
#35860=CARTESIAN_POINT('Ctrl Pts',(40.4590588766433,46.9748,47.3418372106352));
#35861=CARTESIAN_POINT('Ctrl Pts',(40.4269779714417,46.9748,47.4106089552565));
#35862=CARTESIAN_POINT('Ctrl Pts',(40.3985688107134,46.9748,47.480985962799));
#35863=CARTESIAN_POINT('Ctrl Pts',(40.3739722403437,46.9748,47.5526268721434));
#35864=CARTESIAN_POINT('Ctrl Pts',(40.35613377041,46.9748,47.6045838803019));
#35865=CARTESIAN_POINT('Ctrl Pts',(40.3403012776577,46.9748,47.6572065634792));
#35866=CARTESIAN_POINT('Ctrl Pts',(40.3265420108385,46.9748,47.7103741641063));
#35867=CARTESIAN_POINT('Ctrl Pts',(40.3160697598934,46.9748,47.7508403069054));
#35868=CARTESIAN_POINT('Ctrl Pts',(40.3067987099654,46.9748,47.7916222866019));
#35869=CARTESIAN_POINT('Ctrl Pts',(40.2987636881035,46.9748,47.8326688703311));
#35870=CARTESIAN_POINT('Ctrl Pts',(40.295132423041,46.9748,47.8512190408216));
#35871=CARTESIAN_POINT('Ctrl Pts',(40.291752669636,46.9748,47.8698301774986));
#35872=CARTESIAN_POINT('Ctrl Pts',(40.2886337454123,46.9748,47.8884603431078));
#35873=CARTESIAN_POINT('Ctrl Pts',(40.2756479319583,46.9748,47.9660280677026));
#35874=CARTESIAN_POINT('Ctrl Pts',(40.2671589705433,46.9748,48.0440153075512));
#35875=CARTESIAN_POINT('Ctrl Pts',(40.2633055724053,46.9748,48.1220534670357));
#35876=CARTESIAN_POINT('Ctrl Pts',(40.2620603022212,46.9748,48.1472724010129));
#35877=CARTESIAN_POINT('Ctrl Pts',(40.2612994708194,46.9748,48.1724968887305));
#35878=CARTESIAN_POINT('Ctrl Pts',(40.2610287627922,46.9748,48.1977150825715));
#35879=CARTESIAN_POINT('Ctrl Pts',(40.260220477777,46.9748,48.2730120303637));
#35880=CARTESIAN_POINT('Ctrl Pts',(40.2637777325354,46.9748,48.3482521489875));
#35881=CARTESIAN_POINT('Ctrl Pts',(40.2714763918892,46.9748,48.4231811150368));
#35882=CARTESIAN_POINT('Ctrl Pts',(40.2793378346931,46.9748,48.4996944083113));
#35883=CARTESIAN_POINT('Ctrl Pts',(40.2915177567416,46.9748,48.5758840323195));
#35884=CARTESIAN_POINT('Ctrl Pts',(40.3078313114295,46.9748,48.6514834531951));
#35885=CARTESIAN_POINT('Ctrl Pts',(40.3105992632564,46.9748,48.6643105506073));
#35886=CARTESIAN_POINT('Ctrl Pts',(40.3134868120037,46.9748,48.6771226603303));
#35887=CARTESIAN_POINT('Ctrl Pts',(40.3164916889436,46.9748,48.6899120610965));
#35888=CARTESIAN_POINT('Ctrl Pts',(40.334438038668,46.9748,48.7662955747993));
#35889=CARTESIAN_POINT('Ctrl Pts',(40.3565050181593,46.9748,48.8416188377461));
#35890=CARTESIAN_POINT('Ctrl Pts',(40.3824237798636,46.9748,48.9156073690414));
#35891=CARTESIAN_POINT('Ctrl Pts',(40.4090078674698,46.9748,48.9914951610683));
#35892=CARTESIAN_POINT('Ctrl Pts',(40.4396441318805,46.9748,49.0659796543946));
#35893=CARTESIAN_POINT('Ctrl Pts',(40.4740987705517,46.9748,49.138769661897));
#35894=CARTESIAN_POINT('Ctrl Pts',(40.5085534092228,46.9748,49.2115596693994));
#35895=CARTESIAN_POINT('Ctrl Pts',(40.5468267806189,46.9748,49.2826561015899));
#35896=CARTESIAN_POINT('Ctrl Pts',(40.5887367591054,46.9748,49.3517594213202));
#35897=CARTESIAN_POINT('Ctrl Pts',(40.6024581151758,46.9748,49.3743838962045));
#35898=CARTESIAN_POINT('Ctrl Pts',(40.6165696726842,46.9748,49.3967946016751));
#35899=CARTESIAN_POINT('Ctrl Pts',(40.6310661433443,46.9748,49.4189805740005));
#35900=CARTESIAN_POINT('Ctrl Pts',(40.640039849335,46.9748,49.4327142887392));
#35901=CARTESIAN_POINT('Ctrl Pts',(40.6491610622686,46.9748,49.4463618817698));
#35902=CARTESIAN_POINT('Ctrl Pts',(40.6584286263235,46.9748,49.4599206942245));
#35903=CARTESIAN_POINT('Ctrl Pts',(40.6661836146128,46.9748,49.471266548559));
#35904=CARTESIAN_POINT('Ctrl Pts',(40.6740417848548,46.9748,49.4825510866558));
#35905=CARTESIAN_POINT('Ctrl Pts',(40.6819922247109,46.9748,49.4937586649968));
#35906=CARTESIAN_POINT('Ctrl Pts',(40.7302234805214,46.9748,49.5617493155483));
#35907=CARTESIAN_POINT('Ctrl Pts',(40.7819280150356,46.9748,49.6270299832024));
#35908=CARTESIAN_POINT('Ctrl Pts',(40.8368603491323,46.9748,49.6893013090378));
#35909=CARTESIAN_POINT('Ctrl Pts',(40.8917630700629,46.9748,49.751539065371));
#35910=CARTESIAN_POINT('Ctrl Pts',(40.9498905292052,46.9748,49.8107716637567));
#35911=CARTESIAN_POINT('Ctrl Pts',(41.0110467528271,46.9748,49.8666848752274));
#35912=CARTESIAN_POINT('Ctrl Pts',(41.0714906757508,46.9748,49.9219468525765));
#35913=CARTESIAN_POINT('Ctrl Pts',(41.1348936992962,46.9748,49.9739671882265));
#35914=CARTESIAN_POINT('Ctrl Pts',(41.201107808354,46.9748,50.0224141023343));
#35915=CARTESIAN_POINT('Ctrl Pts',(41.2364136632063,46.9748,50.0482463568473));
#35916=CARTESIAN_POINT('Ctrl Pts',(41.2725193969755,46.9748,50.07306209005));
#35917=CARTESIAN_POINT('Ctrl Pts',(41.309406738763,46.9748,50.0968063285493));
#35918=CARTESIAN_POINT('Origin',(42.4,46.9748,48.));
#35919=CARTESIAN_POINT('',(43.5298844544276,46.9748,50.0758977721803));
#35920=CARTESIAN_POINT('',(42.4,46.9748,45.63653));
#35921=CARTESIAN_POINT('Origin',(42.4,46.9748,48.));
#35922=CARTESIAN_POINT('Ctrl Pts',(43.5298844544276,46.9748,50.0758977721802));
#35923=CARTESIAN_POINT('Ctrl Pts',(43.5991352573157,46.9748,50.029019463505));
#35924=CARTESIAN_POINT('Ctrl Pts',(43.6656582922104,46.9748,49.9781660525874));
#35925=CARTESIAN_POINT('Ctrl Pts',(43.7292694101079,46.9748,49.9236952395323));
#35926=CARTESIAN_POINT('Ctrl Pts',(43.783302831196,46.9748,49.877425900522));
#35927=CARTESIAN_POINT('Ctrl Pts',(43.8352347245068,46.9748,49.8285454219465));
#35928=CARTESIAN_POINT('Ctrl Pts',(43.8849274853458,46.9748,49.7772569750236));
#35929=CARTESIAN_POINT('Ctrl Pts',(43.8965951848529,46.9748,49.7652146135855));
#35930=CARTESIAN_POINT('Ctrl Pts',(43.9081376356664,46.9748,49.7530410983771));
#35931=CARTESIAN_POINT('Ctrl Pts',(43.9195457502883,46.9748,49.7407472087553));
#35932=CARTESIAN_POINT('Ctrl Pts',(43.9760402133417,46.9748,49.6798662730318));
#35933=CARTESIAN_POINT('Ctrl Pts',(44.0292971033833,46.9748,49.6159808674749));
#35934=CARTESIAN_POINT('Ctrl Pts',(44.0791167399533,46.9748,49.5494290633886));
#35935=CARTESIAN_POINT('Ctrl Pts',(44.1148930930423,46.9748,49.501637047918));
#35936=CARTESIAN_POINT('Ctrl Pts',(44.1488959960298,46.9748,49.4524693038681));
#35937=CARTESIAN_POINT('Ctrl Pts',(44.1810358371969,46.9748,49.4020455179199));
#35938=CARTESIAN_POINT('Ctrl Pts',(44.1889018950558,46.9748,49.3897045603006));
#35939=CARTESIAN_POINT('Ctrl Pts',(44.1966562900803,46.9748,49.3772883533));
#35940=CARTESIAN_POINT('Ctrl Pts',(44.2042975790103,46.9748,49.3647986325625));
#35941=CARTESIAN_POINT('Ctrl Pts',(44.2119123601123,46.9748,49.3523522389879));
#35942=CARTESIAN_POINT('Ctrl Pts',(44.2194101741558,46.9748,49.3398403918988));
#35943=CARTESIAN_POINT('Ctrl Pts',(44.2267882958736,46.9748,49.3272680159029));
#35944=CARTESIAN_POINT('Ctrl Pts',(44.2678706899769,46.9748,49.2572633012563));
#35945=CARTESIAN_POINT('Ctrl Pts',(44.3052645362015,46.9748,49.1853532663675));
#35946=CARTESIAN_POINT('Ctrl Pts',(44.3387904821095,46.9748,49.1118543951674));
#35947=CARTESIAN_POINT('Ctrl Pts',(44.3715702155164,46.9748,49.0399914442977));
#35948=CARTESIAN_POINT('Ctrl Pts',(44.400652486977,46.9748,48.9666086718443));
#35949=CARTESIAN_POINT('Ctrl Pts',(44.4258221217546,46.9748,48.8919915357821));
#35950=CARTESIAN_POINT('Ctrl Pts',(44.450471949,46.9748,48.8189154053683));
#35951=CARTESIAN_POINT('Ctrl Pts',(44.4713692237863,46.9748,48.7446546031674));
#35952=CARTESIAN_POINT('Ctrl Pts',(44.4882633994834,46.9748,48.6694795181181));
#35953=CARTESIAN_POINT('Ctrl Pts',(44.4959612735851,46.9748,48.6352257995188));
#35954=CARTESIAN_POINT('Ctrl Pts',(44.5028273418609,46.9748,48.6007823587082));
#35955=CARTESIAN_POINT('Ctrl Pts',(44.5088343375696,46.9748,48.56617557783));
#35956=CARTESIAN_POINT('Ctrl Pts',(44.5109619703709,46.9748,48.5539181157449));
#35957=CARTESIAN_POINT('Ctrl Pts',(44.5129809047883,46.9748,48.5416451070528));
#35958=CARTESIAN_POINT('Ctrl Pts',(44.5148890604002,46.9748,48.5293655357747));
#35959=CARTESIAN_POINT('Ctrl Pts',(44.5265958064881,46.9748000000001,48.4540290055026));
#35960=CARTESIAN_POINT('Ctrl Pts',(44.5341527504262,46.9748000000001,48.378355707931));
#35961=CARTESIAN_POINT('Ctrl Pts',(44.5373669491418,46.9748000000001,48.30261096484));
#35962=CARTESIAN_POINT('Ctrl Pts',(44.5384531833379,46.9748000000001,48.2770131292999));
#35963=CARTESIAN_POINT('Ctrl Pts',(44.5390430018181,46.9748,48.2514071468793));
#35964=CARTESIAN_POINT('Ctrl Pts',(44.5391275997232,46.9748,48.2258033809724));
#35965=CARTESIAN_POINT('Ctrl Pts',(44.5393841841558,46.9748,48.1481474657363));
#35966=CARTESIAN_POINT('Ctrl Pts',(44.5349968811804,46.9748,48.0705105032779));
#35967=CARTESIAN_POINT('Ctrl Pts',(44.5261344730417,46.9748,47.9932236009828));
#35968=CARTESIAN_POINT('Ctrl Pts',(44.5175967452688,46.9748,47.9187681570591));
#35969=CARTESIAN_POINT('Ctrl Pts',(44.504905015825,46.9748,47.8446369257264));
#35970=CARTESIAN_POINT('Ctrl Pts',(44.4881708657763,46.9748,47.7711493147464));
#35971=CARTESIAN_POINT('Ctrl Pts',(44.4840507442499,46.9748,47.7530559017529));
#35972=CARTESIAN_POINT('Ctrl Pts',(44.4796836110545,46.9748,47.7349951900705));
#35973=CARTESIAN_POINT('Ctrl Pts',(44.4750802303516,46.9748,47.717007252933));
#35974=CARTESIAN_POINT('Ctrl Pts',(44.4562684669595,46.9748000000001,47.6434993596734));
#35975=CARTESIAN_POINT('Ctrl Pts',(44.433498427294,46.9748,47.5711172123902));
#35976=CARTESIAN_POINT('Ctrl Pts',(44.4069542493271,46.9748,47.5001602010979));
#35977=CARTESIAN_POINT('Ctrl Pts',(44.3805282755863,46.9748000000001,47.4295191694009));
#35978=CARTESIAN_POINT('Ctrl Pts',(44.3503610512703,46.9748000000001,47.3602897711562));
#35979=CARTESIAN_POINT('Ctrl Pts',(44.3165910991924,46.9748,47.292794375311));
#35980=CARTESIAN_POINT('Ctrl Pts',(44.283107711654,46.9748,47.2258717308571));
#35981=CARTESIAN_POINT('Ctrl Pts',(44.2460818591245,46.9748,47.1606530350058));
#35982=CARTESIAN_POINT('Ctrl Pts',(44.2056155224222,46.9748,47.0974908446937));
#35983=CARTESIAN_POINT('Ctrl Pts',(44.1908426060719,46.9748,47.0744324255229));
#35984=CARTESIAN_POINT('Ctrl Pts',(44.1756108890014,46.9748,47.0516485112693));
#35985=CARTESIAN_POINT('Ctrl Pts',(44.1599244680382,46.9748,47.0291578416167));
#35986=CARTESIAN_POINT('Ctrl Pts',(44.1531635220926,46.9748,47.0194642217554));
#35987=CARTESIAN_POINT('Ctrl Pts',(44.14631890799,46.9748,47.0098263625416));
#35988=CARTESIAN_POINT('Ctrl Pts',(44.1393981503246,46.9748,47.0002553228382));
#35989=CARTESIAN_POINT('Ctrl Pts',(44.0965694162336,46.9748000000001,46.9410254618529));
#35990=CARTESIAN_POINT('Ctrl Pts',(44.0507558491961,46.9748,46.8842480501475));
#35991=CARTESIAN_POINT('Ctrl Pts',(44.0020911747138,46.9748,46.8302142717846));
#35992=CARTESIAN_POINT('Ctrl Pts',(43.9547299363546,46.9748,46.7776277357865));
#35993=CARTESIAN_POINT('Ctrl Pts',(43.9046676139366,46.9748,46.7276393346297));
#35994=CARTESIAN_POINT('Ctrl Pts',(43.8520000209609,46.9748,46.6805567605905));
#35995=CARTESIAN_POINT('Ctrl Pts',(43.799933010938,46.9748,46.6340110820073));
#35996=CARTESIAN_POINT('Ctrl Pts',(43.745319295441,46.9748,46.5903048219264));
#35997=CARTESIAN_POINT('Ctrl Pts',(43.6882327293054,46.9748,46.5497817346553));
#35998=CARTESIAN_POINT('Ctrl Pts',(43.6621533214997,46.9748,46.5312691810016));
#35999=CARTESIAN_POINT('Ctrl Pts',(43.6355576110044,46.9748,46.5134216543318));
#36000=CARTESIAN_POINT('Ctrl Pts',(43.6084517554458,46.9748,46.4962756530335));
#36001=CARTESIAN_POINT('Origin',(42.4,46.9748,48.));
#36002=CARTESIAN_POINT('Ctrl Pts',(43.8816454908891,47.2273349779972,46.1547938147578));
#36003=CARTESIAN_POINT('Ctrl Pts',(44.4964807713991,47.1852426082705,46.6484554351011));
#36004=CARTESIAN_POINT('Ctrl Pts',(45.1824651975149,47.1010749910753,48.2904339462144));
#36005=CARTESIAN_POINT('Ctrl Pts',(43.6585580275758,46.9748321264113,50.5015145553006));
#36006=CARTESIAN_POINT('Ctrl Pts',(40.9780001174031,46.8486063840055,50.4096758350311));
#36007=CARTESIAN_POINT('Ctrl Pts',(39.6036218446586,46.7223806415996,48.1087275911241));
#36008=CARTESIAN_POINT('Ctrl Pts',(40.7959828223584,46.5961548991938,45.7064576286955));
#36009=CARTESIAN_POINT('Ctrl Pts',(43.4610518931062,46.4699291567879,45.410456497768));
#36010=CARTESIAN_POINT('Ctrl Pts',(45.1519601603745,46.3437034143821,47.4913191856257));
#36011=CARTESIAN_POINT('Ctrl Pts',(44.3165710055188,46.2174776719761,50.0393512686995));
#36012=CARTESIAN_POINT('Ctrl Pts',(41.7217124725944,46.0912519295704,50.7151277184636));
#36013=CARTESIAN_POINT('Ctrl Pts',(39.7495457958656,45.9650261871645,48.8984192274595));
#36014=CARTESIAN_POINT('Ctrl Pts',(40.2105349755461,45.8388004447587,46.2569221858256));
#36015=CARTESIAN_POINT('Ctrl Pts',(42.6814934434515,45.7125747023527,45.2156125251515));
#36016=CARTESIAN_POINT('Ctrl Pts',(44.8940345654646,45.586348959947,46.7304117848254));
#36017=CARTESIAN_POINT('Ctrl Pts',(44.8170102955553,45.460123217541,49.4107177431346));
#36018=CARTESIAN_POINT('Ctrl Pts',(42.5211290349961,45.3338974751353,50.7959592378664));
#36019=CARTESIAN_POINT('Ctrl Pts',(40.1140494587796,45.2076717327294,49.6144633468875));
#36020=CARTESIAN_POINT('Ctrl Pts',(39.8055112890285,45.0814459903235,46.9508622273783));
#36021=CARTESIAN_POINT('Ctrl Pts',(41.8787579687848,44.9552202479177,45.2503876399901));
#36022=CARTESIAN_POINT('Ctrl Pts',(44.4305136800393,44.8289945055118,46.0741039016234));
#36023=CARTESIAN_POINT('Ctrl Pts',(45.1182232833989,44.702768763106,48.6658256135953));
#36024=CARTESIAN_POINT('Ctrl Pts',(43.3105576378377,44.5765430207001,50.6463080535969));
#36025=CARTESIAN_POINT('Ctrl Pts',(40.6669845849055,44.4503172782943,50.1974346689313));
#36026=CARTESIAN_POINT('Ctrl Pts',(39.6143491799657,44.3240915358884,47.7312788480869));
#36027=CARTESIAN_POINT('Ctrl Pts',(41.1189886446677,44.1978657934826,45.511813621966));
#36028=CARTESIAN_POINT('Ctrl Pts',(43.7996183379206,44.0716400510767,45.5765458419894));
#36029=CARTESIAN_POINT('Ctrl Pts',(45.1953745735294,43.9454143086709,47.8660502307715));
#36030=CARTESIAN_POINT('Ctrl Pts',(44.0249293689912,43.819188566265,50.2785227873245));
#36031=CARTESIAN_POINT('Ctrl Pts',(41.3627713449932,43.6929628238591,50.599272641384));
#36032=CARTESIAN_POINT('Ctrl Pts',(39.6528068814801,43.5667370814533,48.5338459669609));
#36033=CARTESIAN_POINT('Ctrl Pts',(40.4648124622021,43.4405113390474,45.9783396080465));
#36034=CARTESIAN_POINT('Ctrl Pts',(43.0533531424619,43.3142855966417,45.2787519006654));
#36035=CARTESIAN_POINT('Ctrl Pts',(45.0421045168773,43.1880598542357,47.0773162682832));
#36036=CARTESIAN_POINT('Ctrl Pts',(44.6053589721454,43.0618341118299,49.7229200070962));
#36037=CARTESIAN_POINT('Ctrl Pts',(42.1440563524087,42.935608369424,50.7868538526695));
#36038=CARTESIAN_POINT('Ctrl Pts',(39.917714357712,42.8093826270182,49.2924084249837));
#36039=CARTESIAN_POINT('Ctrl Pts',(39.9701528349268,42.6831568846123,46.6115100643995));
#36040=CARTESIAN_POINT('Ctrl Pts',(42.2532323693868,42.5569311422065,45.2052690989143));
#36041=CARTESIAN_POINT('Ctrl Pts',(44.6710470869588,42.4307053998006,46.3646386712122));
#36042=CARTESIAN_POINT('Ctrl Pts',(45.0040019220144,42.3044796573948,49.0252977796835));
#36043=CARTESIAN_POINT('Ctrl Pts',(42.946438668573,42.1782539149889,50.7447160742719));
#36044=CARTESIAN_POINT('Ctrl Pts',(40.3872354161611,42.0520281725831,49.9444382934213));
#36045=CARTESIAN_POINT('Ctrl Pts',(39.6757843120393,41.9258024301772,47.3591330619018));
#36046=CARTESIAN_POINT('Ctrl Pts',(41.4652095797749,41.7995766877714,45.3621545880901));
#36047=CARTESIAN_POINT('Ctrl Pts',(44.1127883648371,41.6733509453655,45.7867631025674));
#36048=CARTESIAN_POINT('Ctrl Pts',(45.1879982767062,41.5471252029597,48.2431607615583));
#36049=CARTESIAN_POINT('Ctrl Pts',(43.7037783145724,41.4208994605538,50.4763327024714));
#36050=CARTESIAN_POINT('Ctrl Pts',(41.0226676673639,41.294673718148,50.4361890715529));
#36051=CARTESIAN_POINT('Ctrl Pts',(39.6059715458142,41.1684479757421,48.1595824052919));
#36052=CARTESIAN_POINT('Ctrl Pts',(40.7542411038366,41.0422222333363,45.7364763746368));
#36053=CARTESIAN_POINT('Ctrl Pts',(43.4133453418658,40.9159964909304,45.3913235606926));
#36054=CARTESIAN_POINT('Ctrl Pts',(45.1421813073775,40.7897707485246,47.4409801216879));
#36055=CARTESIAN_POINT('Ctrl Pts',(44.3536481566047,40.6635450061187,50.0038264463454));
#36056=CARTESIAN_POINT('Ctrl Pts',(41.771632743995,40.5373192637129,50.7271259850728));
#36057=CARTESIAN_POINT('Ctrl Pts',(39.7664691681677,40.411093521307,48.946877449656));
#36058=CARTESIAN_POINT('Ctrl Pts',(40.1789317226774,40.2848677789012,46.2973792981554));
#36059=CARTESIAN_POINT('Ctrl Pts',(42.6303727617419,40.1586420364953,45.2109159321516));
#36060=CARTESIAN_POINT('Ctrl Pts',(44.8703276842312,40.0324162940895,46.6848792149011));
#36061=CARTESIAN_POINT('Ctrl Pts',(44.8424797438481,39.9061905516836,49.3661457637348));
#36062=CARTESIAN_POINT('Ctrl Pts',(42.5723938238785,39.7799648092778,50.7932672475736));
#36063=CARTESIAN_POINT('Ctrl Pts',(40.1440474391825,39.6537390668719,49.6561218524672));
#36064=CARTESIAN_POINT('Ctrl Pts',(39.7867039050733,39.527513324466,46.998628407074));
#36065=CARTESIAN_POINT('Ctrl Pts',(41.8284106683955,39.4012875820602,45.2604111288599));
#36066=CARTESIAN_POINT('Ctrl Pts',(44.3948461674537,39.2750618396543,46.0371830663371));
#36067=CARTESIAN_POINT('Ctrl Pts',(45.1299789294624,39.1488360972485,48.6158543590574));
#36068=CARTESIAN_POINT('Ctrl Pts',(43.3589445658158,39.0226103548426,50.6291608673817));
#36069=CARTESIAN_POINT('Ctrl Pts',(40.7075827680497,38.8963846124368,50.228852947118));
#36070=CARTESIAN_POINT('Ctrl Pts',(39.6098887967391,38.7701588700309,47.7824200829205));
#36071=CARTESIAN_POINT('Ctrl Pts',(41.0735644019736,38.6439331276251,45.5357292861443));
#36072=CARTESIAN_POINT('Ctrl Pts',(43.7549304641552,38.5177073852192,45.5512809503369));
#36073=CARTESIAN_POINT('Ctrl Pts',(45.1924472972574,38.3914816428134,47.8147983830566));
#36074=CARTESIAN_POINT('Ctrl Pts',(44.0664499797616,38.2652559004075,50.2483340525446));
#36075=CARTESIAN_POINT('Ctrl Pts',(41.4106232153221,38.1390301580017,50.6178607917188));
#36076=CARTESIAN_POINT('Ctrl Pts',(39.6630611799201,38.0128044155958,48.5841467641083));
#36077=CARTESIAN_POINT('Ctrl Pts',(40.4280555682283,37.8865786731899,46.0141760639767));
#36078=CARTESIAN_POINT('Ctrl Pts',(43.0033285104073,37.7603529307841,45.2672255388693));
#36079=CARTESIAN_POINT('Ctrl Pts',(45.0247356104603,37.6341271883782,47.0290084850729));
#36080=CARTESIAN_POINT('Ctrl Pts',(44.6365907431038,37.5079014459724,49.6821781697375));
#36081=CARTESIAN_POINT('Ctrl Pts',(42.1952175033893,37.3816757035665,50.7910796613426));
#36082=CARTESIAN_POINT('Ctrl Pts',(39.9418380812742,37.2554499611607,49.3377225153987));
#36083=CARTESIAN_POINT('Ctrl Pts',(39.9450931422177,37.1292242187548,46.6563133302395));
#36084=CARTESIAN_POINT('Ctrl Pts',(42.2019944848676,37.002998476349,45.2084313795187));
#36085=CARTESIAN_POINT('Ctrl Pts',(44.6406682607653,36.8767727339431,46.3232569391591));
#36086=CARTESIAN_POINT('Ctrl Pts',(45.0223704336859,36.7505469915373,48.9773611693779));
#36087=CARTESIAN_POINT('Ctrl Pts',(42.9966919117353,36.6243212491314,50.7342312099288));
#36088=CARTESIAN_POINT('Ctrl Pts',(40.4232400582042,36.4980955067256,49.9810304589759));
#36089=CARTESIAN_POINT('Ctrl Pts',(39.6644874787135,36.3718697643197,47.4092100265205));
#36090=CARTESIAN_POINT('Ctrl Pts',(41.416981956363,36.2456440219139,45.3797448458667));
#36091=CARTESIAN_POINT('Ctrl Pts',(44.0719037305385,36.119418279508,45.7557184974497));
#36092=CARTESIAN_POINT('Ctrl Pts',(45.1919894217268,35.9931925371022,48.1919807694713));
#36093=CARTESIAN_POINT('Ctrl Pts',(43.7489812998462,35.8669667946963,50.4520014273119));
#36094=CARTESIAN_POINT('Ctrl Pts',(41.067585382989,35.7407410522905,50.4610430380741));
#36095=CARTESIAN_POINT('Ctrl Pts',(39.6093687642723,35.6145153098846,48.2108052491722));
#36096=CARTESIAN_POINT('Ctrl Pts',(40.7129991207698,35.4882895674788,45.7670446533085));
#36097=CARTESIAN_POINT('Ctrl Pts',(43.365324999706,35.3620638250729,45.3731750740055));
#36098=CARTESIAN_POINT('Ctrl Pts',(45.1314660976564,35.2358380826671,47.3907754893571));
#36099=CARTESIAN_POINT('Ctrl Pts',(44.3900748241373,35.1096123402612,49.9676543753674));
#36100=CARTESIAN_POINT('Ctrl Pts',(41.821760988144,34.9833865978554,50.7381930523941));
#36101=CARTESIAN_POINT('Ctrl Pts',(39.784280407157,34.8571608554495,48.9950238989286));
#36102=CARTESIAN_POINT('Ctrl Pts',(40.1480749367121,34.7309351130437,46.3384058697562));
#36103=CARTESIAN_POINT('Ctrl Pts',(42.5791750040333,34.6047093706378,45.2071595343498));
#36104=CARTESIAN_POINT('Ctrl Pts',(44.8457893708704,34.478483628232,46.6397882861432));
#36105=CARTESIAN_POINT('Ctrl Pts',(44.8671274581151,34.3522578858261,49.3211145415032));
#36106=CARTESIAN_POINT('Ctrl Pts',(42.623600556591,34.2260321434202,50.7896351656127));
#36107=CARTESIAN_POINT('Ctrl Pts',(40.174804514126,34.0998064010144,49.6972232134327));
#36108=CARTESIAN_POINT('Ctrl Pts',(39.7687758515636,33.9735806586085,47.0467314826819));
#36109=CARTESIAN_POINT('Ctrl Pts',(41.7782556499994,33.8473549162027,45.2713564357832));
#36110=CARTESIAN_POINT('Ctrl Pts',(44.3585075330677,33.7211291737969,46.000922708281));
#36111=CARTESIAN_POINT('Ctrl Pts',(45.1408157896746,33.594903431391,48.5656757993766));
#36112=CARTESIAN_POINT('Ctrl Pts',(43.4070092426123,33.4686776889851,50.6111292011137));
#36113=CARTESIAN_POINT('Ctrl Pts',(40.7487495907286,33.3424519465793,50.2595209084501));
#36114=CARTESIAN_POINT('Ctrl Pts',(39.6063688620587,33.2162262041734,47.8336352383348));
#36115=CARTESIAN_POINT('Ctrl Pts',(41.0285832239457,33.0900004617676,45.5604727126079));
#36116=CARTESIAN_POINT('Ctrl Pts',(43.7097931512442,32.9637747193617,45.5268428077786));
#36117=CARTESIAN_POINT('Ctrl Pts',(45.188567568384,32.8375489769558,47.763603269987));
#36118=CARTESIAN_POINT('Ctrl Pts',(44.1074354187682,32.7113232345501,50.2173998978709));
#36119=CARTESIAN_POINT('Ctrl Pts',(41.4587571919215,32.5850974921442,50.635546029088));
#36120=CARTESIAN_POINT('Ctrl Pts',(39.6743373833067,32.4588717497383,48.6342948602794));
#36121=CARTESIAN_POINT('Ctrl Pts',(40.3917614339282,32.3326460073325,46.0505935321538));
#36122=CARTESIAN_POINT('Ctrl Pts',(42.9535000609079,32.2064202649266,45.2567919948868));
#36123=CARTESIAN_POINT('Ctrl Pts',(45.0056887756311,32.0801945225208,46.9806829244104));
#36124=CARTESIAN_POINT('Ctrl Pts',(44.6686649560567,31.9539687801149,49.641554962929));
#36125=CARTESIAN_POINT('Ctrl Pts',(42.2430969350261,31.8277430377091,50.7930037613584));
#36126=CARTESIAN_POINT('Ctrl Pts',(40.7318882605603,31.7435925427718,49.8543657264344));
#36127=CARTESIAN_POINT('Ctrl Pts',(40.3425084896344,31.7015172953032,49.1690970811863));
#36128=CARTESIAN_POINT('Ctrl Pts',(43.7896421530199,47.1424960903491,46.2693725916266));
#36129=CARTESIAN_POINT('Ctrl Pts',(44.3662990039429,47.1004037206223,46.7323801067006));
#36130=CARTESIAN_POINT('Ctrl Pts',(45.0096869673307,47.0162361034272,48.2723993403344));
#36131=CARTESIAN_POINT('Ctrl Pts',(43.5804073902262,46.8899932387631,50.3461820616432));
#36132=CARTESIAN_POINT('Ctrl Pts',(41.066299738637,46.7637674963574,50.2600461014889));
#36133=CARTESIAN_POINT('Ctrl Pts',(39.7772640052281,46.6375417539514,48.1019761101771));
#36134=CARTESIAN_POINT('Ctrl Pts',(40.8955848764598,46.5113160115457,45.8488760108268));
#36135=CARTESIAN_POINT('Ctrl Pts',(43.3951654739739,46.3850902691396,45.5712551822226));
#36136=CARTESIAN_POINT('Ctrl Pts',(44.9810761520241,46.258864526734,47.5229059134362));
#36137=CARTESIAN_POINT('Ctrl Pts',(44.1975608031085,46.132638784328,49.9127169793489));
#36138=CARTESIAN_POINT('Ctrl Pts',(41.7638309934822,46.0064130419222,50.5465308345424));
#36139=CARTESIAN_POINT('Ctrl Pts',(39.9141267534222,45.8801872995164,48.8426315452909));
#36140=CARTESIAN_POINT('Ctrl Pts',(40.3464906354096,45.7539615571105,46.365159262816));
#36141=CARTESIAN_POINT('Ctrl Pts',(42.6640140014762,45.6277358147047,45.3885101198748));
#36142=CARTESIAN_POINT('Ctrl Pts',(44.7391665446088,45.5015100722988,46.8092473458512));
#36143=CARTESIAN_POINT('Ctrl Pts',(44.6669251259093,45.3752843298929,49.3231186906233));
#36144=CARTESIAN_POINT('Ctrl Pts',(42.5136074816954,45.249058587487,50.6223430901361));
#36145=CARTESIAN_POINT('Ctrl Pts',(40.2559964233466,45.1228328450813,49.5142126339507));
#36146=CARTESIAN_POINT('Ctrl Pts',(39.9666170480926,44.9966071026753,47.0160088346871));
#36147=CARTESIAN_POINT('Ctrl Pts',(41.911124690112,44.8703813602696,45.4211258607879));
#36148=CARTESIAN_POINT('Ctrl Pts',(44.3044281641036,44.7441556178636,46.1936931492063));
#36149=CARTESIAN_POINT('Ctrl Pts',(44.9494341792005,44.6179298754578,48.624480919965));
#36150=CARTESIAN_POINT('Ctrl Pts',(43.2540162164799,44.491704133052,50.4819845528282));
#36151=CARTESIAN_POINT('Ctrl Pts',(40.7745968334143,44.3654783906461,50.0609841309757));
#36152=CARTESIAN_POINT('Ctrl Pts',(39.7873252225867,44.2392526482402,47.7479651897821));
#36153=CARTESIAN_POINT('Ctrl Pts',(41.1985335299076,44.1130269058345,45.6663184974085));
#36154=CARTESIAN_POINT('Ctrl Pts',(43.7127085071794,43.9868011634285,45.727031145715));
#36155=CARTESIAN_POINT('Ctrl Pts',(45.0217947307526,43.8605754210227,47.8743678924197));
#36156=CARTESIAN_POINT('Ctrl Pts',(43.9240287644484,43.7343496786169,50.1370370519486));
#36157=CARTESIAN_POINT('Ctrl Pts',(41.4271784511338,43.6081239362109,50.4378698223493));
#36158=CARTESIAN_POINT('Ctrl Pts',(39.8233948785613,43.4818981938052,48.5006965994701));
#36159=CARTESIAN_POINT('Ctrl Pts',(40.5849786652346,43.3556724513993,46.1038753757059));
#36160=CARTESIAN_POINT('Ctrl Pts',(43.01278293165,43.2294467089935,45.4477288319546));
#36161=CARTESIAN_POINT('Ctrl Pts',(44.878042036313,43.1032209665876,47.1346106640329));
#36162=CARTESIAN_POINT('Ctrl Pts',(44.4684163715807,42.9769952241817,49.6159346367703));
#36163=CARTESIAN_POINT('Ctrl Pts',(42.1599492701339,42.8507694817759,50.6138031072814));
#36164=CARTESIAN_POINT('Ctrl Pts',(40.0718528247337,42.72454373937,49.2121558343877));
#36165=CARTESIAN_POINT('Ctrl Pts',(40.121035114847,42.5983179969642,46.6977288727842));
#36166=CARTESIAN_POINT('Ctrl Pts',(42.2623459609919,42.4720922545583,45.378808972607));
#36167=CARTESIAN_POINT('Ctrl Pts',(44.5300255580282,42.3458665121525,46.4661870522494));
#36168=CARTESIAN_POINT('Ctrl Pts',(44.842305436508,42.2196407697466,48.9616315257646));
#36169=CARTESIAN_POINT('Ctrl Pts',(42.9125073525067,42.0934150273407,50.5742818901914));
#36170=CARTESIAN_POINT('Ctrl Pts',(40.5122187952467,41.9671892849349,49.823697661215));
#36171=CARTESIAN_POINT('Ctrl Pts',(39.8449455168682,41.840963542529,47.3989279371251));
#36172=CARTESIAN_POINT('Ctrl Pts',(41.5232557449324,41.7147378001232,45.5259525979185));
#36173=CARTESIAN_POINT('Ctrl Pts',(44.0064321226742,41.5885120577173,45.9241948858863));
#36174=CARTESIAN_POINT('Ctrl Pts',(45.0148764678742,41.4622863153115,48.2280616019822));
#36175=CARTESIAN_POINT('Ctrl Pts',(43.6228197063765,41.3360605729056,50.3225638855021));
#36176=CARTESIAN_POINT('Ctrl Pts',(41.1081936401671,41.2098348304998,50.2849129885481));
#36177=CARTESIAN_POINT('Ctrl Pts',(39.7794678008006,41.0836090880939,48.1496730754001));
#36178=CARTESIAN_POINT('Ctrl Pts',(40.8564351257576,40.9573833456881,45.8770307313704));
#36179=CARTESIAN_POINT('Ctrl Pts',(43.3504212790996,40.8311576032823,45.5533103121206));
#36180=CARTESIAN_POINT('Ctrl Pts',(44.9719045206072,40.7049318608764,47.4756926727375));
#36181=CARTESIAN_POINT('Ctrl Pts',(44.2323356344563,40.5787061184706,49.8793980842926));
#36182=CARTESIAN_POINT('Ctrl Pts',(41.810651446725,40.4524803760646,50.5577840642425));
#36183=CARTESIAN_POINT('Ctrl Pts',(39.9299992625121,40.3262546336588,48.8880807358286));
#36184=CARTESIAN_POINT('Ctrl Pts',(40.3168497984963,40.200028891253,46.4031041754342));
#36185=CARTESIAN_POINT('Ctrl Pts',(42.6160676778573,40.0738031488471,45.3841051635958));
#36186=CARTESIAN_POINT('Ctrl Pts',(44.7169317511437,39.9475774064413,46.7665421380998));
#36187=CARTESIAN_POINT('Ctrl Pts',(44.6908130391648,39.8213516640354,49.2813144251639));
#36188=CARTESIAN_POINT('Ctrl Pts',(42.5616889640978,39.6951259216296,50.61981826));
#36189=CARTESIAN_POINT('Ctrl Pts',(40.284131667796,39.5689001792237,49.5532843388501));
#36190=CARTESIAN_POINT('Ctrl Pts',(39.9489775157664,39.4426744368179,47.0608089553651));
#36191=CARTESIAN_POINT('Ctrl Pts',(41.8639037244077,39.316448694412,45.4305269373203));
#36192=CARTESIAN_POINT('Ctrl Pts',(44.2709754392195,39.1902229520062,46.1590649271693));
#36193=CARTESIAN_POINT('Ctrl Pts',(44.9604598539699,39.0639972096003,48.5776126494022));
#36194=CARTESIAN_POINT('Ctrl Pts',(43.2993985398404,38.9377714671945,50.4659021276348));
#36195=CARTESIAN_POINT('Ctrl Pts',(40.8126740570015,38.8115457247886,50.0904514792801));
#36196=CARTESIAN_POINT('Ctrl Pts',(39.7831418085458,38.6853199823828,47.795930790271));
#36197=CARTESIAN_POINT('Ctrl Pts',(41.1559299227662,38.5590942399769,45.6887491093625));
#36198=CARTESIAN_POINT('Ctrl Pts',(43.6707955438592,38.432868497571,45.7033350870777));
#36199=CARTESIAN_POINT('Ctrl Pts',(45.0190492248093,38.3066427551652,47.8262985475982));
#36200=CARTESIAN_POINT('Ctrl Pts',(43.9629711371687,38.1804170127594,50.1087228980875));
#36201=CARTESIAN_POINT('Ctrl Pts',(41.4720589414524,38.0541912703535,50.4553037344496));
#36202=CARTESIAN_POINT('Ctrl Pts',(39.8330124324563,37.9279655279477,48.5478739495694));
#36203=CARTESIAN_POINT('Ctrl Pts',(40.5505042045122,37.8017397855418,46.1374865533334));
#36204=CARTESIAN_POINT('Ctrl Pts',(42.9658645980677,37.6755140431359,45.4369182039595));
#36205=CARTESIAN_POINT('Ctrl Pts',(44.8617516587178,37.5492883007301,47.0893025709156));
#36206=CARTESIAN_POINT('Ctrl Pts',(44.4977087938937,37.4230625583242,49.5777226792316));
#36207=CARTESIAN_POINT('Ctrl Pts',(42.2079335500693,37.2968368159184,50.6177665127646));
#36208=CARTESIAN_POINT('Ctrl Pts',(40.0944785765455,37.1706110735125,49.2546561291975));
#36209=CARTESIAN_POINT('Ctrl Pts',(40.0975315132471,37.0443853311067,46.7397500628646));
#36210=CARTESIAN_POINT('Ctrl Pts',(42.2142897123163,36.9181595887008,45.3817748901996));
#36211=CARTESIAN_POINT('Ctrl Pts',(44.5015331165518,36.791933846295,46.4273749345198));
#36212=CARTESIAN_POINT('Ctrl Pts',(44.8595333484911,36.6657081038891,48.9166715574299));
#36213=CARTESIAN_POINT('Ctrl Pts',(42.9596401015033,36.5394823614832,50.5644480874703));
#36214=CARTESIAN_POINT('Ctrl Pts',(40.5459877154068,36.4132566190774,49.8580176223918));
#36215=CARTESIAN_POINT('Ctrl Pts',(39.834350164686,36.2870308766715,47.4458953536611));
#36216=CARTESIAN_POINT('Ctrl Pts',(41.4780228340604,36.1608051342657,45.5424505819768));
#36217=CARTESIAN_POINT('Ctrl Pts',(43.9680862352258,36.0345793918598,45.89507800728));
#36218=CARTESIAN_POINT('Ctrl Pts',(45.0186197812332,35.908353649454,48.1800596508862));
#36219=CARTESIAN_POINT('Ctrl Pts',(43.6652157951609,35.7821279070482,50.2997434700879));
#36220=CARTESIAN_POINT('Ctrl Pts',(41.1503221732296,35.6559021646423,50.3082236386059));
#36221=CARTESIAN_POINT('Ctrl Pts',(39.782654067692,35.5296764222365,48.197715217391));
#36222=CARTESIAN_POINT('Ctrl Pts',(40.8177540792481,35.4034506798305,45.9057008612016));
#36223=CARTESIAN_POINT('Ctrl Pts',(43.3053827782721,35.2772249374248,45.5362887625874));
#36224=CARTESIAN_POINT('Ctrl Pts',(44.9618546758917,35.1509991950188,47.4286055160642));
#36225=CARTESIAN_POINT('Ctrl Pts',(44.2665003742732,35.0247734526131,49.8454721317606));
#36226=CARTESIAN_POINT('Ctrl Pts',(41.8576669585695,34.8985477102072,50.5681639178273));
#36227=CARTESIAN_POINT('Ctrl Pts',(39.9467045058711,34.7723219678014,48.9332375131001));
#36228=CARTESIAN_POINT('Ctrl Pts',(40.2879090763414,34.6460962253955,46.4415831865344));
#36229=CARTESIAN_POINT('Ctrl Pts',(42.5680490643027,34.5198704829896,45.3805820207381));
#36230=CARTESIAN_POINT('Ctrl Pts',(44.693917153644,34.3936447405838,46.7242511476396));
#36231=CARTESIAN_POINT('Ctrl Pts',(44.71393024428,34.2674189981779,49.2390794337307));
#36232=CARTESIAN_POINT('Ctrl Pts',(42.60971599535,34.1411932557721,50.616411713544));
#36233=CARTESIAN_POINT('Ctrl Pts',(40.3129788705228,34.0149675133662,49.591833495241));
#36234=CARTESIAN_POINT('Ctrl Pts',(39.932162711529,33.8887417709604,47.1059250522761));
#36235=CARTESIAN_POINT('Ctrl Pts',(41.8168631008729,33.7625160285545,45.4407925912651));
#36236=CARTESIAN_POINT('Ctrl Pts',(44.2368932660975,33.6362902861487,46.1250561697789));
#36237=CARTESIAN_POINT('Ctrl Pts',(44.9706237952432,33.5100645437428,48.5305499463878));
#36238=CARTESIAN_POINT('Ctrl Pts',(43.3444786223289,33.383838801337,50.4489901445125));
#36239=CARTESIAN_POINT('Ctrl Pts',(40.8512846102357,33.2576130589311,50.1192151019391));
#36240=CARTESIAN_POINT('Ctrl Pts',(39.7798404455423,33.1313873165252,47.8439657212142));
#36241=CARTESIAN_POINT('Ctrl Pts',(41.1137418680227,33.0051615741194,45.7119560833894));
#36242=CARTESIAN_POINT('Ctrl Pts',(43.6284610494873,32.8789358317135,45.6804144402365));
#36243=CARTESIAN_POINT('Ctrl Pts',(45.0154104091695,32.7527100893077,47.7782824144628));
#36244=CARTESIAN_POINT('Ctrl Pts',(44.0014115698186,32.6264843469018,50.0797096114633));
#36245=CARTESIAN_POINT('Ctrl Pts',(41.5172040205462,32.500258604496,50.4718908003069));
#36246=CARTESIAN_POINT('Ctrl Pts',(39.8435884357232,32.3740328620901,48.5949080807171));
#36247=CARTESIAN_POINT('Ctrl Pts',(40.5164637682265,32.2478071196843,46.1716426650325));
#36248=CARTESIAN_POINT('Ctrl Pts',(42.9191302650105,32.1215813772784,45.4271325348419));
#36249=CARTESIAN_POINT('Ctrl Pts',(44.8438875443106,31.9953556348726,47.0439778042436));
#36250=CARTESIAN_POINT('Ctrl Pts',(44.5277913464465,31.8691298924667,49.5396219858342));
#36251=CARTESIAN_POINT('Ctrl Pts',(42.2528398902663,31.7429041500609,50.6195711350613));
#36252=CARTESIAN_POINT('Ctrl Pts',(40.8354702907496,31.6587536551236,49.7392181843865));
#36253=CARTESIAN_POINT('Ctrl Pts',(40.470269204161,31.616678407655,49.0965015551825));
#36254=CARTESIAN_POINT('Ctrl Pts',(43.6976388151507,47.0576572027009,46.3839513684954));
#36255=CARTESIAN_POINT('Ctrl Pts',(44.2361172364869,47.0155648329742,46.8163047783));
#36256=CARTESIAN_POINT('Ctrl Pts',(44.8369087371464,46.9313972157789,48.2543647344542));
#36257=CARTESIAN_POINT('Ctrl Pts',(43.5022567528767,46.805154351115,50.1908495679857));
#36258=CARTESIAN_POINT('Ctrl Pts',(41.1545993598711,46.6789286087091,50.1104163679468));
#36259=CARTESIAN_POINT('Ctrl Pts',(39.9509061657975,46.5527028663033,48.0952246292301));
#36260=CARTESIAN_POINT('Ctrl Pts',(40.9951869305611,46.4264771238975,45.9912943929581));
#36261=CARTESIAN_POINT('Ctrl Pts',(43.3292790548416,46.3002513814916,45.7320538666771));
#36262=CARTESIAN_POINT('Ctrl Pts',(44.8101921436736,46.1740256390857,47.5544926412469));
#36263=CARTESIAN_POINT('Ctrl Pts',(44.078550600698,46.0477998966799,49.7860826899984));
#36264=CARTESIAN_POINT('Ctrl Pts',(41.8059495143702,45.921574154274,50.3779339506211));
#36265=CARTESIAN_POINT('Ctrl Pts',(40.0787077109787,45.7953484118682,48.7868438631224));
#36266=CARTESIAN_POINT('Ctrl Pts',(40.4824462952732,45.6691226694624,46.4733963398063));
#36267=CARTESIAN_POINT('Ctrl Pts',(42.6465345595011,45.5428969270565,45.5614077145981));
#36268=CARTESIAN_POINT('Ctrl Pts',(44.584298523753,45.4166711846506,46.8880829068769));
#36269=CARTESIAN_POINT('Ctrl Pts',(44.5168399562632,45.2904454422447,49.2355196381119));
#36270=CARTESIAN_POINT('Ctrl Pts',(42.5060859283947,45.1642196998389,50.4487269424059));
#36271=CARTESIAN_POINT('Ctrl Pts',(40.3979433879137,45.037993957433,49.413961921014));
#36272=CARTESIAN_POINT('Ctrl Pts',(40.1277228071566,44.9117682150272,47.081155441996));
#36273=CARTESIAN_POINT('Ctrl Pts',(41.9434914114395,44.7855424726214,45.5918640815856));
#36274=CARTESIAN_POINT('Ctrl Pts',(44.1783426481677,44.6593167302155,46.3132823967892));
#36275=CARTESIAN_POINT('Ctrl Pts',(44.7806450750023,44.5330909878097,48.5831362263346));
#36276=CARTESIAN_POINT('Ctrl Pts',(43.197474795122,44.4068652454038,50.3176610520595));
#36277=CARTESIAN_POINT('Ctrl Pts',(40.8822090819232,44.2806395029979,49.9245335930203));
#36278=CARTESIAN_POINT('Ctrl Pts',(39.9603012652077,44.1544137605921,47.7646515314772));
#36279=CARTESIAN_POINT('Ctrl Pts',(41.2780784151475,44.0281880181862,45.8208233728511));
#36280=CARTESIAN_POINT('Ctrl Pts',(43.6257986764382,43.9019622757804,45.8775164494406));
#36281=CARTESIAN_POINT('Ctrl Pts',(44.8482148879759,43.7757365333745,47.882685554068));
#36282=CARTESIAN_POINT('Ctrl Pts',(43.8231281599055,43.6495107909687,49.9955513165726));
#36283=CARTESIAN_POINT('Ctrl Pts',(41.4915855572742,43.5232850485628,50.2764670033147));
#36284=CARTESIAN_POINT('Ctrl Pts',(39.9939828756426,43.397059306157,48.4675472319794));
#36285=CARTESIAN_POINT('Ctrl Pts',(40.7051448682671,43.2708335637511,46.2294111433652));
#36286=CARTESIAN_POINT('Ctrl Pts',(42.9722127208382,43.1446078213453,45.6167057632439));
#36287=CARTESIAN_POINT('Ctrl Pts',(44.7139795557488,43.0183820789394,47.1919050597825));
#36288=CARTESIAN_POINT('Ctrl Pts',(44.3314737710161,42.8921563365336,49.5089492664443));
#36289=CARTESIAN_POINT('Ctrl Pts',(42.1758421878593,42.7659305941277,50.4407523618933));
#36290=CARTESIAN_POINT('Ctrl Pts',(40.2259912917555,42.6397048517219,49.1319032437917));
#36291=CARTESIAN_POINT('Ctrl Pts',(40.2719173947672,42.513479109316,46.7839476811689));
#36292=CARTESIAN_POINT('Ctrl Pts',(42.2714595525971,42.3872533669102,45.5523488462996));
#36293=CARTESIAN_POINT('Ctrl Pts',(44.3890040290975,42.2610276245043,46.5677354332865));
#36294=CARTESIAN_POINT('Ctrl Pts',(44.6806089510015,42.1348018820984,48.8979652718457));
#36295=CARTESIAN_POINT('Ctrl Pts',(42.8785760364404,42.0085761396926,50.4038477061108));
#36296=CARTESIAN_POINT('Ctrl Pts',(40.6372021743322,41.8823503972867,49.7029570290087));
#36297=CARTESIAN_POINT('Ctrl Pts',(40.0141067216971,41.7561246548809,47.4387228123483));
#36298=CARTESIAN_POINT('Ctrl Pts',(41.5813019100897,41.629898912475,45.6897506077468));
#36299=CARTESIAN_POINT('Ctrl Pts',(43.9000758805113,41.5036731700692,46.0616266692049));
#36300=CARTESIAN_POINT('Ctrl Pts',(44.841754659042,41.3774474276633,48.2129624424062));
#36301=CARTESIAN_POINT('Ctrl Pts',(43.5418610981805,41.2512216852575,50.1687950685326));
#36302=CARTESIAN_POINT('Ctrl Pts',(41.1937196129703,41.1249959428516,50.1336369055434));
#36303=CARTESIAN_POINT('Ctrl Pts',(39.9529640557869,40.9987702004458,48.139763745508));
#36304=CARTESIAN_POINT('Ctrl Pts',(40.9586291476786,40.87254445804,46.0175850881041));
#36305=CARTESIAN_POINT('Ctrl Pts',(43.2874972163334,40.746318715634,45.7152970635486));
#36306=CARTESIAN_POINT('Ctrl Pts',(44.8016277338369,40.6200929732283,47.5104052237872));
#36307=CARTESIAN_POINT('Ctrl Pts',(44.1110231123078,40.4938672308223,49.7549697222396));
#36308=CARTESIAN_POINT('Ctrl Pts',(41.8496701494549,40.3676414884165,50.3884421434123));
#36309=CARTESIAN_POINT('Ctrl Pts',(40.0935293568565,40.2414157460107,48.8292840220013));
#36310=CARTESIAN_POINT('Ctrl Pts',(40.4547678743152,40.1151900036048,46.508829052713));
#36311=CARTESIAN_POINT('Ctrl Pts',(42.6017625939728,39.988964261199,45.55729439504));
#36312=CARTESIAN_POINT('Ctrl Pts',(44.563535818056,39.8627385187931,46.8482050612988));
#36313=CARTESIAN_POINT('Ctrl Pts',(44.5391463344816,39.7365127763873,49.1964830865931));
#36314=CARTESIAN_POINT('Ctrl Pts',(42.5509841043168,39.6102870339814,50.4463692724266));
#36315=CARTESIAN_POINT('Ctrl Pts',(40.4242158964095,39.4840612915755,49.4504468252328));
#36316=CARTESIAN_POINT('Ctrl Pts',(40.1112511264596,39.3578355491697,47.1229895036563));
#36317=CARTESIAN_POINT('Ctrl Pts',(41.8993967804196,39.2316098067638,45.6006427457807));
#36318=CARTESIAN_POINT('Ctrl Pts',(44.1471047109853,39.105384064358,46.2809467880016));
#36319=CARTESIAN_POINT('Ctrl Pts',(44.7909407784774,38.9791583219522,48.5393709397469));
#36320=CARTESIAN_POINT('Ctrl Pts',(43.2398525138651,38.8529325795463,50.3026433878879));
#36321=CARTESIAN_POINT('Ctrl Pts',(40.917765345953,38.7267068371405,49.9520500114421));
#36322=CARTESIAN_POINT('Ctrl Pts',(39.9563948203524,38.6004810947346,47.8094414976215));
#36323=CARTESIAN_POINT('Ctrl Pts',(41.2382954435587,38.4742553523287,45.8417689325808));
#36324=CARTESIAN_POINT('Ctrl Pts',(43.5866606235631,38.3480296099229,45.8553892238186));
#36325=CARTESIAN_POINT('Ctrl Pts',(44.8456511523612,38.2218038675171,47.8377987121399));
#36326=CARTESIAN_POINT('Ctrl Pts',(43.8594922945758,38.0955781251112,49.9691117436304));
#36327=CARTESIAN_POINT('Ctrl Pts',(41.5334946675828,37.9693523827053,50.2927466771805));
#36328=CARTESIAN_POINT('Ctrl Pts',(40.0029636849925,37.8431266402995,48.5116011350304));
#36329=CARTESIAN_POINT('Ctrl Pts',(40.6729528407962,37.7169008978936,46.2607970426901));
#36330=CARTESIAN_POINT('Ctrl Pts',(42.9284006857281,37.5906751554878,45.6066108690497));
#36331=CARTESIAN_POINT('Ctrl Pts',(44.6987677069752,37.4644494130819,47.1495966567582));
#36332=CARTESIAN_POINT('Ctrl Pts',(44.3588268446837,37.3382236706761,49.4732671887257));
#36333=CARTESIAN_POINT('Ctrl Pts',(42.2206495967492,37.2119979282702,50.4444533641866));
#36334=CARTESIAN_POINT('Ctrl Pts',(40.2471190718168,37.0857721858644,49.1715897429963));
#36335=CARTESIAN_POINT('Ctrl Pts',(40.2499698842764,36.9595464434585,46.8231867954894));
#36336=CARTESIAN_POINT('Ctrl Pts',(42.2265849397648,36.8333207010527,45.5551184008806));
#36337=CARTESIAN_POINT('Ctrl Pts',(44.3623979723383,36.7070949586468,46.5314929298803));
#36338=CARTESIAN_POINT('Ctrl Pts',(44.6966962632961,36.5808692162409,48.855981945482));
#36339=CARTESIAN_POINT('Ctrl Pts',(42.9225882912717,36.4546434738351,50.3946649650118));
#36340=CARTESIAN_POINT('Ctrl Pts',(40.6687353726094,36.3284177314293,49.7350047858075));
#36341=CARTESIAN_POINT('Ctrl Pts',(40.0042128506585,36.2021919890234,47.482580680802));
#36342=CARTESIAN_POINT('Ctrl Pts',(41.5390637117578,36.0759662466176,45.7051563180868));
#36343=CARTESIAN_POINT('Ctrl Pts',(43.8642687399131,35.9497405042117,46.0344375171106));
#36344=CARTESIAN_POINT('Ctrl Pts',(44.8452501407396,35.8235147618058,48.1681385323011));
#36345=CARTESIAN_POINT('Ctrl Pts',(43.5814502904756,35.6972890194,50.1474855128642));
#36346=CARTESIAN_POINT('Ctrl Pts',(41.2330589634704,35.5710632769941,50.1554042391373));
#36347=CARTESIAN_POINT('Ctrl Pts',(39.9559393711116,35.4448375345883,48.1846251856098));
#36348=CARTESIAN_POINT('Ctrl Pts',(40.9225090377262,35.3186117921824,46.0443570690945));
#36349=CARTESIAN_POINT('Ctrl Pts',(43.2454405568381,35.1923860497766,45.6994024511693));
#36350=CARTESIAN_POINT('Ctrl Pts',(44.7922432541268,35.0661603073707,47.4664355427714));
#36351=CARTESIAN_POINT('Ctrl Pts',(44.1429259244093,34.9399345649648,49.7232898881538));
#36352=CARTESIAN_POINT('Ctrl Pts',(41.893572928995,34.813708822559,50.3981347832605));
#36353=CARTESIAN_POINT('Ctrl Pts',(40.1091286045852,34.6874830801532,48.8714511272717));
#36354=CARTESIAN_POINT('Ctrl Pts',(40.4277432159704,34.5612573377473,46.5447605033124));
#36355=CARTESIAN_POINT('Ctrl Pts',(42.5569231245721,34.4350315953415,45.5540045071265));
#36356=CARTESIAN_POINT('Ctrl Pts',(44.5420449364172,34.3088058529356,46.8087140091359));
#36357=CARTESIAN_POINT('Ctrl Pts',(44.5607330304451,34.1825801105298,49.1570443259581));
#36358=CARTESIAN_POINT('Ctrl Pts',(42.5958314341089,34.0563543681239,50.4431882614755));
#36359=CARTESIAN_POINT('Ctrl Pts',(40.4511532269197,33.930128625718,49.486443777049));
#36360=CARTESIAN_POINT('Ctrl Pts',(40.0955495714944,33.8039028833122,47.1651186218703));
#36361=CARTESIAN_POINT('Ctrl Pts',(41.8554705517465,33.6776771409063,45.610228746747));
#36362=CARTESIAN_POINT('Ctrl Pts',(44.1152789991272,33.5514513985005,46.2491896312768));
#36363=CARTESIAN_POINT('Ctrl Pts',(44.8004318008118,33.4252256560946,48.495424093399));
#36364=CARTESIAN_POINT('Ctrl Pts',(43.2819480020455,33.2989999136888,50.2868510879112));
#36365=CARTESIAN_POINT('Ctrl Pts',(40.9538196297428,33.1727741712829,49.9789092954279));
#36366=CARTESIAN_POINT('Ctrl Pts',(39.9533120290261,33.0465484288771,47.8542962040937));
#36367=CARTESIAN_POINT('Ctrl Pts',(41.1989005120996,32.9203226864712,45.863439454171));
#36368=CARTESIAN_POINT('Ctrl Pts',(43.5471289477304,32.7940969440654,45.8339860726943));
#36369=CARTESIAN_POINT('Ctrl Pts',(44.8422532499551,32.6678712016595,47.7929615589386));
#36370=CARTESIAN_POINT('Ctrl Pts',(43.8953877208691,32.5416454592536,49.9420193250558));
#36371=CARTESIAN_POINT('Ctrl Pts',(41.5756508491709,32.4154197168479,50.3082355715256));
#36372=CARTESIAN_POINT('Ctrl Pts',(40.0128394881397,32.2891939744419,48.555521301155));
#36373=CARTESIAN_POINT('Ctrl Pts',(40.6411661025247,32.1629682320361,46.2926917979112));
#36374=CARTESIAN_POINT('Ctrl Pts',(42.884760469113,32.0367424896302,45.5974730747969));
#36375=CARTESIAN_POINT('Ctrl Pts',(44.68208631299,31.9105167472244,47.1072726840769));
#36376=CARTESIAN_POINT('Ctrl Pts',(44.3869177368363,31.7842910048185,49.4376890087395));
#36377=CARTESIAN_POINT('Ctrl Pts',(42.2625828455065,31.6580652624127,50.4461385087641));
#36378=CARTESIAN_POINT('Ctrl Pts',(40.939052320939,31.5739147674755,49.6240706423386));
#36379=CARTESIAN_POINT('Ctrl Pts',(40.5980299186877,31.5318395200069,49.0239060291786));
#36380=CARTESIAN_POINT('Ctrl Pts',(43.6056354772814,46.9728183150527,46.4985301453641));
#36381=CARTESIAN_POINT('Ctrl Pts',(44.1059354690308,46.930725945326,46.9002294498996));
#36382=CARTESIAN_POINT('Ctrl Pts',(44.6641305069622,46.8465583281308,48.2363301285741));
#36383=CARTESIAN_POINT('Ctrl Pts',(43.4241061155271,46.7203154634668,50.0355170743283));
#36384=CARTESIAN_POINT('Ctrl Pts',(41.242898981105,46.594089721061,49.9607866344046));
#36385=CARTESIAN_POINT('Ctrl Pts',(40.124548326367,46.4678639786551,48.0884731482832));
#36386=CARTESIAN_POINT('Ctrl Pts',(41.0947889846625,46.3416382362493,46.1337127750893));
#36387=CARTESIAN_POINT('Ctrl Pts',(43.2633926357093,46.2154124938433,45.8928525511316));
#36388=CARTESIAN_POINT('Ctrl Pts',(44.6393081353231,46.0891867514376,47.5860793690575));
#36389=CARTESIAN_POINT('Ctrl Pts',(43.9595403982877,45.9629610090316,49.6594484006477));
#36390=CARTESIAN_POINT('Ctrl Pts',(41.8480680352578,45.8367352666259,50.2093370666999));
#36391=CARTESIAN_POINT('Ctrl Pts',(40.2432886685352,45.71050952422,48.7310561809538));
#36392=CARTESIAN_POINT('Ctrl Pts',(40.6184019551368,45.5842837818142,46.5816334167968));
#36393=CARTESIAN_POINT('Ctrl Pts',(42.6290551175259,45.4580580394083,45.7343053093214));
#36394=CARTESIAN_POINT('Ctrl Pts',(44.4294305028971,45.3318322970025,46.9669184679027));
#36395=CARTESIAN_POINT('Ctrl Pts',(44.3667547866172,45.2056065545965,49.1479205856004));
#36396=CARTESIAN_POINT('Ctrl Pts',(42.4985643750939,45.0793808121907,50.2751107946758));
#36397=CARTESIAN_POINT('Ctrl Pts',(40.5398903524809,44.9531550697849,49.3137112080772));
#36398=CARTESIAN_POINT('Ctrl Pts',(40.2888285662205,44.826929327379,47.1463020493048));
#36399=CARTESIAN_POINT('Ctrl Pts',(41.9758581327668,44.7007035849732,45.7626023023833));
#36400=CARTESIAN_POINT('Ctrl Pts',(44.0522571322319,44.5744778425673,46.4328716443721));
#36401=CARTESIAN_POINT('Ctrl Pts',(44.6118559708041,44.4482521001614,48.5417915327042));
#36402=CARTESIAN_POINT('Ctrl Pts',(43.1409333737641,44.3220263577557,50.1533375512908));
#36403=CARTESIAN_POINT('Ctrl Pts',(40.9898213304319,44.1958006153497,49.7880830550646));
#36404=CARTESIAN_POINT('Ctrl Pts',(40.1332773078288,44.0695748729439,47.7813378731723));
#36405=CARTESIAN_POINT('Ctrl Pts',(41.3576233003874,43.9433491305381,45.9753282482937));
#36406=CARTESIAN_POINT('Ctrl Pts',(43.538888845697,43.8171233881322,46.0280017531661));
#36407=CARTESIAN_POINT('Ctrl Pts',(44.6746350451991,43.6908976457263,47.8910032157163));
#36408=CARTESIAN_POINT('Ctrl Pts',(43.7222275553626,43.5646719033205,49.8540655811966));
#36409=CARTESIAN_POINT('Ctrl Pts',(41.5559926634146,43.4384461609146,50.1150641842801));
#36410=CARTESIAN_POINT('Ctrl Pts',(40.1645708727237,43.3122204185088,48.4343978644888));
#36411=CARTESIAN_POINT('Ctrl Pts',(40.8253110712996,43.1859946761029,46.3549469110244));
#36412=CARTESIAN_POINT('Ctrl Pts',(42.9316425100263,43.0597689336971,45.7856826945333));
#36413=CARTESIAN_POINT('Ctrl Pts',(44.5499170751846,42.9335431912913,47.2491994555321));
#36414=CARTESIAN_POINT('Ctrl Pts',(44.1945311704516,42.8073174488854,49.4019638961184));
#36415=CARTESIAN_POINT('Ctrl Pts',(42.1917351055846,42.6810917064796,50.2677016165051));
#36416=CARTESIAN_POINT('Ctrl Pts',(40.3801297587773,42.5548659640736,49.0516506531956));
#36417=CARTESIAN_POINT('Ctrl Pts',(40.4227996746874,42.4286402216679,46.8701664895536));
#36418=CARTESIAN_POINT('Ctrl Pts',(42.2805731442023,42.3024144792619,45.7258887199923));
#36419=CARTESIAN_POINT('Ctrl Pts',(44.2479825001668,42.1761887368562,46.6692838143236));
#36420=CARTESIAN_POINT('Ctrl Pts',(44.5189124654952,42.0499629944503,48.8342990179267));
#36421=CARTESIAN_POINT('Ctrl Pts',(42.8446447203741,41.9237372520444,50.2334135220303));
#36422=CARTESIAN_POINT('Ctrl Pts',(40.7621855534177,41.7975115096386,49.5822163968025));
#36423=CARTESIAN_POINT('Ctrl Pts',(40.183267926526,41.6712857672327,47.4785176875716));
#36424=CARTESIAN_POINT('Ctrl Pts',(41.6393480752472,41.5450600248269,45.8535486175751));
#36425=CARTESIAN_POINT('Ctrl Pts',(43.7937196383484,41.418834282421,46.1990584525238));
#36426=CARTESIAN_POINT('Ctrl Pts',(44.66863285021,41.2926085400152,48.19786328283));
#36427=CARTESIAN_POINT('Ctrl Pts',(43.4609024899845,41.1663827976093,50.0150262515631));
#36428=CARTESIAN_POINT('Ctrl Pts',(41.2792455857734,41.0401570552035,49.9823608225385));
#36429=CARTESIAN_POINT('Ctrl Pts',(40.1264603107733,40.9139313127976,48.1298544156162));
#36430=CARTESIAN_POINT('Ctrl Pts',(41.0608231695995,40.7877055703918,46.1581394448378));
#36431=CARTESIAN_POINT('Ctrl Pts',(43.2245731535674,40.6614798279859,45.8772838149767));
#36432=CARTESIAN_POINT('Ctrl Pts',(44.6313509470666,40.5352540855801,47.5451177748369));
#36433=CARTESIAN_POINT('Ctrl Pts',(43.9897105901593,40.4090283431742,49.6305413601867));
#36434=CARTESIAN_POINT('Ctrl Pts',(41.8886888521848,40.2828026007683,50.2191002225822));
#36435=CARTESIAN_POINT('Ctrl Pts',(40.257059451201,40.1565768583625,48.7704873081738));
#36436=CARTESIAN_POINT('Ctrl Pts',(40.592685950134,40.0303511159566,46.6145539299918));
#36437=CARTESIAN_POINT('Ctrl Pts',(42.5874575100881,39.9041253735508,45.7304836264844));
#36438=CARTESIAN_POINT('Ctrl Pts',(44.4101398849683,39.777899631145,46.9298679844975));
#36439=CARTESIAN_POINT('Ctrl Pts',(44.3874796297982,39.6516738887391,49.1116517480225));
#36440=CARTESIAN_POINT('Ctrl Pts',(42.5402792445361,39.5254481463332,50.272920284853));
#36441=CARTESIAN_POINT('Ctrl Pts',(40.5643001250229,39.3992224039274,49.3476093116157));
#36442=CARTESIAN_POINT('Ctrl Pts',(40.2735247371529,39.2729966615215,47.1851700519474));
#36443=CARTESIAN_POINT('Ctrl Pts',(41.9348898364317,39.1467709191157,45.770758554241));
#36444=CARTESIAN_POINT('Ctrl Pts',(44.0232339827512,39.0205451767098,46.4028286488339));
#36445=CARTESIAN_POINT('Ctrl Pts',(44.6214217029848,38.894319434304,48.5011292300917));
#36446=CARTESIAN_POINT('Ctrl Pts',(43.18030648789,38.7680936918981,50.1393846481409));
#36447=CARTESIAN_POINT('Ctrl Pts',(41.0228566349045,38.6418679494923,49.8136485436042));
#36448=CARTESIAN_POINT('Ctrl Pts',(40.1296478321591,38.5156422070864,47.822952204972));
#36449=CARTESIAN_POINT('Ctrl Pts',(41.3206609643514,38.3894164646805,45.9947887557993));
#36450=CARTESIAN_POINT('Ctrl Pts',(43.502525703267,38.2631907222747,46.0074433605592));
#36451=CARTESIAN_POINT('Ctrl Pts',(44.6722530799132,38.1369649798688,47.8492988766815));
#36452=CARTESIAN_POINT('Ctrl Pts',(43.7560134519829,38.010739237463,49.8295005891734));
#36453=CARTESIAN_POINT('Ctrl Pts',(41.5949303937134,37.8845134950571,50.1301896199112));
#36454=CARTESIAN_POINT('Ctrl Pts',(40.1729149375288,37.7582877526513,48.4753283204915));
#36455=CARTESIAN_POINT('Ctrl Pts',(40.7954014770801,37.6320620102454,46.3841075320469));
#36456=CARTESIAN_POINT('Ctrl Pts',(42.8909367733884,37.5058362678396,45.7763035341399));
#36457=CARTESIAN_POINT('Ctrl Pts',(44.5357837552328,37.3796105254338,47.2098907426008));
#36458=CARTESIAN_POINT('Ctrl Pts',(44.2199448954737,37.2533847830279,49.3688116982201));
#36459=CARTESIAN_POINT('Ctrl Pts',(42.2333656434293,37.127159040622,50.2711402156085));
#36460=CARTESIAN_POINT('Ctrl Pts',(40.3997595670881,37.0009332982162,49.0885233567951));
#36461=CARTESIAN_POINT('Ctrl Pts',(40.4024082553057,36.8747075558104,46.9066235281145));
#36462=CARTESIAN_POINT('Ctrl Pts',(42.2388801672136,36.7484818134045,45.7284619115615));
#36463=CARTESIAN_POINT('Ctrl Pts',(44.2232628281249,36.6222560709986,46.6356109252409));
#36464=CARTESIAN_POINT('Ctrl Pts',(44.5338591781011,36.4960303285928,48.795292333534));
#36465=CARTESIAN_POINT('Ctrl Pts',(42.8855364810398,36.3698045861869,50.2248818425534));
#36466=CARTESIAN_POINT('Ctrl Pts',(40.7914830298119,36.2435788437811,49.6119919492234));
#36467=CARTESIAN_POINT('Ctrl Pts',(40.1740755366309,36.1173531013752,47.5192660079426));
#36468=CARTESIAN_POINT('Ctrl Pts',(41.6001045894553,35.9911273589694,45.8678620541969));
#36469=CARTESIAN_POINT('Ctrl Pts',(43.7604512446002,35.8649016165635,46.1737970269411));
#36470=CARTESIAN_POINT('Ctrl Pts',(44.671880500246,35.7386758741577,48.1562174137159));
#36471=CARTESIAN_POINT('Ctrl Pts',(43.4976847857903,35.6124501317518,49.9952275556402));
#36472=CARTESIAN_POINT('Ctrl Pts',(41.315795753711,35.486224389346,50.0025848396691));
#36473=CARTESIAN_POINT('Ctrl Pts',(40.1292246745312,35.3599986469401,48.1715351538286));
#36474=CARTESIAN_POINT('Ctrl Pts',(41.0272639962045,35.2337729045342,46.1830132769877));
#36475=CARTESIAN_POINT('Ctrl Pts',(43.185498335404,35.1075471621284,45.862516139751));
#36476=CARTESIAN_POINT('Ctrl Pts',(44.6226318323623,34.9813214197226,47.5042655694787));
#36477=CARTESIAN_POINT('Ctrl Pts',(44.0193514745451,34.8550956773167,49.6011076445469));
#36478=CARTESIAN_POINT('Ctrl Pts',(41.9294788994206,34.7288699349108,50.2281056486939));
#36479=CARTESIAN_POINT('Ctrl Pts',(40.2715527032993,34.602644192505,48.8096647414431));
#36480=CARTESIAN_POINT('Ctrl Pts',(40.5675773555997,34.4764184500991,46.6479378200906));
#36481=CARTESIAN_POINT('Ctrl Pts',(42.5457971848414,34.3501927076933,45.7274269935147));
#36482=CARTESIAN_POINT('Ctrl Pts',(44.3901727191906,34.2239669652874,46.8931768706323));
#36483=CARTESIAN_POINT('Ctrl Pts',(44.4075358166101,34.0977412228816,49.0750092181854));
#36484=CARTESIAN_POINT('Ctrl Pts',(42.5819468728678,33.9715154804757,50.2699648094069));
#36485=CARTESIAN_POINT('Ctrl Pts',(40.5893275833166,33.8452897380698,49.3810540588572));
#36486=CARTESIAN_POINT('Ctrl Pts',(40.2589364314598,33.719063995664,47.2243121914646));
#36487=CARTESIAN_POINT('Ctrl Pts',(41.89407800262,33.5928382532582,45.7796649022288));
#36488=CARTESIAN_POINT('Ctrl Pts',(43.993664732157,33.4666125108523,46.3733230927746));
#36489=CARTESIAN_POINT('Ctrl Pts',(44.6302398063803,33.3403867684465,48.4602982404102));
#36490=CARTESIAN_POINT('Ctrl Pts',(43.2194173817619,33.2141610260406,50.12471203131));
#36491=CARTESIAN_POINT('Ctrl Pts',(41.0563546492499,33.0879352836347,49.8386034889169));
#36492=CARTESIAN_POINT('Ctrl Pts',(40.1267836125097,32.9617095412289,47.8646266869731));
#36493=CARTESIAN_POINT('Ctrl Pts',(41.2840591561766,32.835483798823,46.0149228249524));
#36494=CARTESIAN_POINT('Ctrl Pts',(43.4657968459734,32.7092580564172,45.9875577051523));
#36495=CARTESIAN_POINT('Ctrl Pts',(44.6690960907408,32.5830323140114,47.8076407034142));
#36496=CARTESIAN_POINT('Ctrl Pts',(43.7893638719195,32.4568065716055,49.8043290386482));
#36497=CARTESIAN_POINT('Ctrl Pts',(41.6340976777956,32.3305808291997,50.1445803427444));
#36498=CARTESIAN_POINT('Ctrl Pts',(40.1820905405563,32.2043550867938,48.5161345215927));
#36499=CARTESIAN_POINT('Ctrl Pts',(40.765868436823,32.078129344388,46.4137409307898));
#36500=CARTESIAN_POINT('Ctrl Pts',(42.8503906732154,31.951903601982,45.7678136147519));
#36501=CARTESIAN_POINT('Ctrl Pts',(44.5202850816693,31.8256778595762,47.1705675639103));
#36502=CARTESIAN_POINT('Ctrl Pts',(44.2460441272262,31.6994521171704,49.3357560316449));
#36503=CARTESIAN_POINT('Ctrl Pts',(42.2723258007466,31.5732263747646,50.2727058824669));
#36504=CARTESIAN_POINT('Ctrl Pts',(41.0426343511285,31.4890758798273,49.5089231002906));
#36505=CARTESIAN_POINT('Ctrl Pts',(40.7257906332145,31.4470006323587,48.9513105031748));
#36506=CARTESIAN_POINT('Ctrl Pts',(43.4903488624466,46.9748,50.0969334274272));
#36507=CARTESIAN_POINT('Ctrl Pts',(43.5035273931069,46.9748,50.0899215423449));
#36508=CARTESIAN_POINT('Ctrl Pts',(43.5167059237672,46.9748,50.0829096572625));
#36509=CARTESIAN_POINT('Ctrl Pts',(43.5298844544276,46.9748,50.0758977721803));
#36510=CARTESIAN_POINT('Origin',(42.4,46.9748,48.));
#36511=CARTESIAN_POINT('',(42.4,47.1748,45.43653));
#36512=CARTESIAN_POINT('Origin',(42.4,47.1748,48.));
#36513=CARTESIAN_POINT('Origin',(42.4,46.9748,45.43653));
#36514=CARTESIAN_POINT('Origin',(42.4,47.1748,48.));
#36515=CARTESIAN_POINT('',(38.4376,47.1748,48.));
#36516=CARTESIAN_POINT('Origin',(42.4,47.1748,48.));
#36517=CARTESIAN_POINT('Origin',(42.4,31.4998,48.));
#36518=CARTESIAN_POINT('',(40.43653,31.2998,48.));
#36519=CARTESIAN_POINT('',(40.23653,31.4998,48.));
#36520=CARTESIAN_POINT('Origin',(42.4,31.2998,48.));
#36521=CARTESIAN_POINT('Origin',(42.4,31.2998,48.));
#36522=CARTESIAN_POINT('Origin',(46.6323742019726,52.0008,47.4568035581149));
#36523=CARTESIAN_POINT('',(46.3131875668744,47.7748,47.3774433146613));
#36524=CARTESIAN_POINT('',(46.3131875668744,51.6008,47.3774433146613));
#36525=CARTESIAN_POINT('',(46.3131875668744,47.1748,47.3774433146613));
#36526=CARTESIAN_POINT('',(46.1544810775837,47.7748,47.3379836874626));
#36527=CARTESIAN_POINT('',(46.6323742019726,47.7748,47.4568035581149));
#36528=CARTESIAN_POINT('',(46.1544810775837,51.7508,47.3379836874626));
#36529=CARTESIAN_POINT('',(46.1544810775837,52.0008,47.3379836874626));
#36530=CARTESIAN_POINT('Ctrl Pts',(46.3131875668744,51.6008,47.3774433146613));
#36531=CARTESIAN_POINT('Ctrl Pts',(46.2323033520825,51.6775199678396,47.3573328517797));
#36532=CARTESIAN_POINT('Ctrl Pts',(46.1544810775837,51.7508,47.3379836874626));
#36533=CARTESIAN_POINT('Origin',(46.1544810775837,52.0008,47.3379836874626));
#36534=CARTESIAN_POINT('',(46.2901204070909,51.6008,47.2466229507511));
#36535=CARTESIAN_POINT('',(46.2901204070909,47.7748,47.2466229507511));
#36536=CARTESIAN_POINT('',(46.2901204070909,47.1748,47.2466229507511));
#36537=CARTESIAN_POINT('Ctrl Pts',(46.1544810775837,51.7508,47.3379836874626));
#36538=CARTESIAN_POINT('Ctrl Pts',(46.2209922907101,51.6775199678396,47.2931846350574));
#36539=CARTESIAN_POINT('Ctrl Pts',(46.2901204070909,51.6008,47.2466229507511));
#36540=CARTESIAN_POINT('',(46.1544810775837,47.7748,47.3379836874626));
#36541=CARTESIAN_POINT('Origin',(46.3760628220115,47.7748,47.2989128474875));
#36542=CARTESIAN_POINT('Origin',(42.4,47.7748,48.));
#36543=CARTESIAN_POINT('Origin',(42.4,51.8008,48.));
#36544=CARTESIAN_POINT('',(38.5876,51.7508,48.));
#36545=CARTESIAN_POINT('',(38.4381567112477,51.6008,48.0664192394455));
#36546=CARTESIAN_POINT('Ctrl Pts',(38.5876,51.7508,48.));
#36547=CARTESIAN_POINT('Ctrl Pts',(38.5143199678398,51.6775199678398,48.0325689031823));
#36548=CARTESIAN_POINT('Ctrl Pts',(38.4381567112477,51.6008,48.0664192394454));
#36549=CARTESIAN_POINT('',(38.4868124331256,51.6008,48.6225566853387));
#36550=CARTESIAN_POINT('Origin',(42.4,51.6008,48.));
#36551=CARTESIAN_POINT('',(38.6455189224163,51.7508,48.6620163125374));
#36552=CARTESIAN_POINT('Ctrl Pts',(38.4868124331256,51.6008,48.6225566853387));
#36553=CARTESIAN_POINT('Ctrl Pts',(38.5676966479175,51.6775199678396,48.6426671482203));
#36554=CARTESIAN_POINT('Ctrl Pts',(38.6455189224163,51.7508,48.6620163125374));
#36555=CARTESIAN_POINT('',(38.5098795929091,51.6008,48.7533770492488));
#36556=CARTESIAN_POINT('Ctrl Pts',(38.6455189224163,51.7508,48.6620163125374));
#36557=CARTESIAN_POINT('Ctrl Pts',(38.5790077092897,51.6775199678393,48.7068153649427));
#36558=CARTESIAN_POINT('Ctrl Pts',(38.5098795929091,51.6008,48.7533770492488));
#36559=CARTESIAN_POINT('',(38.6543683790546,51.6008,49.2926165402678));
#36560=CARTESIAN_POINT('Origin',(42.4,51.6008,48.));
#36561=CARTESIAN_POINT('',(38.8175158525158,51.7508,49.3039175944148));
#36562=CARTESIAN_POINT('Ctrl Pts',(38.6543683790546,51.6008,49.2926165402678));
#36563=CARTESIAN_POINT('Ctrl Pts',(38.7375159261089,51.6775199678392,49.2983760835296));
#36564=CARTESIAN_POINT('Ctrl Pts',(38.8175158525158,51.7508,49.3039175944148));
#36565=CARTESIAN_POINT('',(38.699801814644,51.6008,49.417443878638));
#36566=CARTESIAN_POINT('Ctrl Pts',(38.8175158525158,51.7508,49.3039175944148));
#36567=CARTESIAN_POINT('Ctrl Pts',(38.7597943679781,51.6775199678396,49.3595855995048));
#36568=CARTESIAN_POINT('Ctrl Pts',(38.699801814644,51.6008,49.417443878638));
#36569=CARTESIAN_POINT('',(38.9357334464049,51.6008,49.9234008957163));
#36570=CARTESIAN_POINT('Origin',(42.4,51.6008,48.));
#36571=CARTESIAN_POINT('',(39.0983647506122,51.7508,49.9062));
#36572=CARTESIAN_POINT('Ctrl Pts',(38.9357334464049,51.6008,49.9234008957163));
#36573=CARTESIAN_POINT('Ctrl Pts',(39.0186179295798,51.6775199678394,49.9146345185509));
#36574=CARTESIAN_POINT('Ctrl Pts',(39.0983647506122,51.7508,49.9062));
#36575=CARTESIAN_POINT('',(39.0021526858504,51.6008,50.038442393036));
#36576=CARTESIAN_POINT('Ctrl Pts',(39.0983647506122,51.7508,49.9062));
#36577=CARTESIAN_POINT('Ctrl Pts',(39.051186832762,51.677519967839,49.9710455136101));
#36578=CARTESIAN_POINT('Ctrl Pts',(39.0021526858504,51.6008,50.038442393036));
#36579=CARTESIAN_POINT('',(39.3223584999828,51.6008,50.4957436882364));
#36580=CARTESIAN_POINT('Origin',(42.4,51.6008,48.));
#36581=CARTESIAN_POINT('',(39.4795321650532,51.7508,50.450563483169));
#36582=CARTESIAN_POINT('Ctrl Pts',(39.3223584999828,51.6008,50.4957436882363));
#36583=CARTESIAN_POINT('Ctrl Pts',(39.4024615161986,51.6775199678397,50.4727177525777));
#36584=CARTESIAN_POINT('Ctrl Pts',(39.4795321650532,51.7508,50.450563483169));
#36585=CARTESIAN_POINT('',(39.4077454283035,51.6008,50.5975038668231));
#36586=CARTESIAN_POINT('Ctrl Pts',(39.4795321650532,51.7508,50.450563483169));
#36587=CARTESIAN_POINT('Ctrl Pts',(39.4443312910517,51.6775199678393,50.5226162071808));
#36588=CARTESIAN_POINT('Ctrl Pts',(39.4077454283035,51.6008,50.5975038668231));
#36589=CARTESIAN_POINT('',(39.8024961331769,51.6008,50.9922545716966));
#36590=CARTESIAN_POINT('Origin',(42.4,51.6008,48.));
#36591=CARTESIAN_POINT('',(39.949436516831,51.7508,50.9204678349468));
#36592=CARTESIAN_POINT('Ctrl Pts',(39.8024961331769,51.6008,50.9922545716966));
#36593=CARTESIAN_POINT('Ctrl Pts',(39.8773837928195,51.6775199678396,50.9556687089481));
#36594=CARTESIAN_POINT('Ctrl Pts',(39.949436516831,51.7508,50.9204678349468));
#36595=CARTESIAN_POINT('',(39.9042563117637,51.6008,51.0776415000173));
#36596=CARTESIAN_POINT('Ctrl Pts',(39.949436516831,51.7508,50.9204678349468));
#36597=CARTESIAN_POINT('Ctrl Pts',(39.9272822474223,51.6775199678397,50.9975384838015));
#36598=CARTESIAN_POINT('Ctrl Pts',(39.9042563117637,51.6008,51.0776415000173));
#36599=CARTESIAN_POINT('',(40.3615576069641,51.6008,51.3978473141496));
#36600=CARTESIAN_POINT('Origin',(42.4,51.6008,48.));
#36601=CARTESIAN_POINT('',(40.4938,51.7508,51.3016352493878));
#36602=CARTESIAN_POINT('Ctrl Pts',(40.3615576069641,51.6008,51.3978473141496));
#36603=CARTESIAN_POINT('Ctrl Pts',(40.4289544863899,51.677519967839,51.348813167238));
#36604=CARTESIAN_POINT('Ctrl Pts',(40.4938,51.7508,51.3016352493878));
#36605=CARTESIAN_POINT('',(40.4765991042837,51.6008,51.4642665535951));
#36606=CARTESIAN_POINT('Ctrl Pts',(40.4938,51.7508,51.3016352493878));
#36607=CARTESIAN_POINT('Ctrl Pts',(40.4853654814492,51.6775199678399,51.3813820704198));
#36608=CARTESIAN_POINT('Ctrl Pts',(40.4765991042837,51.6008,51.4642665535951));
#36609=CARTESIAN_POINT('',(40.982556121362,51.6008,51.700198185356));
#36610=CARTESIAN_POINT('Origin',(42.4,51.6008,48.));
#36611=CARTESIAN_POINT('',(41.0960824055852,51.7508,51.5824841474842));
#36612=CARTESIAN_POINT('Ctrl Pts',(40.982556121362,51.6008,51.700198185356));
#36613=CARTESIAN_POINT('Ctrl Pts',(41.040414400495,51.6775199678393,51.6402056320221));
#36614=CARTESIAN_POINT('Ctrl Pts',(41.0960824055852,51.7508,51.5824841474842));
#36615=CARTESIAN_POINT('',(41.1073834597322,51.6008,51.7456316209454));
#36616=CARTESIAN_POINT('Ctrl Pts',(41.0960824055852,51.7508,51.5824841474842));
#36617=CARTESIAN_POINT('Ctrl Pts',(41.1016239164704,51.6775199678393,51.662484073891));
#36618=CARTESIAN_POINT('Ctrl Pts',(41.1073834597322,51.6008,51.7456316209454));
#36619=CARTESIAN_POINT('',(41.6466229507512,51.6008,51.8901204070909));
#36620=CARTESIAN_POINT('Origin',(42.4,51.6008,48.));
#36621=CARTESIAN_POINT('',(41.7379836874626,51.7508,51.7544810775837));
#36622=CARTESIAN_POINT('Ctrl Pts',(41.6466229507512,51.6008,51.8901204070909));
#36623=CARTESIAN_POINT('Ctrl Pts',(41.6931846350573,51.6775199678395,51.8209922907102));
#36624=CARTESIAN_POINT('Ctrl Pts',(41.7379836874626,51.7508,51.7544810775837));
#36625=CARTESIAN_POINT('',(41.7774433146613,51.6008,51.9131875668744));
#36626=CARTESIAN_POINT('Ctrl Pts',(41.7379836874626,51.7508,51.7544810775837));
#36627=CARTESIAN_POINT('Ctrl Pts',(41.7573328517799,51.6775199678389,51.8323033520833));
#36628=CARTESIAN_POINT('Ctrl Pts',(41.7774433146613,51.6008,51.9131875668744));
#36629=CARTESIAN_POINT('',(42.3335807605545,51.6008,51.9618432887523));
#36630=CARTESIAN_POINT('Origin',(42.4,51.6008,48.));
#36631=CARTESIAN_POINT('',(42.4,51.7508,51.8124));
#36632=CARTESIAN_POINT('Ctrl Pts',(42.3335807605545,51.6008,51.9618432887523));
#36633=CARTESIAN_POINT('Ctrl Pts',(42.3674310968175,51.6775199678395,51.8856800321605));
#36634=CARTESIAN_POINT('Ctrl Pts',(42.4,51.7508,51.8124));
#36635=CARTESIAN_POINT('',(42.4664192394455,51.6008,51.9618432887523));
#36636=CARTESIAN_POINT('Ctrl Pts',(42.4,51.7508,51.8124));
#36637=CARTESIAN_POINT('Ctrl Pts',(42.4325689031826,51.6775199678391,51.8856800321609));
#36638=CARTESIAN_POINT('Ctrl Pts',(42.4664192394455,51.6008,51.9618432887523));
#36639=CARTESIAN_POINT('',(43.0225566853387,51.6008,51.9131875668744));
#36640=CARTESIAN_POINT('Origin',(42.4,51.6008,48.));
#36641=CARTESIAN_POINT('',(43.0620163125374,51.7508,51.7544810775837));
#36642=CARTESIAN_POINT('Ctrl Pts',(43.0225566853387,51.6008,51.9131875668744));
#36643=CARTESIAN_POINT('Ctrl Pts',(43.0426671482202,51.6775199678391,51.832303352083));
#36644=CARTESIAN_POINT('Ctrl Pts',(43.0620163125374,51.7508,51.7544810775837));
#36645=CARTESIAN_POINT('',(43.1533770492489,51.6008,51.8901204070909));
#36646=CARTESIAN_POINT('Ctrl Pts',(43.0620163125374,51.7508,51.7544810775837));
#36647=CARTESIAN_POINT('Ctrl Pts',(43.1068153649428,51.6775199678392,51.8209922907104));
#36648=CARTESIAN_POINT('Ctrl Pts',(43.1533770492489,51.6008,51.8901204070909));
#36649=CARTESIAN_POINT('',(43.6926165402678,51.6008,51.7456316209454));
#36650=CARTESIAN_POINT('Origin',(42.4,51.6008,48.));
#36651=CARTESIAN_POINT('',(43.7039175944148,51.7508,51.5824841474842));
#36652=CARTESIAN_POINT('Ctrl Pts',(43.6926165402678,51.6008,51.7456316209454));
#36653=CARTESIAN_POINT('Ctrl Pts',(43.6983760835296,51.6775199678391,51.6624840738913));
#36654=CARTESIAN_POINT('Ctrl Pts',(43.7039175944148,51.7508,51.5824841474842));
#36655=CARTESIAN_POINT('',(43.817443878638,51.6008,51.700198185356));
#36656=CARTESIAN_POINT('Ctrl Pts',(43.7039175944148,51.7508,51.5824841474842));
#36657=CARTESIAN_POINT('Ctrl Pts',(43.759585599505,51.6775199678393,51.6402056320221));
#36658=CARTESIAN_POINT('Ctrl Pts',(43.817443878638,51.6008,51.700198185356));
#36659=CARTESIAN_POINT('',(44.3234008957163,51.6008,51.4642665535951));
#36660=CARTESIAN_POINT('Origin',(42.4,51.6008,48.));
#36661=CARTESIAN_POINT('',(44.3062,51.7508,51.3016352493878));
#36662=CARTESIAN_POINT('Ctrl Pts',(44.3234008957163,51.6008,51.4642665535951));
#36663=CARTESIAN_POINT('Ctrl Pts',(44.3146345185509,51.6775199678393,51.3813820704204));
#36664=CARTESIAN_POINT('Ctrl Pts',(44.3062,51.7508,51.3016352493878));
#36665=CARTESIAN_POINT('',(44.438442393036,51.6008,51.3978473141496));
#36666=CARTESIAN_POINT('Ctrl Pts',(44.3062,51.7508,51.3016352493878));
#36667=CARTESIAN_POINT('Ctrl Pts',(44.3710455136094,51.6775199678397,51.3488131672376));
#36668=CARTESIAN_POINT('Ctrl Pts',(44.438442393036,51.6008,51.3978473141496));
#36669=CARTESIAN_POINT('',(44.8957436882364,51.6008,51.0776415000172));
#36670=CARTESIAN_POINT('Origin',(42.4,51.6008,48.));
#36671=CARTESIAN_POINT('',(44.850563483169,51.7508,50.9204678349468));
#36672=CARTESIAN_POINT('Ctrl Pts',(44.8957436882364,51.6008,51.0776415000173));
#36673=CARTESIAN_POINT('Ctrl Pts',(44.8727177525779,51.6775199678391,50.9975384838021));
#36674=CARTESIAN_POINT('Ctrl Pts',(44.850563483169,51.7508,50.9204678349468));
#36675=CARTESIAN_POINT('',(44.9975038668231,51.6008,50.9922545716965));
#36676=CARTESIAN_POINT('Ctrl Pts',(44.850563483169,51.7508,50.9204678349468));
#36677=CARTESIAN_POINT('Ctrl Pts',(44.9226162071806,51.6775199678395,50.9556687089482));
#36678=CARTESIAN_POINT('Ctrl Pts',(44.9975038668231,51.6008,50.9922545716965));
#36679=CARTESIAN_POINT('',(45.3922545716966,51.6008,50.5975038668231));
#36680=CARTESIAN_POINT('Origin',(42.4,51.6008,48.));
#36681=CARTESIAN_POINT('',(45.3204678349468,51.7508,50.4505634831689));
#36682=CARTESIAN_POINT('Ctrl Pts',(45.3922545716966,51.6008,50.5975038668231));
#36683=CARTESIAN_POINT('Ctrl Pts',(45.3556687089481,51.6775199678396,50.5226162071804));
#36684=CARTESIAN_POINT('Ctrl Pts',(45.3204678349468,51.7508,50.4505634831689));
#36685=CARTESIAN_POINT('',(45.4776415000172,51.6008,50.4957436882363));
#36686=CARTESIAN_POINT('Ctrl Pts',(45.3204678349468,51.7508,50.4505634831689));
#36687=CARTESIAN_POINT('Ctrl Pts',(45.3975384838014,51.6775199678397,50.4727177525777));
#36688=CARTESIAN_POINT('Ctrl Pts',(45.4776415000172,51.6008,50.4957436882363));
#36689=CARTESIAN_POINT('',(45.7978473141496,51.6008,50.038442393036));
#36690=CARTESIAN_POINT('Origin',(42.4,51.6008,48.));
#36691=CARTESIAN_POINT('',(45.7016352493878,51.7508,49.9062));
#36692=CARTESIAN_POINT('Ctrl Pts',(45.7978473141496,51.6008,50.038442393036));
#36693=CARTESIAN_POINT('Ctrl Pts',(45.7488131672377,51.6775199678395,49.9710455136096));
#36694=CARTESIAN_POINT('Ctrl Pts',(45.7016352493878,51.7508,49.9062));
#36695=CARTESIAN_POINT('',(45.8642665535951,51.6008,49.9234008957163));
#36696=CARTESIAN_POINT('Ctrl Pts',(45.7016352493878,51.7508,49.9062));
#36697=CARTESIAN_POINT('Ctrl Pts',(45.7813820704199,51.6775199678397,49.9146345185508));
#36698=CARTESIAN_POINT('Ctrl Pts',(45.8642665535951,51.6008,49.9234008957163));
#36699=CARTESIAN_POINT('',(46.100198185356,51.6008,49.417443878638));
#36700=CARTESIAN_POINT('Origin',(42.4,51.6008,48.));
#36701=CARTESIAN_POINT('',(45.9824841474842,51.7508,49.3039175944148));
#36702=CARTESIAN_POINT('Ctrl Pts',(46.100198185356,51.6008,49.417443878638));
#36703=CARTESIAN_POINT('Ctrl Pts',(46.0402056320216,51.67751996784,49.3595855995045));
#36704=CARTESIAN_POINT('Ctrl Pts',(45.9824841474842,51.7508,49.3039175944148));
#36705=CARTESIAN_POINT('',(46.1456316209454,51.6008,49.2926165402678));
#36706=CARTESIAN_POINT('Ctrl Pts',(45.9824841474842,51.7508,49.3039175944148));
#36707=CARTESIAN_POINT('Ctrl Pts',(46.0624840738902,51.67751996784,49.2983760835296));
#36708=CARTESIAN_POINT('Ctrl Pts',(46.1456316209454,51.6008,49.2926165402678));
#36709=CARTESIAN_POINT('',(46.2901204070909,51.6008,48.7533770492488));
#36710=CARTESIAN_POINT('Origin',(42.4,51.6008,48.));
#36711=CARTESIAN_POINT('',(46.1544810775837,51.7508,48.6620163125374));
#36712=CARTESIAN_POINT('Ctrl Pts',(46.2901204070909,51.6008,48.7533770492488));
#36713=CARTESIAN_POINT('Ctrl Pts',(46.2209922907101,51.6775199678395,48.7068153649426));
#36714=CARTESIAN_POINT('Ctrl Pts',(46.1544810775837,51.7508,48.6620163125374));
#36715=CARTESIAN_POINT('',(46.3131875668744,51.6008,48.6225566853387));
#36716=CARTESIAN_POINT('Ctrl Pts',(46.1544810775837,51.7508,48.6620163125374));
#36717=CARTESIAN_POINT('Ctrl Pts',(46.2323033520828,51.6775199678393,48.6426671482202));
#36718=CARTESIAN_POINT('Ctrl Pts',(46.3131875668744,51.6008,48.6225566853387));
#36719=CARTESIAN_POINT('',(46.3618432887523,51.6008,48.0664192394455));
#36720=CARTESIAN_POINT('Origin',(42.4,51.6008,48.));
#36721=CARTESIAN_POINT('',(46.2124,51.7508,48.));
#36722=CARTESIAN_POINT('Ctrl Pts',(46.3618432887523,51.6008,48.0664192394455));
#36723=CARTESIAN_POINT('Ctrl Pts',(46.28568003216,51.67751996784,48.0325689031822));
#36724=CARTESIAN_POINT('Ctrl Pts',(46.2124,51.7508,48.));
#36725=CARTESIAN_POINT('',(46.3618432887523,51.6008,47.9335807605545));
#36726=CARTESIAN_POINT('Ctrl Pts',(46.2124,51.7508,48.));
#36727=CARTESIAN_POINT('Ctrl Pts',(46.2856800321602,51.6775199678398,47.9674310968177));
#36728=CARTESIAN_POINT('Ctrl Pts',(46.3618432887523,51.6008,47.9335807605545));
#36729=CARTESIAN_POINT('Origin',(42.4,51.6008,48.));
#36730=CARTESIAN_POINT('',(46.1456316209454,51.6008,46.7073834597322));
#36731=CARTESIAN_POINT('Origin',(42.4,51.6008,48.));
#36732=CARTESIAN_POINT('',(45.9824841474842,51.7508,46.6960824055852));
#36733=CARTESIAN_POINT('Ctrl Pts',(46.1456316209454,51.6008,46.7073834597322));
#36734=CARTESIAN_POINT('Ctrl Pts',(46.0624840738912,51.6775199678392,46.7016239164704));
#36735=CARTESIAN_POINT('Ctrl Pts',(45.9824841474842,51.7508,46.6960824055852));
#36736=CARTESIAN_POINT('',(46.100198185356,51.6008,46.582556121362));
#36737=CARTESIAN_POINT('Ctrl Pts',(45.9824841474842,51.7508,46.6960824055852));
#36738=CARTESIAN_POINT('Ctrl Pts',(46.040205632022,51.6775199678395,46.6404144004951));
#36739=CARTESIAN_POINT('Ctrl Pts',(46.100198185356,51.6008,46.582556121362));
#36740=CARTESIAN_POINT('',(45.8642665535951,51.6008,46.0765991042837));
#36741=CARTESIAN_POINT('Origin',(42.4,51.6008,48.));
#36742=CARTESIAN_POINT('',(45.7016352493878,51.7508,46.0938));
#36743=CARTESIAN_POINT('Ctrl Pts',(45.8642665535951,51.6008,46.0765991042837));
#36744=CARTESIAN_POINT('Ctrl Pts',(45.7813820704199,51.6775199678398,46.0853654814492));
#36745=CARTESIAN_POINT('Ctrl Pts',(45.7016352493878,51.7508,46.0938));
#36746=CARTESIAN_POINT('',(45.7978473141496,51.6008,45.961557606964));
#36747=CARTESIAN_POINT('Ctrl Pts',(45.7016352493878,51.7508,46.0938));
#36748=CARTESIAN_POINT('Ctrl Pts',(45.7488131672375,51.6775199678399,46.0289544863907));
#36749=CARTESIAN_POINT('Ctrl Pts',(45.7978473141496,51.6008,45.961557606964));
#36750=CARTESIAN_POINT('',(45.4776415000172,51.6008,45.5042563117636));
#36751=CARTESIAN_POINT('Origin',(42.4,51.6008,48.));
#36752=CARTESIAN_POINT('',(45.3204678349468,51.7508,45.549436516831));
#36753=CARTESIAN_POINT('Ctrl Pts',(45.4776415000173,51.6008,45.5042563117637));
#36754=CARTESIAN_POINT('Ctrl Pts',(45.3975384838014,51.6775199678398,45.5272822474223));
#36755=CARTESIAN_POINT('Ctrl Pts',(45.3204678349468,51.7508,45.549436516831));
#36756=CARTESIAN_POINT('',(45.3922545716966,51.6008,45.4024961331769));
#36757=CARTESIAN_POINT('Ctrl Pts',(45.3204678349468,51.7508,45.549436516831));
#36758=CARTESIAN_POINT('Ctrl Pts',(45.3556687089482,51.6775199678395,45.4773837928194));
#36759=CARTESIAN_POINT('Ctrl Pts',(45.3922545716966,51.6008,45.4024961331769));
#36760=CARTESIAN_POINT('',(44.9975038668231,51.6008,45.0077454283035));
#36761=CARTESIAN_POINT('Origin',(42.4,51.6008,48.));
#36762=CARTESIAN_POINT('',(44.850563483169,51.7508,45.0795321650532));
#36763=CARTESIAN_POINT('Ctrl Pts',(44.9975038668231,51.6008,45.0077454283034));
#36764=CARTESIAN_POINT('Ctrl Pts',(44.9226162071805,51.6775199678396,45.0443312910519));
#36765=CARTESIAN_POINT('Ctrl Pts',(44.850563483169,51.7508,45.0795321650532));
#36766=CARTESIAN_POINT('',(44.8957436882364,51.6008,44.9223584999827));
#36767=CARTESIAN_POINT('Ctrl Pts',(44.850563483169,51.7508,45.0795321650532));
#36768=CARTESIAN_POINT('Ctrl Pts',(44.8727177525775,51.6775199678404,45.0024615161993));
#36769=CARTESIAN_POINT('Ctrl Pts',(44.8957436882364,51.6008,44.9223584999828));
#36770=CARTESIAN_POINT('',(44.4384423930359,51.6008,44.6021526858504));
#36771=CARTESIAN_POINT('Origin',(42.4,51.6008,48.));
#36772=CARTESIAN_POINT('',(44.3062,51.7508,44.6983647506122));
#36773=CARTESIAN_POINT('Ctrl Pts',(44.4384423930359,51.6008,44.6021526858504));
#36774=CARTESIAN_POINT('Ctrl Pts',(44.37104551361,51.6775199678391,44.651186832762));
#36775=CARTESIAN_POINT('Ctrl Pts',(44.3062,51.7508,44.6983647506122));
#36776=CARTESIAN_POINT('',(44.3234008957163,51.6008,44.5357334464049));
#36777=CARTESIAN_POINT('Ctrl Pts',(44.3062,51.7508,44.6983647506122));
#36778=CARTESIAN_POINT('Ctrl Pts',(44.3146345185509,51.6775199678395,44.6186179295799));
#36779=CARTESIAN_POINT('Ctrl Pts',(44.3234008957163,51.6008,44.5357334464049));
#36780=CARTESIAN_POINT('',(43.817443878638,51.6008,44.299801814644));
#36781=CARTESIAN_POINT('Origin',(42.4,51.6008,48.));
#36782=CARTESIAN_POINT('',(43.7039175944148,51.7508,44.4175158525158));
#36783=CARTESIAN_POINT('Ctrl Pts',(43.817443878638,51.6008,44.299801814644));
#36784=CARTESIAN_POINT('Ctrl Pts',(43.7595855995047,51.6775199678397,44.3597943679782));
#36785=CARTESIAN_POINT('Ctrl Pts',(43.7039175944148,51.7508,44.4175158525158));
#36786=CARTESIAN_POINT('',(43.6926165402678,51.6008,44.2543683790546));
#36787=CARTESIAN_POINT('Ctrl Pts',(43.7039175944148,51.7508,44.4175158525158));
#36788=CARTESIAN_POINT('Ctrl Pts',(43.6983760835296,51.6775199678396,44.3375159261093));
#36789=CARTESIAN_POINT('Ctrl Pts',(43.6926165402678,51.6008,44.2543683790546));
#36790=CARTESIAN_POINT('',(43.1533770492489,51.6008,44.1098795929091));
#36791=CARTESIAN_POINT('Origin',(42.4,51.6008,48.));
#36792=CARTESIAN_POINT('',(43.0620163125374,51.7508,44.2455189224163));
#36793=CARTESIAN_POINT('Ctrl Pts',(43.1533770492489,51.6008,44.1098795929091));
#36794=CARTESIAN_POINT('Ctrl Pts',(43.1068153649429,51.6775199678391,44.1790077092895));
#36795=CARTESIAN_POINT('Ctrl Pts',(43.0620163125374,51.7508,44.2455189224163));
#36796=CARTESIAN_POINT('',(43.0225566853387,51.6008,44.0868124331256));
#36797=CARTESIAN_POINT('Ctrl Pts',(43.0620163125374,51.7508,44.2455189224163));
#36798=CARTESIAN_POINT('Ctrl Pts',(43.0426671482202,51.6775199678393,44.1676966479172));
#36799=CARTESIAN_POINT('Ctrl Pts',(43.0225566853387,51.6008,44.0868124331256));
#36800=CARTESIAN_POINT('',(42.4664192394455,51.6008,44.0381567112477));
#36801=CARTESIAN_POINT('Origin',(42.4,51.6008,48.));
#36802=CARTESIAN_POINT('',(42.4,51.7508,44.1876));
#36803=CARTESIAN_POINT('Ctrl Pts',(42.4664192394455,51.6008,44.0381567112477));
#36804=CARTESIAN_POINT('Ctrl Pts',(42.4325689031828,51.6775199678388,44.1143199678388));
#36805=CARTESIAN_POINT('Ctrl Pts',(42.4,51.7508,44.1876));
#36806=CARTESIAN_POINT('',(42.3335807605545,51.6008,44.0381567112477));
#36807=CARTESIAN_POINT('Ctrl Pts',(42.4,51.7508,44.1876));
#36808=CARTESIAN_POINT('Ctrl Pts',(42.3674310968175,51.6775199678393,44.1143199678393));
#36809=CARTESIAN_POINT('Ctrl Pts',(42.3335807605545,51.6008,44.0381567112477));
#36810=CARTESIAN_POINT('',(41.7774433146613,51.6008,44.0868124331256));
#36811=CARTESIAN_POINT('Origin',(42.4,51.6008,48.));
#36812=CARTESIAN_POINT('',(41.7379836874626,51.7508,44.2455189224162));
#36813=CARTESIAN_POINT('Ctrl Pts',(41.7774433146613,51.6008,44.0868124331256));
#36814=CARTESIAN_POINT('Ctrl Pts',(41.7573328517799,51.6775199678389,44.1676966479167));
#36815=CARTESIAN_POINT('Ctrl Pts',(41.7379836874626,51.7508,44.2455189224162));
#36816=CARTESIAN_POINT('',(41.6466229507512,51.6008,44.1098795929091));
#36817=CARTESIAN_POINT('Ctrl Pts',(41.7379836874626,51.7508,44.2455189224162));
#36818=CARTESIAN_POINT('Ctrl Pts',(41.693184635057,51.6775199678389,44.1790077092893));
#36819=CARTESIAN_POINT('Ctrl Pts',(41.6466229507511,51.6008,44.1098795929091));
#36820=CARTESIAN_POINT('',(41.1073834597322,51.6008,44.2543683790546));
#36821=CARTESIAN_POINT('Origin',(42.4,51.6008,48.));
#36822=CARTESIAN_POINT('',(41.0960824055852,51.7508,44.4175158525158));
#36823=CARTESIAN_POINT('Ctrl Pts',(41.1073834597322,51.6008,44.2543683790546));
#36824=CARTESIAN_POINT('Ctrl Pts',(41.1016239164704,51.6775199678393,44.337515926109));
#36825=CARTESIAN_POINT('Ctrl Pts',(41.0960824055852,51.7508,44.4175158525158));
#36826=CARTESIAN_POINT('',(40.982556121362,51.6008,44.299801814644));
#36827=CARTESIAN_POINT('Ctrl Pts',(41.0960824055852,51.7508,44.4175158525158));
#36828=CARTESIAN_POINT('Ctrl Pts',(41.0404144004952,51.6775199678396,44.3597943679781));
#36829=CARTESIAN_POINT('Ctrl Pts',(40.982556121362,51.6008,44.299801814644));
#36830=CARTESIAN_POINT('',(40.4765991042837,51.6008,44.5357334464049));
#36831=CARTESIAN_POINT('Origin',(42.4,51.6008,48.));
#36832=CARTESIAN_POINT('',(40.4938,51.7508,44.6983647506122));
#36833=CARTESIAN_POINT('Ctrl Pts',(40.4765991042837,51.6008,44.5357334464049));
#36834=CARTESIAN_POINT('Ctrl Pts',(40.4853654814491,51.6775199678393,44.6186179295796));
#36835=CARTESIAN_POINT('Ctrl Pts',(40.4938,51.7508,44.6983647506122));
#36836=CARTESIAN_POINT('',(40.3615576069641,51.6008,44.6021526858504));
#36837=CARTESIAN_POINT('Ctrl Pts',(40.4938,51.7508,44.6983647506122));
#36838=CARTESIAN_POINT('Ctrl Pts',(40.4289544863898,51.6775199678389,44.6511868327619));
#36839=CARTESIAN_POINT('Ctrl Pts',(40.3615576069641,51.6008,44.6021526858504));
#36840=CARTESIAN_POINT('',(39.9042563117637,51.6008,44.9223584999827));
#36841=CARTESIAN_POINT('Origin',(42.4,51.6008,48.));
#36842=CARTESIAN_POINT('',(39.949436516831,51.7508,45.0795321650532));
#36843=CARTESIAN_POINT('Ctrl Pts',(39.9042563117637,51.6008,44.9223584999827));
#36844=CARTESIAN_POINT('Ctrl Pts',(39.9272822474223,51.6775199678396,45.0024615161984));
#36845=CARTESIAN_POINT('Ctrl Pts',(39.949436516831,51.7508,45.0795321650532));
#36846=CARTESIAN_POINT('',(39.8024961331769,51.6008,45.0077454283035));
#36847=CARTESIAN_POINT('Ctrl Pts',(39.949436516831,51.7508,45.0795321650532));
#36848=CARTESIAN_POINT('Ctrl Pts',(39.8773837928197,51.6775199678398,45.0443312910519));
#36849=CARTESIAN_POINT('Ctrl Pts',(39.8024961331769,51.6008,45.0077454283035));
#36850=CARTESIAN_POINT('',(39.4077454283035,51.6008,45.4024961331769));
#36851=CARTESIAN_POINT('Origin',(42.4,51.6008,48.));
#36852=CARTESIAN_POINT('',(39.4795321650532,51.7508,45.549436516831));
#36853=CARTESIAN_POINT('Ctrl Pts',(39.4077454283035,51.6008,45.4024961331769));
#36854=CARTESIAN_POINT('Ctrl Pts',(39.4443312910519,51.6775199678397,45.4773837928196));
#36855=CARTESIAN_POINT('Ctrl Pts',(39.4795321650532,51.7508,45.549436516831));
#36856=CARTESIAN_POINT('',(39.3223584999828,51.6008,45.5042563117637));
#36857=CARTESIAN_POINT('Ctrl Pts',(39.4795321650532,51.7508,45.549436516831));
#36858=CARTESIAN_POINT('Ctrl Pts',(39.4024615161982,51.6775199678394,45.5272822474222));
#36859=CARTESIAN_POINT('Ctrl Pts',(39.3223584999828,51.6008,45.5042563117637));
#36860=CARTESIAN_POINT('',(39.0021526858504,51.6008,45.961557606964));
#36861=CARTESIAN_POINT('Origin',(42.4,51.6008,48.));
#36862=CARTESIAN_POINT('',(39.0983647506122,51.7508,46.0938));
#36863=CARTESIAN_POINT('Ctrl Pts',(39.0021526858504,51.6008,45.961557606964));
#36864=CARTESIAN_POINT('Ctrl Pts',(39.0511868327623,51.6775199678396,46.0289544863904));
#36865=CARTESIAN_POINT('Ctrl Pts',(39.0983647506122,51.7508,46.0938));
#36866=CARTESIAN_POINT('',(38.9357334464049,51.6008,46.0765991042837));
#36867=CARTESIAN_POINT('Ctrl Pts',(39.0983647506122,51.7508,46.0938));
#36868=CARTESIAN_POINT('Ctrl Pts',(39.0186179295797,51.6775199678394,46.0853654814491));
#36869=CARTESIAN_POINT('Ctrl Pts',(38.9357334464049,51.6008,46.0765991042837));
#36870=CARTESIAN_POINT('',(38.699801814644,51.6008,46.582556121362));
#36871=CARTESIAN_POINT('Origin',(42.4,51.6008,48.));
#36872=CARTESIAN_POINT('',(38.8175158525158,51.7508,46.6960824055852));
#36873=CARTESIAN_POINT('Ctrl Pts',(38.699801814644,51.6008,46.582556121362));
#36874=CARTESIAN_POINT('Ctrl Pts',(38.7597943679782,51.6775199678396,46.6404144004952));
#36875=CARTESIAN_POINT('Ctrl Pts',(38.8175158525158,51.7508,46.6960824055852));
#36876=CARTESIAN_POINT('',(38.6543683790546,51.6008,46.7073834597322));
#36877=CARTESIAN_POINT('Ctrl Pts',(38.8175158525158,51.7508,46.6960824055852));
#36878=CARTESIAN_POINT('Ctrl Pts',(38.7375159261091,51.6775199678394,46.7016239164704));
#36879=CARTESIAN_POINT('Ctrl Pts',(38.6543683790546,51.6008,46.7073834597322));
#36880=CARTESIAN_POINT('',(38.5098795929091,51.6008,47.2466229507512));
#36881=CARTESIAN_POINT('Origin',(42.4,51.6008,48.));
#36882=CARTESIAN_POINT('',(38.6455189224163,51.7508,47.3379836874626));
#36883=CARTESIAN_POINT('Ctrl Pts',(38.5098795929091,51.6008,47.2466229507512));
#36884=CARTESIAN_POINT('Ctrl Pts',(38.5790077092902,51.6775199678398,47.2931846350576));
#36885=CARTESIAN_POINT('Ctrl Pts',(38.6455189224163,51.7508,47.3379836874626));
#36886=CARTESIAN_POINT('',(38.4868124331256,51.6008,47.3774433146613));
#36887=CARTESIAN_POINT('Ctrl Pts',(38.6455189224163,51.7508,47.3379836874626));
#36888=CARTESIAN_POINT('Ctrl Pts',(38.5676966479172,51.6775199678394,47.3573328517798));
#36889=CARTESIAN_POINT('Ctrl Pts',(38.4868124331256,51.6008,47.3774433146613));
#36890=CARTESIAN_POINT('',(38.4381567112477,51.6008,47.9335807605545));
#36891=CARTESIAN_POINT('Origin',(42.4,51.6008,48.));
#36892=CARTESIAN_POINT('Ctrl Pts',(38.4381567112477,51.6008,47.9335807605545));
#36893=CARTESIAN_POINT('Ctrl Pts',(38.5143199678391,51.6775199678391,47.9674310968174));
#36894=CARTESIAN_POINT('Ctrl Pts',(38.5876,51.7508,48.));
#36895=CARTESIAN_POINT('',(38.8376,52.0008,48.));
#36896=CARTESIAN_POINT('',(38.6376,51.8008,48.));
#36897=CARTESIAN_POINT('Origin',(42.4,52.0008,48.));
#36898=CARTESIAN_POINT('Origin',(46.473749855503,52.0008,46.7301118652459));
#36899=CARTESIAN_POINT('',(46.1456316209454,47.7748,46.7073834597322));
#36900=CARTESIAN_POINT('',(46.1456316209454,47.1748,46.7073834597322));
#36901=CARTESIAN_POINT('',(45.9824841474842,47.7748,46.6960824055852));
#36902=CARTESIAN_POINT('',(46.473749855503,47.7748,46.7301118652459));
#36903=CARTESIAN_POINT('',(45.9824841474842,52.0008,46.6960824055852));
#36904=CARTESIAN_POINT('Origin',(45.9824841474842,52.0008,46.6960824055852));
#36905=CARTESIAN_POINT('',(46.100198185356,47.7748,46.582556121362));
#36906=CARTESIAN_POINT('',(46.100198185356,47.1748,46.582556121362));
#36907=CARTESIAN_POINT('',(45.9824841474842,47.7748,46.6960824055852));
#36908=CARTESIAN_POINT('Origin',(46.193914987161,47.7748,46.6191278733369));
#36909=CARTESIAN_POINT('Origin',(42.4,47.7748,48.));
#36910=CARTESIAN_POINT('Origin',(46.1913466810908,52.0008,46.0420050807569));
#36911=CARTESIAN_POINT('',(45.8642665535951,47.7748,46.0765991042837));
#36912=CARTESIAN_POINT('',(45.8642665535951,47.1748,46.0765991042837));
#36913=CARTESIAN_POINT('',(45.7016352493878,47.7748,46.0938));
#36914=CARTESIAN_POINT('',(46.1913466810908,47.7748,46.0420050807569));
#36915=CARTESIAN_POINT('',(45.7016352493878,52.0008,46.0938));
#36916=CARTESIAN_POINT('Origin',(45.7016352493878,52.0008,46.0938));
#36917=CARTESIAN_POINT('',(45.7978473141496,47.7748,45.961557606964));
#36918=CARTESIAN_POINT('',(45.7978473141496,47.1748,45.961557606964));
#36919=CARTESIAN_POINT('',(45.7016352493878,47.7748,46.0938));
#36920=CARTESIAN_POINT('Origin',(45.8964909652393,47.7748,45.9813));
#36921=CARTESIAN_POINT('Origin',(42.4,47.7748,48.));
#36922=CARTESIAN_POINT('Origin',(45.7937453562877,52.0008,45.4133909810959));
#36923=CARTESIAN_POINT('',(45.4776415000172,47.7748,45.5042563117636));
#36924=CARTESIAN_POINT('',(45.4776415000172,47.1748,45.5042563117636));
#36925=CARTESIAN_POINT('',(45.3204678349468,47.7748,45.549436516831));
#36926=CARTESIAN_POINT('',(45.7937453562877,47.7748,45.4133909810959));
#36927=CARTESIAN_POINT('',(45.3204678349468,52.0008,45.549436516831));
#36928=CARTESIAN_POINT('Origin',(45.3204678349468,52.0008,45.549436516831));
#36929=CARTESIAN_POINT('',(45.3922545716966,47.7748,45.4024961331769));
#36930=CARTESIAN_POINT('',(45.3922545716966,47.1748,45.4024961331769));
#36931=CARTESIAN_POINT('',(45.3204678349468,47.7748,45.549436516831));
#36932=CARTESIAN_POINT('Origin',(45.4928278346486,47.7748,45.4048093046516));
#36933=CARTESIAN_POINT('Origin',(42.4,47.7748,48.));
#36934=CARTESIAN_POINT('Origin',(45.2930267961517,52.0008,44.863369687587));
#36935=CARTESIAN_POINT('',(44.9975038668231,47.7748,45.0077454283035));
#36936=CARTESIAN_POINT('',(44.9975038668231,47.1748,45.0077454283035));
#36937=CARTESIAN_POINT('',(44.850563483169,47.7748,45.0795321650532));
#36938=CARTESIAN_POINT('',(45.2930267961517,47.7748,44.863369687587));
#36939=CARTESIAN_POINT('',(44.850563483169,52.0008,45.0795321650532));
#36940=CARTESIAN_POINT('Origin',(44.850563483169,52.0008,45.0795321650532));
#36941=CARTESIAN_POINT('',(44.8957436882364,47.7748,44.9223584999827));
#36942=CARTESIAN_POINT('',(44.8957436882364,47.1748,44.9223584999827));
#36943=CARTESIAN_POINT('',(44.850563483169,47.7748,45.0795321650532));
#36944=CARTESIAN_POINT('Origin',(44.9951906953484,47.7748,44.9071721653514));
#36945=CARTESIAN_POINT('Origin',(42.4,47.7748,48.));
#36946=CARTESIAN_POINT('Origin',(44.7044050807569,52.0008,44.4086533189092));
#36947=CARTESIAN_POINT('',(44.4384423930359,47.7748,44.6021526858504));
#36948=CARTESIAN_POINT('',(44.4384423930359,47.1748,44.6021526858504));
#36949=CARTESIAN_POINT('',(44.3062,47.7748,44.6983647506122));
#36950=CARTESIAN_POINT('',(44.7044050807569,47.7748,44.4086533189092));
#36951=CARTESIAN_POINT('',(44.3062,52.0008,44.6983647506122));
#36952=CARTESIAN_POINT('Origin',(44.3062,52.0008,44.6983647506122));
#36953=CARTESIAN_POINT('',(44.3234008957163,47.7748,44.5357334464049));
#36954=CARTESIAN_POINT('',(44.3234008957163,47.1748,44.5357334464049));
#36955=CARTESIAN_POINT('',(44.3062,47.7748,44.6983647506122));
#36956=CARTESIAN_POINT('Origin',(44.4187,47.7748,44.5035090347607));
#36957=CARTESIAN_POINT('Origin',(42.4,47.7748,48.));
#36958=CARTESIAN_POINT('Origin',(44.0457651830685,52.0008,44.0630582018273));
#36959=CARTESIAN_POINT('',(43.817443878638,47.7748,44.299801814644));
#36960=CARTESIAN_POINT('',(43.817443878638,47.1748,44.299801814644));
#36961=CARTESIAN_POINT('',(43.7039175944148,47.7748,44.4175158525158));
#36962=CARTESIAN_POINT('',(44.0457651830685,47.7748,44.0630582018273));
#36963=CARTESIAN_POINT('',(43.7039175944148,52.0008,44.4175158525158));
#36964=CARTESIAN_POINT('Origin',(43.7039175944148,52.0008,44.4175158525158));
#36965=CARTESIAN_POINT('',(43.6926165402678,47.7748,44.2543683790546));
#36966=CARTESIAN_POINT('',(43.6926165402678,47.1748,44.2543683790546));
#36967=CARTESIAN_POINT('',(43.7039175944148,47.7748,44.4175158525158));
#36968=CARTESIAN_POINT('Origin',(43.7808721266631,47.7748,44.206085012839));
#36969=CARTESIAN_POINT('Origin',(42.4,47.7748,48.));
#36970=CARTESIAN_POINT('Origin',(43.33711954309,52.0008,43.8370850690942));
#36971=CARTESIAN_POINT('',(43.1533770492489,47.7748,44.1098795929091));
#36972=CARTESIAN_POINT('',(43.1533770492489,47.1748,44.1098795929091));
#36973=CARTESIAN_POINT('',(43.0620163125374,47.7748,44.2455189224163));
#36974=CARTESIAN_POINT('',(43.33711954309,47.7748,43.8370850690942));
#36975=CARTESIAN_POINT('',(43.0620163125374,52.0008,44.2455189224163));
#36976=CARTESIAN_POINT('Origin',(43.0620163125374,52.0008,44.2455189224163));
#36977=CARTESIAN_POINT('',(43.0225566853387,47.7748,44.0868124331256));
#36978=CARTESIAN_POINT('',(43.0225566853387,47.1748,44.0868124331256));
#36979=CARTESIAN_POINT('',(43.0620163125374,47.7748,44.2455189224163));
#36980=CARTESIAN_POINT('Origin',(43.1010871525125,47.7748,44.0239371779885));
#36981=CARTESIAN_POINT('Origin',(42.4,47.7748,48.));
#36982=CARTESIAN_POINT('Origin',(42.6,52.0008,43.7376));
#36983=CARTESIAN_POINT('',(42.4664192394455,47.7748,44.0381567112477));
#36984=CARTESIAN_POINT('',(42.4664192394455,47.1748,44.0381567112477));
#36985=CARTESIAN_POINT('',(42.4,47.7748,44.1876));
#36986=CARTESIAN_POINT('',(42.6,47.7748,43.7376));
#36987=CARTESIAN_POINT('',(42.4,52.0008,44.1876));
#36988=CARTESIAN_POINT('Origin',(42.4,52.0008,44.1876));
#36989=CARTESIAN_POINT('',(42.3335807605545,47.7748,44.0381567112477));
#36990=CARTESIAN_POINT('',(42.3335807605545,47.1748,44.0381567112477));
#36991=CARTESIAN_POINT('',(42.4,47.7748,44.1876));
#36992=CARTESIAN_POINT('Origin',(42.4,47.7748,43.9626));
#36993=CARTESIAN_POINT('Origin',(42.4,47.7748,48.));
#36994=CARTESIAN_POINT('Origin',(41.8568035581149,52.0008,43.7676257980274));
#36995=CARTESIAN_POINT('',(41.7774433146613,47.7748,44.0868124331256));
#36996=CARTESIAN_POINT('',(41.7774433146613,47.1748,44.0868124331256));
#36997=CARTESIAN_POINT('',(41.7379836874626,47.7748,44.2455189224162));
#36998=CARTESIAN_POINT('',(41.8568035581149,47.7748,43.7676257980274));
#36999=CARTESIAN_POINT('',(41.7379836874626,52.0008,44.2455189224162));
#37000=CARTESIAN_POINT('Origin',(41.7379836874626,52.0008,44.2455189224162));
#37001=CARTESIAN_POINT('',(41.6466229507512,47.7748,44.1098795929091));
#37002=CARTESIAN_POINT('',(41.6466229507512,47.1748,44.1098795929091));
#37003=CARTESIAN_POINT('',(41.7379836874626,47.7748,44.2455189224162));
#37004=CARTESIAN_POINT('Origin',(41.6989128474875,47.7748,44.0239371779885));
#37005=CARTESIAN_POINT('Origin',(42.4,47.7748,48.));
#37006=CARTESIAN_POINT('Origin',(41.1301118652459,52.0008,43.926250144497));
#37007=CARTESIAN_POINT('',(41.1073834597322,47.7748,44.2543683790546));
#37008=CARTESIAN_POINT('',(41.1073834597322,47.1748,44.2543683790546));
#37009=CARTESIAN_POINT('',(41.0960824055852,47.7748,44.4175158525158));
#37010=CARTESIAN_POINT('',(41.1301118652459,47.7748,43.926250144497));
#37011=CARTESIAN_POINT('',(41.0960824055852,52.0008,44.4175158525158));
#37012=CARTESIAN_POINT('Origin',(41.0960824055852,52.0008,44.4175158525158));
#37013=CARTESIAN_POINT('',(40.982556121362,47.7748,44.299801814644));
#37014=CARTESIAN_POINT('',(40.982556121362,47.1748,44.299801814644));
#37015=CARTESIAN_POINT('',(41.0960824055852,47.7748,44.4175158525158));
#37016=CARTESIAN_POINT('Origin',(41.0191278733369,47.7748,44.206085012839));
#37017=CARTESIAN_POINT('Origin',(42.4,47.7748,48.));
#37018=CARTESIAN_POINT('Origin',(40.4420050807569,52.0008,44.2086533189092));
#37019=CARTESIAN_POINT('',(40.4765991042837,47.7748,44.5357334464049));
#37020=CARTESIAN_POINT('',(40.4765991042837,47.1748,44.5357334464049));
#37021=CARTESIAN_POINT('',(40.4938,47.7748,44.6983647506122));
#37022=CARTESIAN_POINT('',(40.4420050807569,47.7748,44.2086533189092));
#37023=CARTESIAN_POINT('',(40.4938,52.0008,44.6983647506122));
#37024=CARTESIAN_POINT('Origin',(40.4938,52.0008,44.6983647506122));
#37025=CARTESIAN_POINT('',(40.3615576069641,47.7748,44.6021526858504));
#37026=CARTESIAN_POINT('',(40.3615576069641,47.1748,44.6021526858504));
#37027=CARTESIAN_POINT('',(40.4938,47.7748,44.6983647506122));
#37028=CARTESIAN_POINT('Origin',(40.3813,47.7748,44.5035090347607));
#37029=CARTESIAN_POINT('Origin',(42.4,47.7748,48.));
#37030=CARTESIAN_POINT('Origin',(39.8133909810959,52.0008,44.6062546437123));
#37031=CARTESIAN_POINT('',(39.9042563117637,47.7748,44.9223584999827));
#37032=CARTESIAN_POINT('',(39.9042563117637,47.1748,44.9223584999827));
#37033=CARTESIAN_POINT('',(39.949436516831,47.7748,45.0795321650532));
#37034=CARTESIAN_POINT('',(39.8133909810959,47.7748,44.6062546437123));
#37035=CARTESIAN_POINT('',(39.949436516831,52.0008,45.0795321650532));
#37036=CARTESIAN_POINT('Origin',(39.949436516831,52.0008,45.0795321650532));
#37037=CARTESIAN_POINT('',(39.8024961331769,47.7748,45.0077454283035));
#37038=CARTESIAN_POINT('',(39.8024961331769,47.1748,45.0077454283035));
#37039=CARTESIAN_POINT('',(39.949436516831,47.7748,45.0795321650532));
#37040=CARTESIAN_POINT('Origin',(39.8048093046516,47.7748,44.9071721653514));
#37041=CARTESIAN_POINT('Origin',(42.4,47.7748,48.));
#37042=CARTESIAN_POINT('Origin',(39.263369687587,52.0008,45.1069732038483));
#37043=CARTESIAN_POINT('',(39.4077454283035,47.7748,45.4024961331769));
#37044=CARTESIAN_POINT('',(39.4077454283035,47.1748,45.4024961331769));
#37045=CARTESIAN_POINT('',(39.4795321650532,47.7748,45.549436516831));
#37046=CARTESIAN_POINT('',(39.263369687587,47.7748,45.1069732038483));
#37047=CARTESIAN_POINT('',(39.4795321650532,52.0008,45.549436516831));
#37048=CARTESIAN_POINT('Origin',(39.4795321650532,52.0008,45.549436516831));
#37049=CARTESIAN_POINT('',(39.3223584999828,47.7748,45.5042563117637));
#37050=CARTESIAN_POINT('',(39.3223584999828,47.1748,45.5042563117637));
#37051=CARTESIAN_POINT('',(39.4795321650532,47.7748,45.549436516831));
#37052=CARTESIAN_POINT('Origin',(39.3071721653514,47.7748,45.4048093046516));
#37053=CARTESIAN_POINT('Origin',(42.4,47.7748,48.));
#37054=CARTESIAN_POINT('Origin',(38.8086533189092,52.0008,45.6955949192431));
#37055=CARTESIAN_POINT('',(39.0021526858504,47.7748,45.961557606964));
#37056=CARTESIAN_POINT('',(39.0021526858504,47.1748,45.961557606964));
#37057=CARTESIAN_POINT('',(39.0983647506122,47.7748,46.0938));
#37058=CARTESIAN_POINT('',(38.8086533189092,47.7748,45.6955949192431));
#37059=CARTESIAN_POINT('',(39.0983647506122,52.0008,46.0938));
#37060=CARTESIAN_POINT('Origin',(39.0983647506122,52.0008,46.0938));
#37061=CARTESIAN_POINT('',(38.9357334464049,47.7748,46.0765991042837));
#37062=CARTESIAN_POINT('',(38.9357334464049,47.1748,46.0765991042837));
#37063=CARTESIAN_POINT('',(39.0983647506122,47.7748,46.0938));
#37064=CARTESIAN_POINT('Origin',(38.9035090347607,47.7748,45.9813));
#37065=CARTESIAN_POINT('Origin',(42.4,47.7748,48.));
#37066=CARTESIAN_POINT('Origin',(38.4630582018273,52.0008,46.3542348169315));
#37067=CARTESIAN_POINT('',(38.699801814644,47.7748,46.582556121362));
#37068=CARTESIAN_POINT('',(38.699801814644,47.1748,46.582556121362));
#37069=CARTESIAN_POINT('',(38.8175158525158,47.7748,46.6960824055852));
#37070=CARTESIAN_POINT('',(38.4630582018273,47.7748,46.3542348169315));
#37071=CARTESIAN_POINT('',(38.8175158525158,52.0008,46.6960824055852));
#37072=CARTESIAN_POINT('Origin',(38.8175158525158,52.0008,46.6960824055852));
#37073=CARTESIAN_POINT('',(38.6543683790546,47.7748,46.7073834597322));
#37074=CARTESIAN_POINT('',(38.6543683790546,47.1748,46.7073834597322));
#37075=CARTESIAN_POINT('',(38.8175158525158,47.7748,46.6960824055852));
#37076=CARTESIAN_POINT('Origin',(38.606085012839,47.7748,46.619127873337));
#37077=CARTESIAN_POINT('Origin',(42.4,47.7748,48.));
#37078=CARTESIAN_POINT('Origin',(38.2370850690942,52.0008,47.06288045691));
#37079=CARTESIAN_POINT('',(38.5098795929091,47.7748,47.2466229507512));
#37080=CARTESIAN_POINT('',(38.5098795929091,47.1748,47.2466229507512));
#37081=CARTESIAN_POINT('',(38.6455189224163,47.7748,47.3379836874626));
#37082=CARTESIAN_POINT('',(38.2370850690942,47.7748,47.06288045691));
#37083=CARTESIAN_POINT('',(38.6455189224163,52.0008,47.3379836874626));
#37084=CARTESIAN_POINT('Origin',(38.6455189224163,52.0008,47.3379836874626));
#37085=CARTESIAN_POINT('',(38.4868124331256,47.7748,47.3774433146613));
#37086=CARTESIAN_POINT('',(38.4868124331256,47.1748,47.3774433146613));
#37087=CARTESIAN_POINT('',(38.6455189224163,47.7748,47.3379836874626));
#37088=CARTESIAN_POINT('Origin',(38.4239371779885,47.7748,47.2989128474875));
#37089=CARTESIAN_POINT('Origin',(42.4,47.7748,48.));
#37090=CARTESIAN_POINT('Origin',(38.1376,52.0008,47.8));
#37091=CARTESIAN_POINT('',(38.4381567112477,47.7748,47.9335807605545));
#37092=CARTESIAN_POINT('',(38.4381567112477,47.1748,47.9335807605545));
#37093=CARTESIAN_POINT('',(38.5876,47.7748,48.));
#37094=CARTESIAN_POINT('',(38.1376,47.7748,47.8));
#37095=CARTESIAN_POINT('',(38.5876,52.0008,48.));
#37096=CARTESIAN_POINT('Origin',(38.5876,52.0008,48.));
#37097=CARTESIAN_POINT('',(38.4381567112477,47.7748,48.0664192394455));
#37098=CARTESIAN_POINT('',(38.4381567112477,47.1748,48.0664192394455));
#37099=CARTESIAN_POINT('',(38.5876,47.7748,48.));
#37100=CARTESIAN_POINT('Origin',(38.3626,47.7748,48.));
#37101=CARTESIAN_POINT('',(38.4376,47.7748,48.));
#37102=CARTESIAN_POINT('Origin',(42.4,47.7748,48.));
#37103=CARTESIAN_POINT('Origin',(42.4,47.7748,48.));
#37104=CARTESIAN_POINT('Origin',(38.1676257980274,52.0008,48.5431964418851));
#37105=CARTESIAN_POINT('',(38.4868124331256,47.7748,48.6225566853387));
#37106=CARTESIAN_POINT('',(38.4868124331256,47.1748,48.6225566853387));
#37107=CARTESIAN_POINT('',(38.6455189224163,47.7748,48.6620163125374));
#37108=CARTESIAN_POINT('',(38.1676257980274,47.7748,48.5431964418851));
#37109=CARTESIAN_POINT('',(38.6455189224163,52.0008,48.6620163125374));
#37110=CARTESIAN_POINT('Origin',(38.6455189224163,52.0008,48.6620163125374));
#37111=CARTESIAN_POINT('',(38.5098795929091,47.7748,48.7533770492488));
#37112=CARTESIAN_POINT('',(38.5098795929091,47.1748,48.7533770492488));
#37113=CARTESIAN_POINT('',(38.6455189224163,47.7748,48.6620163125374));
#37114=CARTESIAN_POINT('Origin',(38.4239371779885,47.7748,48.7010871525125));
#37115=CARTESIAN_POINT('Origin',(42.4,47.7748,48.));
#37116=CARTESIAN_POINT('Origin',(38.326250144497,52.0008,49.2698881347541));
#37117=CARTESIAN_POINT('',(38.6543683790546,47.7748,49.2926165402678));
#37118=CARTESIAN_POINT('',(38.6543683790546,47.1748,49.2926165402678));
#37119=CARTESIAN_POINT('',(38.8175158525158,47.7748,49.3039175944148));
#37120=CARTESIAN_POINT('',(38.326250144497,47.7748,49.2698881347541));
#37121=CARTESIAN_POINT('',(38.8175158525158,52.0008,49.3039175944148));
#37122=CARTESIAN_POINT('Origin',(38.8175158525158,52.0008,49.3039175944148));
#37123=CARTESIAN_POINT('',(38.699801814644,47.7748,49.417443878638));
#37124=CARTESIAN_POINT('',(38.699801814644,47.1748,49.417443878638));
#37125=CARTESIAN_POINT('',(38.8175158525158,47.7748,49.3039175944148));
#37126=CARTESIAN_POINT('Origin',(38.606085012839,47.7748,49.380872126663));
#37127=CARTESIAN_POINT('Origin',(42.4,47.7748,48.));
#37128=CARTESIAN_POINT('Origin',(38.6086533189092,52.0008,49.9579949192431));
#37129=CARTESIAN_POINT('',(38.9357334464049,47.7748,49.9234008957163));
#37130=CARTESIAN_POINT('',(38.9357334464049,47.1748,49.9234008957163));
#37131=CARTESIAN_POINT('',(39.0983647506122,47.7748,49.9062));
#37132=CARTESIAN_POINT('',(38.6086533189092,47.7748,49.9579949192431));
#37133=CARTESIAN_POINT('',(39.0983647506122,52.0008,49.9062));
#37134=CARTESIAN_POINT('Origin',(39.0983647506122,52.0008,49.9062));
#37135=CARTESIAN_POINT('',(39.0021526858504,47.7748,50.038442393036));
#37136=CARTESIAN_POINT('',(39.0021526858504,47.1748,50.038442393036));
#37137=CARTESIAN_POINT('',(39.0983647506122,47.7748,49.9062));
#37138=CARTESIAN_POINT('Origin',(38.9035090347607,47.7748,50.0187));
#37139=CARTESIAN_POINT('Origin',(42.4,47.7748,48.));
#37140=CARTESIAN_POINT('Origin',(39.0062546437124,52.0008,50.5866090189041));
#37141=CARTESIAN_POINT('',(39.3223584999828,47.7748,50.4957436882364));
#37142=CARTESIAN_POINT('',(39.3223584999828,47.1748,50.4957436882364));
#37143=CARTESIAN_POINT('',(39.4795321650532,47.7748,50.450563483169));
#37144=CARTESIAN_POINT('',(39.0062546437124,47.7748,50.5866090189041));
#37145=CARTESIAN_POINT('',(39.4795321650532,52.0008,50.450563483169));
#37146=CARTESIAN_POINT('Origin',(39.4795321650532,52.0008,50.450563483169));
#37147=CARTESIAN_POINT('',(39.4077454283035,47.7748,50.5975038668231));
#37148=CARTESIAN_POINT('',(39.4077454283035,47.1748,50.5975038668231));
#37149=CARTESIAN_POINT('',(39.4795321650532,47.7748,50.450563483169));
#37150=CARTESIAN_POINT('Origin',(39.3071721653514,47.7748,50.5951906953484));
#37151=CARTESIAN_POINT('Origin',(42.4,47.7748,48.));
#37152=CARTESIAN_POINT('Origin',(39.5069732038483,52.0008,51.136630312413));
#37153=CARTESIAN_POINT('',(39.8024961331769,47.7748,50.9922545716966));
#37154=CARTESIAN_POINT('',(39.8024961331769,47.1748,50.9922545716966));
#37155=CARTESIAN_POINT('',(39.949436516831,47.7748,50.9204678349468));
#37156=CARTESIAN_POINT('',(39.5069732038483,47.7748,51.136630312413));
#37157=CARTESIAN_POINT('',(39.949436516831,52.0008,50.9204678349468));
#37158=CARTESIAN_POINT('Origin',(39.949436516831,52.0008,50.9204678349468));
#37159=CARTESIAN_POINT('',(39.9042563117637,47.7748,51.0776415000173));
#37160=CARTESIAN_POINT('',(39.9042563117637,47.1748,51.0776415000173));
#37161=CARTESIAN_POINT('',(39.949436516831,47.7748,50.9204678349468));
#37162=CARTESIAN_POINT('Origin',(39.8048093046516,47.7748,51.0928278346486));
#37163=CARTESIAN_POINT('Origin',(42.4,47.7748,48.));
#37164=CARTESIAN_POINT('Origin',(40.0955949192431,52.0008,51.5913466810908));
#37165=CARTESIAN_POINT('',(40.3615576069641,47.7748,51.3978473141496));
#37166=CARTESIAN_POINT('',(40.3615576069641,47.1748,51.3978473141496));
#37167=CARTESIAN_POINT('',(40.4938,47.7748,51.3016352493878));
#37168=CARTESIAN_POINT('',(40.0955949192431,47.7748,51.5913466810908));
#37169=CARTESIAN_POINT('',(40.4938,52.0008,51.3016352493878));
#37170=CARTESIAN_POINT('Origin',(40.4938,52.0008,51.3016352493878));
#37171=CARTESIAN_POINT('',(40.4765991042837,47.7748,51.4642665535951));
#37172=CARTESIAN_POINT('',(40.4765991042837,47.1748,51.4642665535951));
#37173=CARTESIAN_POINT('',(40.4938,47.7748,51.3016352493878));
#37174=CARTESIAN_POINT('Origin',(40.3813,47.7748,51.4964909652393));
#37175=CARTESIAN_POINT('Origin',(42.4,47.7748,48.));
#37176=CARTESIAN_POINT('Origin',(40.7542348169315,52.0008,51.9369417981727));
#37177=CARTESIAN_POINT('',(40.982556121362,47.7748,51.700198185356));
#37178=CARTESIAN_POINT('',(40.982556121362,47.1748,51.700198185356));
#37179=CARTESIAN_POINT('',(41.0960824055852,47.7748,51.5824841474842));
#37180=CARTESIAN_POINT('',(40.7542348169315,47.7748,51.9369417981727));
#37181=CARTESIAN_POINT('',(41.0960824055852,52.0008,51.5824841474842));
#37182=CARTESIAN_POINT('Origin',(41.0960824055852,52.0008,51.5824841474842));
#37183=CARTESIAN_POINT('',(41.1073834597322,47.7748,51.7456316209454));
#37184=CARTESIAN_POINT('',(41.1073834597322,47.1748,51.7456316209454));
#37185=CARTESIAN_POINT('',(41.0960824055852,47.7748,51.5824841474842));
#37186=CARTESIAN_POINT('Origin',(41.0191278733369,47.7748,51.793914987161));
#37187=CARTESIAN_POINT('Origin',(42.4,47.7748,48.));
#37188=CARTESIAN_POINT('Origin',(41.46288045691,52.0008,52.1629149309059));
#37189=CARTESIAN_POINT('',(41.6466229507512,47.7748,51.8901204070909));
#37190=CARTESIAN_POINT('',(41.6466229507512,47.1748,51.8901204070909));
#37191=CARTESIAN_POINT('',(41.7379836874626,47.7748,51.7544810775837));
#37192=CARTESIAN_POINT('',(41.46288045691,47.7748,52.1629149309059));
#37193=CARTESIAN_POINT('',(41.7379836874626,52.0008,51.7544810775837));
#37194=CARTESIAN_POINT('Origin',(41.7379836874626,52.0008,51.7544810775837));
#37195=CARTESIAN_POINT('',(41.7774433146613,47.7748,51.9131875668744));
#37196=CARTESIAN_POINT('',(41.7774433146613,47.1748,51.9131875668744));
#37197=CARTESIAN_POINT('',(41.7379836874626,47.7748,51.7544810775837));
#37198=CARTESIAN_POINT('Origin',(41.6989128474875,47.7748,51.9760628220115));
#37199=CARTESIAN_POINT('Origin',(42.4,47.7748,48.));
#37200=CARTESIAN_POINT('Origin',(42.2,52.0008,52.2624));
#37201=CARTESIAN_POINT('',(42.3335807605545,47.7748,51.9618432887523));
#37202=CARTESIAN_POINT('',(42.3335807605545,47.1748,51.9618432887523));
#37203=CARTESIAN_POINT('',(42.4,47.7748,51.8124));
#37204=CARTESIAN_POINT('',(42.2,47.7748,52.2624));
#37205=CARTESIAN_POINT('',(42.4,52.0008,51.8124));
#37206=CARTESIAN_POINT('Origin',(42.4,52.0008,51.8124));
#37207=CARTESIAN_POINT('',(42.4664192394455,47.7748,51.9618432887523));
#37208=CARTESIAN_POINT('',(42.4664192394455,47.1748,51.9618432887523));
#37209=CARTESIAN_POINT('',(42.4,47.7748,51.8124));
#37210=CARTESIAN_POINT('Origin',(42.4,47.7748,52.0374));
#37211=CARTESIAN_POINT('Origin',(42.4,47.7748,48.));
#37212=CARTESIAN_POINT('Origin',(42.9431964418851,52.0008,52.2323742019726));
#37213=CARTESIAN_POINT('',(43.0225566853387,47.7748,51.9131875668744));
#37214=CARTESIAN_POINT('',(43.0225566853387,47.1748,51.9131875668744));
#37215=CARTESIAN_POINT('',(43.0620163125374,47.7748,51.7544810775837));
#37216=CARTESIAN_POINT('',(42.9431964418851,47.7748,52.2323742019726));
#37217=CARTESIAN_POINT('',(43.0620163125374,52.0008,51.7544810775837));
#37218=CARTESIAN_POINT('Origin',(43.0620163125374,52.0008,51.7544810775837));
#37219=CARTESIAN_POINT('',(43.1533770492489,47.7748,51.8901204070909));
#37220=CARTESIAN_POINT('',(43.1533770492489,47.1748,51.8901204070909));
#37221=CARTESIAN_POINT('',(43.0620163125374,47.7748,51.7544810775837));
#37222=CARTESIAN_POINT('Origin',(43.1010871525125,47.7748,51.9760628220115));
#37223=CARTESIAN_POINT('Origin',(42.4,47.7748,48.));
#37224=CARTESIAN_POINT('Origin',(43.6698881347541,52.0008,52.073749855503));
#37225=CARTESIAN_POINT('',(43.6926165402678,47.7748,51.7456316209454));
#37226=CARTESIAN_POINT('',(43.6926165402678,47.1748,51.7456316209454));
#37227=CARTESIAN_POINT('',(43.7039175944148,47.7748,51.5824841474842));
#37228=CARTESIAN_POINT('',(43.6698881347541,47.7748,52.073749855503));
#37229=CARTESIAN_POINT('',(43.7039175944148,52.0008,51.5824841474842));
#37230=CARTESIAN_POINT('Origin',(43.7039175944148,52.0008,51.5824841474842));
#37231=CARTESIAN_POINT('',(43.817443878638,47.7748,51.700198185356));
#37232=CARTESIAN_POINT('',(43.817443878638,47.1748,51.700198185356));
#37233=CARTESIAN_POINT('',(43.7039175944148,47.7748,51.5824841474842));
#37234=CARTESIAN_POINT('Origin',(43.7808721266631,47.7748,51.793914987161));
#37235=CARTESIAN_POINT('Origin',(42.4,47.7748,48.));
#37236=CARTESIAN_POINT('Origin',(44.3579949192431,52.0008,51.7913466810908));
#37237=CARTESIAN_POINT('',(44.3234008957163,47.7748,51.4642665535951));
#37238=CARTESIAN_POINT('',(44.3234008957163,47.1748,51.4642665535951));
#37239=CARTESIAN_POINT('',(44.3062,47.7748,51.3016352493878));
#37240=CARTESIAN_POINT('',(44.3579949192431,47.7748,51.7913466810908));
#37241=CARTESIAN_POINT('',(44.3062,52.0008,51.3016352493878));
#37242=CARTESIAN_POINT('Origin',(44.3062,52.0008,51.3016352493878));
#37243=CARTESIAN_POINT('',(44.438442393036,47.7748,51.3978473141496));
#37244=CARTESIAN_POINT('',(44.438442393036,47.1748,51.3978473141496));
#37245=CARTESIAN_POINT('',(44.3062,47.7748,51.3016352493878));
#37246=CARTESIAN_POINT('Origin',(44.4187,47.7748,51.4964909652393));
#37247=CARTESIAN_POINT('Origin',(42.4,47.7748,48.));
#37248=CARTESIAN_POINT('Origin',(44.9866090189041,52.0008,51.3937453562876));
#37249=CARTESIAN_POINT('',(44.8957436882364,47.7748,51.0776415000172));
#37250=CARTESIAN_POINT('',(44.8957436882364,47.1748,51.0776415000172));
#37251=CARTESIAN_POINT('',(44.850563483169,47.7748,50.9204678349468));
#37252=CARTESIAN_POINT('',(44.9866090189041,47.7748,51.3937453562876));
#37253=CARTESIAN_POINT('',(44.850563483169,52.0008,50.9204678349468));
#37254=CARTESIAN_POINT('Origin',(44.850563483169,52.0008,50.9204678349468));
#37255=CARTESIAN_POINT('',(44.9975038668231,47.7748,50.9922545716965));
#37256=CARTESIAN_POINT('',(44.9975038668231,47.1748,50.9922545716965));
#37257=CARTESIAN_POINT('',(44.850563483169,47.7748,50.9204678349468));
#37258=CARTESIAN_POINT('Origin',(44.9951906953484,47.7748,51.0928278346486));
#37259=CARTESIAN_POINT('Origin',(42.4,47.7748,48.));
#37260=CARTESIAN_POINT('Origin',(45.536630312413,52.0008,50.8930267961517));
#37261=CARTESIAN_POINT('',(45.3922545716966,47.7748,50.5975038668231));
#37262=CARTESIAN_POINT('',(45.3922545716966,47.1748,50.5975038668231));
#37263=CARTESIAN_POINT('',(45.3204678349468,47.7748,50.4505634831689));
#37264=CARTESIAN_POINT('',(45.536630312413,47.7748,50.8930267961517));
#37265=CARTESIAN_POINT('',(45.3204678349468,52.0008,50.4505634831689));
#37266=CARTESIAN_POINT('Origin',(45.3204678349468,52.0008,50.4505634831689));
#37267=CARTESIAN_POINT('',(45.4776415000172,47.7748,50.4957436882363));
#37268=CARTESIAN_POINT('',(45.4776415000172,47.1748,50.4957436882363));
#37269=CARTESIAN_POINT('',(45.3204678349468,47.7748,50.4505634831689));
#37270=CARTESIAN_POINT('Origin',(45.4928278346486,47.7748,50.5951906953484));
#37271=CARTESIAN_POINT('Origin',(42.4,47.7748,48.));
#37272=CARTESIAN_POINT('Origin',(45.9913466810908,52.0008,50.3044050807569));
#37273=CARTESIAN_POINT('',(45.7978473141496,47.7748,50.038442393036));
#37274=CARTESIAN_POINT('',(45.7978473141496,47.1748,50.038442393036));
#37275=CARTESIAN_POINT('',(45.7016352493878,47.7748,49.9062));
#37276=CARTESIAN_POINT('',(45.9913466810908,47.7748,50.3044050807569));
#37277=CARTESIAN_POINT('',(45.7016352493878,52.0008,49.9062));
#37278=CARTESIAN_POINT('Origin',(45.7016352493878,52.0008,49.9062));
#37279=CARTESIAN_POINT('',(45.8642665535951,47.7748,49.9234008957163));
#37280=CARTESIAN_POINT('',(45.8642665535951,47.1748,49.9234008957163));
#37281=CARTESIAN_POINT('',(45.7016352493878,47.7748,49.9062));
#37282=CARTESIAN_POINT('Origin',(45.8964909652393,47.7748,50.0187));
#37283=CARTESIAN_POINT('Origin',(42.4,47.7748,48.));
#37284=CARTESIAN_POINT('Origin',(46.3369417981727,52.0008,49.6457651830685));
#37285=CARTESIAN_POINT('',(46.100198185356,47.7748,49.417443878638));
#37286=CARTESIAN_POINT('',(46.100198185356,47.1748,49.417443878638));
#37287=CARTESIAN_POINT('',(45.9824841474842,47.7748,49.3039175944148));
#37288=CARTESIAN_POINT('',(46.3369417981727,47.7748,49.6457651830685));
#37289=CARTESIAN_POINT('',(45.9824841474842,52.0008,49.3039175944148));
#37290=CARTESIAN_POINT('Origin',(45.9824841474842,52.0008,49.3039175944148));
#37291=CARTESIAN_POINT('',(46.1456316209454,47.7748,49.2926165402678));
#37292=CARTESIAN_POINT('',(46.1456316209454,47.1748,49.2926165402678));
#37293=CARTESIAN_POINT('',(45.9824841474842,47.7748,49.3039175944148));
#37294=CARTESIAN_POINT('Origin',(46.193914987161,47.7748,49.3808721266631));
#37295=CARTESIAN_POINT('Origin',(42.4,47.7748,48.));
#37296=CARTESIAN_POINT('Origin',(46.5629149309058,52.0008,48.93711954309));
#37297=CARTESIAN_POINT('',(46.2901204070909,47.7748,48.7533770492488));
#37298=CARTESIAN_POINT('',(46.2901204070909,47.1748,48.7533770492488));
#37299=CARTESIAN_POINT('',(46.1544810775837,47.7748,48.6620163125374));
#37300=CARTESIAN_POINT('',(46.5629149309058,47.7748,48.93711954309));
#37301=CARTESIAN_POINT('',(46.1544810775837,52.0008,48.6620163125374));
#37302=CARTESIAN_POINT('Origin',(46.1544810775837,52.0008,48.6620163125374));
#37303=CARTESIAN_POINT('',(46.3131875668744,47.7748,48.6225566853387));
#37304=CARTESIAN_POINT('',(46.3131875668744,47.1748,48.6225566853387));
#37305=CARTESIAN_POINT('',(46.1544810775837,47.7748,48.6620163125374));
#37306=CARTESIAN_POINT('Origin',(46.3760628220115,47.7748,48.7010871525125));
#37307=CARTESIAN_POINT('Origin',(42.4,47.7748,48.));
#37308=CARTESIAN_POINT('Origin',(46.6624,52.0008,48.2));
#37309=CARTESIAN_POINT('',(46.3618432887523,47.7748,48.0664192394455));
#37310=CARTESIAN_POINT('',(46.3618432887523,47.1748,48.0664192394455));
#37311=CARTESIAN_POINT('',(46.2124,47.7748,48.));
#37312=CARTESIAN_POINT('',(46.6624,47.7748,48.2));
#37313=CARTESIAN_POINT('',(46.2124,52.0008,48.));
#37314=CARTESIAN_POINT('Origin',(46.2124,52.0008,48.));
#37315=CARTESIAN_POINT('',(46.3618432887523,47.7748,47.9335807605545));
#37316=CARTESIAN_POINT('',(46.3618432887523,47.1748,47.9335807605545));
#37317=CARTESIAN_POINT('',(46.2124,47.7748,48.));
#37318=CARTESIAN_POINT('Origin',(46.4374,47.7748,48.));
#37319=CARTESIAN_POINT('Origin',(42.4,47.7748,48.));
#37320=CARTESIAN_POINT('Origin',(42.4,47.1748,48.));
#37321=CARTESIAN_POINT('',(38.4376,47.1748,48.));
#37322=CARTESIAN_POINT('Origin',(42.4,52.0008,48.));
#37323=CARTESIAN_POINT('',(40.1086411191537,52.0008,48.));
#37324=CARTESIAN_POINT('',(41.2543205595768,52.0008,46.015625));
#37325=CARTESIAN_POINT('',(40.3950609792595,52.0008,47.50390625));
#37326=CARTESIAN_POINT('',(43.5456794404232,52.0008,46.015625));
#37327=CARTESIAN_POINT('',(41.8271602797884,52.0008,46.015625));
#37328=CARTESIAN_POINT('',(44.6913588808463,52.0008,48.));
#37329=CARTESIAN_POINT('',(43.832099300529,52.0008,46.51171875));
#37330=CARTESIAN_POINT('',(43.5456794404232,52.0008,49.984375));
#37331=CARTESIAN_POINT('',(44.4049390207405,52.0008,48.49609375));
#37332=CARTESIAN_POINT('',(41.2543205595768,52.0008,49.984375));
#37333=CARTESIAN_POINT('',(42.9728397202116,52.0008,49.984375));
#37334=CARTESIAN_POINT('',(40.967900699471,52.0008,49.48828125));
#37335=CARTESIAN_POINT('Origin',(44.6913588808463,49.6008,48.));
#37336=CARTESIAN_POINT('',(40.1086411191537,49.6008,48.));
#37337=CARTESIAN_POINT('',(41.2543205595768,49.6008,46.015625));
#37338=CARTESIAN_POINT('',(40.1086411191537,49.6008,48.));
#37339=CARTESIAN_POINT('Origin',(42.4,49.6008,48.));
#37340=CARTESIAN_POINT('Origin',(44.6913588808463,49.6008,48.));
#37341=CARTESIAN_POINT('',(43.5456794404232,49.6008,46.015625));
#37342=CARTESIAN_POINT('',(41.2543205595768,49.6008,46.015625));
#37343=CARTESIAN_POINT('Origin',(42.4,49.6008,48.));
#37344=CARTESIAN_POINT('Origin',(44.6913588808463,49.6008,48.));
#37345=CARTESIAN_POINT('',(44.6913588808463,49.6008,48.));
#37346=CARTESIAN_POINT('',(43.5456794404232,49.6008,46.015625));
#37347=CARTESIAN_POINT('Origin',(42.4,49.6008,48.));
#37348=CARTESIAN_POINT('Origin',(44.6913588808463,49.6008,48.));
#37349=CARTESIAN_POINT('',(43.5456794404232,49.6008,49.984375));
#37350=CARTESIAN_POINT('',(44.6913588808463,49.6008,48.));
#37351=CARTESIAN_POINT('Origin',(42.4,49.6008,48.));
#37352=CARTESIAN_POINT('Origin',(44.6913588808463,49.6008,48.));
#37353=CARTESIAN_POINT('',(41.2543205595768,49.6008,49.984375));
#37354=CARTESIAN_POINT('',(43.5456794404232,49.6008,49.984375));
#37355=CARTESIAN_POINT('Origin',(42.4,49.6008,48.));
#37356=CARTESIAN_POINT('Origin',(44.6913588808463,49.6008,48.));
#37357=CARTESIAN_POINT('',(41.2543205595768,49.6008,49.984375));
#37358=CARTESIAN_POINT('Origin',(42.4,49.6008,48.));
#37359=CARTESIAN_POINT('Origin',(42.4,49.6008,48.));
#37360=CARTESIAN_POINT('',(42.4,48.2240126844404,48.));
#37361=CARTESIAN_POINT('',(40.1086411191537,49.6008,48.));
#37362=CARTESIAN_POINT('Origin',(40.1086411191537,52.0008,48.));
#37363=CARTESIAN_POINT('',(40.1086411191537,52.0008,48.));
#37364=CARTESIAN_POINT('',(41.2543205595768,52.0008,46.015625));
#37365=CARTESIAN_POINT('Origin',(41.2543205595768,52.0008,49.984375));
#37366=CARTESIAN_POINT('',(41.2543205595768,52.0008,49.984375));
#37367=CARTESIAN_POINT('Origin',(43.5456794404232,52.0008,49.984375));
#37368=CARTESIAN_POINT('',(43.5456794404232,52.0008,49.984375));
#37369=CARTESIAN_POINT('Origin',(44.6913588808463,52.0008,48.));
#37370=CARTESIAN_POINT('',(44.6913588808463,52.0008,48.));
#37371=CARTESIAN_POINT('Origin',(43.5456794404232,52.0008,46.015625));
#37372=CARTESIAN_POINT('',(43.5456794404232,52.0008,46.015625));
#37373=CARTESIAN_POINT('Origin',(41.2543205595768,52.0008,46.015625));
#71780=UNCERTAINTY_MEASURE_WITH_UNIT(LENGTH_MEASURE(0.01),#71796,
'DISTANCE_ACCURACY_VALUE',
'Maximum model space distance between geometric entities at asserted c
onnectivities');
#71783=UNCERTAINTY_MEASURE_WITH_UNIT(LENGTH_MEASURE(0.01),#71796,
'DISTANCE_ACCURACY_VALUE',
'Maximum model space distance between geometric entities at asserted c
onnectivities');
#71792=(
GEOMETRIC_REPRESENTATION_CONTEXT(3)
GLOBAL_UNCERTAINTY_ASSIGNED_CONTEXT((#71780))
GLOBAL_UNIT_ASSIGNED_CONTEXT((#71796,#71798,#71799))
REPRESENTATION_CONTEXT('','3D')
);
#71795=(
GEOMETRIC_REPRESENTATION_CONTEXT(3)
GLOBAL_UNCERTAINTY_ASSIGNED_CONTEXT((#71783))
GLOBAL_UNIT_ASSIGNED_CONTEXT((#71796,#71798,#71799))
REPRESENTATION_CONTEXT('','3D')
);
#71796=(
LENGTH_UNIT()
NAMED_UNIT(*)
SI_UNIT(.MILLI.,.METRE.)
);
#71798=(
NAMED_UNIT(*)
PLANE_ANGLE_UNIT()
SI_UNIT($,.RADIAN.)
);
#71799=(
NAMED_UNIT(*)
SI_UNIT($,.STERADIAN.)
SOLID_ANGLE_UNIT()
);
#71808=SHAPE_DEFINITION_REPRESENTATION(#71819,#72024);
#71819=PRODUCT_DEFINITION_SHAPE('',$,#72036);
#72024=SHAPE_REPRESENTATION('',(#14114),#71792);
#72027=PRODUCT_DEFINITION_CONTEXT('part definition',#72062,'design');
#72036=PRODUCT_DEFINITION('ASME B18.3 SHCS 10-32 UNF x 0.625',
'ASME B18.3 SHCS 10-32 UNF x 0.625',#72047,#72027);
#72047=PRODUCT_DEFINITION_FORMATION('',$,#72072);
#72062=APPLICATION_CONTEXT(
'Core Data for Automotive Mechanical Design Process');
#72063=PRODUCT_CONTEXT('part definition',#72062,'mechanical');
#72072=PRODUCT('ASME B18.3 SHCS 10-32 UNF x 0.625',
'ASME B18.3 SHCS 10-32 UNF x 0.625',$,(#72063));
#72083=PRESENTATION_STYLE_ASSIGNMENT((#72094));
#72094=SURFACE_STYLE_USAGE(.BOTH.,#72105);
#72105=SURFACE_SIDE_STYLE('',(#72116));
#72116=SURFACE_STYLE_FILL_AREA(#72127);
#72127=FILL_AREA_STYLE('Opaque(199,204,210)',(#72138));
#72138=FILL_AREA_STYLE_COLOUR('Opaque(199,204,210)',#72149);
#72149=COLOUR_RGB('Opaque(199,204,210)', 0.66274510, 0.83137255, 0.94901961);
ENDSEC;
END-ISO-10303-21;
